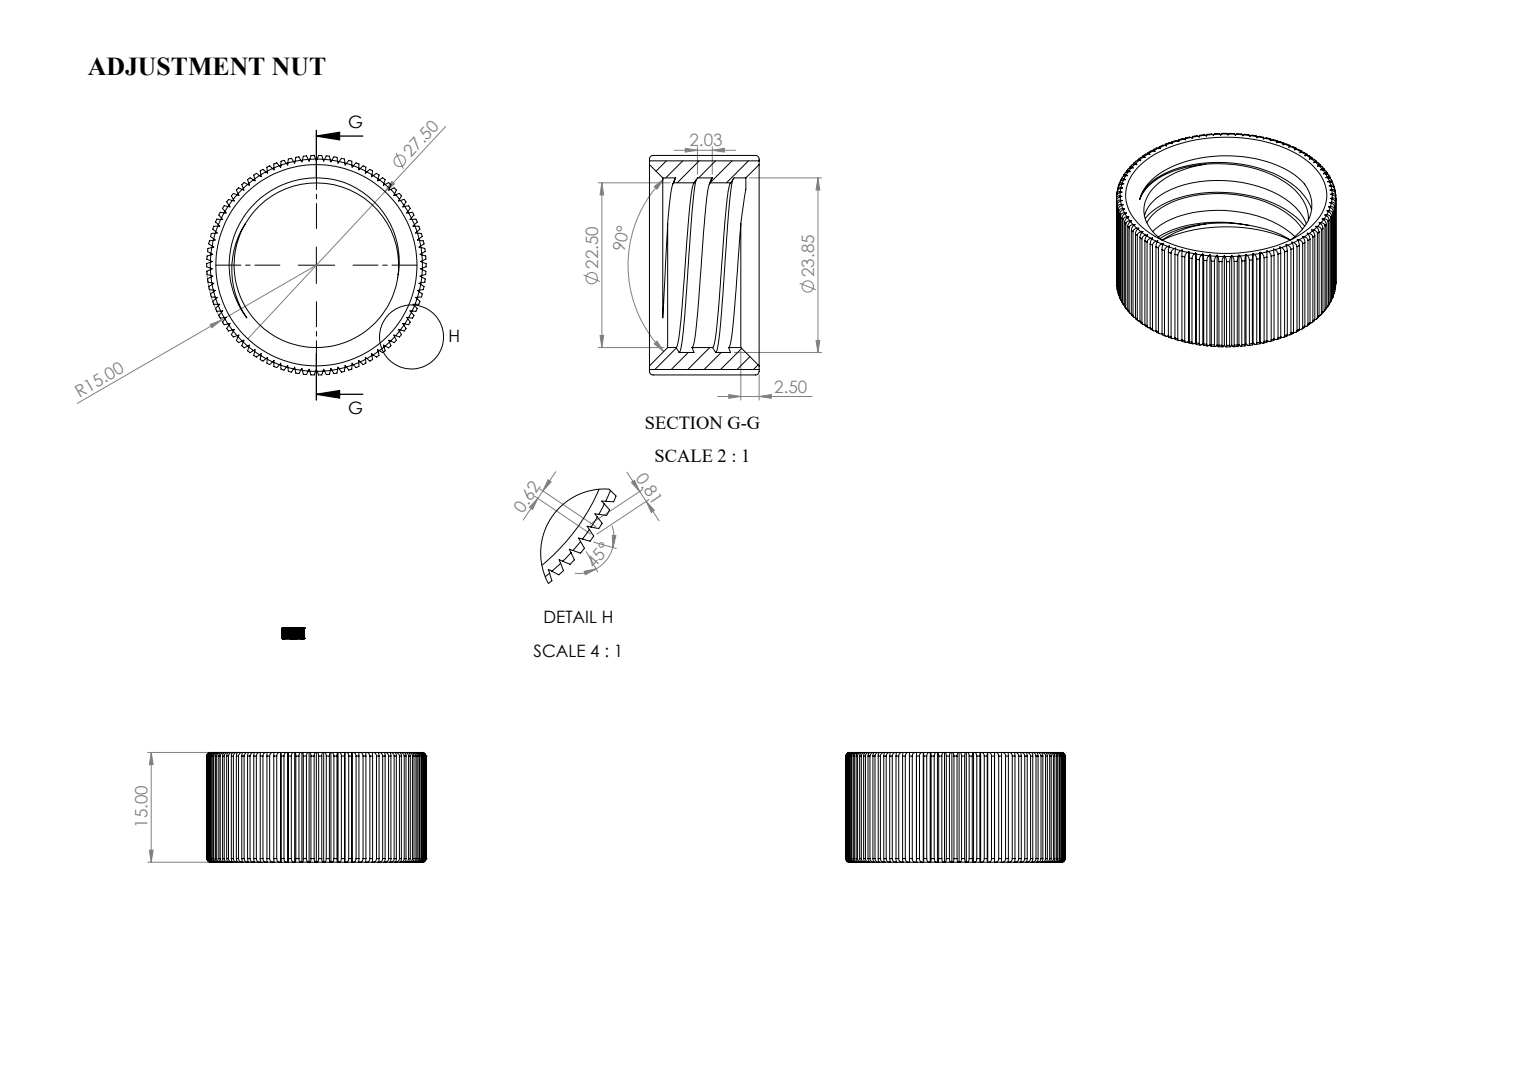
ISO-10303-21;
HEADER;
FILE_DESCRIPTION (('STEP AP214'),
    '1' );
FILE_NAME ('1.3 Adjustment Nut.step',
    '2026-10-07T05:30:18',
    ( '' ),
    ( '' ),
    'SwSTEP 2.0',
    'SolidWorks 2021',
    '' );
FILE_SCHEMA (( 'AUTOMOTIVE_DESIGN' ));
ENDSEC;

DATA;
#2=CARTESIAN_POINT ( 'NONE',  ( 14.03351048042397231, -0.03417435944610275333, -2.474486531753715024 ) ) ;
#4=CARTESIAN_POINT ( 'NONE',  ( 14.71525861348289865, 0.5000000000000004441, -2.908807992686582633 ) ) ;
#7=B_SPLINE_CURVE_WITH_KNOTS ( 'NONE', 3,
 ( #85792, #56757, #94261, #25787, #71286, #3780 ),
 .UNSPECIFIED., .F., .F.,
 ( 4, 2, 4 ),
 ( 0.0002800003243993068715, 0.0006862055569927260918, 0.001092410789586145421 ),
 .UNSPECIFIED. ) ;
#8=CARTESIAN_POINT ( 'NONE',  ( 7.082119434687054849, -1.529584498419354954, 12.26659068614894288 ) ) ;
#12=ORIENTED_EDGE ( 'NONE', *, *, #89075, .F. ) ;
#15=CARTESIAN_POINT ( 'NONE',  ( 1.915564264621432589, 3.914659629196372862E-16, -14.37291249357990530 ) ) ;
#20=DIRECTION ( 'NONE',  ( -0.000000000000000000, 1.000000000000000000, -0.000000000000000000 ) ) ;
#24=CARTESIAN_POINT ( 'NONE',  ( -10.88017736071110342, 33.06368534415485527, 3.903127820947815962E-15 ) ) ;
#31=ORIENTED_EDGE ( 'NONE', *, *, #54443, .T. ) ;
#32=EDGE_CURVE ( 'NONE', #89546, #61124, #1756, .T. ) ;
#33=VECTOR ( 'NONE', #15415, 1000.000000000000114 ) ;
#36=CARTESIAN_POINT ( 'NONE',  ( 0.000000000000000000, 0.000000000000000000, 0.000000000000000000 ) ) ;
#44=ORIENTED_EDGE ( 'NONE', *, *, #85385, .F. ) ;
#55=CARTESIAN_POINT ( 'NONE',  ( 5.361923921558577000, 0.000000000000000000, -0.9937738586171993571 ) ) ;
#57=CARTESIAN_POINT ( 'NONE',  ( -14.09394518620607606, 3.895088541583166744E-16, -3.407449058785548157 ) ) ;
#59=CARTESIAN_POINT ( 'NONE',  ( -14.35840480524194440, 15.00000000000000000, -4.340070442839038201 ) ) ;
#67=LINE ( 'NONE', #92990, #97116 ) ;
#68=FACE_OUTER_BOUND ( 'NONE', #36092, .T. ) ;
#73=ADVANCED_FACE ( 'NONE', ( #77721, #92241 ), #62222, .F. ) ;
#77=CARTESIAN_POINT ( 'NONE',  ( 8.527530157486175710, 13.92559781766745886, -4.923371831947298993 ) ) ;
#79=CARTESIAN_POINT ( 'NONE',  ( -6.715867195167276371, 15.00000000000000000, -12.85095824508335838 ) ) ;
#80=ORIENTED_EDGE ( 'NONE', *, *, #34109, .F. ) ;
#93=ORIENTED_EDGE ( 'NONE', *, *, #11884, .T. ) ;
#101=CIRCLE ( 'NONE', #95854, 15.00000000000000000 ) ;
#112=DIRECTION ( 'NONE',  ( 0.000000000000000000, 1.000000000000000000, 0.000000000000000000 ) ) ;
#117=CARTESIAN_POINT ( 'NONE',  ( -10.32896413005679648, 5.104976035794177136, 5.963430220938290560 ) ) ;
#127=ORIENTED_EDGE ( 'NONE', *, *, #93931, .T. ) ;
#135=DIRECTION ( 'NONE',  ( 0.000000000000000000, 0.000000000000000000, -1.000000000000000000 ) ) ;
#139=CARTESIAN_POINT ( 'NONE',  ( -10.88017736071110342, -6.936314655845155386, 3.903127820947815962E-15 ) ) ;
#141=CARTESIAN_POINT ( 'NONE',  ( 13.59972906620400401, 0.04962881387626714991, -5.718800721548577215 ) ) ;
#143=CARTESIAN_POINT ( 'NONE',  ( 11.29222593019770393, 14.76930270348882068, 9.783848334571327854 ) ) ;
#145=CARTESIAN_POINT ( 'NONE',  ( 1.460619146402132233E-15, 35.00000000000000000, 11.92686044187656513 ) ) ;
#154=AXIS2_PLACEMENT_3D ( 'NONE', #61355, #15392, #78324 ) ;
#166=DIRECTION ( 'NONE',  ( 0.000000000000000000, 1.000000000000000000, 0.000000000000000000 ) ) ;
#169=ORIENTED_EDGE ( 'NONE', *, *, #60294, .T. ) ;
#172=ADVANCED_FACE ( 'NONE', ( #58883 ), #90560, .T. ) ;
#181=LINE ( 'NONE', #61621, #10834 ) ;
#184=CARTESIAN_POINT ( 'NONE',  ( -8.527530157486182816, -29.40773551566588040, -4.923371831947288335 ) ) ;
#186=CARTESIAN_POINT ( 'NONE',  ( 0.2074183518478781019, 14.95123636042159454, -14.75075219811622773 ) ) ;
#187=CARTESIAN_POINT ( 'NONE',  ( 0.7375392941517235901, 0.5000000000000004441, 14.98185688723471110 ) ) ;
#189=VERTEX_POINT ( 'NONE', #73386 ) ;
#190=CARTESIAN_POINT ( 'NONE',  ( -0.8653096853335169314, -2.832054659144752395E-15, 14.59999144042650521 ) ) ;
#198=CARTESIAN_POINT ( 'NONE',  ( 12.81628187352647608, 21.41530133659708923, 3.434112377981052511 ) ) ;
#203=ORIENTED_EDGE ( 'NONE', *, *, #30154, .T. ) ;
#205=EDGE_CURVE ( 'NONE', #59600, #64703, #44234, .T. ) ;
#213=EDGE_CURVE ( 'NONE', #70990, #82368, #80902, .T. ) ;
#217=CARTESIAN_POINT ( 'NONE',  ( 0.7375392941518293943, 15.00000000000000000, -14.98185688723470932 ) ) ;
#219=CARTESIAN_POINT ( 'NONE',  ( -9.010802615327746068, 0.2301505768537817076, -11.91753657575794811 ) ) ;
#220=ORIENTED_EDGE ( 'NONE', *, *, #48530, .T. ) ;
#226=CARTESIAN_POINT ( 'NONE',  ( 0.000000000000000000, 15.00000000000000000, 0.000000000000000000 ) ) ;
#227=CARTESIAN_POINT ( 'NONE',  ( -14.15281240980449873, -3.182726299308032341E-15, 3.688687068602606089 ) ) ;
#230=DIRECTION ( 'NONE',  ( 0.000000000000000000, 1.000000000000000000, 0.000000000000000000 ) ) ;
#234=LINE ( 'NONE', #46200, #73516 ) ;
#241=DIRECTION ( 'NONE',  ( -0.2164396139381037087, 0.000000000000000000, 0.9762960071199331402 ) ) ;
#243=VERTEX_POINT ( 'NONE', #19901 ) ;
#248=LINE ( 'NONE', #13741, #50377 ) ;
#255=CARTESIAN_POINT ( 'NONE',  ( 14.16423886937410437, 14.09541550158063750, 3.795296366450304770 ) ) ;
#259=CARTESIAN_POINT ( 'NONE',  ( -10.17177286909477552, 0.2301502795151870728, 10.94336654633674399 ) ) ;
#260=AXIS2_PLACEMENT_3D ( 'NONE', #53452, #62422, #47430 ) ;
#264=B_SPLINE_CURVE_WITH_KNOTS ( 'NONE', 3,
 ( #34760, #66749, #89251, #97273, #64755, #95267 ),
 .UNSPECIFIED., .F., .F.,
 ( 4, 2, 4 ),
 ( 3.409110551496085967E-05, 0.0004400426677367861379, 0.0008459942299586114840 ),
 .UNSPECIFIED. ) ;
#269=ORIENTED_EDGE ( 'NONE', *, *, #30362, .T. ) ;
#275=CARTESIAN_POINT ( 'NONE',  ( -11.49658347684029813, 0.04962891477616592634, 9.245857368719700986 ) ) ;
#279=EDGE_LOOP ( 'NONE', ( #9235, #51853, #64977, #5678 ) ) ;
#282=CARTESIAN_POINT ( 'NONE',  ( 5.795997163830076460, -0.03417435944610275333, 13.01802277140709663 ) ) ;
#285=DIRECTION ( 'NONE',  ( -0.9999619230641714207, 0.000000000000000000, 0.008726535498367550894 ) ) ;
#290=CARTESIAN_POINT ( 'NONE',  ( 5.817157072110707539, 0.3640475087720986824, 13.82608706751091532 ) ) ;
#294=AXIS2_PLACEMENT_3D ( 'NONE', #67632, #98653, #53107 ) ;
#296=ORIENTED_EDGE ( 'NONE', *, *, #42464, .F. ) ;
#297=CARTESIAN_POINT ( 'NONE',  ( -14.73551000134586353, 0.04962893459885742153, 0.7225335126796733620 ) ) ;
#311=EDGE_CURVE ( 'NONE', #38139, #1776, #53773, .T. ) ;
#315=AXIS2_PLACEMENT_3D ( 'NONE', #61065, #112, #24072 ) ;
#316=ORIENTED_EDGE ( 'NONE', *, *, #50365, .T. ) ;
#318=ORIENTED_EDGE ( 'NONE', *, *, #77420, .F. ) ;
#323=ORIENTED_EDGE ( 'NONE', *, *, #6440, .F. ) ;
#325=VERTEX_POINT ( 'NONE', #97886 ) ;
#334=DIRECTION ( 'NONE',  ( -0.000000000000000000, -1.000000000000000000, -0.000000000000000000 ) ) ;
#339=VERTEX_POINT ( 'NONE', #7364 ) ;
#344=CARTESIAN_POINT ( 'NONE',  ( 7.684764310694891520, 14.49999999999999112, -12.88194075009941564 ) ) ;
#357=CARTESIAN_POINT ( 'NONE',  ( 12.21130863673200473, -3.098870037529856607E-15, 8.049375889233058246 ) ) ;
#364=CARTESIAN_POINT ( 'NONE',  ( -0.7575892234029697470, 0.2306972965111908358, -14.92193396517714099 ) ) ;
#368=EDGE_CURVE ( 'NONE', #36285, #1044, #68358, .T. ) ;
#370=B_SPLINE_CURVE_WITH_KNOTS ( 'NONE', 3,
 ( #59553, #52060, #6070, #61027, #30031, #36570 ),
 .UNSPECIFIED., .F., .F.,
 ( 4, 2, 4 ),
 ( 0.0002800267093156125989, 0.0006862322000234134670, 0.001092437690731214335 ),
 .UNSPECIFIED. ) ;
#373=CIRCLE ( 'NONE', #80196, 14.49999999999999822 ) ;
#380=PLANE ( 'NONE',  #76873 ) ;
#382=DIRECTION ( 'NONE',  ( 0.000000000000000000, 0.000000000000000000, 1.000000000000000000 ) ) ;
#389=EDGE_CURVE ( 'NONE', #33071, #18961, #10309, .T. ) ;
#392=DIRECTION ( 'NONE',  ( -0.9170600743851266001, 0.000000000000000000, 0.3987490689252404796 ) ) ;
#399=DIRECTION ( 'NONE',  ( 0.8870108331782213806, 0.000000000000000000, -0.4617486132350345773 ) ) ;
#405=LINE ( 'NONE', #8848, #3141 ) ;
#411=DIRECTION ( 'NONE',  ( 0.9537169507482300412, 0.000000000000000000, -0.3007057995042635157 ) ) ;
#414=AXIS2_PLACEMENT_3D ( 'NONE', #78877, #40404, #49357 ) ;
#436=ORIENTED_EDGE ( 'NONE', *, *, #19518, .T. ) ;
#438=CARTESIAN_POINT ( 'NONE',  ( 4.096035146093440993, 4.852245006323173772E-16, 13.90943910019262120 ) ) ;
#441=DIRECTION ( 'NONE',  ( -0.2503800040544453820, 0.000000000000000000, 0.9681476403781066331 ) ) ;
#443=CARTESIAN_POINT ( 'NONE',  ( 0.000000000000000000, 0.000000000000000000, 0.000000000000000000 ) ) ;
#446=AXIS2_PLACEMENT_3D ( 'NONE', #98952, #30408, #60911 ) ;
#460=EDGE_LOOP ( 'NONE', ( #79001, #10921, #93802, #41323 ) ) ;
#471=DIRECTION ( 'NONE',  ( 0.9537169507482238240, 0.000000000000000000, 0.3007057995042832221 ) ) ;
#483=CARTESIAN_POINT ( 'NONE',  ( -10.96178847474192075, 12.64502661508361214, -3.125209426587095329 ) ) ;
#489=CARTESIAN_POINT ( 'NONE',  ( -9.705452947461466806, 12.49999999999999289, -5.689172442861226031 ) ) ;
#492=EDGE_CURVE ( 'NONE', #47923, #47609, #86304, .T. ) ;
#501=CARTESIAN_POINT ( 'NONE',  ( 7.082119434687054849, -6.529584498419358951, 12.26659068614894288 ) ) ;
#502=VECTOR ( 'NONE', #65777, 1000.000000000000114 ) ;
#505=EDGE_CURVE ( 'NONE', #98966, #86629, #49108, .T. ) ;
#509=VECTOR ( 'NONE', #13114, 1000.000000000000000 ) ;
#512=CARTESIAN_POINT ( 'NONE',  ( 1.881645754503864953, -2.851112900457974152E-15, -14.50406564081096406 ) ) ;
#518=CARTESIAN_POINT ( 'NONE',  ( -6.728956594450633766, -2.083701050245576615E-16, -12.98689685418151640 ) ) ;
#527=CARTESIAN_POINT ( 'NONE',  ( 0.000000000000000000, 0.000000000000000000, 0.000000000000000000 ) ) ;
#536=CARTESIAN_POINT ( 'NONE',  ( 13.30119215211282047, 0.2301510699511992164, -6.804450086557198851 ) ) ;
#543=EDGE_CURVE ( 'NONE', #1556, #53389, #1840, .T. ) ;
#544=AXIS2_PLACEMENT_3D ( 'NONE', #93741, #61758, #9760 ) ;
#553=EDGE_CURVE ( 'NONE', #69641, #95502, #9313, .T. ) ;
#563=DIRECTION ( 'NONE',  ( -8.881784197001252323E-16, 0.000000000000000000, 1.000000000000000000 ) ) ;
#568=LINE ( 'NONE', #15061, #79560 ) ;
#571=CARTESIAN_POINT ( 'NONE',  ( -3.434112377981067610, -41.91803199673623936, -12.81628187352647252 ) ) ;
#572=ORIENTED_EDGE ( 'NONE', *, *, #57066, .F. ) ;
#574=ORIENTED_EDGE ( 'NONE', *, *, #38436, .F. ) ;
#584=AXIS2_PLACEMENT_3D ( 'NONE', #70041, #3034, #55528 ) ;
#587=VERTEX_POINT ( 'NONE', #25325 ) ;
#590=ORIENTED_EDGE ( 'NONE', *, *, #95067, .T. ) ;
#594=ADVANCED_FACE ( 'NONE', ( #47799 ), #2628, .T. ) ;
#602=ORIENTED_EDGE ( 'NONE', *, *, #96478, .F. ) ;
#604=ORIENTED_EDGE ( 'NONE', *, *, #21453, .F. ) ;
#605=ORIENTED_EDGE ( 'NONE', *, *, #79248, .F. ) ;
#606=CARTESIAN_POINT ( 'NONE',  ( -2.261421327065782805, 0.000000000000000000, 4.962236210031227834 ) ) ;
#607=CARTESIAN_POINT ( 'NONE',  ( 15.99538290524656503, 15.00000000000000000, 0.1584996864329874799 ) ) ;
#618=PLANE ( 'NONE',  #88836 ) ;
#623=ORIENTED_EDGE ( 'NONE', *, *, #11453, .T. ) ;
#630=DIRECTION ( 'NONE',  ( 0.000000000000000000, 1.000000000000000000, 0.000000000000000000 ) ) ;
#632=CARTESIAN_POINT ( 'NONE',  ( 7.313705784284644906, 14.49999999999999112, -13.09617149020747817 ) ) ;
#636=CARTESIAN_POINT ( 'NONE',  ( 5.440088680355549045, -8.602981322511817908, -9.422509992056141925 ) ) ;
#639=DIRECTION ( 'NONE',  ( 0.000000000000000000, 0.000000000000000000, 1.000000000000000000 ) ) ;
#640=CARTESIAN_POINT ( 'NONE',  ( -14.62617646268086524, 0.3639308321805994062, -3.327906561567071986 ) ) ;
#649=DIRECTION ( 'NONE',  ( 0.000000000000000000, 1.000000000000000000, 0.000000000000000000 ) ) ;
#675=CARTESIAN_POINT ( 'NONE',  ( -8.606322355891443010, 15.00000000000000000, 11.66967075398801335 ) ) ;
#678=CARTESIAN_POINT ( 'NONE',  ( -4.923371831947292776, -8.157735515665876846, 8.527530157486181039 ) ) ;
#691=CARTESIAN_POINT ( 'NONE',  ( 12.81628187352647608, 26.62363466993042493, -2.602085213965210642E-15 ) ) ;
#696=EDGE_LOOP ( 'NONE', ( #40227, #25908, #8282, #49239, #90855, #86389 ) ) ;
#704=EDGE_CURVE ( 'NONE', #20604, #37674, #29970, .T. ) ;
#705=CARTESIAN_POINT ( 'NONE',  ( 0.000000000000000000, 14.49999999999999822, 0.000000000000000000 ) ) ;
#706=CARTESIAN_POINT ( 'NONE',  ( -14.35840480524201190, 14.49999999999999112, -4.340070442839034648 ) ) ;
#712=CARTESIAN_POINT ( 'NONE',  ( -15.94536257719939698, 15.00000000000000000, -1.273895096820171657 ) ) ;
#714=AXIS2_PLACEMENT_3D ( 'NONE', #93061, #56067, #79045 ) ;
#719=CARTESIAN_POINT ( 'NONE',  ( -11.59580422753514384, 14.76984949557107640, -9.421229451860563486 ) ) ;
#723=FACE_OUTER_BOUND ( 'NONE', #60066, .T. ) ;
#735=CARTESIAN_POINT ( 'NONE',  ( 14.82269085861167390, 14.49999999999999822, 2.299529454047062327 ) ) ;
#741=CARTESIAN_POINT ( 'NONE',  ( 3.195792623639593266, 4.120456701841152203, 11.92686044187653494 ) ) ;
#746=CARTESIAN_POINT ( 'NONE',  ( 14.16423886937410082, 19.51208216824730712, -3.795296366450314096 ) ) ;
#749=CARTESIAN_POINT ( 'NONE',  ( 3.270351084886796933, 14.95037111082768000, -14.38617789677962655 ) ) ;
#755=DIRECTION ( 'NONE',  ( -0.000000000000000000, -1.000000000000000000, -0.000000000000000000 ) ) ;
#756=ORIENTED_EDGE ( 'NONE', *, *, #56154, .F. ) ;
#765=VERTEX_POINT ( 'NONE', #66241 ) ;
#781=CARTESIAN_POINT ( 'NONE',  ( 14.03351048042397231, 0.000000000000000000, -2.474486531753715024 ) ) ;
#787=LINE ( 'NONE', #31240, #15154 ) ;
#792=AXIS2_PLACEMENT_3D ( 'NONE', #36008, #73504, #34024 ) ;
#797=LINE ( 'NONE', #31249, #42721 ) ;
#798=ORIENTED_EDGE ( 'NONE', *, *, #95058, .F. ) ;
#804=CARTESIAN_POINT ( 'NONE',  ( -5.803070148808146200, 15.00000000000000000, -13.28812917035395813 ) ) ;
#807=CARTESIAN_POINT ( 'NONE',  ( 2.602060718268849104, 0.000000000000000000, -4.792399674598859072 ) ) ;
#808=VECTOR ( 'NONE', #6367, 1000.000000000000000 ) ;
#811=FACE_OUTER_BOUND ( 'NONE', #83164, .T. ) ;
#819=B_SPLINE_CURVE_WITH_KNOTS ( 'NONE', 3,
 ( #42826, #41374, #64319, #73311, #4834, #33813 ),
 .UNSPECIFIED., .F., .F.,
 ( 4, 2, 4 ),
 ( 0.0002800005319459006065, 0.0006862057665691816740, 0.001092411001192462741 ),
 .UNSPECIFIED. ) ;
#850=DIRECTION ( 'NONE',  ( 0.5664062369248313855, 0.000000000000000000, -0.8241261886220165866 ) ) ;
#853=CARTESIAN_POINT ( 'NONE',  ( 14.29730467489532408, 4.491438197698105257E-16, 2.416004766803315995 ) ) ;
#857=DIRECTION ( 'NONE',  ( 0.000000000000000000, 0.000000000000000000, 1.000000000000000000 ) ) ;
#858=CARTESIAN_POINT ( 'NONE',  ( 6.742022620658236320, 0.04962897188439623769, -13.12259272460504533 ) ) ;
#864=DIRECTION ( 'NONE',  ( 0.000000000000000000, 1.000000000000000000, -0.000000000000000000 ) ) ;
#865=STYLED_ITEM ( 'NONE', ( #71034 ), #8224 ) ;
#877=CARTESIAN_POINT ( 'NONE',  ( -14.93875075227008509, 0.2301502577613187550, -0.2365588874161651534 ) ) ;
#882=CARTESIAN_POINT ( 'NONE',  ( 9.519554572442958218, 15.00000000000000178, -11.10344954678180329 ) ) ;
#887=DIRECTION ( 'NONE',  ( 0.1650476058606741014, 0.000000000000000000, 0.9862856015372319929 ) ) ;
#907=ORIENTED_EDGE ( 'NONE', *, *, #41162, .F. ) ;
#921=ORIENTED_EDGE ( 'NONE', *, *, #98148, .F. ) ;
#930=EDGE_CURVE ( 'NONE', #78202, #91469, #93678, .T. ) ;
#931=AXIS2_PLACEMENT_3D ( 'NONE', #97642, #90596, #92936 ) ;
#933=CARTESIAN_POINT ( 'NONE',  ( -9.876730923139145801, 0.5000000000000004441, -11.28938378619076843 ) ) ;
#934=EDGE_CURVE ( 'NONE', #70902, #7776, #71189, .T. ) ;
#935=VERTEX_POINT ( 'NONE', #12147 ) ;
#949=CARTESIAN_POINT ( 'NONE',  ( 12.25993886608599759, 0.3640475087720986269, 8.642563219313707634 ) ) ;
#952=VERTEX_POINT ( 'NONE', #4168 ) ;
#953=CARTESIAN_POINT ( 'NONE',  ( 2.863771337576527021, 0.04962896698837649528, -14.47259902956229283 ) ) ;
#960=ADVANCED_FACE ( 'NONE', ( #34637 ), #97527, .T. ) ;
#966=CARTESIAN_POINT ( 'NONE',  ( -8.235571585149862983, 10.74303362898264602, 8.235571585149875418 ) ) ;
#975=CARTESIAN_POINT ( 'NONE',  ( 14.16423886937410082, -5.487917831752695541, -3.795296366450314096 ) ) ;
#984=CARTESIAN_POINT ( 'NONE',  ( 0.000000000000000000, 15.00000000000000000, -11.25000000000000178 ) ) ;
#986=CARTESIAN_POINT ( 'NONE',  ( 7.154372922009559765, -0.03417435944610275333, -14.30707323420376831 ) ) ;
#1000=DIRECTION ( 'NONE',  ( -0.9426414910921759871, 0.000000000000000000, -0.3338068592337775642 ) ) ;
#1010=CARTESIAN_POINT ( 'NONE',  ( 13.16767742306216604, 0.04962884061926501472, -6.653539137814636462 ) ) ;
#1011=CARTESIAN_POINT ( 'NONE',  ( 0.000000000000000000, 0.000000000000000000, 0.000000000000000000 ) ) ;
#1013=ORIENTED_EDGE ( 'NONE', *, *, #57799, .T. ) ;
#1021=DIRECTION ( 'NONE',  ( -0.02617694830787627158, 0.000000000000000000, 0.9996573249755572599 ) ) ;
#1023=VERTEX_POINT ( 'NONE', #50645 ) ;
#1024=CIRCLE ( 'NONE', #98383, 15.00000000000000000 ) ;
#1027=LINE ( 'NONE', #92490, #16884 ) ;
#1042=CARTESIAN_POINT ( 'NONE',  ( -4.923371831947302546, 30.17559781766745886, -8.527530157486173934 ) ) ;
#1043=EDGE_LOOP ( 'NONE', ( #66084, #36581, #93814, #49851, #67190, #80121 ) ) ;
#1044=VERTEX_POINT ( 'NONE', #73627 ) ;
#1052=ORIENTED_EDGE ( 'NONE', *, *, #1534, .F. ) ;
#1057=EDGE_LOOP ( 'NONE', ( #46401, #67806, #92729, #95178, #5184, #32431 ) ) ;
#1062=B_SPLINE_CURVE_WITH_KNOTS ( 'NONE', 3,
 ( #33138, #63633, #11628, #71651, #19621, #50115 ),
 .UNSPECIFIED., .F., .F.,
 ( 4, 2, 4 ),
 ( 0.0002800452451301727584, 0.0006862509172429725589, 0.001092456589355772414 ),
 .UNSPECIFIED. ) ;
#1073=ORIENTED_EDGE ( 'NONE', *, *, #35562, .F. ) ;
#1074=AXIS2_PLACEMENT_3D ( 'NONE', #31900, #47402, #86886 ) ;
#1077=EDGE_LOOP ( 'NONE', ( #4944, #29200, #60589, #70264, #59437, #51331 ) ) ;
#1082=EDGE_CURVE ( 'NONE', #46208, #94458, #57424, .T. ) ;
#1085=DIRECTION ( 'NONE',  ( 0.000000000000000000, 0.000000000000000000, 1.000000000000000000 ) ) ;
#1089=ORIENTED_EDGE ( 'NONE', *, *, #45048, .F. ) ;
#1094=CARTESIAN_POINT ( 'NONE',  ( 7.618485323809272458, 15.00000000000000888, -12.48587314215760458 ) ) ;
#1099=EDGE_LOOP ( 'NONE', ( #77070, #42549, #66446, #65909, #31655, #89303 ) ) ;
#1111=CARTESIAN_POINT ( 'NONE',  ( 9.422509992056141925, 0.1470186774881754310, 5.440088680355547268 ) ) ;
#1114=CARTESIAN_POINT ( 'NONE',  ( 4.862001128006775197, 15.00000000000000000, -13.66056166602457367 ) ) ;
#1116=DIRECTION ( 'NONE',  ( 0.000000000000000000, 1.000000000000000000, 0.000000000000000000 ) ) ;
#1122=CARTESIAN_POINT ( 'NONE',  ( 8.209432707284918251, 14.49999999999999112, -12.55409154915490255 ) ) ;
#1132=CARTESIAN_POINT ( 'NONE',  ( -12.58781651029209492, -3.178914651045387989E-15, 7.446837378630629445 ) ) ;
#1138=CARTESIAN_POINT ( 'NONE',  ( 0.000000000000000000, 0.000000000000000000, 0.000000000000000000 ) ) ;
#1140=VECTOR ( 'NONE', #36904, 1000.000000000000000 ) ;
#1141=EDGE_CURVE ( 'NONE', #84500, #74647, #63450, .T. ) ;
#1143=CARTESIAN_POINT ( 'NONE',  ( 5.806616290881413178, -3.171291354520099286E-15, -13.42355087257362278 ) ) ;
#1145=AXIS2_PLACEMENT_3D ( 'NONE', #11568, #56586, #78594 ) ;
#1146=VERTEX_POINT ( 'NONE', #6136 ) ;
#1159=DIRECTION ( 'NONE',  ( -0.7604059656000340395, 0.000000000000000000, 0.6494480483301799945 ) ) ;
#1161=CARTESIAN_POINT ( 'NONE',  ( 3.469446951953614189E-15, -12.74106884899921255, 9.846743663894594434 ) ) ;
#1162=VERTEX_POINT ( 'NONE', #38126 ) ;
#1163=FACE_OUTER_BOUND ( 'NONE', #27124, .T. ) ;
#1164=EDGE_LOOP ( 'NONE', ( #40551, #53847, #17244, #68763 ) ) ;
#1165=AXIS2_PLACEMENT_3D ( 'NONE', #34895, #57889, #50892 ) ;
#1166=FACE_OUTER_BOUND ( 'NONE', #61543, .T. ) ;
#1167=EDGE_CURVE ( 'NONE', #65699, #33104, #6078, .T. ) ;
#1178=ADVANCED_FACE ( 'NONE', ( #20644 ), #36125, .F. ) ;
#1179=VERTEX_POINT ( 'NONE', #14643 ) ;
#1182=EDGE_LOOP ( 'NONE', ( #21964, #53207, #68054, #84302 ) ) ;
#1192=FACE_OUTER_BOUND ( 'NONE', #20968, .T. ) ;
#1195=CARTESIAN_POINT ( 'NONE',  ( 9.065164099344512394, 14.49999999999999112, 11.95084933600776722 ) ) ;
#1197=FACE_OUTER_BOUND ( 'NONE', #80893, .T. ) ;
#1198=ORIENTED_EDGE ( 'NONE', *, *, #54099, .T. ) ;
#1199=EDGE_CURVE ( 'NONE', #67320, #77856, #28630, .T. ) ;
#1205=EDGE_CURVE ( 'NONE', #2423, #23291, #59166, .T. ) ;
#1206=CARTESIAN_POINT ( 'NONE',  ( -14.24131928502211863, 15.00000000000000000, 0.4973178280104966764 ) ) ;
#1207=VECTOR ( 'NONE', #86265, 1000.000000000000000 ) ;
#1208=VERTEX_POINT ( 'NONE', #30098 ) ;
#1210=FACE_OUTER_BOUND ( 'NONE', #79066, .T. ) ;
#1219=VECTOR ( 'NONE', #42137, 1000.000000000000114 ) ;
#1224=ORIENTED_EDGE ( 'NONE', *, *, #61317, .F. ) ;
#1225=CARTESIAN_POINT ( 'NONE',  ( -8.375939845167600595, -0.03417435944610275333, -11.52849216984310310 ) ) ;
#1229=DIRECTION ( 'NONE',  ( 1.776356839400250780E-14, 0.000000000000000000, 1.000000000000000000 ) ) ;
#1230=CARTESIAN_POINT ( 'NONE',  ( -7.684764310694971456, 0.5000000000000004441, 12.88194075009929840 ) ) ;
#1231=CARTESIAN_POINT ( 'NONE',  ( 3.195792623639528873, 6.203790035174478135, -11.92686044187656513 ) ) ;
#1236=CARTESIAN_POINT ( 'NONE',  ( -10.36894250292378317, 32.42874883491396076, 10.36894250292379560 ) ) ;
#1245=ORIENTED_EDGE ( 'NONE', *, *, #9371, .T. ) ;
#1250=DIRECTION ( 'NONE',  ( 0.000000000000000000, 0.000000000000000000, 1.000000000000000000 ) ) ;
#1251=CARTESIAN_POINT ( 'NONE',  ( 0.000000000000000000, 15.00000000000000000, 0.000000000000000000 ) ) ;
#1262=AXIS2_PLACEMENT_3D ( 'NONE', #21741, #97750, #29215 ) ;
#1274=ORIENTED_EDGE ( 'NONE', *, *, #47851, .F. ) ;
#1275=ORIENTED_EDGE ( 'NONE', *, *, #42360, .T. ) ;
#1276=DIRECTION ( 'NONE',  ( 0.000000000000000000, 1.000000000000000000, 0.000000000000000000 ) ) ;
#1293=CARTESIAN_POINT ( 'NONE',  ( -14.47650479471830387, 14.49999999999999112, 3.928206833721953561 ) ) ;
#1294=ORIENTED_EDGE ( 'NONE', *, *, #27831, .T. ) ;
#1297=ORIENTED_EDGE ( 'NONE', *, *, #81961, .T. ) ;
#1302=VERTEX_POINT ( 'NONE', #29114 ) ;
#1305=EDGE_CURVE ( 'NONE', #76195, #10376, #22926, .T. ) ;
#1307=EDGE_CURVE ( 'NONE', #94129, #86936, #40796, .T. ) ;
#1310=ORIENTED_EDGE ( 'NONE', *, *, #27596, .T. ) ;
#1314=CARTESIAN_POINT ( 'NONE',  ( 14.16722289976681814, 0.5000000000000004441, 4.928467845925615265 ) ) ;
#1318=ORIENTED_EDGE ( 'NONE', *, *, #78245, .F. ) ;
#1322=CARTESIAN_POINT ( 'NONE',  ( -1.354709868695727959, 0.3640475087720941305, 14.93870011653151231 ) ) ;
#1324=CARTESIAN_POINT ( 'NONE',  ( 11.75249112336553381, 0.04962895880866900755, 8.918310463590511716 ) ) ;
#1330=PLANE ( 'NONE',  #13321 ) ;
#1334=DIRECTION ( 'NONE',  ( 0.1822355254921578516, 0.000000000000000000, -0.9832549075639526182 ) ) ;
#1346=CARTESIAN_POINT ( 'NONE',  ( 0.000000000000000000, 0.5000000000000004441, 0.000000000000000000 ) ) ;
#1355=CIRCLE ( 'NONE', #90757, 15.00000000000000000 ) ;
#1356=CARTESIAN_POINT ( 'NONE',  ( -5.795997163829992083, -0.03417435944610275333, -13.01802277140713926 ) ) ;
#1357=VECTOR ( 'NONE', #75041, 1000.000000000000114 ) ;
#1362=ORIENTED_EDGE ( 'NONE', *, *, #16997, .T. ) ;
#1366=CARTESIAN_POINT ( 'NONE',  ( 4.431036607602471200, 14.63595249122791131, 14.33059365769914173 ) ) ;
#1372=VERTEX_POINT ( 'NONE', #7635 ) ;
#1373=CARTESIAN_POINT ( 'NONE',  ( 0.7166339456633684657, 15.00000000000000000, -15.98010739087745868 ) ) ;
#1387=EDGE_CURVE ( 'NONE', #78530, #49977, #45607, .T. ) ;
#1391=LINE ( 'NONE', #31846, #2543 ) ;
#1400=ORIENTED_EDGE ( 'NONE', *, *, #12642, .F. ) ;
#1407=EDGE_LOOP ( 'NONE', ( #82520, #59091, #75364, #18143 ) ) ;
#1410=EDGE_CURVE ( 'NONE', #51188, #59403, #75116, .T. ) ;
#1425=DIRECTION ( 'NONE',  ( -0.000000000000000000, -1.000000000000000000, -0.000000000000000000 ) ) ;
#1431=CARTESIAN_POINT ( 'NONE',  ( -9.641450013144313047, 0.04962892333243928977, -11.16690429682362407 ) ) ;
#1436=VERTEX_POINT ( 'NONE', #60103 ) ;
#1437=EDGE_CURVE ( 'NONE', #63858, #63123, #76557, .T. ) ;
#1441=CARTESIAN_POINT ( 'NONE',  ( 10.64017930668209466, 14.63606904708525747, -10.57291749337217368 ) ) ;
#1444=FACE_OUTER_BOUND ( 'NONE', #61728, .T. ) ;
#1446=VECTOR ( 'NONE', #14096, 1000.000000000000114 ) ;
#1450=VERTEX_POINT ( 'NONE', #71076 ) ;
#1456=CARTESIAN_POINT ( 'NONE',  ( -14.11874224319634763, 0.2301510088455466507, 4.887061453529934596 ) ) ;
#1471=CARTESIAN_POINT ( 'NONE',  ( 3.795296366450306547, -4.654584498419360727, -14.16423886937410259 ) ) ;
#1475=VERTEX_POINT ( 'NONE', #31088 ) ;
#1477=CARTESIAN_POINT ( 'NONE',  ( -4.792102989642738287, -0.03417435944610275333, -15.26149223938179134 ) ) ;
#1478=LINE ( 'NONE', #16961, #22770 ) ;
#1497=CIRCLE ( 'NONE', #4696, 14.49999999999999822 ) ;
#1503=B_SPLINE_CURVE_WITH_KNOTS ( 'NONE', 3,
 ( #37866, #6860, #858, #15368, #76338, #23356 ),
 .UNSPECIFIED., .F., .F.,
 ( 4, 2, 4 ),
 ( 0.0002800011564896236595, 0.0006862063972211524237, 0.001092411637952681296 ),
 .UNSPECIFIED. ) ;
#1507=B_SPLINE_CURVE_WITH_KNOTS ( 'NONE', 3,
 ( #54219, #55204, #84735, #8248, #69247, #85718 ),
 .UNSPECIFIED., .F., .F.,
 ( 4, 2, 4 ),
 ( 0.0002800026249563192867, 0.0006862078800502534673, 0.001092413135144187485 ),
 .UNSPECIFIED. ) ;
#1515=EDGE_LOOP ( 'NONE', ( #41990, #18383, #25113, #84572 ) ) ;
#1516=CARTESIAN_POINT ( 'NONE',  ( 3.866399090317181653, 0.04922511925147171619, 14.23717170745775107 ) ) ;
#1523=DIRECTION ( 'NONE',  ( 0.1822355254921448342, -0.000000000000000000, 0.9832549075639550606 ) ) ;
#1525=ORIENTED_EDGE ( 'NONE', *, *, #93455, .T. ) ;
#1526=CARTESIAN_POINT ( 'NONE',  ( 0.000000000000000000, 15.00000000000000000, 0.000000000000000000 ) ) ;
#1534=EDGE_CURVE ( 'NONE', #10597, #8161, #55979, .T. ) ;
#1545=CARTESIAN_POINT ( 'NONE',  ( -3.469446951953614189E-15, 29.75893115100078390, -9.846743663894594434 ) ) ;
#1554=TOROIDAL_SURFACE ( 'NONE', #49394, 14.49999999999999822, 0.5000000000000000000 ) ;
#1556=VERTEX_POINT ( 'NONE', #77571 ) ;
#1561=VERTEX_POINT ( 'NONE', #39601 ) ;
#1566=CARTESIAN_POINT ( 'NONE',  ( -10.19513985507818177, 0.3640475087720994041, -11.00268709613231977 ) ) ;
#1567=EDGE_CURVE ( 'NONE', #22543, #76539, #36838, .T. ) ;
#1570=ORIENTED_EDGE ( 'NONE', *, *, #53671, .F. ) ;
#1579=LINE ( 'NONE', #33027, #36213 ) ;
#1580=LINE ( 'NONE', #93040, #88114 ) ;
#1584=ORIENTED_EDGE ( 'NONE', *, *, #76121, .F. ) ;
#1587=VECTOR ( 'NONE', #22324, 1000.000000000000000 ) ;
#1590=CARTESIAN_POINT ( 'NONE',  ( 7.640917710489005366, 14.95077488074853456, -12.61992379908754458 ) ) ;
#1592=CARTESIAN_POINT ( 'NONE',  ( -6.189644032515865035, 0.04922511925147087658, 13.39157970158793276 ) ) ;
#1594=ORIENTED_EDGE ( 'NONE', *, *, #90193, .F. ) ;
#1605=DIRECTION ( 'NONE',  ( -0.000000000000000000, -1.000000000000000000, -0.000000000000000000 ) ) ;
#1606=CIRCLE ( 'NONE', #6355, 14.49999999999999822 ) ;
#1609=CARTESIAN_POINT ( 'NONE',  ( -9.422509992056136596, -1.519647989178487979, 5.440088680355559703 ) ) ;
#1619=DIRECTION ( 'NONE',  ( -0.000000000000000000, -1.000000000000000000, -0.000000000000000000 ) ) ;
#1620=CARTESIAN_POINT ( 'NONE',  ( 11.92686044187655980, 12.39664270246084676, -3.195792623639533314 ) ) ;
#1622=EDGE_CURVE ( 'NONE', #36305, #50106, #94278, .T. ) ;
#1626=CARTESIAN_POINT ( 'NONE',  ( 9.383624259804085099, 0.2301501999354983174, -11.62625599701879509 ) ) ;
#1628=ORIENTED_EDGE ( 'NONE', *, *, #70114, .F. ) ;
#1631=CARTESIAN_POINT ( 'NONE',  ( -12.83294900548071205, 0.3639312116172442879, 7.766300266068302705 ) ) ;
#1650=B_SPLINE_CURVE_WITH_KNOTS ( 'NONE', 3,
 ( #92412, #93890, #85907, #25418, #40902, #2919 ),
 .UNSPECIFIED., .F., .F.,
 ( 4, 2, 4 ),
 ( 0.0002800075630785962052, 0.0006862128664728917634, 0.001092418169867187322 ),
 .UNSPECIFIED. ) ;
#1653=FACE_OUTER_BOUND ( 'NONE', #20086, .T. ) ;
#1656=CARTESIAN_POINT ( 'NONE',  ( 4.923371831947301658, -12.32440218233254292, 8.527530157486175710 ) ) ;
#1657=ORIENTED_EDGE ( 'NONE', *, *, #930, .T. ) ;
#1658=CYLINDRICAL_SURFACE ( 'NONE', #12376, 15.00000000000000000 ) ;
#1659=ORIENTED_EDGE ( 'NONE', *, *, #52501, .T. ) ;
#1660=FACE_OUTER_BOUND ( 'NONE', #3950, .T. ) ;
#1661=VECTOR ( 'NONE', #96367, 1000.000000000000000 ) ;
#1662=ORIENTED_EDGE ( 'NONE', *, *, #74034, .F. ) ;
#1672=ORIENTED_EDGE ( 'NONE', *, *, #41805, .F. ) ;
#1676=AXIS2_PLACEMENT_3D ( 'NONE', #76704, #7236, #53220 ) ;
#1680=CARTESIAN_POINT ( 'NONE',  ( 10.39655283154076848, 14.95077488074853456, 10.46698568711271093 ) ) ;
#1683=B_SPLINE_CURVE_WITH_KNOTS ( 'NONE', 3,
 ( #94947, #20440, #87450, #88930, #57928, #73423 ),
 .UNSPECIFIED., .F., .F.,
 ( 4, 2, 4 ),
 ( 3.409110551495869127E-05, 0.0004400426677367973052, 0.0008459942299586359869 ),
 .UNSPECIFIED. ) ;
#1687=ORIENTED_EDGE ( 'NONE', *, *, #24059, .T. ) ;
#1692=CARTESIAN_POINT ( 'NONE',  ( 14.47650479471822216, 0.5000000000000004441, -3.928206833722012625 ) ) ;
#1705=VERTEX_POINT ( 'NONE', #76594 ) ;
#1707=DIRECTION ( 'NONE',  ( -0.9914448613738113814, 0.000000000000000000, 0.1305261922200445512 ) ) ;
#1714=CARTESIAN_POINT ( 'NONE',  ( -9.159723438033276821, 0.000000000000000000, 10.91613331444536250 ) ) ;
#1715=VECTOR ( 'NONE', #13530, 1000.000000000000000 ) ;
#1720=CARTESIAN_POINT ( 'NONE',  ( 2.915334737309928315, -35.47798132251182324, 10.88017736071109987 ) ) ;
#1733=ORIENTED_EDGE ( 'NONE', *, *, #95525, .T. ) ;
#1740=EDGE_CURVE ( 'NONE', #77207, #79612, #51888, .T. ) ;
#1744=ORIENTED_EDGE ( 'NONE', *, *, #48499, .F. ) ;
#1745=CARTESIAN_POINT ( 'NONE',  ( 12.83294900548063744, 0.5000000000000004441, -7.766300266068363101 ) ) ;
#1746=CARTESIAN_POINT ( 'NONE',  ( 0.000000000000000000, 0.000000000000000000, 0.000000000000000000 ) ) ;
#1756=LINE ( 'NONE', #53749, #85727 ) ;
#1757=VERTEX_POINT ( 'NONE', #35887 ) ;
#1759=AXIS2_PLACEMENT_3D ( 'NONE', #38100, #97133, #68094 ) ;
#1761=DIRECTION ( 'NONE',  ( -0.5224985647159612334, -0.000000000000000000, 0.8526401643540847397 ) ) ;
#1767=CARTESIAN_POINT ( 'NONE',  ( 0.000000000000000000, 0.5000000000000004441, 0.000000000000000000 ) ) ;
#1770=DIRECTION ( 'NONE',  ( 0.000000000000000000, 0.000000000000000000, 1.000000000000000000 ) ) ;
#1776=VERTEX_POINT ( 'NONE', #64034 ) ;
#1780=VERTEX_POINT ( 'NONE', #21394 ) ;
#1788=CARTESIAN_POINT ( 'NONE',  ( 14.75001642003105395, 0.04962894700187066993, 0.3071237627330382636 ) ) ;
#1789=CARTESIAN_POINT ( 'NONE',  ( -6.408140936763246032, -6.709698663402908991, -11.09922568453594316 ) ) ;
#1790=ORIENTED_EDGE ( 'NONE', *, *, #67877, .F. ) ;
#1792=VECTOR ( 'NONE', #20290, 1000.000000000000000 ) ;
#1802=ORIENTED_EDGE ( 'NONE', *, *, #84904, .T. ) ;
#1810=EDGE_CURVE ( 'NONE', #65059, #16083, #5417, .T. ) ;
#1822=EDGE_CURVE ( 'NONE', #51220, #2779, #49053, .T. ) ;
#1840=LINE ( 'NONE', #10798, #58539 ) ;
#1847=ADVANCED_FACE ( 'NONE', ( #82370 ), #1554, .T. ) ;
#1848=CARTESIAN_POINT ( 'NONE',  ( -15.41943733314634635, -0.03417435944610275333, 4.256565371896233962 ) ) ;
#1851=DIRECTION ( 'NONE',  ( -0.4771587602596096822, 0.000000000000000000, 0.8788171126619647167 ) ) ;
#1854=CARTESIAN_POINT ( 'NONE',  ( -8.564643372776448160, 0.5000000000000004441, -12.31449893000752205 ) ) ;
#1861=ORIENTED_EDGE ( 'NONE', *, *, #32, .T. ) ;
#1863=CARTESIAN_POINT ( 'NONE',  ( 0.000000000000000000, 0.5000000000000004441, 0.000000000000000000 ) ) ;
#1868=CARTESIAN_POINT ( 'NONE',  ( -0.9082943533635161604, 4.683954948888111413E-16, -14.47152380945586359 ) ) ;
#1869=CARTESIAN_POINT ( 'NONE',  ( -1.983216688681034068, 15.00000000000000000, 14.11131997956736406 ) ) ;
#1873=CARTESIAN_POINT ( 'NONE',  ( 5.419894505350487002, 0.5000000000000004441, 13.98659156302462314 ) ) ;
#1874=AXIS2_PLACEMENT_3D ( 'NONE', #4581, #86104, #3112 ) ;
#1884=CARTESIAN_POINT ( 'NONE',  ( 0.000000000000000000, 15.00000000000000000, 0.000000000000000000 ) ) ;
#1897=AXIS2_PLACEMENT_3D ( 'NONE', #81738, #73253, #28746 ) ;
#1901=VERTEX_POINT ( 'NONE', #73886 ) ;
#1924=ORIENTED_EDGE ( 'NONE', *, *, #27259, .T. ) ;
#1935=CARTESIAN_POINT ( 'NONE',  ( -13.95692576442123034, 0.2301500530278518253, -5.331646315825927296 ) ) ;
#1940=DIRECTION ( 'NONE',  ( 0.000000000000000000, 1.000000000000000000, 0.000000000000000000 ) ) ;
#1943=DIRECTION ( 'NONE',  ( -0.9588197348681947174, 0.000000000000000000, 0.2840153447039170387 ) ) ;
#1948=DIRECTION ( 'NONE',  ( 0.000000000000000000, 1.000000000000000000, 0.000000000000000000 ) ) ;
#1955=CARTESIAN_POINT ( 'NONE',  ( 13.61912076658542325, 15.00000000000000888, 5.334594295380997053 ) ) ;
#1962=CARTESIAN_POINT ( 'NONE',  ( -7.082119434687044190, -2.362917831752693765, 12.26659068614894998 ) ) ;
#1964=PLANE ( 'NONE',  #68910 ) ;
#1965=AXIS2_PLACEMENT_3D ( 'NONE', #90045, #52540, #82549 ) ;
#1969=DIRECTION ( 'NONE',  ( 0.04361938736534638067, 0.000000000000000000, -0.9990482215818573541 ) ) ;
#1970=CARTESIAN_POINT ( 'NONE',  ( 1.780824192092501423, 0.5000000000000004441, -14.89391369643513485 ) ) ;
#1971=CARTESIAN_POINT ( 'NONE',  ( -5.991992585808429972, 15.00000000000000000, -13.20401548210301357 ) ) ;
#1974=EDGE_CURVE ( 'NONE', #13755, #54264, #90903, .T. ) ;
#1998=AXIS2_PLACEMENT_3D ( 'NONE', #63257, #93765, #25292 ) ;
#2003=ORIENTED_EDGE ( 'NONE', *, *, #2547, .F. ) ;
#2015=CARTESIAN_POINT ( 'NONE',  ( 12.00809552683958614, 0.5000000000000004441, -8.989195838243546177 ) ) ;
#2016=EDGE_CURVE ( 'NONE', #38851, #45156, #79036, .T. ) ;
#2019=VECTOR ( 'NONE', #11768, 999.9999999999998863 ) ;
#2020=ORIENTED_EDGE ( 'NONE', *, *, #74478, .T. ) ;
#2027=CARTESIAN_POINT ( 'NONE',  ( -9.402796353260987061, 14.49999999999999112, -11.68706210897776465 ) ) ;
#2034=AXIS2_PLACEMENT_3D ( 'NONE', #76436, #7952, #38447 ) ;
#2036=CARTESIAN_POINT ( 'NONE',  ( -4.923371831947302546, 25.17559781766745530, -8.527530157486173934 ) ) ;
#2037=EDGE_LOOP ( 'NONE', ( #97126, #36813, #40941, #13080 ) ) ;
#2046=CIRCLE ( 'NONE', #96235, 14.49999999999999822 ) ;
#2048=ORIENTED_EDGE ( 'NONE', *, *, #64961, .T. ) ;
#2058=EDGE_CURVE ( 'NONE', #58154, #8981, #69489, .T. ) ;
#2063=VECTOR ( 'NONE', #88908, 1000.000000000000000 ) ;
#2065=LINE ( 'NONE', #63025, #37451 ) ;
#2068=ORIENTED_EDGE ( 'NONE', *, *, #24511, .F. ) ;
#2077=CARTESIAN_POINT ( 'NONE',  ( 13.82671409943293739, -0.03417435944610275333, 3.447387012295318076 ) ) ;
#2089=EDGE_CURVE ( 'NONE', #62241, #76019, #83370, .T. ) ;
#2090=EDGE_LOOP ( 'NONE', ( #32914, #87501, #15357, #45766, #28426, #93141 ) ) ;
#2091=ORIENTED_EDGE ( 'NONE', *, *, #77384, .F. ) ;
#2104=CARTESIAN_POINT ( 'NONE',  ( 10.88017736071110164, 0.3553520108215071915, 2.915334737309921209 ) ) ;
#2110=DIRECTION ( 'NONE',  ( 3.375077994860475883E-14, 0.000000000000000000, 1.000000000000000000 ) ) ;
#2114=CARTESIAN_POINT ( 'NONE',  ( -11.62719953690074881, 14.49999999999999112, 9.476720473301769587 ) ) ;
#2115=CARTESIAN_POINT ( 'NONE',  ( 5.963430220938279902, 13.02164270246083966, -10.32896413005680181 ) ) ;
#2122=VERTEX_POINT ( 'NONE', #45871 ) ;
#2134=EDGE_CURVE ( 'NONE', #92052, #81238, #82877, .T. ) ;
#2135=CARTESIAN_POINT ( 'NONE',  ( 5.803070148808322948, 4.011383936018713867E-16, -13.28812917035388175 ) ) ;
#2136=DIRECTION ( 'NONE',  ( 0.000000000000000000, 1.000000000000000000, 0.000000000000000000 ) ) ;
#2138=ORIENTED_EDGE ( 'NONE', *, *, #4766, .T. ) ;
#2149=CARTESIAN_POINT ( 'NONE',  ( 0.000000000000000000, 15.00000000000000000, 0.000000000000000000 ) ) ;
#2153=CARTESIAN_POINT ( 'NONE',  ( -2.638427012816824124, -7.949402182332544697, 9.846743663894596210 ) ) ;
#2155=ORIENTED_EDGE ( 'NONE', *, *, #40456, .T. ) ;
#2158=EDGE_LOOP ( 'NONE', ( #70563, #51808, #69008, #45306, #49863, #97582 ) ) ;
#2159=DIRECTION ( 'NONE',  ( 0.000000000000000000, 0.000000000000000000, 1.000000000000000000 ) ) ;
#2160=ORIENTED_EDGE ( 'NONE', *, *, #16954, .T. ) ;
#2165=DIRECTION ( 'NONE',  ( -0.09584575252021386438, 0.000000000000000000, -0.9953961983671798519 ) ) ;
#2166=CARTESIAN_POINT ( 'NONE',  ( 8.439016546559898302, 4.734672723634894724E-16, -11.79122553964973541 ) ) ;
#2168=ORIENTED_EDGE ( 'NONE', *, *, #97101, .T. ) ;
#2170=ORIENTED_EDGE ( 'NONE', *, *, #68560, .F. ) ;
#2180=AXIS2_PLACEMENT_3D ( 'NONE', #30426, #471, #30918 ) ;
#2188=DIRECTION ( 'NONE',  ( -0.2503800040544453820, 0.000000000000000000, 0.9681476403781066331 ) ) ;
#2201=CARTESIAN_POINT ( 'NONE',  ( 12.83294900548060724, 14.63606878838274206, 7.766300266068485669 ) ) ;
#2209=TOROIDAL_SURFACE ( 'NONE', #46864, 14.49999999999999822, 0.5000000000000000000 ) ;
#2211=DIRECTION ( 'NONE',  ( 0.000000000000000000, 1.000000000000000000, 0.000000000000000000 ) ) ;
#2212=DIRECTION ( 'NONE',  ( 0.000000000000000000, 1.000000000000000000, 0.000000000000000000 ) ) ;
#2215=CARTESIAN_POINT ( 'NONE',  ( -3.795296366450300773, 27.84541550158064283, 14.16423886937410437 ) ) ;
#2217=B_SPLINE_CURVE_WITH_KNOTS ( 'NONE', 3,
 ( #34173, #49193, #72665, #64663, #64178, #4199 ),
 .UNSPECIFIED., .F., .F.,
 ( 4, 2, 4 ),
 ( 3.409110551496104941E-05, 0.0004400426677367861921, 0.0008459942299586112671 ),
 .UNSPECIFIED. ) ;
#2232=CARTESIAN_POINT ( 'NONE',  ( 0.000000000000000000, 0.5000000000000004441, 0.000000000000000000 ) ) ;
#2238=DIRECTION ( 'NONE',  ( 0.9238795325112876267, 0.000000000000000000, -0.3826834323650877279 ) ) ;
#2248=EDGE_CURVE ( 'NONE', #61223, #42327, #18320, .T. ) ;
#2255=DIRECTION ( 'NONE',  ( 0.000000000000000000, 0.000000000000000000, 1.000000000000000000 ) ) ;
#2271=ORIENTED_EDGE ( 'NONE', *, *, #89095, .F. ) ;
#2275=ORIENTED_EDGE ( 'NONE', *, *, #34522, .F. ) ;
#2279=CARTESIAN_POINT ( 'NONE',  ( -2.849309504156504413, 0.000000000000000000, 4.649650521509808954 ) ) ;
#2280=ORIENTED_EDGE ( 'NONE', *, *, #80937, .F. ) ;
#2282=CARTESIAN_POINT ( 'NONE',  ( 12.54397927573563365, 14.76930270348881180, 8.117058495689102315 ) ) ;
#2283=VECTOR ( 'NONE', #25246, 1000.000000000000000 ) ;
#2284=CARTESIAN_POINT ( 'NONE',  ( 6.408140936763243367, -4.209698663402907215, 11.09922568453594494 ) ) ;
#2285=ORIENTED_EDGE ( 'NONE', *, *, #5834, .T. ) ;
#2288=VERTEX_POINT ( 'NONE', #63306 ) ;
#2296=ADVANCED_FACE ( 'NONE', ( #40339 ), #95730, .T. ) ;
#2298=CARTESIAN_POINT ( 'NONE',  ( 1.326515405096126976, 0.2306972965111660223, -14.88215077106012529 ) ) ;
#2304=EDGE_CURVE ( 'NONE', #91405, #41669, #8746, .T. ) ;
#2317=EDGE_CURVE ( 'NONE', #39241, #14667, #25347, .T. ) ;
#2337=CARTESIAN_POINT ( 'NONE',  ( -0.1558200433086290304, 15.00000000000000178, -14.62618286184525829 ) ) ;
#2355=DIRECTION ( 'NONE',  ( 0.000000000000000000, 1.000000000000000000, 0.000000000000000000 ) ) ;
#2361=DIRECTION ( 'NONE',  ( -0.000000000000000000, -1.000000000000000000, -0.000000000000000000 ) ) ;
#2371=VECTOR ( 'NONE', #55317, 1000.000000000000000 ) ;
#2376=DIRECTION ( 'NONE',  ( -0.3007057995042766718, 0.000000000000000000, 0.9537169507482258224 ) ) ;
#2386=EDGE_CURVE ( 'NONE', #63123, #89545, #48801, .T. ) ;
#2392=EDGE_CURVE ( 'NONE', #70551, #70990, #85834, .T. ) ;
#2398=FACE_OUTER_BOUND ( 'NONE', #84995, .T. ) ;
#2401=VERTEX_POINT ( 'NONE', #47818 ) ;
#2411=CARTESIAN_POINT ( 'NONE',  ( 0.000000000000000000, 15.00000000000000000, 0.000000000000000000 ) ) ;
#2419=VECTOR ( 'NONE', #1334, 1000.000000000000114 ) ;
#2423=VERTEX_POINT ( 'NONE', #39357 ) ;
#2424=ORIENTED_EDGE ( 'NONE', *, *, #97101, .F. ) ;
#2429=DIRECTION ( 'NONE',  ( -0.000000000000000000, -1.000000000000000000, -0.000000000000000000 ) ) ;
#2430=DIRECTION ( 'NONE',  ( -0.000000000000000000, -1.000000000000000000, -0.000000000000000000 ) ) ;
#2432=DIRECTION ( 'NONE',  ( 0.000000000000000000, 1.000000000000000000, 0.000000000000000000 ) ) ;
#2436=DIRECTION ( 'NONE',  ( 0.000000000000000000, 1.000000000000000000, 0.000000000000000000 ) ) ;
#2439=CARTESIAN_POINT ( 'NONE',  ( -14.47650479471817242, 0.5000000000000004441, -3.928206833722204028 ) ) ;
#2443=CARTESIAN_POINT ( 'NONE',  ( -7.860426697680325425, 15.00000000000000000, -13.93165778241942832 ) ) ;
#2461=CARTESIAN_POINT ( 'NONE',  ( -14.49440716394873085, 4.311470567659570904E-16, -0.4026921475168178111 ) ) ;
#2464=CARTESIAN_POINT ( 'NONE',  ( 10.36894250292379027, 8.678748834913974974, 10.36894250292378672 ) ) ;
#2468=AXIS2_PLACEMENT_3D ( 'NONE', #2232, #32691, #26186 ) ;
#2470=CARTESIAN_POINT ( 'NONE',  ( -6.090257717040430840, -2.687212025164267037E-15, -13.29726560978576799 ) ) ;
#2472=CARTESIAN_POINT ( 'NONE',  ( -6.336512077239706109, 14.76930270348881180, -13.53095227201393413 ) ) ;
#2480=AXIS2_PLACEMENT_3D ( 'NONE', #27488, #19503, #42990 ) ;
#2484=AXIS2_PLACEMENT_3D ( 'NONE', #92075, #85069, #39580 ) ;
#2489=VERTEX_POINT ( 'NONE', #92832 ) ;
#2495=TOROIDAL_SURFACE ( 'NONE', #71133, 14.49999999999999822, 0.5000000000000000000 ) ;
#2499=CARTESIAN_POINT ( 'NONE',  ( -4.862001128006866679, 15.00000000000000000, 13.66056166602454347 ) ) ;
#2500=CARTESIAN_POINT ( 'NONE',  ( 10.76493118081685019, 1.524659305057740610E-16, 9.902252441915806003 ) ) ;
#2512=ORIENTED_EDGE ( 'NONE', *, *, #65266, .T. ) ;
#2514=EDGE_CURVE ( 'NONE', #98693, #52439, #24845, .T. ) ;
#2516=DIRECTION ( 'NONE',  ( 0.000000000000000000, 0.000000000000000000, 1.000000000000000000 ) ) ;
#2522=DIRECTION ( 'NONE',  ( 0.000000000000000000, 0.000000000000000000, -1.000000000000000000 ) ) ;
#2528=B_SPLINE_CURVE_WITH_KNOTS ( 'NONE', 3,
 ( #81225, #81706, #5246, #96244, #97245, #59701 ),
 .UNSPECIFIED., .F., .F.,
 ( 4, 2, 4 ),
 ( 3.409110551496071059E-05, 0.0004400426677367861921, 0.0008459942299586115924 ),
 .UNSPECIFIED. ) ;
#2532=CARTESIAN_POINT ( 'NONE',  ( 9.846743663894590881, 28.71726448433412671, -2.638427012816833894 ) ) ;
#2541=AXIS2_PLACEMENT_3D ( 'NONE', #67737, #14747, #67235 ) ;
#2543=VECTOR ( 'NONE', #8861, 1000.000000000000227 ) ;
#2547=EDGE_CURVE ( 'NONE', #23291, #42121, #26615, .T. ) ;
#2555=CARTESIAN_POINT ( 'NONE',  ( -5.376821459229932820, 0.2301511342434834628, -13.93958558162645112 ) ) ;
#2560=CIRCLE ( 'NONE', #58395, 15.00000000000000000 ) ;
#2564=ORIENTED_EDGE ( 'NONE', *, *, #16836, .T. ) ;
#2573=DIRECTION ( 'NONE',  ( -0.4461978131098131573, 0.000000000000000000, 0.8949343616020228875 ) ) ;
#2592=LINE ( 'NONE', #10555, #38498 ) ;
#2598=CARTESIAN_POINT ( 'NONE',  ( -2.915334737309934532, -2.977981322511826789, -10.88017736071109987 ) ) ;
#2605=PLANE ( 'NONE',  #62401 ) ;
#2620=CARTESIAN_POINT ( 'NONE',  ( 14.94699059465108171, 14.49999999999999112, -1.259949270174796965 ) ) ;
#2628=TOROIDAL_SURFACE ( 'NONE', #18587, 14.49999999999999822, 0.5000000000000000000 ) ;
#2629=EDGE_CURVE ( 'NONE', #59148, #50110, #58257, .T. ) ;
#2632=VECTOR ( 'NONE', #83832, 1000.000000000000000 ) ;
#2634=ORIENTED_EDGE ( 'NONE', *, *, #82984, .T. ) ;
#2645=CARTESIAN_POINT ( 'NONE',  ( 9.997910040112605756, 4.102332422533249404E-16, -10.50199004140717562 ) ) ;
#2647=CARTESIAN_POINT ( 'NONE',  ( 9.846743663894590881, -6.699402182332541145, 2.638427012816828565 ) ) ;
#2648=ORIENTED_EDGE ( 'NONE', *, *, #71276, .F. ) ;
#2650=ORIENTED_EDGE ( 'NONE', *, *, #57319, .T. ) ;
#2667=ORIENTED_EDGE ( 'NONE', *, *, #23207, .T. ) ;
#2675=VECTOR ( 'NONE', #43581, 1000.000000000000000 ) ;
#2677=LINE ( 'NONE', #80977, #85163 ) ;
#2683=DIRECTION ( 'NONE',  ( 0.000000000000000000, 0.000000000000000000, -1.000000000000000000 ) ) ;
#2684=CARTESIAN_POINT ( 'NONE',  ( -8.209432707285007069, 14.49999999999999112, 12.55409154915484393 ) ) ;
#2689=CARTESIAN_POINT ( 'NONE',  ( 14.04391541078763161, 15.00000000000000000, 3.608107528142933340 ) ) ;
#2694=EDGE_CURVE ( 'NONE', #7312, #11472, #19363, .T. ) ;
#2697=DIRECTION ( 'NONE',  ( -1.154631945610162802E-14, 0.000000000000000000, 1.000000000000000000 ) ) ;
#2702=CARTESIAN_POINT ( 'NONE',  ( -14.03351048042393856, 0.000000000000000000, -2.474486531753901541 ) ) ;
#2706=CARTESIAN_POINT ( 'NONE',  ( 10.91036564011041676, 0.2301503799940547990, -10.20716212663437261 ) ) ;
#2711=CARTESIAN_POINT ( 'NONE',  ( 3.469446951953614189E-15, 33.05374883491396787, 14.16423886937410259 ) ) ;
#2719=TOROIDAL_SURFACE ( 'NONE', #58571, 14.49999999999999822, 0.5000000000000000000 ) ;
#2722=VERTEX_POINT ( 'NONE', #4306 ) ;
#2728=DIRECTION ( 'NONE',  ( 0.000000000000000000, 1.000000000000000000, 0.000000000000000000 ) ) ;
#2739=DIRECTION ( 'NONE',  ( -0.000000000000000000, -1.000000000000000000, -0.000000000000000000 ) ) ;
#2740=DIRECTION ( 'NONE',  ( 0.000000000000000000, 1.000000000000000000, 0.000000000000000000 ) ) ;
#2741=ADVANCED_FACE ( 'NONE', ( #5781 ), #20283, .F. ) ;
#2742=CARTESIAN_POINT ( 'NONE',  ( 0.000000000000000000, 0.000000000000000000, 0.000000000000000000 ) ) ;
#2747=DIRECTION ( 'NONE',  ( 0.000000000000000000, 1.000000000000000000, 0.000000000000000000 ) ) ;
#2755=FACE_OUTER_BOUND ( 'NONE', #4071, .T. ) ;
#2760=CARTESIAN_POINT ( 'NONE',  ( 11.39601241150452182, -0.03417435944610275333, 11.22534175661874301 ) ) ;
#2767=ORIENTED_EDGE ( 'NONE', *, *, #73708, .F. ) ;
#2778=CARTESIAN_POINT ( 'NONE',  ( -12.81628187352647252, -5.668031996736239364, 3.434112377981066722 ) ) ;
#2779=VERTEX_POINT ( 'NONE', #1745 ) ;
#2782=EDGE_CURVE ( 'NONE', #60677, #50878, #54707, .T. ) ;
#2796=CARTESIAN_POINT ( 'NONE',  ( 9.402796353261049234, 0.3640475087720986824, 11.68706210897764031 ) ) ;
#2810=CARTESIAN_POINT ( 'NONE',  ( 13.75543905097946151, 14.95037102630295500, -5.333404663735534790 ) ) ;
#2815=PRESENTATION_STYLE_ASSIGNMENT (( #41300 ) ) ;
#2817=AXIS2_PLACEMENT_3D ( 'NONE', #13902, #44387, #20418 ) ;
#2818=ORIENTED_EDGE ( 'NONE', *, *, #9036, .F. ) ;
#2829=CARTESIAN_POINT ( 'NONE',  ( 0.000000000000000000, 14.49999999999999822, 0.000000000000000000 ) ) ;
#2839=ORIENTED_EDGE ( 'NONE', *, *, #66128, .F. ) ;
#2841=DIRECTION ( 'NONE',  ( 0.2672383760782636175, 0.000000000000000000, -0.9636304532086211738 ) ) ;
#2843=B_SPLINE_CURVE_WITH_KNOTS ( 'NONE', 3,
 ( #83444, #37960, #46425, #98476, #61908, #46907 ),
 .UNSPECIFIED., .F., .F.,
 ( 4, 2, 4 ),
 ( 0.0002800098399050243367, 0.0006862151655664761127, 0.001092420491227927889 ),
 .UNSPECIFIED. ) ;
#2852=CARTESIAN_POINT ( 'NONE',  ( -12.74414838903283531, 7.504711912673099032E-16, 7.178093659841884744 ) ) ;
#2861=CIRCLE ( 'NONE', #97072, 15.00000000000000000 ) ;
#2868=LINE ( 'NONE', #39860, #28051 ) ;
#2869=EDGE_CURVE ( 'NONE', #16281, #17551, #93201, .T. ) ;
#2870=ADVANCED_FACE ( 'NONE', ( #78203 ), #33188, .F. ) ;
#2887=CARTESIAN_POINT ( 'NONE',  ( 13.07751017357379730, 4.171195230237741069E-16, 6.263284095430596388 ) ) ;
#2888=DIRECTION ( 'NONE',  ( -5.151434834260726979E-14, 0.000000000000000000, 1.000000000000000000 ) ) ;
#2902=DIRECTION ( 'NONE',  ( 0.000000000000000000, 0.000000000000000000, 1.000000000000000000 ) ) ;
#2907=CARTESIAN_POINT ( 'NONE',  ( 0.000000000000000000, 14.49999999999999822, 0.000000000000000000 ) ) ;
#2911=ORIENTED_EDGE ( 'NONE', *, *, #30927, .T. ) ;
#2919=CARTESIAN_POINT ( 'NONE',  ( -1.780824192092605562, 0.5000000000000004441, 14.89391369643512064 ) ) ;
#2922=LINE ( 'NONE', #56872, #56403 ) ;
#2924=TOROIDAL_SURFACE ( 'NONE', #6113, 14.49999999999999822, 0.5000000000000000000 ) ;
#2925=CARTESIAN_POINT ( 'NONE',  ( 0.7575892234030736638, 0.2306972965111896423, 14.92193396517714454 ) ) ;
#2926=FACE_OUTER_BOUND ( 'NONE', #51310, .T. ) ;
#2929=CIRCLE ( 'NONE', #60423, 14.49999999999999822 ) ;
#2946=CARTESIAN_POINT ( 'NONE',  ( 3.881909499400429286, -2.725328507790710552E-15, -14.10103859407594840 ) ) ;
#2947=ADVANCED_FACE ( 'NONE', ( #70724 ), #63680, .F. ) ;
#2950=CARTESIAN_POINT ( 'NONE',  ( -3.795296366450322534, 5.762082168247310676, -14.16423886937409904 ) ) ;
#2957=CARTESIAN_POINT ( 'NONE',  ( 0.000000000000000000, 0.000000000000000000, 0.000000000000000000 ) ) ;
#2966=CARTESIAN_POINT ( 'NONE',  ( 12.83294900548063744, 0.5000000000000004441, -7.766300266068363101 ) ) ;
#2974=ORIENTED_EDGE ( 'NONE', *, *, #76441, .T. ) ;
#2981=EDGE_CURVE ( 'NONE', #27481, #37579, #94009, .T. ) ;
#2985=CARTESIAN_POINT ( 'NONE',  ( -4.838527690343711996, 14.63595249122789177, 14.19819177887725026 ) ) ;
#2987=DIRECTION ( 'NONE',  ( 0.000000000000000000, 0.000000000000000000, 1.000000000000000000 ) ) ;
#2989=B_SPLINE_CURVE_WITH_KNOTS ( 'NONE', 3,
 ( #57896, #80423, #41458, #26417, #48924, #2966 ),
 .UNSPECIFIED., .F., .F.,
 ( 4, 2, 4 ),
 ( 0.0002800591277523076304, 0.0006862649357714271578, 0.001092470743790546848 ),
 .UNSPECIFIED. ) ;
#2992=VECTOR ( 'NONE', #61922, 1000.000000000000000 ) ;
#3001=AXIS2_PLACEMENT_3D ( 'NONE', #73934, #5463, #59417 ) ;
#3002=ORIENTED_EDGE ( 'NONE', *, *, #70897, .T. ) ;
#3007=CARTESIAN_POINT ( 'NONE',  ( 0.000000000000000000, 15.00000000000000000, 0.000000000000000000 ) ) ;
#3012=CARTESIAN_POINT ( 'NONE',  ( 7.684764310694791156, 15.00000000000000000, 12.88194075009940498 ) ) ;
#3016=CARTESIAN_POINT ( 'NONE',  ( -12.81628187352647963, -31.08469866340290721, -3.434112377981046293 ) ) ;
#3034=DIRECTION ( 'NONE',  ( 0.000000000000000000, 1.000000000000000000, 0.000000000000000000 ) ) ;
#3042=DIRECTION ( 'NONE',  ( 0.000000000000000000, 1.000000000000000000, 0.000000000000000000 ) ) ;
#3045=CARTESIAN_POINT ( 'NONE',  ( -12.25993886608615568, 14.49999999999999112, 8.642563219313586842 ) ) ;
#3067=CARTESIAN_POINT ( 'NONE',  ( 12.26659068614894821, -36.11291783175269643, 7.082119434687044190 ) ) ;
#3075=DIRECTION ( 'NONE',  ( 0.000000000000000000, 0.000000000000000000, 1.000000000000000000 ) ) ;
#3079=CARTESIAN_POINT ( 'NONE',  ( 10.88017736071109987, 20.77201867748817676, -2.915334737309928315 ) ) ;
#3085=DIRECTION ( 'NONE',  ( 0.7933533402912281707, 0.000000000000000000, 0.6087614290087297597 ) ) ;
#3089=EDGE_CURVE ( 'NONE', #70273, #56575, #35655, .T. ) ;
#3099=ORIENTED_EDGE ( 'NONE', *, *, #32567, .T. ) ;
#3107=VECTOR ( 'NONE', #88381, 1000.000000000000114 ) ;
#3110=DIRECTION ( 'NONE',  ( -0.1132032137678971873, 0.000000000000000000, -0.9935718556765885667 ) ) ;
#3112=DIRECTION ( 'NONE',  ( 0.000000000000000000, 0.000000000000000000, 1.000000000000000000 ) ) ;
#3114=EDGE_LOOP ( 'NONE', ( #52086, #27172, #32033, #12314 ) ) ;
#3124=CARTESIAN_POINT ( 'NONE',  ( 3.469446951953614189E-15, -2.741068848999210328, 9.846743663894594434 ) ) ;
#3125=ORIENTED_EDGE ( 'NONE', *, *, #49226, .F. ) ;
#3133=CARTESIAN_POINT ( 'NONE',  ( -14.11874224319625348, 14.76984899115443994, -4.887061453530224142 ) ) ;
#3141=VECTOR ( 'NONE', #37398, 1000.000000000000114 ) ;
#3151=DIRECTION ( 'NONE',  ( 0.000000000000000000, 0.000000000000000000, 1.000000000000000000 ) ) ;
#3157=DIRECTION ( 'NONE',  ( 0.000000000000000000, 0.000000000000000000, 1.000000000000000000 ) ) ;
#3160=ORIENTED_EDGE ( 'NONE', *, *, #47359, .F. ) ;
#3170=ORIENTED_EDGE ( 'NONE', *, *, #59868, .F. ) ;
#3172=CARTESIAN_POINT ( 'NONE',  ( -0.7375392941515958034, 14.49999999999999112, -14.98185688723478215 ) ) ;
#3175=CARTESIAN_POINT ( 'NONE',  ( 6.236392532960747914, 13.06690530480599577, -10.05961789237413129 ) ) ;
#3177=DIRECTION ( 'NONE',  ( 0.000000000000000000, 1.000000000000000000, 0.000000000000000000 ) ) ;
#3181=CARTESIAN_POINT ( 'NONE',  ( -10.88017736071110342, -31.93631465584515539, 3.903127820947815962E-15 ) ) ;
#3193=ORIENTED_EDGE ( 'NONE', *, *, #78604, .T. ) ;
#3195=EDGE_CURVE ( 'NONE', #95706, #77766, #60460, .T. ) ;
#3200=CARTESIAN_POINT ( 'NONE',  ( -2.361410439757122059, 14.76930270348881180, -14.75336556272939781 ) ) ;
#3208=AXIS2_PLACEMENT_3D ( 'NONE', #58771, #7135, #42302 ) ;
#3216=VERTEX_POINT ( 'NONE', #4685 ) ;
#3218=ORIENTED_EDGE ( 'NONE', *, *, #60294, .F. ) ;
#3220=CARTESIAN_POINT ( 'NONE',  ( -4.698669664746495833, 0.000000000000000000, 2.767727949825290690 ) ) ;
#3225=DIRECTION ( 'NONE',  ( -0.000000000000000000, -1.000000000000000000, -0.000000000000000000 ) ) ;
#3236=DIRECTION ( 'NONE',  ( -0.4461978131098006117, 0.000000000000000000, -0.8949343616020291048 ) ) ;
#3246=CARTESIAN_POINT ( 'NONE',  ( -12.81628187352647963, -6.084698663402908991, -3.434112377981046293 ) ) ;
#3247=ORIENTED_EDGE ( 'NONE', *, *, #16788, .T. ) ;
#3253=CARTESIAN_POINT ( 'NONE',  ( 14.52844422123121682, -3.613442552986844458E-15, -1.683098224408302368 ) ) ;
#3255=LINE ( 'NONE', #66703, #12827 ) ;
#3262=CARTESIAN_POINT ( 'NONE',  ( 13.95692576442126942, 0.2301500530278525469, 5.331646315825828708 ) ) ;
#3265=VECTOR ( 'NONE', #52377, 1000.000000000000000 ) ;
#3273=CARTESIAN_POINT ( 'NONE',  ( 9.075906804202286793, -0.03417435944610275333, -13.17214151599837990 ) ) ;
#3274=DIRECTION ( 'NONE',  ( 0.000000000000000000, 0.000000000000000000, 1.000000000000000000 ) ) ;
#3277=CARTESIAN_POINT ( 'NONE',  ( 9.820682251645170169, 0.2306972965111888652, -11.26020669458359436 ) ) ;
#3280=EDGE_CURVE ( 'NONE', #54272, #19669, #65298, .T. ) ;
#3283=( NAMED_UNIT ( * ) SI_UNIT ( $, .STERADIAN. ) SOLID_ANGLE_UNIT ( ) );
#3284=CARTESIAN_POINT ( 'NONE',  ( -0.8649609010931206265, -2.456395547037469011E-16, -14.60103384664012971 ) ) ;
#3299=CIRCLE ( 'NONE', #38429, 14.49999999999999822 ) ;
#3302=EDGE_CURVE ( 'NONE', #86850, #53420, #50661, .T. ) ;
#3305=DIRECTION ( 'NONE',  ( -0.000000000000000000, -1.000000000000000000, -0.000000000000000000 ) ) ;
#3312=EDGE_CURVE ( 'NONE', #2779, #94935, #84456, .T. ) ;
#3314=DIRECTION ( 'NONE',  ( 0.000000000000000000, 0.000000000000000000, 1.000000000000000000 ) ) ;
#3319=CARTESIAN_POINT ( 'NONE',  ( 0.1034006766821536916, 0.000000000000000000, -14.49963131600461352 ) ) ;
#3324=CARTESIAN_POINT ( 'NONE',  ( -14.82679024690672875, 14.76930270348881002, 1.845086899513189049 ) ) ;
#3337=CARTESIAN_POINT ( 'NONE',  ( 14.24131928502211331, 15.00000000000000000, 0.4973178280106892446 ) ) ;
#3342=LINE ( 'NONE', #95316, #42729 ) ;
#3346=EDGE_LOOP ( 'NONE', ( #87923, #29571, #54331, #19511, #55798, #63038 ) ) ;
#3350=CARTESIAN_POINT ( 'NONE',  ( 2.518025504887051458, 0.000000000000000000, 4.837081990145644106 ) ) ;
#3357=CARTESIAN_POINT ( 'NONE',  ( 14.82269085861175384, 14.49999999999999112, -2.299529454046946864 ) ) ;
#3366=B_SPLINE_CURVE_WITH_KNOTS ( 'NONE', 3,
 ( #72381, #41919, #47423, #9430, #1955, #39934 ),
 .UNSPECIFIED., .F., .F.,
 ( 4, 2, 4 ),
 ( 3.409110551494645334E-05, 0.0004400426677367947573, 0.0008459942299586430342 ),
 .UNSPECIFIED. ) ;
#3378=DIRECTION ( 'NONE',  ( 0.000000000000000000, 1.000000000000000000, 0.000000000000000000 ) ) ;
#3382=EDGE_LOOP ( 'NONE', ( #10392, #45282, #71683, #68252 ) ) ;
#3389=CIRCLE ( 'NONE', #11373, 14.49999999999999822 ) ;
#3396=EDGE_CURVE ( 'NONE', #83574, #67150, #22221, .T. ) ;
#3399=VECTOR ( 'NONE', #5653, 1000.000000000000114 ) ;
#3404=ADVANCED_FACE ( 'NONE', ( #74637 ), #83632, .F. ) ;
#3405=CARTESIAN_POINT ( 'NONE',  ( -1.915564264621232748, 15.00000000000000000, -14.37291249357993372 ) ) ;
#3407=ADVANCED_FACE ( 'NONE', ( #61113 ), #83128, .F. ) ;
#3418=VECTOR ( 'NONE', #96069, 1000.000000000000114 ) ;
#3422=VERTEX_POINT ( 'NONE', #30113 ) ;
#3426=DIRECTION ( 'NONE',  ( -0.000000000000000000, -1.000000000000000000, -0.000000000000000000 ) ) ;
#3427=CARTESIAN_POINT ( 'NONE',  ( -7.082119434687058401, 0.9704155015806334994, -12.26659068614894110 ) ) ;
#3430=ORIENTED_EDGE ( 'NONE', *, *, #28357, .T. ) ;
#3454=VERTEX_POINT ( 'NONE', #45119 ) ;
#3476=EDGE_CURVE ( 'NONE', #587, #18033, #97663, .T. ) ;
#3485=CARTESIAN_POINT ( 'NONE',  ( -8.564643372776705732, 14.63595249122789177, 12.31449893000736040 ) ) ;
#3493=CIRCLE ( 'NONE', #6686, 14.49999999999999822 ) ;
#3495=CARTESIAN_POINT ( 'NONE',  ( -11.09922568453594316, -35.45969866340291077, 6.408140936763246920 ) ) ;
#3505=CARTESIAN_POINT ( 'NONE',  ( -14.97687855664607248, 0.5000000000000004441, -0.8325315005902533816 ) ) ;
#3509=CARTESIAN_POINT ( 'NONE',  ( -14.82269085861165792, 0.5000000000000004441, -2.299529454047158250 ) ) ;
#3511=ORIENTED_EDGE ( 'NONE', *, *, #78014, .T. ) ;
#3513=CARTESIAN_POINT ( 'NONE',  ( 8.731067818237031375, 7.813309369127511061, -8.731067818237036704 ) ) ;
#3516=ADVANCED_FACE ( 'NONE', ( #98158 ), #51654, .T. ) ;
#3520=FILL_AREA_STYLE_COLOUR ( '', #12041 ) ;
#3525=AXIS2_PLACEMENT_3D ( 'NONE', #97580, #29041, #59549 ) ;
#3529=FACE_OUTER_BOUND ( 'NONE', #93113, .T. ) ;
#3534=FACE_OUTER_BOUND ( 'NONE', #20812, .T. ) ;
#3540=CARTESIAN_POINT ( 'NONE',  ( -1.829604203029787435, 15.00000000000000000, 15.89119079541584334 ) ) ;
#3541=VERTEX_POINT ( 'NONE', #60619 ) ;
#3549=DIRECTION ( 'NONE',  ( 0.000000000000000000, 1.000000000000000000, 0.000000000000000000 ) ) ;
#3551=CARTESIAN_POINT ( 'NONE',  ( 3.795296366450306547, -34.65458449841935362, -14.16423886937410259 ) ) ;
#3555=EDGE_LOOP ( 'NONE', ( #49020, #19116, #92730, #26142 ) ) ;
#3561=CIRCLE ( 'NONE', #80194, 14.49999999999999822 ) ;
#3562=CARTESIAN_POINT ( 'NONE',  ( 1.114591949024916984, 15.00000000000000000, 14.45709807627962817 ) ) ;
#3563=CARTESIAN_POINT ( 'NONE',  ( 0.000000000000000000, 15.00000000000000000, 0.000000000000000000 ) ) ;
#3566=VECTOR ( 'NONE', #79091, 1000.000000000000000 ) ;
#3570=CARTESIAN_POINT ( 'NONE',  ( 10.88017736071110519, 15.56368534415484461, -2.602085213965210642E-15 ) ) ;
#3572=VECTOR ( 'NONE', #46827, 1000.000000000000114 ) ;
#3575=DIRECTION ( 'NONE',  ( -0.8703556959398977000, 0.000000000000000000, -0.4924235601034707699 ) ) ;
#3579=DIRECTION ( 'NONE',  ( 0.000000000000000000, 0.000000000000000000, 1.000000000000000000 ) ) ;
#3597=CARTESIAN_POINT ( 'NONE',  ( 9.065164099344587001, 14.49999999999999112, -11.95084933600771038 ) ) ;
#3604=CARTESIAN_POINT ( 'NONE',  ( 11.36220558718857099, 4.586546245355948473E-16, 9.008345252845320061 ) ) ;
#3609=CARTESIAN_POINT ( 'NONE',  ( 9.846743663894590881, -1.699402182332547362, 2.638427012816828565 ) ) ;
#3623=ORIENTED_EDGE ( 'NONE', *, *, #17437, .T. ) ;
#3629=ORIENTED_EDGE ( 'NONE', *, *, #87817, .F. ) ;
#3639=ORIENTED_EDGE ( 'NONE', *, *, #10567, .T. ) ;
#3645=VECTOR ( 'NONE', #52937, 1000.000000000000000 ) ;
#3649=CARTESIAN_POINT ( 'NONE',  ( 0.000000000000000000, 14.49999999999999822, 0.000000000000000000 ) ) ;
#3663=EDGE_CURVE ( 'NONE', #95321, #60992, #18094, .T. ) ;
#3666=FACE_OUTER_BOUND ( 'NONE', #86022, .T. ) ;
#3669=CARTESIAN_POINT ( 'NONE',  ( 11.23445519025490036, 12.65797429472845792, -2.010653977028116213 ) ) ;
#3671=EDGE_CURVE ( 'NONE', #42104, #71871, #71908, .T. ) ;
#3676=CARTESIAN_POINT ( 'NONE',  ( 7.964842623401177768, -18.81131465584515894, -7.964842623401181321 ) ) ;
#3680=CARTESIAN_POINT ( 'NONE',  ( 8.470897558477529898, 2.354751593366954943E-16, 11.92401951126086779 ) ) ;
#3681=DIRECTION ( 'NONE',  ( 0.000000000000000000, 1.000000000000000000, 0.000000000000000000 ) ) ;
#3698=ORIENTED_EDGE ( 'NONE', *, *, #74061, .F. ) ;
#3708=CIRCLE ( 'NONE', #14922, 15.00000000000000000 ) ;
#3709=CARTESIAN_POINT ( 'NONE',  ( 0.000000000000000000, 15.00000000000000000, 0.000000000000000000 ) ) ;
#3711=ORIENTED_EDGE ( 'NONE', *, *, #553, .F. ) ;
#3714=ORIENTED_EDGE ( 'NONE', *, *, #98402, .F. ) ;
#3715=CARTESIAN_POINT ( 'NONE',  ( -5.302565485995475392, 0.000000000000000000, -1.273033341818904818 ) ) ;
#3727=FACE_OUTER_BOUND ( 'NONE', #57692, .T. ) ;
#3731=CARTESIAN_POINT ( 'NONE',  ( -3.469446951953614189E-15, -40.24106884899921255, -9.846743663894594434 ) ) ;
#3732=VERTEX_POINT ( 'NONE', #2620 ) ;
#3737=ORIENTED_EDGE ( 'NONE', *, *, #98702, .T. ) ;
#3747=CARTESIAN_POINT ( 'NONE',  ( -11.09922568453594316, 14.54030133659709634, 6.408140936763246920 ) ) ;
#3748=ORIENTED_EDGE ( 'NONE', *, *, #55444, .F. ) ;
#3750=EDGE_LOOP ( 'NONE', ( #53698, #7579, #8790, #57197, #21652, #23651 ) ) ;
#3751=EDGE_LOOP ( 'NONE', ( #70168, #28982, #43924, #31444, #82295, #45389 ) ) ;
#3758=CARTESIAN_POINT ( 'NONE',  ( 10.09777502097877289, 0.04922511925147150802, 10.75551206493387824 ) ) ;
#3760=TOROIDAL_SURFACE ( 'NONE', #30867, 14.49999999999999822, 0.5000000000000000000 ) ;
#3763=CARTESIAN_POINT ( 'NONE',  ( 1.915564264621439472, 15.00000000000000000, -14.37291249357988043 ) ) ;
#3765=AXIS2_PLACEMENT_3D ( 'NONE', #39904, #85900, #55400 ) ;
#3771=LINE ( 'NONE', #25294, #10607 ) ;
#3774=AXIS2_PLACEMENT_3D ( 'NONE', #88231, #42743, #4260 ) ;
#3780=CARTESIAN_POINT ( 'NONE',  ( 4.838527690343520149, 14.49999999999999112, 14.19819177887736927 ) ) ;
#3798=FACE_OUTER_BOUND ( 'NONE', #59290, .T. ) ;
#3799=ADVANCED_FACE ( 'NONE', ( #72541 ), #9510, .T. ) ;
#3800=CARTESIAN_POINT ( 'NONE',  ( -12.60589901313216998, 14.49999999999999112, -8.129656208642240145 ) ) ;
#3803=VERTEX_POINT ( 'NONE', #41595 ) ;
#3814=ORIENTED_EDGE ( 'NONE', *, *, #25409, .F. ) ;
#3821=CARTESIAN_POINT ( 'NONE',  ( -2.815433093576927170, 0.5000000000000004441, -14.73340885523753663 ) ) ;
#3822=CARTESIAN_POINT ( 'NONE',  ( -7.595945211628163385, 4.385640548506873962E-16, -12.35117874301652030 ) ) ;
#3841=PLANE ( 'NONE',  #95399 ) ;
#3843=CIRCLE ( 'NONE', #67712, 11.92686044187656513 ) ;
#3845=CARTESIAN_POINT ( 'NONE',  ( 13.75801628063879711, 15.00000000000000000, -4.578972376164444746 ) ) ;
#3849=VERTEX_POINT ( 'NONE', #58034 ) ;
#3851=EDGE_CURVE ( 'NONE', #88606, #59795, #66031, .T. ) ;
#3853=ORIENTED_EDGE ( 'NONE', *, *, #76791, .T. ) ;
#3855=DIRECTION ( 'NONE',  ( -0.8338858220671658827, 0.000000000000000000, -0.5519369853120617009 ) ) ;
#3856=CARTESIAN_POINT ( 'NONE',  ( 0.000000000000000000, 0.5000000000000004441, 0.000000000000000000 ) ) ;
#3873=VERTEX_POINT ( 'NONE', #12051 ) ;
#3877=DIRECTION ( 'NONE',  ( 0.000000000000000000, 1.000000000000000000, 0.000000000000000000 ) ) ;
#3890=CARTESIAN_POINT ( 'NONE',  ( 14.94699059465101776, 0.5000000000000004441, -1.259949270174818059 ) ) ;
#3893=LINE ( 'NONE', #34361, #45735 ) ;
#3895=ORIENTED_EDGE ( 'NONE', *, *, #37450, .T. ) ;
#3911=CARTESIAN_POINT ( 'NONE',  ( -8.209432707284724628, 0.3639311627136666005, -12.55409154915499492 ) ) ;
#3915=EDGE_CURVE ( 'NONE', #62655, #12737, #90924, .T. ) ;
#3919=VERTEX_POINT ( 'NONE', #42552 ) ;
#3923=CARTESIAN_POINT ( 'NONE',  ( -12.25993886608593364, 0.5000000000000004441, -8.642563219313787570 ) ) ;
#3926=CARTESIAN_POINT ( 'NONE',  ( -14.35840480524201190, 14.49999999999999112, -4.340070442839034648 ) ) ;
#3928=VERTEX_POINT ( 'NONE', #58529 ) ;
#3930=ADVANCED_FACE ( 'NONE', ( #57545 ), #81039, .F. ) ;
#3934=CARTESIAN_POINT ( 'NONE',  ( 4.181050312905074229, 2.541098841762901017E-16, -14.01631781289604106 ) ) ;
#3942=TOROIDAL_SURFACE ( 'NONE', #74139, 14.49999999999999822, 0.5000000000000000000 ) ;
#3950=EDGE_LOOP ( 'NONE', ( #20486, #28079, #72349, #18746 ) ) ;
#3951=CARTESIAN_POINT ( 'NONE',  ( 4.873787042390789637, 15.00000000000000000, -13.39061984619918988 ) ) ;
#3959=VERTEX_POINT ( 'NONE', #80056 ) ;
#3960=VECTOR ( 'NONE', #4331, 1000.000000000000000 ) ;
#3964=DIRECTION ( 'NONE',  ( -0.2164396139380971307, 0.000000000000000000, -0.9762960071199346945 ) ) ;
#3979=AXIS2_PLACEMENT_3D ( 'NONE', #75483, #92447, #10437 ) ;
#3981=VECTOR ( 'NONE', #89387, 1000.000000000000000 ) ;
#3984=CARTESIAN_POINT ( 'NONE',  ( -6.408140936763246032, -36.70969866340291077, -11.09922568453594316 ) ) ;
#3986=AXIS2_PLACEMENT_3D ( 'NONE', #30316, #15352, #45838 ) ;
#3997=AXIS2_PLACEMENT_3D ( 'NONE', #60355, #44853, #91851 ) ;
#4000=EDGE_LOOP ( 'NONE', ( #88897, #61277, #8691, #69244, #4087, #19191 ) ) ;
#4004=LINE ( 'NONE', #4497, #95246 ) ;
#4015=CARTESIAN_POINT ( 'NONE',  ( -14.47650479471830387, 14.49999999999999112, 3.928206833721953561 ) ) ;
#4018=ORIENTED_EDGE ( 'NONE', *, *, #69832, .T. ) ;
#4019=CARTESIAN_POINT ( 'NONE',  ( -9.065164099344617199, 0.3640475087720972946, 11.95084933600761623 ) ) ;
#4024=B_SPLINE_CURVE_WITH_KNOTS ( 'NONE', 3,
 ( #18326, #33307, #48807, #79315, #41343, #3822 ),
 .UNSPECIFIED., .F., .F.,
 ( 4, 2, 4 ),
 ( 3.409110551496115105E-05, 0.0004400426677367866800, 0.0008459942299586121345 ),
 .UNSPECIFIED. ) ;
#4025=CARTESIAN_POINT ( 'NONE',  ( 0.000000000000000000, 0.5000000000000004441, 0.000000000000000000 ) ) ;
#4028=LINE ( 'NONE', #73476, #50263 ) ;
#4031=CARTESIAN_POINT ( 'NONE',  ( -6.689969769698787871, 0.000000000000000000, -12.58200319823979285 ) ) ;
#4039=EDGE_CURVE ( 'NONE', #7321, #79142, #30291, .T. ) ;
#4041=CARTESIAN_POINT ( 'NONE',  ( 12.26659068614894466, -30.27958449841936428, -7.082119434687053960 ) ) ;
#4044=ORIENTED_EDGE ( 'NONE', *, *, #36141, .F. ) ;
#4045=DIRECTION ( 'NONE',  ( -0.000000000000000000, 1.000000000000000000, -0.000000000000000000 ) ) ;
#4046=AXIS2_PLACEMENT_3D ( 'NONE', #90205, #20241, #50744 ) ;
#4052=CARTESIAN_POINT ( 'NONE',  ( -14.88232117145532030, 14.63606897487788849, -1.875237731503358152 ) ) ;
#4057=CARTESIAN_POINT ( 'NONE',  ( 2.915334737309921209, 16.60535201082150891, -10.88017736071110164 ) ) ;
#4071=EDGE_LOOP ( 'NONE', ( #17052, #49010, #96186, #82986, #22920, #1584 ) ) ;
#4081=CARTESIAN_POINT ( 'NONE',  ( -8.549759589250404801, 14.76984986100782393, -12.25250350990841319 ) ) ;
#4083=CARTESIAN_POINT ( 'NONE',  ( 6.689969769698956625, 0.000000000000000000, -12.58200319823970226 ) ) ;
#4086=VERTEX_POINT ( 'NONE', #61437 ) ;
#4087=ORIENTED_EDGE ( 'NONE', *, *, #95830, .F. ) ;
#4093=CARTESIAN_POINT ( 'NONE',  ( -1.354709868695410657, 14.49999999999999822, -14.93870011653153718 ) ) ;
#4094=DIRECTION ( 'NONE',  ( 0.7132504491541801217, -0.000000000000000000, 0.7009092642998523415 ) ) ;
#4099=EDGE_CURVE ( 'NONE', #40524, #88245, #31425, .T. ) ;
#4100=DIRECTION ( 'NONE',  ( 2.220446049250313396E-14, 0.000000000000000000, 1.000000000000000000 ) ) ;
#4102=CARTESIAN_POINT ( 'NONE',  ( 3.469446951953614189E-15, 2.258931151000794113, 9.846743663894594434 ) ) ;
#4103=ORIENTED_EDGE ( 'NONE', *, *, #18120, .T. ) ;
#4118=ORIENTED_EDGE ( 'NONE', *, *, #43513, .T. ) ;
#4127=CARTESIAN_POINT ( 'NONE',  ( 1.236172813752370869, 0.04922511925149002099, -14.70095156538450176 ) ) ;
#4129=CARTESIAN_POINT ( 'NONE',  ( 9.997910040112534702, 15.00000000000000000, 10.50199004140724490 ) ) ;
#4136=DIRECTION ( 'NONE',  ( 0.000000000000000000, 0.000000000000000000, 1.000000000000000000 ) ) ;
#4138=DIRECTION ( 'NONE',  ( 0.000000000000000000, 0.000000000000000000, 1.000000000000000000 ) ) ;
#4141=CARTESIAN_POINT ( 'NONE',  ( -3.420591144908373682, 0.3639311400139669250, -14.60477854057963931 ) ) ;
#4144=VERTEX_POINT ( 'NONE', #489 ) ;
#4153=FACE_OUTER_BOUND ( 'NONE', #9824, .T. ) ;
#4154=ORIENTED_EDGE ( 'NONE', *, *, #35093, .F. ) ;
#4159=CARTESIAN_POINT ( 'NONE',  ( 10.90209973789213116, 12.73026364691592072, -3.659052390917571174 ) ) ;
#4164=CARTESIAN_POINT ( 'NONE',  ( 2.915334737309928315, -20.47798132251182679, 10.88017736071109987 ) ) ;
#4168=CARTESIAN_POINT ( 'NONE',  ( -6.767445849361341637, 14.49999999999999112, 13.38662304974498873 ) ) ;
#4169=CARTESIAN_POINT ( 'NONE',  ( 7.684764310694791156, 0.5000000000000004441, 12.88194075009940498 ) ) ;
#4172=DIRECTION ( 'NONE',  ( 0.000000000000000000, 1.000000000000000000, 0.000000000000000000 ) ) ;
#4180=CARTESIAN_POINT ( 'NONE',  ( 0.000000000000000000, 14.49999999999999822, 0.000000000000000000 ) ) ;
#4195=LINE ( 'NONE', #20166, #16040 ) ;
#4197=EDGE_CURVE ( 'NONE', #61531, #89575, #68957, .T. ) ;
#4198=EDGE_LOOP ( 'NONE', ( #31507, #60425, #30575, #60085, #77162, #13104 ) ) ;
#4199=CARTESIAN_POINT ( 'NONE',  ( -4.862001128006591344, 4.779775600002961917E-16, -13.66056166602466604 ) ) ;
#4201=ORIENTED_EDGE ( 'NONE', *, *, #92578, .T. ) ;
#4203=CARTESIAN_POINT ( 'NONE',  ( 0.000000000000000000, 0.5000000000000004441, 0.000000000000000000 ) ) ;
#4218=DIRECTION ( 'NONE',  ( 0.000000000000000000, 1.000000000000000000, 0.000000000000000000 ) ) ;
#4219=CARTESIAN_POINT ( 'NONE',  ( -2.638427012816840111, -40.03273551566587685, -9.846743663894590881 ) ) ;
#4221=CARTESIAN_POINT ( 'NONE',  ( -7.551349515323020789, -0.03417435944610275333, -12.08468537022916323 ) ) ;
#4222=ORIENTED_EDGE ( 'NONE', *, *, #59994, .F. ) ;
#4225=VECTOR ( 'NONE', #90119, 1000.000000000000000 ) ;
#4232=CARTESIAN_POINT ( 'NONE',  ( 6.408140936763243367, 10.79030133659709279, 11.09922568453594494 ) ) ;
#4246=FACE_OUTER_BOUND ( 'NONE', #85101, .T. ) ;
#4256=LINE ( 'NONE', #82208, #74544 ) ;
#4260=DIRECTION ( 'NONE',  ( 0.000000000000000000, 0.000000000000000000, 1.000000000000000000 ) ) ;
#4267=VECTOR ( 'NONE', #45715, 1000.000000000000114 ) ;
#4273=CARTESIAN_POINT ( 'NONE',  ( -11.25000000000000178, 2.921802177851545945, 3.951965214266261022E-15 ) ) ;
#4277=DIRECTION ( 'NONE',  ( 0.000000000000000000, 1.000000000000000000, 0.000000000000000000 ) ) ;
#4280=DIRECTION ( 'NONE',  ( 0.000000000000000000, 1.000000000000000000, 0.000000000000000000 ) ) ;
#4290=VECTOR ( 'NONE', #80103, 1000.000000000000227 ) ;
#4293=ORIENTED_EDGE ( 'NONE', *, *, #65811, .F. ) ;
#4297=CARTESIAN_POINT ( 'NONE',  ( -12.80781515976318907, 0.000000000000000000, 6.246788841744232990 ) ) ;
#4304=ORIENTED_EDGE ( 'NONE', *, *, #93124, .F. ) ;
#4306=CARTESIAN_POINT ( 'NONE',  ( 0.000000000000000000, 0.000000000000000000, -14.25000000000000000 ) ) ;
#4311=CARTESIAN_POINT ( 'NONE',  ( -11.62719953690051788, 15.00000000000000000, -9.476720473301954328 ) ) ;
#4324=DIRECTION ( 'NONE',  ( 0.000000000000000000, 0.000000000000000000, 1.000000000000000000 ) ) ;
#4331=DIRECTION ( 'NONE',  ( 0.000000000000000000, 1.000000000000000000, 0.000000000000000000 ) ) ;
#4333=EDGE_CURVE ( 'NONE', #7776, #62748, #65865, .T. ) ;
#4336=DIRECTION ( 'NONE',  ( 0.000000000000000000, 0.000000000000000000, 1.000000000000000000 ) ) ;
#4339=CARTESIAN_POINT ( 'NONE',  ( 14.17193700899789022, 15.00000000000000000, 1.489530601564113654 ) ) ;
#4340=ORIENTED_EDGE ( 'NONE', *, *, #58179, .T. ) ;
#4342=PRODUCT_DEFINITION ( 'UNKNOWN', '', #18381, #74461 ) ;
#4343=ORIENTED_EDGE ( 'NONE', *, *, #22957, .T. ) ;
#4346=EDGE_LOOP ( 'NONE', ( #80800, #84672, #36624, #58557 ) ) ;
#4347=CARTESIAN_POINT ( 'NONE',  ( -9.383624259803923451, 14.76984980006450066, -11.62625599701892298 ) ) ;
#4348=TOROIDAL_SURFACE ( 'NONE', #42655, 14.49999999999999822, 0.5000000000000000000 ) ;
#4350=VERTEX_POINT ( 'NONE', #89851 ) ;
#4351=VECTOR ( 'NONE', #72548, 1000.000000000000000 ) ;
#4354=CARTESIAN_POINT ( 'NONE',  ( -10.64017930668212664, 15.00000000000000000, 10.57291749337208309 ) ) ;
#4355=DIRECTION ( 'NONE',  ( 0.000000000000000000, 1.000000000000000000, 0.000000000000000000 ) ) ;
#4363=VERTEX_POINT ( 'NONE', #58352 ) ;
#4364=DIRECTION ( 'NONE',  ( 0.000000000000000000, 0.000000000000000000, -1.000000000000000000 ) ) ;
#4369=CARTESIAN_POINT ( 'NONE',  ( -7.793944756043282851, 2.100340034815855628, -8.673230486701367425 ) ) ;
#4375=EDGE_LOOP ( 'NONE', ( #49231, #70006, #82050, #1924, #46258, #57177 ) ) ;
#4381=CARTESIAN_POINT ( 'NONE',  ( 11.96291822454875842, 4.834832779786913688E-16, 8.193813980849165901 ) ) ;
#4407=CARTESIAN_POINT ( 'NONE',  ( 7.313705784284644906, 14.49999999999999112, -13.09617149020747817 ) ) ;
#4415=EDGE_CURVE ( 'NONE', #45767, #94563, #26889, .T. ) ;
#4417=VECTOR ( 'NONE', #17180, 1000.000000000000227 ) ;
#4418=TOROIDAL_SURFACE ( 'NONE', #53878, 14.49999999999999822, 0.5000000000000000000 ) ;
#4427=CARTESIAN_POINT ( 'NONE',  ( 11.35178980618980304, 14.49999999999999112, -9.804941009311946232 ) ) ;
#4436=CARTESIAN_POINT ( 'NONE',  ( -13.21236992757665973, -0.03417435944610275333, -5.338143956176898186 ) ) ;
#4452=ORIENTED_EDGE ( 'NONE', *, *, #61724, .F. ) ;
#4453=LINE ( 'NONE', #3951, #67648 ) ;
#4454=CARTESIAN_POINT ( 'NONE',  ( 0.7117905103454439386, 0.000000000000000000, 5.406585696355436177 ) ) ;
#4456=DIRECTION ( 'NONE',  ( -0.7604059656000257128, 0.000000000000000000, -0.6494480483301898754 ) ) ;
#4460=ORIENTED_EDGE ( 'NONE', *, *, #38762, .F. ) ;
#4463=CARTESIAN_POINT ( 'NONE',  ( 6.336512077239887297, 0.2306972965111900864, -13.53095227201384354 ) ) ;
#4469=DIRECTION ( 'NONE',  ( -0.9025852843498589628, 0.000000000000000000, -0.4305110968082987433 ) ) ;
#4479=CARTESIAN_POINT ( 'NONE',  ( 3.434112377981054287, -32.33469866340291077, -12.81628187352647608 ) ) ;
#4488=EDGE_CURVE ( 'NONE', #96588, #16656, #12865, .T. ) ;
#4495=DIRECTION ( 'NONE',  ( 0.000000000000000000, 0.000000000000000000, 1.000000000000000000 ) ) ;
#4497=CARTESIAN_POINT ( 'NONE',  ( -9.075906804202377387, 15.00000000000000000, 13.17214151599831595 ) ) ;
#4498=VERTEX_POINT ( 'NONE', #4407 ) ;
#4500=CARTESIAN_POINT ( 'NONE',  ( 11.92686044187655980, 7.396642702460839658, -3.195792623639533314 ) ) ;
#4517=FACE_OUTER_BOUND ( 'NONE', #44073, .T. ) ;
#4530=CARTESIAN_POINT ( 'NONE',  ( 12.00809552683958614, 0.5000000000000004441, -8.989195838243546177 ) ) ;
#4531=EDGE_CURVE ( 'NONE', #22303, #88333, #57870, .T. ) ;
#4533=CARTESIAN_POINT ( 'NONE',  ( -14.16423886937410437, -28.40458449841936428, -3.795296366450299885 ) ) ;
#4538=CARTESIAN_POINT ( 'NONE',  ( -11.35178980618960409, 15.00000000000000000, -9.804941009312079458 ) ) ;
#4544=CARTESIAN_POINT ( 'NONE',  ( -4.873787042390880231, 15.00000000000000000, 13.39061984619915791 ) ) ;
#4546=CARTESIAN_POINT ( 'NONE',  ( -6.728851239469183732, -2.645283894275179170E-15, 12.98580270086196542 ) ) ;
#4547=AXIS2_PLACEMENT_3D ( 'NONE', #15217, #54657, #91691 ) ;
#4549=CARTESIAN_POINT ( 'NONE',  ( 9.422509992056141925, 15.14701867748818209, 5.440088680355547268 ) ) ;
#4553=CARTESIAN_POINT ( 'NONE',  ( 0.000000000000000000, 0.000000000000000000, 0.000000000000000000 ) ) ;
#4559=EDGE_CURVE ( 'NONE', #97832, #31539, #1606, .T. ) ;
#4567=EDGE_LOOP ( 'NONE', ( #94794, #37321, #67176, #9373 ) ) ;
#4569=EDGE_CURVE ( 'NONE', #84772, #86520, #32600, .T. ) ;
#4581=CARTESIAN_POINT ( 'NONE',  ( 0.000000000000000000, 14.49999999999999822, 0.000000000000000000 ) ) ;
#4583=ORIENTED_EDGE ( 'NONE', *, *, #90769, .T. ) ;
#4584=ORIENTED_EDGE ( 'NONE', *, *, #9279, .T. ) ;
#4590=CARTESIAN_POINT ( 'NONE',  ( 8.606322355891363074, 4.859979058039186735E-16, -11.66967075398807374 ) ) ;
#4593=DIRECTION ( 'NONE',  ( -0.000000000000000000, -1.000000000000000000, -0.000000000000000000 ) ) ;
#4595=CARTESIAN_POINT ( 'NONE',  ( -4.922013193295410538, 0.000000000000000000, -2.347679864819515405 ) ) ;
#4596=CARTESIAN_POINT ( 'NONE',  ( -7.208316651077756099, -3.366068848999213881, 7.208316651077766757 ) ) ;
#4600=EDGE_LOOP ( 'NONE', ( #55398, #23260, #22155, #55093, #53646, #56206 ) ) ;
#4609=EDGE_CURVE ( 'NONE', #15452, #82266, #97377, .T. ) ;
#4614=ORIENTED_EDGE ( 'NONE', *, *, #90296, .T. ) ;
#4616=ORIENTED_EDGE ( 'NONE', *, *, #36367, .F. ) ;
#4622=CARTESIAN_POINT ( 'NONE',  ( 5.991992585808628036, 15.00000000000000000, -13.20401548210295140 ) ) ;
#4625=CARTESIAN_POINT ( 'NONE',  ( -10.64017930668191170, 15.00000000000000000, -10.57291749337230158 ) ) ;
#4626=ORIENTED_EDGE ( 'NONE', *, *, #54069, .T. ) ;
#4630=DIRECTION ( 'NONE',  ( 0.000000000000000000, 1.000000000000000000, 0.000000000000000000 ) ) ;
#4633=LINE ( 'NONE', #5616, #50786 ) ;
#4638=CARTESIAN_POINT ( 'NONE',  ( -14.02068044289382875, 15.00000000000000000, 5.331089937175565119 ) ) ;
#4640=CARTESIAN_POINT ( 'NONE',  ( -5.204170427930421283E-15, 3.438309369127513726, -11.92686044187656513 ) ) ;
#4646=CARTESIAN_POINT ( 'NONE',  ( -4.096035146093346846, 4.802464241948007172E-16, -13.90943910019264429 ) ) ;
#4660=DIRECTION ( 'NONE',  ( 0.000000000000000000, 1.000000000000000000, 0.000000000000000000 ) ) ;
#4666=CARTESIAN_POINT ( 'NONE',  ( 10.88017736071109987, -19.22798132251182324, -2.915334737309928315 ) ) ;
#4671=DIRECTION ( 'NONE',  ( 0.9099612708765425495, -0.000000000000000000, 0.4146932426562403018 ) ) ;
#4679=DIRECTION ( 'NONE',  ( 0.7372773368101250835, 0.000000000000000000, 0.6755902076156591329 ) ) ;
#4683=VERTEX_POINT ( 'NONE', #853 ) ;
#4685=CARTESIAN_POINT ( 'NONE',  ( 8.375939845167756914, 15.00000000000000000, -11.52849216984298941 ) ) ;
#4694=FACE_OUTER_BOUND ( 'NONE', #6859, .T. ) ;
#4695=CARTESIAN_POINT ( 'NONE',  ( -4.494156999534613561, 0.000000000000000000, 3.088748530746243670 ) ) ;
#4696=AXIS2_PLACEMENT_3D ( 'NONE', #8045, #84038, #91032 ) ;
#4697=VERTEX_POINT ( 'NONE', #75340 ) ;
#4700=VERTEX_POINT ( 'NONE', #15362 ) ;
#4719=ORIENTED_EDGE ( 'NONE', *, *, #18023, .F. ) ;
#4725=DIRECTION ( 'NONE',  ( -0.000000000000000000, -1.000000000000000000, -0.000000000000000000 ) ) ;
#4727=CARTESIAN_POINT ( 'NONE',  ( 9.382169495545419124, 5.998634669930423158, 9.382169495545417348 ) ) ;
#4731=ORIENTED_EDGE ( 'NONE', *, *, #94472, .F. ) ;
#4738=CARTESIAN_POINT ( 'NONE',  ( 12.60874940350947959, 4.146618495107105809E-16, -7.160268045227032196 ) ) ;
#4739=ORIENTED_EDGE ( 'NONE', *, *, #87973, .F. ) ;
#4740=CARTESIAN_POINT ( 'NONE',  ( 0.000000000000000000, 14.49999999999999822, 0.000000000000000000 ) ) ;
#4748=CARTESIAN_POINT ( 'NONE',  ( 13.48255862862752430, 15.00000000000000000, -5.335786055104087211 ) ) ;
#4755=EDGE_CURVE ( 'NONE', #29308, #48625, #45847, .T. ) ;
#4766=EDGE_CURVE ( 'NONE', #75327, #39241, #33467, .T. ) ;
#4771=AXIS2_PLACEMENT_3D ( 'NONE', #57895, #5901, #5422 ) ;
#4779=LINE ( 'NONE', #12262, #6644 ) ;
#4780=VECTOR ( 'NONE', #71970, 1000.000000000000114 ) ;
#4793=ORIENTED_EDGE ( 'NONE', *, *, #98702, .F. ) ;
#4802=PLANE ( 'NONE',  #6401 ) ;
#4803=VECTOR ( 'NONE', #82347, 1000.000000000000000 ) ;
#4804=LINE ( 'NONE', #27779, #1792 ) ;
#4813=ORIENTED_EDGE ( 'NONE', *, *, #70131, .F. ) ;
#4820=DIRECTION ( 'NONE',  ( 0.6626200482157357241, -0.000000000000000000, 0.7489557207890036317 ) ) ;
#4832=ORIENTED_EDGE ( 'NONE', *, *, #8372, .T. ) ;
#4833=LINE ( 'NONE', #24027, #89754 ) ;
#4834=CARTESIAN_POINT ( 'NONE',  ( 13.61464873478171178, 14.63606918187825201, -6.296136897217842865 ) ) ;
#4837=AXIS2_PLACEMENT_3D ( 'NONE', #3709, #88659, #96178 ) ;
#4840=CARTESIAN_POINT ( 'NONE',  ( -10.32896413005679470, 13.07879003517447458, 5.963430220938290560 ) ) ;
#4847=VERTEX_POINT ( 'NONE', #61812 ) ;
#4848=EDGE_CURVE ( 'NONE', #14809, #75433, #98872, .T. ) ;
#4858=EDGE_LOOP ( 'NONE', ( #269, #32627, #83795, #19104 ) ) ;
#4865=VERTEX_POINT ( 'NONE', #29834 ) ;
#4878=EDGE_LOOP ( 'NONE', ( #22808, #90174, #23553, #77987 ) ) ;
#4879=CYLINDRICAL_SURFACE ( 'NONE', #7182, 15.00000000000000000 ) ;
#4880=EDGE_CURVE ( 'NONE', #84834, #53609, #31354, .T. ) ;
#4884=CYLINDRICAL_SURFACE ( 'NONE', #21739, 11.25000000000000178 ) ;
#4903=EDGE_LOOP ( 'NONE', ( #95175, #80610, #75450, #11905, #78013 ) ) ;
#4910=CARTESIAN_POINT ( 'NONE',  ( -7.264948169187289473, 14.76930270348881002, -13.05597881399728699 ) ) ;
#4913=ORIENTED_EDGE ( 'NONE', *, *, #67842, .F. ) ;
#4921=DIRECTION ( 'NONE',  ( 0.008726535498360278933, 0.000000000000000000, 0.9999619230641714207 ) ) ;
#4944=ORIENTED_EDGE ( 'NONE', *, *, #42116, .T. ) ;
#4947=CARTESIAN_POINT ( 'NONE',  ( -12.54342190210052621, 14.76984988503095764, 8.116945096741206456 ) ) ;
#4952=DIRECTION ( 'NONE',  ( -0.4305110968082986878, 0.000000000000000000, 0.9025852843498588518 ) ) ;
#4960=CARTESIAN_POINT ( 'NONE',  ( 3.715841784917714108, -0.03417435944610275333, 15.55859621770270529 ) ) ;
#4961=CARTESIAN_POINT ( 'NONE',  ( -4.838527690343430443, 0.5000000000000004441, -14.19819177887733375 ) ) ;
#4966=CARTESIAN_POINT ( 'NONE',  ( 12.81628187352647252, -28.16803199673624292, -3.434112377981059172 ) ) ;
#4976=CIRCLE ( 'NONE', #8186, 14.49999999999999822 ) ;
#4991=CARTESIAN_POINT ( 'NONE',  ( -14.17193700899788134, 15.00000000000000000, -1.489530601564206247 ) ) ;
#4994=VERTEX_POINT ( 'NONE', #11273 ) ;
#4995=LINE ( 'NONE', #52455, #67780 ) ;
#5001=EDGE_CURVE ( 'NONE', #41516, #16129, #40805, .T. ) ;
#5002=FACE_OUTER_BOUND ( 'NONE', #78804, .T. ) ;
#5016=DIRECTION ( 'NONE',  ( 0.000000000000000000, 1.000000000000000000, 0.000000000000000000 ) ) ;
#5018=CARTESIAN_POINT ( 'NONE',  ( -3.795296366450322534, -34.23791783175269643, -14.16423886937409904 ) ) ;
#5032=CARTESIAN_POINT ( 'NONE',  ( 5.440088680355556150, 14.73035201082151247, 9.422509992056138373 ) ) ;
#5033=DIRECTION ( 'NONE',  ( -0.7132504491541751257, 0.000000000000000000, -0.7009092642998574485 ) ) ;
#5037=ORIENTED_EDGE ( 'NONE', *, *, #82084, .F. ) ;
#5042=VECTOR ( 'NONE', #62567, 1000.000000000000000 ) ;
#5044=FACE_OUTER_BOUND ( 'NONE', #18124, .T. ) ;
#5049=CARTESIAN_POINT ( 'NONE',  ( 13.75801628063878645, 15.00000000000000000, 4.578972376164554881 ) ) ;
#5050=CARTESIAN_POINT ( 'NONE',  ( 9.159723438033129383, -0.03417435944610275333, 10.91613331444548507 ) ) ;
#5052=ORIENTED_EDGE ( 'NONE', *, *, #47299, .T. ) ;
#5065=CARTESIAN_POINT ( 'NONE',  ( 13.95749458852080949, 0.2306972965111896423, -5.331641351773021675 ) ) ;
#5066=ORIENTED_EDGE ( 'NONE', *, *, #32622, .F. ) ;
#5079=CARTESIAN_POINT ( 'NONE',  ( 9.846743663894590881, 8.300597817667446421, 2.638427012816828565 ) ) ;
#5083=VERTEX_POINT ( 'NONE', #55299 ) ;
#5089=ADVANCED_FACE ( 'NONE', ( #66742 ), #24009, .T. ) ;
#5092=ORIENTED_EDGE ( 'NONE', *, *, #42012, .F. ) ;
#5095=VERTEX_POINT ( 'NONE', #43737 ) ;
#5114=AXIS2_PLACEMENT_3D ( 'NONE', #27559, #73547, #21060 ) ;
#5115=B_SPLINE_CURVE_WITH_KNOTS ( 'NONE', 3,
 ( #76016, #68032, #59037, #60019, #75520, #30010 ),
 .UNSPECIFIED., .F., .F.,
 ( 4, 2, 4 ),
 ( 0.0002800452451363350925, 0.0006862509172491815680, 0.001092456589362028043 ),
 .UNSPECIFIED. ) ;
#5117=VERTEX_POINT ( 'NONE', #41793 ) ;
#5123=ORIENTED_EDGE ( 'NONE', *, *, #30312, .T. ) ;
#5141=DIRECTION ( 'NONE',  ( 0.000000000000000000, 1.000000000000000000, 0.000000000000000000 ) ) ;
#5142=CARTESIAN_POINT ( 'NONE',  ( 8.606322355891363074, 4.859979058039186735E-16, -11.66967075398807374 ) ) ;
#5146=CARTESIAN_POINT ( 'NONE',  ( -5.440088680355547268, -26.10298132251182324, 9.422509992056143702 ) ) ;
#5150=CARTESIAN_POINT ( 'NONE',  ( 0.000000000000000000, 14.49999999999999822, 0.000000000000000000 ) ) ;
#5151=LINE ( 'NONE', #57151, #10080 ) ;
#5152=B_SPLINE_CURVE_WITH_KNOTS ( 'NONE', 3,
 ( #3505, #64467, #41998, #94001, #95978, #10993 ),
 .UNSPECIFIED., .F., .F.,
 ( 4, 2, 4 ),
 ( 3.409110551496115783E-05, 0.0004400426677367864632, 0.0008459942299586117008 ),
 .UNSPECIFIED. ) ;
#5154=ADVANCED_FACE ( 'NONE', ( #89245 ), #73246, .F. ) ;
#5178=CARTESIAN_POINT ( 'NONE',  ( 0.000000000000000000, 15.00000000000000000, 0.000000000000000000 ) ) ;
#5180=AXIS2_PLACEMENT_3D ( 'NONE', #6702, #73703, #5237 ) ;
#5181=CARTESIAN_POINT ( 'NONE',  ( 14.88232117145531141, 0.5000000000000004441, -1.875237731503139438 ) ) ;
#5184=ORIENTED_EDGE ( 'NONE', *, *, #64565, .F. ) ;
#5185=LINE ( 'NONE', #51169, #75688 ) ;
#5191=DIRECTION ( 'NONE',  ( -0.7132504491541751257, 0.000000000000000000, -0.7009092642998575595 ) ) ;
#5196=AXIS2_PLACEMENT_3D ( 'NONE', #85784, #86766, #47272 ) ;
#5199=AXIS2_PLACEMENT_3D ( 'NONE', #49610, #49136, #12119 ) ;
#5200=DIRECTION ( 'NONE',  ( 0.000000000000000000, 1.000000000000000000, 0.000000000000000000 ) ) ;
#5203=CARTESIAN_POINT ( 'NONE',  ( 0.000000000000000000, 15.00000000000000000, 0.000000000000000000 ) ) ;
#5212=CARTESIAN_POINT ( 'NONE',  ( 0.000000000000000000, 14.49999999999999822, 0.000000000000000000 ) ) ;
#5216=EDGE_CURVE ( 'NONE', #42731, #37334, #43103, .T. ) ;
#5219=CARTESIAN_POINT ( 'NONE',  ( -6.408140936763232709, 9.956968003263760636, 11.09922568453595026 ) ) ;
#5224=ORIENTED_EDGE ( 'NONE', *, *, #23694, .T. ) ;
#5225=TOROIDAL_SURFACE ( 'NONE', #37128, 14.49999999999999822, 0.5000000000000000000 ) ;
#5230=EDGE_CURVE ( 'NONE', #73066, #9875, #69217, .T. ) ;
#5237=DIRECTION ( 'NONE',  ( 4.263256414560601115E-14, 0.000000000000000000, 1.000000000000000000 ) ) ;
#5242=ADVANCED_FACE ( 'NONE', ( #13745 ), #52235, .F. ) ;
#5244=VERTEX_POINT ( 'NONE', #61211 ) ;
#5246=CARTESIAN_POINT ( 'NONE',  ( -13.30156849913876904, 0.2306972965111889762, -6.804875469488247397 ) ) ;
#5250=CARTESIAN_POINT ( 'NONE',  ( -14.47650479471817242, 0.5000000000000004441, -3.928206833722204028 ) ) ;
#5253=DIRECTION ( 'NONE',  ( 0.000000000000000000, 1.000000000000000000, 0.000000000000000000 ) ) ;
#5260=ORIENTED_EDGE ( 'NONE', *, *, #66249, .T. ) ;
#5261=CIRCLE ( 'NONE', #77052, 15.00000000000000000 ) ;
#5274=CARTESIAN_POINT ( 'NONE',  ( 3.795296366450314540, 3.262082168247304015, 14.16423886937410082 ) ) ;
#5286=DIRECTION ( 'NONE',  ( -0.9799247046208311440, 0.000000000000000000, 0.1993679344171901957 ) ) ;
#5287=CARTESIAN_POINT ( 'NONE',  ( 0.000000000000000000, 14.49999999999999822, 0.000000000000000000 ) ) ;
#5292=VERTEX_POINT ( 'NONE', #90719 ) ;
#5311=DIRECTION ( 'NONE',  ( -0.5075383629606967650, 0.000000000000000000, -0.8616291604415300398 ) ) ;
#5316=CARTESIAN_POINT ( 'NONE',  ( 0.000000000000000000, 15.00000000000000000, 0.000000000000000000 ) ) ;
#5328=ORIENTED_EDGE ( 'NONE', *, *, #4766, .F. ) ;
#5336=DIRECTION ( 'NONE',  ( -0.5519369853120617009, 0.000000000000000000, 0.8338858220671658827 ) ) ;
#5340=VECTOR ( 'NONE', #53191, 1000.000000000000227 ) ;
#5365=CARTESIAN_POINT ( 'NONE',  ( 10.64017930668202183, 0.3639309529147286004, 10.57291749337224296 ) ) ;
#5375=ORIENTED_EDGE ( 'NONE', *, *, #66083, .F. ) ;
#5378=CARTESIAN_POINT ( 'NONE',  ( 6.898461952320324109, 15.00000000000000000, 12.75387089053312373 ) ) ;
#5384=ORIENTED_EDGE ( 'NONE', *, *, #66318, .F. ) ;
#5385=CARTESIAN_POINT ( 'NONE',  ( -9.399392868737665552, 3.795627280083113010E-16, -11.04089732309487104 ) ) ;
#5392=LINE ( 'NONE', #81367, #64332 ) ;
#5399=CARTESIAN_POINT ( 'NONE',  ( 4.267749253172036461, 0.000000000000000000, 3.394721039305376387 ) ) ;
#5402=ORIENTED_EDGE ( 'NONE', *, *, #67548, .T. ) ;
#5403=CIRCLE ( 'NONE', #61273, 15.00000000000000000 ) ;
#5408=CARTESIAN_POINT ( 'NONE',  ( -3.014428414850141458, 6.880135511184874986, -11.24999999999999822 ) ) ;
#5414=ORIENTED_EDGE ( 'NONE', *, *, #90421, .T. ) ;
#5416=CARTESIAN_POINT ( 'NONE',  ( -10.82078848414227146, 15.00000000000000000, 11.78082904627290795 ) ) ;
#5417=LINE ( 'NONE', #35395, #87722 ) ;
#5420=CARTESIAN_POINT ( 'NONE',  ( 14.43100913236846772, 15.00000000000000000, 1.412789942453269054 ) ) ;
#5422=DIRECTION ( 'NONE',  ( 0.000000000000000000, 0.000000000000000000, 1.000000000000000000 ) ) ;
#5428=DIRECTION ( 'NONE',  ( -0.000000000000000000, -1.000000000000000000, -0.000000000000000000 ) ) ;
#5447=ORIENTED_EDGE ( 'NONE', *, *, #15921, .F. ) ;
#5450=CARTESIAN_POINT ( 'NONE',  ( 5.991992585808628036, 4.207234274712436881E-16, -13.20401548210295140 ) ) ;
#5454=ADVANCED_FACE ( 'NONE', ( #61689 ), #60712, .T. ) ;
#5456=CARTESIAN_POINT ( 'NONE',  ( 14.82269085861167035, 0.5000000000000004441, 2.299529454047060550 ) ) ;
#5461=FACE_OUTER_BOUND ( 'NONE', #89791, .T. ) ;
#5463=DIRECTION ( 'NONE',  ( 0.000000000000000000, 1.000000000000000000, 0.000000000000000000 ) ) ;
#5466=DIRECTION ( 'NONE',  ( -0.1650476058606810681, 0.000000000000000000, 0.9862856015372308827 ) ) ;
#5468=CARTESIAN_POINT ( 'NONE',  ( -3.434112377981067610, -11.91803199673624292, -12.81628187352647252 ) ) ;
#5484=ORIENTED_EDGE ( 'NONE', *, *, #27324, .F. ) ;
#5501=DIRECTION ( 'NONE',  ( 0.000000000000000000, 1.000000000000000000, 0.000000000000000000 ) ) ;
#5507=ORIENTED_EDGE ( 'NONE', *, *, #65382, .T. ) ;
#5514=AXIS2_PLACEMENT_3D ( 'NONE', #1767, #78227, #10237 ) ;
#5515=DIRECTION ( 'NONE',  ( 0.000000000000000000, 1.000000000000000000, 0.000000000000000000 ) ) ;
#5517=CARTESIAN_POINT ( 'NONE',  ( -14.16423886937410437, -23.40458449841936428, -3.795296366450299885 ) ) ;
#5531=CARTESIAN_POINT ( 'NONE',  ( -5.440088680355547268, 33.89701867748817676, 9.422509992056143702 ) ) ;
#5535=ORIENTED_EDGE ( 'NONE', *, *, #71276, .T. ) ;
#5548=CARTESIAN_POINT ( 'NONE',  ( 13.96552416078064063, 14.95037115134969241, 4.756200848675177006 ) ) ;
#5557=CARTESIAN_POINT ( 'NONE',  ( 0.000000000000000000, 0.5000000000000004441, 0.000000000000000000 ) ) ;
#5562=CARTESIAN_POINT ( 'NONE',  ( 5.795997163830165277, -0.03417435944610275333, -13.01802277140705932 ) ) ;
#5564=LINE ( 'NONE', #36040, #53827 ) ;
#5571=EDGE_CURVE ( 'NONE', #83513, #20604, #50436, .T. ) ;
#5573=AXIS2_PLACEMENT_3D ( 'NONE', #5287, #6262, #36765 ) ;
#5575=DIRECTION ( 'NONE',  ( 0.000000000000000000, 1.000000000000000000, 0.000000000000000000 ) ) ;
#5581=CARTESIAN_POINT ( 'NONE',  ( -14.26139399674459263, 4.837279266207889341E-16, 2.619664342929711509 ) ) ;
#5584=CARTESIAN_POINT ( 'NONE',  ( 9.846743663894590881, 18.30059781766744820, 2.638427012816828565 ) ) ;
#5585=ORIENTED_EDGE ( 'NONE', *, *, #97321, .F. ) ;
#5586=VERTEX_POINT ( 'NONE', #77194 ) ;
#5605=DIRECTION ( 'NONE',  ( -0.000000000000000000, -1.000000000000000000, -0.000000000000000000 ) ) ;
#5608=ORIENTED_EDGE ( 'NONE', *, *, #17531, .T. ) ;
#5616=CARTESIAN_POINT ( 'NONE',  ( 12.80781515976314822, 15.00000000000000000, -6.246788841744324472 ) ) ;
#5620=CARTESIAN_POINT ( 'NONE',  ( -9.065164099344370285, 0.5000000000000004441, -11.95084933600779564 ) ) ;
#5622=DIRECTION ( 'NONE',  ( 0.000000000000000000, 1.000000000000000000, 0.000000000000000000 ) ) ;
#5627=DIRECTION ( 'NONE',  ( 0.000000000000000000, 1.000000000000000000, 0.000000000000000000 ) ) ;
#5630=CARTESIAN_POINT ( 'NONE',  ( 0.000000000000000000, 0.5000000000000004441, 0.000000000000000000 ) ) ;
#5631=CIRCLE ( 'NONE', #50358, 14.49999999999999822 ) ;
#5638=CARTESIAN_POINT ( 'NONE',  ( -4.084234479374258875, 0.000000000000000000, -3.613425430272983352 ) ) ;
#5645=CARTESIAN_POINT ( 'NONE',  ( -7.964842623401179544, -22.56131465584515894, -7.964842623401174215 ) ) ;
#5650=CARTESIAN_POINT ( 'NONE',  ( 0.000000000000000000, 0.5000000000000004441, 0.000000000000000000 ) ) ;
#5651=VECTOR ( 'NONE', #850, 1000.000000000000000 ) ;
#5653=DIRECTION ( 'NONE',  ( -0.9890158633619177131, 0.000000000000000000, 0.1478094111296046342 ) ) ;
#5658=VECTOR ( 'NONE', #2728, 1000.000000000000000 ) ;
#5672=CARTESIAN_POINT ( 'NONE',  ( -7.551349515323269479, 15.00000000000000000, 12.08468537022900868 ) ) ;
#5678=ORIENTED_EDGE ( 'NONE', *, *, #87817, .T. ) ;
#5679=CARTESIAN_POINT ( 'NONE',  ( -14.88232117145529365, 0.3640475087720984049, -1.875237731503342609 ) ) ;
#5695=CARTESIAN_POINT ( 'NONE',  ( 7.208316651077762316, -35.86606884899921255, -7.208316651077764980 ) ) ;
#5698=ORIENTED_EDGE ( 'NONE', *, *, #88507, .F. ) ;
#5703=CARTESIAN_POINT ( 'NONE',  ( 10.64017930668205736, 15.00000000000000000, -10.57291749337215592 ) ) ;
#5707=CARTESIAN_POINT ( 'NONE',  ( 3.434112377981054287, 12.66530133659709101, -12.81628187352647608 ) ) ;
#5708=ORIENTED_EDGE ( 'NONE', *, *, #7546, .T. ) ;
#5711=VERTEX_POINT ( 'NONE', #40186 ) ;
#5713=ADVANCED_FACE ( 'NONE', ( #24702 ), #9690, .F. ) ;
#5717=DIRECTION ( 'NONE',  ( -0.3826834323650877279, 0.000000000000000000, -0.9238795325112876267 ) ) ;
#5724=FACE_OUTER_BOUND ( 'NONE', #13078, .T. ) ;
#5731=ADVANCED_FACE ( 'NONE', ( #84709 ), #70693, .T. ) ;
#5738=CARTESIAN_POINT ( 'NONE',  ( -14.42571047809455642, 0.2306972965111904750, -3.890621016588054815 ) ) ;
#5742=TOROIDAL_SURFACE ( 'NONE', #87158, 14.49999999999999822, 0.5000000000000000000 ) ;
#5745=FACE_OUTER_BOUND ( 'NONE', #26438, .T. ) ;
#5746=AXIS2_PLACEMENT_3D ( 'NONE', #95832, #27314, #58297 ) ;
#5749=ORIENTED_EDGE ( 'NONE', *, *, #4333, .F. ) ;
#5750=CARTESIAN_POINT ( 'NONE',  ( 3.897244926436219892, 4.401207273199346175E-16, -13.96644127841330807 ) ) ;
#5757=CARTESIAN_POINT ( 'NONE',  ( 0.000000000000000000, 0.5000000000000004441, 0.000000000000000000 ) ) ;
#5761=CARTESIAN_POINT ( 'NONE',  ( -12.26659068614895354, 11.38708216824730535, -7.082119434687038861 ) ) ;
#5769=EDGE_LOOP ( 'NONE', ( #94368, #14118, #42047, #79944 ) ) ;
#5773=FACE_OUTER_BOUND ( 'NONE', #62963, .T. ) ;
#5781=FACE_OUTER_BOUND ( 'NONE', #20887, .T. ) ;
#5797=ADVANCED_FACE ( 'NONE', ( #63165 ), #53575, .T. ) ;
#5809=ORIENTED_EDGE ( 'NONE', *, *, #98463, .T. ) ;
#5811=EDGE_LOOP ( 'NONE', ( #23535, #58184, #19969, #31551 ) ) ;
#5813=VERTEX_POINT ( 'NONE', #17208 ) ;
#5820=PLANE ( 'NONE',  #35601 ) ;
#5824=ORIENTED_EDGE ( 'NONE', *, *, #68460, .T. ) ;
#5826=ORIENTED_EDGE ( 'NONE', *, *, #43014, .T. ) ;
#5831=CARTESIAN_POINT ( 'NONE',  ( 14.24131928502211686, -0.03417435944610275333, -0.4973178280105898241 ) ) ;
#5834=EDGE_CURVE ( 'NONE', #92561, #38139, #98147, .T. ) ;
#5835=AXIS2_PLACEMENT_3D ( 'NONE', #47170, #64133, #94155 ) ;
#5853=FACE_OUTER_BOUND ( 'NONE', #69431, .T. ) ;
#5856=CARTESIAN_POINT ( 'NONE',  ( -10.70613742633263321, 15.00000000000000000, 9.778988772285140740 ) ) ;
#5857=DIRECTION ( 'NONE',  ( 0.000000000000000000, 0.000000000000000000, -1.000000000000000000 ) ) ;
#5860=CARTESIAN_POINT ( 'NONE',  ( 5.624999999999999112, 8.451366962315987053, -9.742785792574936821 ) ) ;
#5864=ORIENTED_EDGE ( 'NONE', *, *, #69035, .F. ) ;
#5865=EDGE_CURVE ( 'NONE', #34058, #91342, #57562, .T. ) ;
#5866=LINE ( 'NONE', #22849, #40869 ) ;
#5872=CARTESIAN_POINT ( 'NONE',  ( -10.93781366033354097, 0.5000000000000004441, 10.26470809774057713 ) ) ;
#5876=LINE ( 'NONE', #60835, #64089 ) ;
#5896=ORIENTED_EDGE ( 'NONE', *, *, #74548, .T. ) ;
#5901=DIRECTION ( 'NONE',  ( 0.000000000000000000, 1.000000000000000000, 0.000000000000000000 ) ) ;
#5912=AXIS2_PLACEMENT_3D ( 'NONE', #17568, #11518, #18051 ) ;
#5923=EDGE_CURVE ( 'NONE', #19871, #84722, #88762, .T. ) ;
#5926=PRODUCT ( '1.3 Adjustment Nut', '1.3 Adjustment Nut', '', ( #13731 ) ) ;
#5928=VERTEX_POINT ( 'NONE', #88132 ) ;
#5935=ORIENTED_EDGE ( 'NONE', *, *, #46190, .T. ) ;
#5942=CARTESIAN_POINT ( 'NONE',  ( 1.377727649040772586E-15, 2.500000000000005773, 11.25000000000000178 ) ) ;
#5946=AXIS2_PLACEMENT_3D ( 'NONE', #16920, #55902, #47396 ) ;
#5950=ORIENTED_EDGE ( 'NONE', *, *, #29158, .T. ) ;
#5952=CARTESIAN_POINT ( 'NONE',  ( 3.469446951953614189E-15, -24.62636533006957507, 12.81628187352647608 ) ) ;
#5960=CARTESIAN_POINT ( 'NONE',  ( -13.34343830728408697, 0.5000000000000004441, 6.852200678592504701 ) ) ;
#5961=ORIENTED_EDGE ( 'NONE', *, *, #60392, .T. ) ;
#5968=TOROIDAL_SURFACE ( 'NONE', #18749, 14.49999999999999822, 0.5000000000000000000 ) ;
#5973=EDGE_CURVE ( 'NONE', #14667, #61835, #64761, .T. ) ;
#5978=CARTESIAN_POINT ( 'NONE',  ( 12.15129255554608534, 15.00000000000000000, 10.40305174771247998 ) ) ;
#6005=CARTESIAN_POINT ( 'NONE',  ( 12.26659068614894466, -20.27958449841936073, -7.082119434687053960 ) ) ;
#6021=CARTESIAN_POINT ( 'NONE',  ( -7.964842623401179544, 27.43868534415484461, -7.964842623401174215 ) ) ;
#6026=ORIENTED_EDGE ( 'NONE', *, *, #28276, .F. ) ;
#6049=CARTESIAN_POINT ( 'NONE',  ( 13.07751017357383994, 4.340377266345630487E-16, -6.263284095430506682 ) ) ;
#6051=CARTESIAN_POINT ( 'NONE',  ( -14.29730467490344736, 15.00000000000000000, 2.416004766801328696 ) ) ;
#6053=AXIS2_PLACEMENT_3D ( 'NONE', #16267, #78731, #15780 ) ;
#6064=PLANE ( 'NONE',  #71575 ) ;
#6067=CARTESIAN_POINT ( 'NONE',  ( -2.638427012816824124, 17.05059781766745530, 9.846743663894596210 ) ) ;
#6070=CARTESIAN_POINT ( 'NONE',  ( 1.236355250167371800, 14.95037107271117982, -14.70131747622448515 ) ) ;
#6078=B_SPLINE_CURVE_WITH_KNOTS ( 'NONE', 3,
 ( #59617, #98649, #36641, #67124, #51639, #15131 ),
 .UNSPECIFIED., .F., .F.,
 ( 4, 2, 4 ),
 ( 3.409110551496073092E-05, 0.0004400426677367845658, 0.0008459942299586083398 ),
 .UNSPECIFIED. ) ;
#6089=EDGE_CURVE ( 'NONE', #72594, #61531, #72629, .T. ) ;
#6090=FACE_OUTER_BOUND ( 'NONE', #59272, .T. ) ;
#6093=EDGE_CURVE ( 'NONE', #37275, #74987, #90320, .T. ) ;
#6094=AXIS2_PLACEMENT_3D ( 'NONE', #88938, #89430, #29899 ) ;
#6096=ORIENTED_EDGE ( 'NONE', *, *, #42064, .T. ) ;
#6104=CARTESIAN_POINT ( 'NONE',  ( -7.595945211628411187, 15.00000000000000000, 12.35117874301633734 ) ) ;
#6106=LINE ( 'NONE', #21611, #17970 ) ;
#6110=DIRECTION ( 'NONE',  ( 0.8870108331782213806, 0.000000000000000000, -0.4617486132350345773 ) ) ;
#6113=AXIS2_PLACEMENT_3D ( 'NONE', #45266, #91755, #10715 ) ;
#6116=EDGE_CURVE ( 'NONE', #84655, #12575, #23277, .T. ) ;
#6118=EDGE_CURVE ( 'NONE', #66530, #50127, #36633, .T. ) ;
#6127=DIRECTION ( 'NONE',  ( 0.9723699203976789995, 0.000000000000000000, -0.2334453638558957045 ) ) ;
#6132=CARTESIAN_POINT ( 'NONE',  ( 5.440088680355556150, -5.269647989178491088, 9.422509992056138373 ) ) ;
#6136=CARTESIAN_POINT ( 'NONE',  ( 4.862001128006773421, 4.807100664002271835E-16, -13.66056166602460031 ) ) ;
#6143=EDGE_CURVE ( 'NONE', #10324, #49672, #16466, .T. ) ;
#6147=ORIENTED_EDGE ( 'NONE', *, *, #58991, .T. ) ;
#6155=LINE ( 'NONE', #21160, #74563 ) ;
#6162=ORIENTED_EDGE ( 'NONE', *, *, #19398, .F. ) ;
#6180=CARTESIAN_POINT ( 'NONE',  ( 7.208316651077764980, -22.11606884899921610, 7.208316651077762316 ) ) ;
#6191=LINE ( 'NONE', #82675, #29461 ) ;
#6192=TOROIDAL_SURFACE ( 'NONE', #62051, 14.49999999999999822, 0.5000000000000000000 ) ;
#6196=CARTESIAN_POINT ( 'NONE',  ( 3.434112377981054287, 27.66530133659709279, -12.81628187352647608 ) ) ;
#6197=ORIENTED_EDGE ( 'NONE', *, *, #11929, .F. ) ;
#6200=ORIENTED_EDGE ( 'NONE', *, *, #28772, .T. ) ;
#6206=PLANE ( 'NONE',  #46385 ) ;
#6209=ADVANCED_FACE ( 'NONE', ( #67117 ), #90107, .F. ) ;
#6210=CARTESIAN_POINT ( 'NONE',  ( -1.087200977609927843, 0.000000000000000000, -5.343763529286924552 ) ) ;
#6211=ORIENTED_EDGE ( 'NONE', *, *, #22377, .F. ) ;
#6212=CARTESIAN_POINT ( 'NONE',  ( -13.55255535720589322, 0.000000000000000000, -4.403492169843143067 ) ) ;
#6213=DIRECTION ( 'NONE',  ( -0.9238795325112876267, 0.000000000000000000, -0.3826834323650877279 ) ) ;
#6218=CARTESIAN_POINT ( 'NONE',  ( 3.897244926435189161, 15.00000000000000000, 13.96644127842154148 ) ) ;
#6219=ORIENTED_EDGE ( 'NONE', *, *, #72351, .T. ) ;
#6226=B_SPLINE_CURVE_WITH_KNOTS ( 'NONE', 3,
 ( #38452, #38943, #7956, #31414, #83943, #23946 ),
 .UNSPECIFIED., .F., .F.,
 ( 4, 2, 4 ),
 ( 3.409110551495695654E-05, 0.0004400426677367964921, 0.0008459942299586360953 ),
 .UNSPECIFIED. ) ;
#6227=PLANE ( 'NONE',  #43194 ) ;
#6228=CARTESIAN_POINT ( 'NONE',  ( 8.721827932831768493, -3.224654430197120208E-15, 11.74045266257181375 ) ) ;
#6230=CARTESIAN_POINT ( 'NONE',  ( -10.93781366033333136, 0.5000000000000004441, -10.26470809774080628 ) ) ;
#6234=EDGE_CURVE ( 'NONE', #86532, #77069, #8953, .T. ) ;
#6237=EDGE_CURVE ( 'NONE', #43424, #85655, #91911, .T. ) ;
#6248=CARTESIAN_POINT ( 'NONE',  ( 1.796645268984623511, 0.2306972965111892537, 14.83273813124059615 ) ) ;
#6249=CARTESIAN_POINT ( 'NONE',  ( -5.204170427930421283E-15, 15.55374883491396965, -14.16423886937410082 ) ) ;
#6262=DIRECTION ( 'NONE',  ( 0.000000000000000000, 1.000000000000000000, 0.000000000000000000 ) ) ;
#6279=EDGE_CURVE ( 'NONE', #21503, #3919, #24908, .T. ) ;
#6285=DIRECTION ( 'NONE',  ( -0.9238795325112876267, 0.000000000000000000, 0.3826834323650877279 ) ) ;
#6298=VECTOR ( 'NONE', #51862, 1000.000000000000227 ) ;
#6302=ORIENTED_EDGE ( 'NONE', *, *, #34725, .T. ) ;
#6305=DIRECTION ( 'NONE',  ( 0.7372773368101297464, 0.000000000000000000, -0.6755902076156540259 ) ) ;
#6306=VERTEX_POINT ( 'NONE', #52118 ) ;
#6316=DIRECTION ( 'NONE',  ( -0.4146932426562339180, 0.000000000000000000, -0.9099612708765455471 ) ) ;
#6319=EDGE_CURVE ( 'NONE', #45246, #51268, #6614, .T. ) ;
#6325=DIRECTION ( 'NONE',  ( -0.7132504491541751257, 0.000000000000000000, -0.7009092642998574485 ) ) ;
#6332=AXIS2_PLACEMENT_3D ( 'NONE', #5831, #6316, #36823 ) ;
#6334=LINE ( 'NONE', #19856, #69491 ) ;
#6338=EDGE_LOOP ( 'NONE', ( #83126, #95982, #84054, #41437 ) ) ;
#6348=EDGE_CURVE ( 'NONE', #29544, #97832, #39949, .T. ) ;
#6355=AXIS2_PLACEMENT_3D ( 'NONE', #21367, #27867, #43363 ) ;
#6367=DIRECTION ( 'NONE',  ( -0.5664062369248259454, 0.000000000000000000, -0.8241261886220204724 ) ) ;
#6387=ADVANCED_FACE ( 'NONE', ( #98132 ), #54933, .F. ) ;
#6401=AXIS2_PLACEMENT_3D ( 'NONE', #35278, #28275, #49788 ) ;
#6405=ORIENTED_EDGE ( 'NONE', *, *, #65569, .F. ) ;
#6417=DIRECTION ( 'NONE',  ( -0.000000000000000000, -1.000000000000000000, -0.000000000000000000 ) ) ;
#6421=CARTESIAN_POINT ( 'NONE',  ( 8.470640952597488393, 15.00000000000000711, 11.92295067084773130 ) ) ;
#6428=CARTESIAN_POINT ( 'NONE',  ( 9.382169495545419124, -24.00136533006957507, 9.382169495545417348 ) ) ;
#6431=CARTESIAN_POINT ( 'NONE',  ( -4.838527690343710219, 14.49999999999999112, 14.19819177887730355 ) ) ;
#6438=EDGE_CURVE ( 'NONE', #87330, #86977, #58613, .T. ) ;
#6440=EDGE_CURVE ( 'NONE', #43121, #57214, #76516, .T. ) ;
#6450=EDGE_CURVE ( 'NONE', #70139, #94698, #18080, .T. ) ;
#6460=AXIS2_PLACEMENT_3D ( 'NONE', #14285, #44758, #22771 ) ;
#6462=LINE ( 'NONE', #21474, #34205 ) ;
#6466=VECTOR ( 'NONE', #21900, 1000.000000000000000 ) ;
#6468=CARTESIAN_POINT ( 'NONE',  ( -14.82629065241270716, 0.2301504708693010715, 1.844815641835153563 ) ) ;
#6476=CARTESIAN_POINT ( 'NONE',  ( -11.36220558718868290, 15.00000000000000000, 9.008345252845137097 ) ) ;
#6480=AXIS2_PLACEMENT_3D ( 'NONE', #53177, #45680, #76178 ) ;
#6486=CARTESIAN_POINT ( 'NONE',  ( 7.082119434687054849, -21.52958449841935717, 12.26659068614894288 ) ) ;
#6498=CARTESIAN_POINT ( 'NONE',  ( -6.761389522993706436, 0.2306972965111901419, -13.32372569557309028 ) ) ;
#6499=VECTOR ( 'NONE', #7123, 1000.000000000000000 ) ;
#6500=CARTESIAN_POINT ( 'NONE',  ( -9.422509992056145478, 22.64701867748818032, -5.440088680355541939 ) ) ;
#6506=VERTEX_POINT ( 'NONE', #3923 ) ;
#6509=EDGE_CURVE ( 'NONE', #74408, #84772, #45669, .T. ) ;
#6520=ORIENTED_EDGE ( 'NONE', *, *, #79035, .T. ) ;
#6530=CARTESIAN_POINT ( 'NONE',  ( 0.000000000000000000, 0.5000000000000004441, 0.000000000000000000 ) ) ;
#6542=CARTESIAN_POINT ( 'NONE',  ( 3.881909499399555319, 14.99999999999807976, 14.10103859408278915 ) ) ;
#6549=AXIS2_PLACEMENT_3D ( 'NONE', #70594, #83753, #18574 ) ;
#6551=CARTESIAN_POINT ( 'NONE',  ( 2.638427012816829897, 9.550597817667449974, -9.846743663894592657 ) ) ;
#6553=ORIENTED_EDGE ( 'NONE', *, *, #6116, .T. ) ;
#6555=ADVANCED_FACE ( 'NONE', ( #78433 ), #80407, .T. ) ;
#6569=ORIENTED_EDGE ( 'NONE', *, *, #88215, .F. ) ;
#6577=EDGE_CURVE ( 'NONE', #43285, #68868, #65601, .T. ) ;
#6578=AXIS2_PLACEMENT_3D ( 'NONE', #11279, #54801, #72270 ) ;
#6579=LINE ( 'NONE', #92529, #65035 ) ;
#6580=ORIENTED_EDGE ( 'NONE', *, *, #85472, .F. ) ;
#6581=AXIS2_PLACEMENT_3D ( 'NONE', #81999, #75488, #29975 ) ;
#6583=ORIENTED_EDGE ( 'NONE', *, *, #75639, .T. ) ;
#6584=DIRECTION ( 'NONE',  ( 0.000000000000000000, 1.000000000000000000, 0.000000000000000000 ) ) ;
#6586=EDGE_CURVE ( 'NONE', #12985, #90692, #50887, .T. ) ;
#6590=DIRECTION ( 'NONE',  ( 0.000000000000000000, 0.000000000000000000, 1.000000000000000000 ) ) ;
#6593=ORIENTED_EDGE ( 'NONE', *, *, #40925, .T. ) ;
#6596=FACE_OUTER_BOUND ( 'NONE', #91739, .T. ) ;
#6611=DIRECTION ( 'NONE',  ( -0.3338068592337842810, -0.000000000000000000, 0.9426414910921737667 ) ) ;
#6613=LINE ( 'NONE', #37620, #91767 ) ;
#6614=LINE ( 'NONE', #89620, #28022 ) ;
#6618=CARTESIAN_POINT ( 'NONE',  ( -9.422509992056145478, -12.35298132251182146, -5.440088680355541939 ) ) ;
#6627=B_SPLINE_CURVE_WITH_KNOTS ( 'NONE', 3,
 ( #82035, #74531, #5065, #57556, #36042, #50064 ),
 .UNSPECIFIED., .F., .F.,
 ( 4, 2, 4 ),
 ( 3.409110551496108329E-05, 0.0004400426677367861921, 0.0008459942299586113755 ),
 .UNSPECIFIED. ) ;
#6642=CARTESIAN_POINT ( 'NONE',  ( 0.000000000000000000, 15.00000000000000000, 0.000000000000000000 ) ) ;
#6644=VECTOR ( 'NONE', #42771, 1000.000000000000000 ) ;
#6646=ORIENTED_EDGE ( 'NONE', *, *, #5230, .F. ) ;
#6652=AXIS2_PLACEMENT_3D ( 'NONE', #63315, #69860, #62832 ) ;
#6653=CARTESIAN_POINT ( 'NONE',  ( -14.40939250469963895, 4.354406223596783273E-16, -1.618458416365949226 ) ) ;
#6669=CARTESIAN_POINT ( 'NONE',  ( -3.469446951953614189E-15, -25.24106884899920900, -9.846743663894594434 ) ) ;
#6673=ORIENTED_EDGE ( 'NONE', *, *, #69829, .F. ) ;
#6683=CARTESIAN_POINT ( 'NONE',  ( 11.09922568453594671, 22.04030133659709634, -6.408140936763241591 ) ) ;
#6684=EDGE_CURVE ( 'NONE', #42806, #68457, #93409, .T. ) ;
#6686=AXIS2_PLACEMENT_3D ( 'NONE', #65324, #88338, #52796 ) ;
#6689=ORIENTED_EDGE ( 'NONE', *, *, #1534, .T. ) ;
#6696=CARTESIAN_POINT ( 'NONE',  ( -3.715841784917612856, -0.03417435944610275333, -15.55859621770273193 ) ) ;
#6700=ORIENTED_EDGE ( 'NONE', *, *, #93124, .T. ) ;
#6702=CARTESIAN_POINT ( 'NONE',  ( 0.000000000000000000, 14.49999999999999822, 0.000000000000000000 ) ) ;
#6704=CARTESIAN_POINT ( 'NONE',  ( -12.50534872682736065, 15.00000000000000000, 7.339363270777414350 ) ) ;
#6711=DIRECTION ( 'NONE',  ( 0.000000000000000000, 0.000000000000000000, 1.000000000000000000 ) ) ;
#6724=FACE_OUTER_BOUND ( 'NONE', #70596, .T. ) ;
#6725=AXIS2_PLACEMENT_3D ( 'NONE', #87202, #18230, #1770 ) ;
#6728=DIRECTION ( 'NONE',  ( 0.000000000000000000, 0.000000000000000000, 1.000000000000000000 ) ) ;
#6732=CARTESIAN_POINT ( 'NONE',  ( -14.62617646268082972, 0.5000000000000004441, -3.327906561567078647 ) ) ;
#6733=DIRECTION ( 'NONE',  ( -0.3007057995042635157, 0.000000000000000000, -0.9537169507482300412 ) ) ;
#6738=PRODUCT_DEFINITION_SHAPE ( 'NONE', 'NONE',  #4342 ) ;
#6741=CARTESIAN_POINT ( 'NONE',  ( 10.36894250292378850, 19.92874883491397497, -10.36894250292379027 ) ) ;
#6754=LINE ( 'NONE', #70713, #24832 ) ;
#6773=AXIS2_PLACEMENT_3D ( 'NONE', #92335, #68370, #8347 ) ;
#6776=EDGE_CURVE ( 'NONE', #4994, #23295, #36530, .T. ) ;
#6794=ORIENTED_EDGE ( 'NONE', *, *, #69233, .F. ) ;
#6801=ORIENTED_EDGE ( 'NONE', *, *, #18314, .F. ) ;
#6803=CIRCLE ( 'NONE', #62663, 14.49999999999999822 ) ;
#6804=EDGE_CURVE ( 'NONE', #97117, #46057, #21886, .T. ) ;
#6805=EDGE_CURVE ( 'NONE', #48230, #25555, #61427, .T. ) ;
#6808=DIRECTION ( 'NONE',  ( 0.000000000000000000, 0.000000000000000000, 1.000000000000000000 ) ) ;
#6812=DIRECTION ( 'NONE',  ( 0.000000000000000000, 1.000000000000000000, 0.000000000000000000 ) ) ;
#6818=ORIENTED_EDGE ( 'NONE', *, *, #66898, .F. ) ;
#6827=CARTESIAN_POINT ( 'NONE',  ( -14.54804176595373555, -0.03417435944610275333, -6.650705016170777917 ) ) ;
#6837=EDGE_CURVE ( 'NONE', #69558, #40424, #80612, .T. ) ;
#6859=EDGE_LOOP ( 'NONE', ( #14580, #4614, #64215, #56215 ) ) ;
#6860=CARTESIAN_POINT ( 'NONE',  ( 6.728851239469101131, -3.114116630580434013E-15, -12.98580270086200628 ) ) ;
#6863=B_SPLINE_CURVE_WITH_KNOTS ( 'NONE', 3,
 ( #88681, #88184, #42214, #26698, #13176, #35685 ),
 .UNSPECIFIED., .F., .F.,
 ( 4, 2, 4 ),
 ( 3.409110551495928758E-05, 0.0004400426677367854332, 0.0008459942299586115924 ),
 .UNSPECIFIED. ) ;
#6869=EDGE_LOOP ( 'NONE', ( #67732, #17552, #6553, #46287 ) ) ;
#6872=FACE_OUTER_BOUND ( 'NONE', #76542, .T. ) ;
#6873=CARTESIAN_POINT ( 'NONE',  ( -12.98685442714190508, 15.00000000000000000, -6.449155920601135072 ) ) ;
#6879=ORIENTED_EDGE ( 'NONE', *, *, #53053, .F. ) ;
#6885=DIRECTION ( 'NONE',  ( -0.000000000000000000, -1.000000000000000000, -0.000000000000000000 ) ) ;
#6886=LINE ( 'NONE', #12897, #3265 ) ;
#6891=CARTESIAN_POINT ( 'NONE',  ( -8.731067818237040257, 2.037123368507817389, -8.731067818237033151 ) ) ;
#6895=AXIS2_PLACEMENT_3D ( 'NONE', #70355, #76855, #8368 ) ;
#6900=CIRCLE ( 'NONE', #49997, 15.00000000000000000 ) ;
#6904=CARTESIAN_POINT ( 'NONE',  ( 5.803070148808322948, 15.00000000000000000, -13.28812917035385510 ) ) ;
#6913=VECTOR ( 'NONE', #30304, 1000.000000000000000 ) ;
#6917=CARTESIAN_POINT ( 'NONE',  ( -12.25993886608597094, 14.49999999999999112, -8.642563219313844414 ) ) ;
#6919=ORIENTED_EDGE ( 'NONE', *, *, #76963, .T. ) ;
#6928=CARTESIAN_POINT ( 'NONE',  ( 8.134956207566084174, -0.03417435944610275333, -13.77315809598639085 ) ) ;
#6933=ORIENTED_EDGE ( 'NONE', *, *, #25432, .F. ) ;
#6935=CARTESIAN_POINT ( 'NONE',  ( -12.81628187352647252, -15.66803199673624114, 3.434112377981066722 ) ) ;
#6945=VECTOR ( 'NONE', #38937, 1000.000000000000000 ) ;
#6958=EDGE_CURVE ( 'NONE', #49583, #50673, #45861, .T. ) ;
#6970=VECTOR ( 'NONE', #74583, 1000.000000000000000 ) ;
#6974=ADVANCED_FACE ( 'NONE', ( #30842 ), #98218, .T. ) ;
#6980=CARTESIAN_POINT ( 'NONE',  ( -3.836325488035984499, 14.63606917487569703, -14.50112432709431864 ) ) ;
#6984=B_SPLINE_CURVE_WITH_KNOTS ( 'NONE', 3,
 ( #45132, #44138, #29139, #30122, #67151, #52150 ),
 .UNSPECIFIED., .F., .F.,
 ( 4, 2, 4 ),
 ( 3.409110551494650755E-05, 0.0004400426677367923721, 0.0008459942299586382638 ),
 .UNSPECIFIED. ) ;
#6988=DIRECTION ( 'NONE',  ( -1.776356839400250780E-14, 0.000000000000000000, 1.000000000000000000 ) ) ;
#6991=CARTESIAN_POINT ( 'NONE',  ( -14.16423886937409726, -22.98791783175269643, 3.795296366450320757 ) ) ;
#7002=CARTESIAN_POINT ( 'NONE',  ( 1.354709868695545216, 14.49999999999999112, 14.93870011653158336 ) ) ;
#7004=CARTESIAN_POINT ( 'NONE',  ( 7.964842623401181321, 24.93868534415484461, 7.964842623401174215 ) ) ;
#7009=DIRECTION ( 'NONE',  ( 0.000000000000000000, 0.000000000000000000, 1.000000000000000000 ) ) ;
#7012=EDGE_CURVE ( 'NONE', #92653, #97221, #25730, .T. ) ;
#7014=PLANE ( 'NONE',  #20966 ) ;
#7022=DIRECTION ( 'NONE',  ( -0.000000000000000000, -1.000000000000000000, -0.000000000000000000 ) ) ;
#7037=FACE_OUTER_BOUND ( 'NONE', #13198, .T. ) ;
#7044=EDGE_CURVE ( 'NONE', #9285, #27759, #54393, .T. ) ;
#7047=AXIS2_PLACEMENT_3D ( 'NONE', #88666, #49196, #19193 ) ;
#7053=CARTESIAN_POINT ( 'NONE',  ( -14.66148682522524993, 0.2301506158824424275, 2.874551585517085783 ) ) ;
#7055=EDGE_CURVE ( 'NONE', #96379, #91469, #53345, .T. ) ;
#7057=CARTESIAN_POINT ( 'NONE',  ( 9.065164099344466209, 14.63595249122789177, 11.95084933600773880 ) ) ;
#7058=CARTESIAN_POINT ( 'NONE',  ( -8.527530157486173934, 11.42559781766745708, 4.923371831947302546 ) ) ;
#7059=EDGE_LOOP ( 'NONE', ( #67714, #6646, #43305, #98960, #52308, #26480 ) ) ;
#7061=DIRECTION ( 'NONE',  ( 0.9999619230641713097, -0.000000000000000000, 0.008726535498374266009 ) ) ;
#7062=ORIENTED_EDGE ( 'NONE', *, *, #18281, .T. ) ;
#7072=ORIENTED_EDGE ( 'NONE', *, *, #21856, .F. ) ;
#7077=ORIENTED_EDGE ( 'NONE', *, *, #6577, .F. ) ;
#7083=ADVANCED_FACE ( 'NONE', ( #29852 ), #45445, .T. ) ;
#7086=EDGE_LOOP ( 'NONE', ( #64096, #44288, #39872, #83251 ) ) ;
#7088=ORIENTED_EDGE ( 'NONE', *, *, #50943, .T. ) ;
#7092=CARTESIAN_POINT ( 'NONE',  ( -1.114591949024815731, 15.00000000000000000, -14.45709807627963350 ) ) ;
#7095=DIRECTION ( 'NONE',  ( 0.000000000000000000, 1.000000000000000000, 0.000000000000000000 ) ) ;
#7097=VERTEX_POINT ( 'NONE', #84360 ) ;
#7098=CARTESIAN_POINT ( 'NONE',  ( -5.963430220938278126, 5.521642702460839658, 10.32896413005680358 ) ) ;
#7100=CARTESIAN_POINT ( 'NONE',  ( -13.30156849913890937, 14.76930270348882068, 6.804875469487965844 ) ) ;
#7108=VECTOR ( 'NONE', #50983, 1000.000000000000000 ) ;
#7119=CARTESIAN_POINT ( 'NONE',  ( -2.915334737309934532, -12.97798132251181968, -10.88017736071109987 ) ) ;
#7123=DIRECTION ( 'NONE',  ( -0.8433914458128813907, 0.000000000000000000, -0.5372996083468306594 ) ) ;
#7131=EDGE_CURVE ( 'NONE', #34423, #47878, #9327, .T. ) ;
#7135=DIRECTION ( 'NONE',  ( 0.1993679344172039347, 0.000000000000000000, -0.9799247046208282574 ) ) ;
#7137=EDGE_LOOP ( 'NONE', ( #50573, #56976, #12048, #88462 ) ) ;
#7139=DIRECTION ( 'NONE',  ( -0.000000000000000000, -1.000000000000000000, -0.000000000000000000 ) ) ;
#7149=CARTESIAN_POINT ( 'NONE',  ( -11.96291822454869802, 4.725512573308054359E-16, -8.193813980849247613 ) ) ;
#7168=CARTESIAN_POINT ( 'NONE',  ( 7.208316651077762316, -25.86606884899920900, -7.208316651077764980 ) ) ;
#7169=VERTEX_POINT ( 'NONE', #10809 ) ;
#7170=CARTESIAN_POINT ( 'NONE',  ( 13.55101055326450599, 0.2301500585724599590, 6.292244619294732999 ) ) ;
#7174=EDGE_LOOP ( 'NONE', ( #45175, #67917, #83781, #48638 ) ) ;
#7182=AXIS2_PLACEMENT_3D ( 'NONE', #66341, #97867, #5857 ) ;
#7183=VECTOR ( 'NONE', #3225, 1000.000000000000000 ) ;
#7184=CARTESIAN_POINT ( 'NONE',  ( 11.09922568453595026, 21.20696800326375708, 6.408140936763232709 ) ) ;
#7189=ORIENTED_EDGE ( 'NONE', *, *, #53785, .T. ) ;
#7195=CARTESIAN_POINT ( 'NONE',  ( -2.393480905992944496, 0.5000000000000004441, -14.80781041047754520 ) ) ;
#7198=CARTESIAN_POINT ( 'NONE',  ( -11.81378540890942119, 15.00000000000000000, 7.968498874458034287 ) ) ;
#7210=ORIENTED_EDGE ( 'NONE', *, *, #29282, .F. ) ;
#7216=FACE_OUTER_BOUND ( 'NONE', #89771, .T. ) ;
#7225=FACE_OUTER_BOUND ( 'NONE', #70406, .T. ) ;
#7228=DIRECTION ( 'NONE',  ( 0.000000000000000000, 1.000000000000000000, 0.000000000000000000 ) ) ;
#7234=CARTESIAN_POINT ( 'NONE',  ( 11.92686044187657224, 4.953790035174480799, 3.195792623639526209 ) ) ;
#7236=DIRECTION ( 'NONE',  ( 0.7826081568524149157, 0.000000000000000000, 0.6225146366376184126 ) ) ;
#7240=DIRECTION ( 'NONE',  ( 0.9935718556765885667, 0.000000000000000000, -0.1132032137678971873 ) ) ;
#7241=CARTESIAN_POINT ( 'NONE',  ( 10.36894250292378850, 24.92874883491397497, -10.36894250292379027 ) ) ;
#7250=EDGE_CURVE ( 'NONE', #5928, #59170, #21264, .T. ) ;
#7251=VERTEX_POINT ( 'NONE', #27268 ) ;
#7258=CARTESIAN_POINT ( 'NONE',  ( -9.402796353261203777, 15.00000000000000000, 11.68706210897750708 ) ) ;
#7262=B_SPLINE_CURVE_WITH_KNOTS ( 'NONE', 3,
 ( #14108, #67102, #98624, #60077, #88605, #52585 ),
 .UNSPECIFIED., .F., .F.,
 ( 4, 2, 4 ),
 ( 3.409110551494646011E-05, 0.0004400426677367926974, 0.0008459942299586389143 ),
 .UNSPECIFIED. ) ;
#7299=ORIENTED_EDGE ( 'NONE', *, *, #86151, .F. ) ;
#7311=ORIENTED_EDGE ( 'NONE', *, *, #27705, .T. ) ;
#7312=VERTEX_POINT ( 'NONE', #88271 ) ;
#7316=DIRECTION ( 'NONE',  ( 0.000000000000000000, 1.000000000000000000, 0.000000000000000000 ) ) ;
#7320=VECTOR ( 'NONE', #52176, 1000.000000000000000 ) ;
#7321=VERTEX_POINT ( 'NONE', #42781 ) ;
#7322=AXIS2_PLACEMENT_3D ( 'NONE', #33384, #95891, #80873 ) ;
#7324=CARTESIAN_POINT ( 'NONE',  ( 0.000000000000000000, 0.5000000000000004441, 0.000000000000000000 ) ) ;
#7327=B_SPLINE_CURVE_WITH_KNOTS ( 'NONE', 3,
 ( #56363, #11340, #42340, #64814, #55869, #3357 ),
 .UNSPECIFIED., .F., .F.,
 ( 4, 2, 4 ),
 ( 0.0002800056097769385239, 0.0006862108940652357231, 0.001092416178353533031 ),
 .UNSPECIFIED. ) ;
#7335=DIRECTION ( 'NONE',  ( 0.000000000000000000, 1.000000000000000000, 0.000000000000000000 ) ) ;
#7343=ADVANCED_FACE ( 'NONE', ( #36262 ), #72619, .T. ) ;
#7347=VERTEX_POINT ( 'NONE', #28261 ) ;
#7356=CARTESIAN_POINT ( 'NONE',  ( -11.81378540890942119, -0.03417435944610275333, 7.968498874458034287 ) ) ;
#7364=CARTESIAN_POINT ( 'NONE',  ( -14.48718990079891888, 4.171500096121077077E-16, -0.6093675230842403590 ) ) ;
#7365=AXIS2_PLACEMENT_3D ( 'NONE', #10225, #2740, #79197 ) ;
#7366=ORIENTED_EDGE ( 'NONE', *, *, #85870, .T. ) ;
#7367=LINE ( 'NONE', #8338, #96015 ) ;
#7369=DIRECTION ( 'NONE',  ( -0.000000000000000000, -1.000000000000000000, -0.000000000000000000 ) ) ;
#7373=EDGE_CURVE ( 'NONE', #8435, #4994, #26315, .T. ) ;
#7375=VERTEX_POINT ( 'NONE', #74241 ) ;
#7379=DIRECTION ( 'NONE',  ( 0.000000000000000000, 1.000000000000000000, 0.000000000000000000 ) ) ;
#7382=EDGE_CURVE ( 'NONE', #52640, #98966, #82197, .T. ) ;
#7385=ORIENTED_EDGE ( 'NONE', *, *, #16385, .F. ) ;
#7393=CARTESIAN_POINT ( 'NONE',  ( -14.74963345907814016, 14.95077488074853456, -0.3072669459662672464 ) ) ;
#7398=CARTESIAN_POINT ( 'NONE',  ( 14.88232117145531319, 14.63595249122790598, -1.875237731503143879 ) ) ;
#7399=CARTESIAN_POINT ( 'NONE',  ( -5.963430220938278126, 3.495456701841148650, 10.32896413005680358 ) ) ;
#7401=VECTOR ( 'NONE', #33935, 1000.000000000000000 ) ;
#7403=TOROIDAL_SURFACE ( 'NONE', #85612, 14.49999999999999822, 0.5000000000000000000 ) ;
#7416=CARTESIAN_POINT ( 'NONE',  ( 11.22915323889580463, 0.000000000000000000, -8.773176023390609757 ) ) ;
#7424=AXIS2_PLACEMENT_3D ( 'NONE', #17687, #34129, #79652 ) ;
#7430=LINE ( 'NONE', #38410, #70046 ) ;
#7436=CARTESIAN_POINT ( 'NONE',  ( -14.99847009497948669, 14.63606908182952715, 0.2142307401079193430 ) ) ;
#7439=CARTESIAN_POINT ( 'NONE',  ( 12.81628187352647608, -23.58469866340291432, 3.434112377981052511 ) ) ;
#7455=VERTEX_POINT ( 'NONE', #4297 ) ;
#7459=AXIS2_PLACEMENT_3D ( 'NONE', #53332, #37864, #37370 ) ;
#7462=FACE_OUTER_BOUND ( 'NONE', #47362, .T. ) ;
#7464=ADVANCED_FACE ( 'NONE', ( #34771 ), #31159, .T. ) ;
#7466=CARTESIAN_POINT ( 'NONE',  ( -5.795997163830251431, -0.03417435944610275333, 13.01802277140702024 ) ) ;
#7468=AXIS2_PLACEMENT_3D ( 'NONE', #71794, #19282, #65254 ) ;
#7471=DIRECTION ( 'NONE',  ( -0.09584575252021386438, 0.000000000000000000, -0.9953961983671798519 ) ) ;
#7493=VECTOR ( 'NONE', #31432, 1000.000000000000000 ) ;
#7495=CARTESIAN_POINT ( 'NONE',  ( -14.16423886937410437, -18.40458449841936073, -3.795296366450299885 ) ) ;
#7508=CYLINDRICAL_SURFACE ( 'NONE', #84814, 15.00000000000000000 ) ;
#7510=CARTESIAN_POINT ( 'NONE',  ( -6.715867195167276371, 4.396228481599465503E-16, -12.85095824508335838 ) ) ;
#7513=CARTESIAN_POINT ( 'NONE',  ( 10.88017736071110519, 30.56368534415485172, -2.602085213965210642E-15 ) ) ;
#7519=ORIENTED_EDGE ( 'NONE', *, *, #30483, .F. ) ;
#7522=DIRECTION ( 'NONE',  ( 0.4146932426562462415, 0.000000000000000000, -0.9099612708765399960 ) ) ;
#7531=EDGE_LOOP ( 'NONE', ( #29161, #50480, #72220, #63227, #60300, #25160 ) ) ;
#7545=DIRECTION ( 'NONE',  ( -0.000000000000000000, -1.000000000000000000, -0.000000000000000000 ) ) ;
#7546=EDGE_CURVE ( 'NONE', #47538, #32615, #74267, .T. ) ;
#7555=CARTESIAN_POINT ( 'NONE',  ( -4.181050312904877941, 15.00000000000000888, -14.01631781289607659 ) ) ;
#7556=CARTESIAN_POINT ( 'NONE',  ( 2.361410439757328117, 0.2306972965111871443, -14.75336556272936228 ) ) ;
#7566=CARTESIAN_POINT ( 'NONE',  ( -3.469446951953614189E-15, 19.75893115100078745, -9.846743663894594434 ) ) ;
#7576=AXIS2_PLACEMENT_3D ( 'NONE', #15215, #81830, #51345 ) ;
#7577=CIRCLE ( 'NONE', #79348, 14.49999999999999822 ) ;
#7579=ORIENTED_EDGE ( 'NONE', *, *, #88779, .F. ) ;
#7584=ORIENTED_EDGE ( 'NONE', *, *, #9982, .T. ) ;
#7596=ORIENTED_EDGE ( 'NONE', *, *, #97466, .T. ) ;
#7598=DIRECTION ( 'NONE',  ( -0.000000000000000000, -1.000000000000000000, -0.000000000000000000 ) ) ;
#7603=ORIENTED_EDGE ( 'NONE', *, *, #44754, .T. ) ;
#7604=DIRECTION ( 'NONE',  ( 0.000000000000000000, 0.000000000000000000, 1.000000000000000000 ) ) ;
#7614=CIRCLE ( 'NONE', #63474, 15.00000000000000000 ) ;
#7618=ORIENTED_EDGE ( 'NONE', *, *, #70921, .F. ) ;
#7626=EDGE_CURVE ( 'NONE', #46052, #62525, #95039, .T. ) ;
#7627=CARTESIAN_POINT ( 'NONE',  ( -14.09397099617986093, 0.04962897248923128779, -4.360881834954357217 ) ) ;
#7631=CARTESIAN_POINT ( 'NONE',  ( -9.422509992056136596, -16.51964798917849109, 5.440088680355559703 ) ) ;
#7635=CARTESIAN_POINT ( 'NONE',  ( -4.096035146093626622, 4.358906096699807873E-16, 13.90943910019256258 ) ) ;
#7646=CARTESIAN_POINT ( 'NONE',  ( -13.34343830728408697, 0.5000000000000004441, 6.852200678592504701 ) ) ;
#7648=VERTEX_POINT ( 'NONE', #30225 ) ;
#7658=EDGE_CURVE ( 'NONE', #22307, #3873, #96637, .T. ) ;
#7661=ORIENTED_EDGE ( 'NONE', *, *, #98035, .F. ) ;
#7662=ORIENTED_EDGE ( 'NONE', *, *, #55770, .T. ) ;
#7675=CARTESIAN_POINT ( 'NONE',  ( -4.923371831947292776, -28.15773551566587685, 8.527530157486181039 ) ) ;
#7677=CARTESIAN_POINT ( 'NONE',  ( 1.514341385896460501, -0.03417435944610275333, 15.92432625271834112 ) ) ;
#7678=ORIENTED_EDGE ( 'NONE', *, *, #13044, .T. ) ;
#7679=VERTEX_POINT ( 'NONE', #84247 ) ;
#7680=DIRECTION ( 'NONE',  ( 0.9636304532086191754, 0.000000000000000000, 0.2672383760782702788 ) ) ;
#7687=CARTESIAN_POINT ( 'NONE',  ( -9.382169495545422677, 18.49863466993041428, -9.382169495545417348 ) ) ;
#7694=CIRCLE ( 'NONE', #63545, 14.49999999999999822 ) ;
#7698=CARTESIAN_POINT ( 'NONE',  ( 12.98685442714194949, 4.417933709739653524E-16, 6.449155920601044478 ) ) ;
#7701=AXIS2_PLACEMENT_3D ( 'NONE', #90716, #52718, #30206 ) ;
#7705=CARTESIAN_POINT ( 'NONE',  ( -14.82269085861169344, 0.3639308522293647763, -2.299529454047150701 ) ) ;
#7711=CARTESIAN_POINT ( 'NONE',  ( 6.715867195167361636, 15.00000000000000000, 12.85095824508331930 ) ) ;
#7714=CARTESIAN_POINT ( 'NONE',  ( 11.10175276307590586, 0.04962894967561130161, 9.716398248524756198 ) ) ;
#7715=ORIENTED_EDGE ( 'NONE', *, *, #83458, .T. ) ;
#7716=CARTESIAN_POINT ( 'NONE',  ( 6.715867195167446901, 15.00000000000000000, -12.85095824508324469 ) ) ;
#7726=PLANE ( 'NONE',  #1262 ) ;
#7727=EDGE_CURVE ( 'NONE', #89266, #28441, #6754, .T. ) ;
#7734=DIRECTION ( 'NONE',  ( 0.000000000000000000, 0.000000000000000000, -1.000000000000000000 ) ) ;
#7743=CARTESIAN_POINT ( 'NONE',  ( 7.082119434687047743, 25.13708216824731068, -12.26659068614894821 ) ) ;
#7746=CARTESIAN_POINT ( 'NONE',  ( 3.420591144908569081, 14.63606885998601825, -14.60477854057959490 ) ) ;
#7752=VERTEX_POINT ( 'NONE', #85711 ) ;
#7758=DIRECTION ( 'NONE',  ( 0.000000000000000000, 0.000000000000000000, -1.000000000000000000 ) ) ;
#7764=DIRECTION ( 'NONE',  ( 0.000000000000000000, 0.000000000000000000, 1.000000000000000000 ) ) ;
#7767=DIRECTION ( 'NONE',  ( -0.000000000000000000, -1.000000000000000000, -0.000000000000000000 ) ) ;
#7776=VERTEX_POINT ( 'NONE', #55194 ) ;
#7784=LINE ( 'NONE', #22293, #83731 ) ;
#7802=ORIENTED_EDGE ( 'NONE', *, *, #67208, .T. ) ;
#7804=CARTESIAN_POINT ( 'NONE',  ( -5.803070148808147088, 3.900978891399319278E-16, -13.28812917035395813 ) ) ;
#7806=ORIENTED_EDGE ( 'NONE', *, *, #30838, .F. ) ;
#7816=ADVANCED_FACE ( 'NONE', ( #71688 ), #92707, .F. ) ;
#7820=DIRECTION ( 'NONE',  ( 0.000000000000000000, 0.000000000000000000, 1.000000000000000000 ) ) ;
#7823=EDGE_CURVE ( 'NONE', #88606, #11086, #5631, .T. ) ;
#7825=DIRECTION ( 'NONE',  ( -0.000000000000000000, -1.000000000000000000, -0.000000000000000000 ) ) ;
#7832=DIRECTION ( 'NONE',  ( 0.000000000000000000, 1.000000000000000000, 0.000000000000000000 ) ) ;
#7835=CARTESIAN_POINT ( 'NONE',  ( 0.000000000000000000, 0.5000000000000004441, 0.000000000000000000 ) ) ;
#7841=CARTESIAN_POINT ( 'NONE',  ( -0.7375392941516176748, 0.5000000000000004441, -14.98185688723471820 ) ) ;
#7845=DIRECTION ( 'NONE',  ( 0.000000000000000000, 0.000000000000000000, 1.000000000000000000 ) ) ;
#7856=CIRCLE ( 'NONE', #25421, 15.00000000000000000 ) ;
#7867=CARTESIAN_POINT ( 'NONE',  ( -13.34343830728398927, 14.49999999999999112, -6.852200678592835104 ) ) ;
#7881=LINE ( 'NONE', #75872, #90972 ) ;
#7883=CARTESIAN_POINT ( 'NONE',  ( 14.73551000134585820, 0.04962893459885754643, -0.7225335126797688412 ) ) ;
#7885=DIRECTION ( 'NONE',  ( 0.2334453638559024768, 0.000000000000000000, 0.9723699203976772232 ) ) ;
#7888=CARTESIAN_POINT ( 'NONE',  ( -3.195792623639463592, 3.703790035174482131, 11.92686044187660421 ) ) ;
#7898=CARTESIAN_POINT ( 'NONE',  ( 5.806645064956531321, 15.00000000000000888, -13.42464971016994113 ) ) ;
#7913=DIRECTION ( 'NONE',  ( -0.9588197348681908316, 0.000000000000000000, -0.2840153447039300283 ) ) ;
#7917=CARTESIAN_POINT ( 'NONE',  ( -13.95697193428315330, 15.00000000000000711, 4.371663894958725649 ) ) ;
#7924=CARTESIAN_POINT ( 'NONE',  ( -12.81628187352647252, -10.66803199673624825, 3.434112377981066722 ) ) ;
#7936=EDGE_LOOP ( 'NONE', ( #14023, #18032, #5066, #7210 ) ) ;
#7939=EDGE_CURVE ( 'NONE', #72059, #69558, #78698, .T. ) ;
#7947=CARTESIAN_POINT ( 'NONE',  ( -12.60589901313210071, 0.5000000000000004441, -8.129656208642224158 ) ) ;
#7948=VECTOR ( 'NONE', #17828, 1000.000000000000114 ) ;
#7952=DIRECTION ( 'NONE',  ( 0.000000000000000000, 1.000000000000000000, 0.000000000000000000 ) ) ;
#7956=CARTESIAN_POINT ( 'NONE',  ( 11.59608414876348448, 14.76930270348882068, -9.421724210956282874 ) ) ;
#7973=LINE ( 'NONE', #84942, #97806 ) ;
#7975=CARTESIAN_POINT ( 'NONE',  ( 12.00809552683965364, 14.49999999999999112, -8.989195838243565717 ) ) ;
#7978=CARTESIAN_POINT ( 'NONE',  ( 14.16423886937410082, -0.4879178317526934872, -3.795296366450314096 ) ) ;
#7985=DIRECTION ( 'NONE',  ( -0.000000000000000000, 1.000000000000000000, -0.000000000000000000 ) ) ;
#7988=DIRECTION ( 'NONE',  ( -0.000000000000000000, 1.000000000000000000, -0.000000000000000000 ) ) ;
#7990=CARTESIAN_POINT ( 'NONE',  ( -6.767445849361066301, 0.3640475087720979608, -13.38662304974506512 ) ) ;
#8001=AXIS2_PLACEMENT_3D ( 'NONE', #60383, #70739, #2255 ) ;
#8004=CARTESIAN_POINT ( 'NONE',  ( 0.1034006766821532752, 4.444999227851523509E-16, 14.49963131600461175 ) ) ;
#8009=DIRECTION ( 'NONE',  ( -0.8433914458128884961, 0.000000000000000000, 0.5372996083468194461 ) ) ;
#8012=ORIENTED_EDGE ( 'NONE', *, *, #56486, .T. ) ;
#8014=CARTESIAN_POINT ( 'NONE',  ( 0.000000000000000000, 15.00000000000000000, 0.000000000000000000 ) ) ;
#8025=EDGE_CURVE ( 'NONE', #73183, #71843, #14594, .T. ) ;
#8027=DIRECTION ( 'NONE',  ( 0.000000000000000000, 1.000000000000000000, 0.000000000000000000 ) ) ;
#8042=CARTESIAN_POINT ( 'NONE',  ( -5.204170427930421283E-15, -42.12636533006957507, -12.81628187352647608 ) ) ;
#8044=B_SPLINE_CURVE_WITH_KNOTS ( 'NONE', 3,
 ( #73704, #43707, #65213, #81217, #65711, #12222 ),
 .UNSPECIFIED., .F., .F.,
 ( 4, 2, 4 ),
 ( 3.409110551417103194E-05, 0.0004400426677359989529, 0.0008459942299578269553 ),
 .UNSPECIFIED. ) ;
#8045=CARTESIAN_POINT ( 'NONE',  ( 0.000000000000000000, 15.00000000000000000, 0.000000000000000000 ) ) ;
#8046=ORIENTED_EDGE ( 'NONE', *, *, #43468, .T. ) ;
#8064=AXIS2_PLACEMENT_3D ( 'NONE', #73280, #91113, #12288 ) ;
#8073=ORIENTED_EDGE ( 'NONE', *, *, #2694, .F. ) ;
#8089=EDGE_CURVE ( 'NONE', #5244, #52640, #47126, .T. ) ;
#8093=AXIS2_PLACEMENT_3D ( 'NONE', #35104, #43601, #58604 ) ;
#8096=ORIENTED_EDGE ( 'NONE', *, *, #54951, .F. ) ;
#8104=CARTESIAN_POINT ( 'NONE',  ( 7.313705784284628031, 14.63606873438734901, -13.09617149020746751 ) ) ;
#8108=CARTESIAN_POINT ( 'NONE',  ( -5.440088680355558814, -7.769647989178493752, -9.422509992056136596 ) ) ;
#8110=CARTESIAN_POINT ( 'NONE',  ( 13.78891971893208357, 0.5000000000000004441, -5.904717858191528279 ) ) ;
#8112=DIRECTION ( 'NONE',  ( -0.000000000000000000, -1.000000000000000000, -0.000000000000000000 ) ) ;
#8113=FACE_OUTER_BOUND ( 'NONE', #54263, .T. ) ;
#8119=CARTESIAN_POINT ( 'NONE',  ( -7.002992508388866888, -2.668153783851045279E-15, -12.84003923133027492 ) ) ;
#8122=CARTESIAN_POINT ( 'NONE',  ( 9.876730923139225737, 0.5000000000000004441, 11.28938378619069560 ) ) ;
#8135=DIRECTION ( 'NONE',  ( 0.000000000000000000, 1.000000000000000000, 0.000000000000000000 ) ) ;
#8137=ADVANCED_FACE ( 'NONE', ( #10513 ), #13613, .T. ) ;
#8139=CARTESIAN_POINT ( 'NONE',  ( 3.469446951953614189E-15, 5.938309369127516391, 11.92686044187656513 ) ) ;
#8156=CARTESIAN_POINT ( 'NONE',  ( -9.846743663894594434, -18.99106884899921255, 3.469446951953614189E-15 ) ) ;
#8159=VERTEX_POINT ( 'NONE', #72481 ) ;
#8161=VERTEX_POINT ( 'NONE', #4015 ) ;
#8162=AXIS2_PLACEMENT_3D ( 'NONE', #83103, #73616, #88622 ) ;
#8163=DIRECTION ( 'NONE',  ( 0.000000000000000000, 1.000000000000000000, 0.000000000000000000 ) ) ;
#8168=DIRECTION ( 'NONE',  ( 0.9953961983671798519, 0.000000000000000000, -0.09584575252021386438 ) ) ;
#8172=CARTESIAN_POINT ( 'NONE',  ( -12.81628187352647252, 24.33196800326376064, 3.434112377981066722 ) ) ;
#8185=CARTESIAN_POINT ( 'NONE',  ( 1.180296924652914470, 0.000000000000000000, -5.323975374878053834 ) ) ;
#8186=AXIS2_PLACEMENT_3D ( 'NONE', #21844, #45823, #30301 ) ;
#8187=DIRECTION ( 'NONE',  ( 0.000000000000000000, 1.000000000000000000, 0.000000000000000000 ) ) ;
#8193=CARTESIAN_POINT ( 'NONE',  ( 6.761335002693003027, 14.76984993307862482, 13.32315948060042743 ) ) ;
#8198=ORIENTED_EDGE ( 'NONE', *, *, #14233, .F. ) ;
#8200=CARTESIAN_POINT ( 'NONE',  ( 0.000000000000000000, 15.00000000000000000, 0.000000000000000000 ) ) ;
#8204=DIRECTION ( 'NONE',  ( -0.000000000000000000, -1.000000000000000000, -0.000000000000000000 ) ) ;
#8210=EDGE_CURVE ( 'NONE', #67800, #37192, #74579, .T. ) ;
#8212=CARTESIAN_POINT ( 'NONE',  ( -0.1034006766821533585, 15.00000000000000000, -14.49963131600461175 ) ) ;
#8224=MANIFOLD_SOLID_BREP ( 'CirPattern1', #25068 ) ;
#8227=CARTESIAN_POINT ( 'NONE',  ( 10.36894250292379027, 23.67874883491397142, 10.36894250292378672 ) ) ;
#8237=ORIENTED_EDGE ( 'NONE', *, *, #9740, .F. ) ;
#8246=VERTEX_POINT ( 'NONE', #33491 ) ;
#8248=CARTESIAN_POINT ( 'NONE',  ( 14.56311970191028138, 14.76984991344722253, -3.337330457605880873 ) ) ;
#8255=EDGE_CURVE ( 'NONE', #60677, #94458, #49001, .T. ) ;
#8261=CARTESIAN_POINT ( 'NONE',  ( 6.767445849361160448, 14.49999999999999112, 13.38662304974508110 ) ) ;
#8276=ORIENTED_EDGE ( 'NONE', *, *, #58455, .T. ) ;
#8277=DIRECTION ( 'NONE',  ( -0.6360782202777751637, -0.000000000000000000, 0.7716245833877106719 ) ) ;
#8282=ORIENTED_EDGE ( 'NONE', *, *, #19548, .T. ) ;
#8296=DIRECTION ( 'NONE',  ( 0.000000000000000000, 0.000000000000000000, 1.000000000000000000 ) ) ;
#8301=EDGE_LOOP ( 'NONE', ( #15157, #94152, #5535, #44717, #58647, #34551 ) ) ;
#8318=CARTESIAN_POINT ( 'NONE',  ( -10.84451454131299997, 15.00000000000000000, 9.625305416633544553 ) ) ;
#8334=CARTESIAN_POINT ( 'NONE',  ( 9.876730923139286134, 14.49999999999999112, 11.28938378619072935 ) ) ;
#8338=CARTESIAN_POINT ( 'NONE',  ( -10.19513985507817821, 15.00000000000000000, -11.00268709613231088 ) ) ;
#8347=DIRECTION ( 'NONE',  ( 0.000000000000000000, 0.000000000000000000, 1.000000000000000000 ) ) ;
#8368=DIRECTION ( 'NONE',  ( 0.000000000000000000, 0.000000000000000000, 1.000000000000000000 ) ) ;
#8372=EDGE_CURVE ( 'NONE', #43197, #7097, #74450, .T. ) ;
#8386=ORIENTED_EDGE ( 'NONE', *, *, #78748, .T. ) ;
#8396=CARTESIAN_POINT ( 'NONE',  ( -14.04391541078760675, 15.00000000000000000, -3.608107528143027043 ) ) ;
#8400=CARTESIAN_POINT ( 'NONE',  ( 0.000000000000000000, 14.49999999999999822, 0.000000000000000000 ) ) ;
#8401=AXIS2_PLACEMENT_3D ( 'NONE', #87395, #9933, #41433 ) ;
#8404=ADVANCED_FACE ( 'NONE', ( #36470 ), #65968, .F. ) ;
#8411=CARTESIAN_POINT ( 'NONE',  ( -12.34086200392831678, 15.00000000000000000, 7.124999999999885425 ) ) ;
#8422=ORIENTED_EDGE ( 'NONE', *, *, #311, .F. ) ;
#8423=AXIS2_PLACEMENT_3D ( 'NONE', #66964, #49986, #12480 ) ;
#8432=CARTESIAN_POINT ( 'NONE',  ( -14.48718990079891888, 15.00000000000000000, -0.6093675230842395818 ) ) ;
#8435=VERTEX_POINT ( 'NONE', #42983 ) ;
#8437=CARTESIAN_POINT ( 'NONE',  ( 3.014428414850129911, 3.659700295649314761, -11.25000000000000000 ) ) ;
#8447=CARTESIAN_POINT ( 'NONE',  ( -3.014428414850141458, 9.076366962315983500, -11.25000000000000000 ) ) ;
#8452=DIRECTION ( 'NONE',  ( -0.3826834323650877834, 0.000000000000000000, -0.9238795325112876267 ) ) ;
#8454=ADVANCED_FACE ( 'NONE', ( #72977 ), #5225, .T. ) ;
#8458=CARTESIAN_POINT ( 'NONE',  ( -3.795296366450300773, -12.15458449841936250, 14.16423886937410437 ) ) ;
#8474=LINE ( 'NONE', #38980, #65951 ) ;
#8477=LINE ( 'NONE', #32935, #27224 ) ;
#8485=EDGE_CURVE ( 'NONE', #50974, #88806, #26987, .T. ) ;
#8496=CARTESIAN_POINT ( 'NONE',  ( 0.000000000000000000, 15.00000000000000000, 0.000000000000000000 ) ) ;
#8497=( BOUNDED_CURVE ( )  B_SPLINE_CURVE ( 2, ( #81723, #27739, #36740, #29220, #89238, #50239, #43731, #57743, #88246, #88742, #59220, #73732, #66228 ),
 .UNSPECIFIED., .F., .T. ) 
 B_SPLINE_CURVE_WITH_KNOTS ( ( 3, 2, 2, 2, 2, 2, 3 ),
 ( 0.5999999999999999778, 0.6055555555555555136, 0.6111111111111111605, 0.6166666666666666963, 0.6222222222222222321, 0.6277777777777777679, 0.6333333333333333037 ),
 .UNSPECIFIED. ) 
 CURVE ( )  GEOMETRIC_REPRESENTATION_ITEM ( )  RATIONAL_B_SPLINE_CURVE ( ( 1.000000000000000000, 0.9659258262890684232, 1.000000000000000000, 0.9659258262890684232, 1.000000000000000000, 0.9659258262890684232, 1.000000000000000000, 0.9659258262890684232, 1.000000000000000000, 0.9659258262890684232, 1.000000000000000000, 0.9659258262890684232, 1.000000000000000000 ) ) 
 REPRESENTATION_ITEM ( '' )  );
#8499=ORIENTED_EDGE ( 'NONE', *, *, #48768, .F. ) ;
#8506=DIRECTION ( 'NONE',  ( 0.000000000000000000, 0.000000000000000000, -1.000000000000000000 ) ) ;
#8512=LINE ( 'NONE', #39015, #96684 ) ;
#8521=CARTESIAN_POINT ( 'NONE',  ( -10.17198128013151326, 14.76930270348881002, 10.94389562857658760 ) ) ;
#8526=EDGE_CURVE ( 'NONE', #20839, #98896, #12969, .T. ) ;
#8530=EDGE_CURVE ( 'NONE', #54264, #43197, #50476, .T. ) ;
#8532=CARTESIAN_POINT ( 'NONE',  ( -7.208316651077764980, 30.38393115100079456, -7.208316651077759651 ) ) ;
#8535=ORIENTED_EDGE ( 'NONE', *, *, #73858, .F. ) ;
#8543=VECTOR ( 'NONE', #93323, 1000.000000000000227 ) ;
#8546=TOROIDAL_SURFACE ( 'NONE', #78767, 14.49999999999999822, 0.5000000000000000000 ) ;
#8557=CARTESIAN_POINT ( 'NONE',  ( -10.04796213703165186, 9.757819552369537934E-16, -10.62905469192480723 ) ) ;
#8560=VERTEX_POINT ( 'NONE', #82453 ) ;
#8567=CARTESIAN_POINT ( 'NONE',  ( -7.595945211628415628, 4.258289072137175049E-16, 12.35117874301636398 ) ) ;
#8568=LINE ( 'NONE', #78044, #67357 ) ;
#8571=ORIENTED_EDGE ( 'NONE', *, *, #2248, .F. ) ;
#8593=CARTESIAN_POINT ( 'NONE',  ( 3.469446951953614189E-15, -0.6863146558451562740, 10.88017736071110342 ) ) ;
#8598=CARTESIAN_POINT ( 'NONE',  ( -9.898881779040801021, -0.03417435944610275333, 10.25059215482569641 ) ) ;
#8608=CARTESIAN_POINT ( 'NONE',  ( -10.64017930668213374, 0.3640475087720987379, 10.57291749337208842 ) ) ;
#8610=ORIENTED_EDGE ( 'NONE', *, *, #45037, .F. ) ;
#8612=AXIS2_PLACEMENT_3D ( 'NONE', #58116, #5141, #20132 ) ;
#8620=CARTESIAN_POINT ( 'NONE',  ( 0.9082943533636183009, 15.00000000000000000, 14.47152380945585648 ) ) ;
#8622=DIRECTION ( 'NONE',  ( 0.07845909572783234254, 0.000000000000000000, 0.9969173337331289630 ) ) ;
#8636=CARTESIAN_POINT ( 'NONE',  ( 12.60589901313222327, 0.3640475087720989600, -8.129656208642053627 ) ) ;
#8638=CARTESIAN_POINT ( 'NONE',  ( 9.846743663894590881, -11.28273551566587685, -2.638427012816833894 ) ) ;
#8639=ORIENTED_EDGE ( 'NONE', *, *, #15606, .T. ) ;
#8643=ORIENTED_EDGE ( 'NONE', *, *, #4333, .T. ) ;
#8664=DIRECTION ( 'NONE',  ( 0.000000000000000000, -1.000000000000000000, 0.000000000000000000 ) ) ;
#8665=ORIENTED_EDGE ( 'NONE', *, *, #57584, .T. ) ;
#8667=AXIS2_PLACEMENT_3D ( 'NONE', #62403, #44947, #75452 ) ;
#8676=DIRECTION ( 'NONE',  ( 0.02617694830788287394, 0.000000000000000000, -0.9996573249755570378 ) ) ;
#8687=EDGE_CURVE ( 'NONE', #26584, #48509, #53933, .T. ) ;
#8689=CARTESIAN_POINT ( 'NONE',  ( -8.731067818237029599, 8.287123368507817389, 8.731067818237043809 ) ) ;
#8691=ORIENTED_EDGE ( 'NONE', *, *, #78213, .T. ) ;
#8692=FACE_OUTER_BOUND ( 'NONE', #73450, .T. ) ;
#8696=CARTESIAN_POINT ( 'NONE',  ( -14.97687855664608847, 15.00000000000000000, 0.8325315005899532883 ) ) ;
#8698=CARTESIAN_POINT ( 'NONE',  ( 13.78891971893209245, 14.49999999999999112, 5.904717858191670388 ) ) ;
#8703=CARTESIAN_POINT ( 'NONE',  ( -9.422509992056145478, -37.35298132251182324, -5.440088680355541939 ) ) ;
#8718=DIRECTION ( 'NONE',  ( 0.000000000000000000, 1.000000000000000000, 0.000000000000000000 ) ) ;
#8723=ORIENTED_EDGE ( 'NONE', *, *, #39252, .F. ) ;
#8732=CARTESIAN_POINT ( 'NONE',  ( -7.674241358950697922, 14.76984990496856831, -12.81905807005896136 ) ) ;
#8737=ORIENTED_EDGE ( 'NONE', *, *, #29591, .F. ) ;
#8745=DIRECTION ( 'NONE',  ( -0.8788171126619678253, 0.000000000000000000, 0.4771587602596037425 ) ) ;
#8746=B_SPLINE_CURVE_WITH_KNOTS ( 'NONE', 3,
 ( #93816, #16848, #78318, #33301, #26298, #86817 ),
 .UNSPECIFIED., .F., .F.,
 ( 4, 2, 4 ),
 ( 3.409110551494476605E-05, 0.0004400426677367900953, 0.0008459942299586354448 ),
 .UNSPECIFIED. ) ;
#8751=DIRECTION ( 'NONE',  ( 0.000000000000000000, 0.000000000000000000, 1.000000000000000000 ) ) ;
#8759=CIRCLE ( 'NONE', #85405, 15.00000000000000000 ) ;
#8760=EDGE_LOOP ( 'NONE', ( #62169, #18141, #85288, #16881 ) ) ;
#8762=VERTEX_POINT ( 'NONE', #21974 ) ;
#8766=EDGE_CURVE ( 'NONE', #50677, #65059, #97465, .T. ) ;
#8768=ORIENTED_EDGE ( 'NONE', *, *, #76445, .F. ) ;
#8770=CARTESIAN_POINT ( 'NONE',  ( 12.07856007377819907, 15.00000000000000000, 8.022367888854917695 ) ) ;
#8771=AXIS2_PLACEMENT_3D ( 'NONE', #36382, #74361, #96407 ) ;
#8772=ORIENTED_EDGE ( 'NONE', *, *, #81136, .T. ) ;
#8774=VERTEX_POINT ( 'NONE', #8432 ) ;
#8777=CARTESIAN_POINT ( 'NONE',  ( 0.000000000000000000, 15.00000000000000000, 0.000000000000000000 ) ) ;
#8783=CARTESIAN_POINT ( 'NONE',  ( 0.000000000000000000, 0.000000000000000000, 0.000000000000000000 ) ) ;
#8785=CARTESIAN_POINT ( 'NONE',  ( -1.354709868695722852, 0.5000000000000004441, 14.93870011653150698 ) ) ;
#8790=ORIENTED_EDGE ( 'NONE', *, *, #36598, .T. ) ;
#8797=AXIS2_PLACEMENT_3D ( 'NONE', #83805, #60794, #85282 ) ;
#8802=FACE_OUTER_BOUND ( 'NONE', #69291, .T. ) ;
#8810=FACE_OUTER_BOUND ( 'NONE', #6338, .T. ) ;
#8812=EDGE_CURVE ( 'NONE', #62525, #77069, #79564, .T. ) ;
#8813=VECTOR ( 'NONE', #47781, 1000.000000000000000 ) ;
#8823=CARTESIAN_POINT ( 'NONE',  ( -0.3093388210927633386, 14.63723947401114067, -14.99680997725065978 ) ) ;
#8824=CARTESIAN_POINT ( 'NONE',  ( -13.07907619356921636, 0.2301500790491314286, -7.222187741820853546 ) ) ;
#8830=EDGE_CURVE ( 'NONE', #67262, #10027, #31410, .T. ) ;
#8833=LINE ( 'NONE', #75858, #49853 ) ;
#8834=CARTESIAN_POINT ( 'NONE',  ( 13.14228782657341732, 14.49999999999999112, 7.230509711182337540 ) ) ;
#8841=VERTEX_POINT ( 'NONE', #36965 ) ;
#8848=CARTESIAN_POINT ( 'NONE',  ( 8.375939845167756914, 15.00000000000000000, -11.52849216984298941 ) ) ;
#8849=LINE ( 'NONE', #38871, #33638 ) ;
#8853=CARTESIAN_POINT ( 'NONE',  ( 5.419894505350611347, 14.63606864254977502, -13.98659156302462314 ) ) ;
#8856=AXIS2_PLACEMENT_3D ( 'NONE', #1346, #55296, #94274 ) ;
#8861=DIRECTION ( 'NONE',  ( 0.3007057995042701770, -0.000000000000000000, 0.9537169507482278208 ) ) ;
#8873=ADVANCED_FACE ( 'NONE', ( #23942, #67461 ), #97982, .T. ) ;
#8875=CIRCLE ( 'NONE', #48764, 14.49999999999999822 ) ;
#8880=CARTESIAN_POINT ( 'NONE',  ( -14.47650479471822393, 14.49999999999999112, -3.928206833722243108 ) ) ;
#8883=ORIENTED_EDGE ( 'NONE', *, *, #24810, .F. ) ;
#8885=VECTOR ( 'NONE', #1000, 1000.000000000000114 ) ;
#8899=DIRECTION ( 'NONE',  ( -0.000000000000000000, -1.000000000000000000, -0.000000000000000000 ) ) ;
#8900=ORIENTED_EDGE ( 'NONE', *, *, #86042, .T. ) ;
#8906=CARTESIAN_POINT ( 'NONE',  ( 3.115783986955464435, 4.832823856176936692E-16, 14.16128137375399731 ) ) ;
#8910=CARTESIAN_POINT ( 'NONE',  ( 10.64017930668211598, 14.49999999999999112, -10.57291749337218256 ) ) ;
#8914=TOROIDAL_SURFACE ( 'NONE', #98320, 14.49999999999999822, 0.5000000000000000000 ) ;
#8919=EDGE_CURVE ( 'NONE', #23491, #54920, #44942, .T. ) ;
#8921=EDGE_LOOP ( 'NONE', ( #20040, #85019, #6689, #74280 ) ) ;
#8924=ADVANCED_FACE ( 'NONE', ( #30429 ), #45098, .T. ) ;
#8928=CARTESIAN_POINT ( 'NONE',  ( -0.9940297508535884674, -0.03417435944610275333, -14.21528771620250886 ) ) ;
#8934=CARTESIAN_POINT ( 'NONE',  ( -3.881909499400240104, 15.00000000000000178, -14.10103859407600169 ) ) ;
#8940=CARTESIAN_POINT ( 'NONE',  ( 14.71525861348293063, 0.3639310978437776956, -2.908807992686601285 ) ) ;
#8943=CARTESIAN_POINT ( 'NONE',  ( -14.16423886937410082, -13.19625116508602680, 4.336808689942017736E-15 ) ) ;
#8953=LINE ( 'NONE', #75108, #32798 ) ;
#8962=DIRECTION ( 'NONE',  ( 0.000000000000000000, 1.000000000000000000, 0.000000000000000000 ) ) ;
#8970=ORIENTED_EDGE ( 'NONE', *, *, #78248, .F. ) ;
#8981=VERTEX_POINT ( 'NONE', #33857 ) ;
#8990=DIRECTION ( 'NONE',  ( 0.000000000000000000, 1.000000000000000000, 0.000000000000000000 ) ) ;
#8992=ORIENTED_EDGE ( 'NONE', *, *, #52734, .F. ) ;
#8993=VECTOR ( 'NONE', #41411, 1000.000000000000000 ) ;
#8996=EDGE_LOOP ( 'NONE', ( #98076, #95760, #52171, #44849, #12868, #43804 ) ) ;
#8997=ORIENTED_EDGE ( 'NONE', *, *, #63713, .F. ) ;
#9003=CARTESIAN_POINT ( 'NONE',  ( 0.000000000000000000, 15.00000000000000000, 0.000000000000000000 ) ) ;
#9011=CARTESIAN_POINT ( 'NONE',  ( 7.208316651077764980, 27.88393115100078745, 7.208316651077762316 ) ) ;
#9024=VERTEX_POINT ( 'NONE', #62901 ) ;
#9025=VECTOR ( 'NONE', #76551, 1000.000000000000114 ) ;
#9036=EDGE_CURVE ( 'NONE', #59690, #23318, #47308, .T. ) ;
#9039=CARTESIAN_POINT ( 'NONE',  ( -12.84737282370062061, 15.00000000000000000, -9.530079116402557560 ) ) ;
#9040=CIRCLE ( 'NONE', #36157, 15.00000000000000000 ) ;
#9046=TOROIDAL_SURFACE ( 'NONE', #77698, 14.49999999999999822, 0.5000000000000000000 ) ;
#9077=CARTESIAN_POINT ( 'NONE',  ( 14.62617646268087768, 0.5000000000000004441, -3.327906561566883692 ) ) ;
#9083=CARTESIAN_POINT ( 'NONE',  ( 5.440088680355556150, 4.730352010821510689, 9.422509992056138373 ) ) ;
#9088=CARTESIAN_POINT ( 'NONE',  ( 8.209432707284774366, 14.49999999999999822, 12.55409154915492032 ) ) ;
#9092=LINE ( 'NONE', #70096, #42535 ) ;
#9093=LINE ( 'NONE', #56563, #33146 ) ;
#9094=VECTOR ( 'NONE', #93648, 1000.000000000000000 ) ;
#9098=CARTESIAN_POINT ( 'NONE',  ( -10.27191093752570339, 9.232659125071871724E-16, 10.41278984915619432 ) ) ;
#9100=ORIENTED_EDGE ( 'NONE', *, *, #47309, .T. ) ;
#9127=CARTESIAN_POINT ( 'NONE',  ( 4.923371831947295441, -15.65773551566587685, -8.527530157486179263 ) ) ;
#9129=ORIENTED_EDGE ( 'NONE', *, *, #54687, .F. ) ;
#9140=EDGE_CURVE ( 'NONE', #22285, #41784, #72464, .T. ) ;
#9150=LINE ( 'NONE', #42004, #21850 ) ;
#9157=CARTESIAN_POINT ( 'NONE',  ( 0.1558200433086288639, 4.218224077326415689E-16, -14.62618286184525829 ) ) ;
#9159=EDGE_CURVE ( 'NONE', #81080, #44839, #52195, .T. ) ;
#9161=CARTESIAN_POINT ( 'NONE',  ( 0.000000000000000000, 0.5000000000000004441, 0.000000000000000000 ) ) ;
#9162=ORIENTED_EDGE ( 'NONE', *, *, #368, .T. ) ;
#9163=FACE_OUTER_BOUND ( 'NONE', #30817, .T. ) ;
#9166=ADVANCED_FACE ( 'NONE', ( #21209 ), #51707, .F. ) ;
#9168=CARTESIAN_POINT ( 'NONE',  ( 8.375939845167682307, 15.00000000000000000, 11.52849216984304448 ) ) ;
#9170=CARTESIAN_POINT ( 'NONE',  ( 14.42525372082711144, 0.2301507929055687240, -3.890283033989180517 ) ) ;
#9175=VERTEX_POINT ( 'NONE', #36708 ) ;
#9176=CARTESIAN_POINT ( 'NONE',  ( -11.62719953690051788, 0.5000000000000004441, -9.476720473301954328 ) ) ;
#9178=CIRCLE ( 'NONE', #23623, 15.00000000000000000 ) ;
#9184=CIRCLE ( 'NONE', #69868, 14.49999999999999822 ) ;
#9186=EDGE_LOOP ( 'NONE', ( #64457, #92181, #23407, #74927, #76119, #26006 ) ) ;
#9192=CARTESIAN_POINT ( 'NONE',  ( -8.549759589250339076, 0.2301501389895029837, 12.25250350990691572 ) ) ;
#9200=CARTESIAN_POINT ( 'NONE',  ( -7.082119434687044190, 32.63708216824731778, 12.26659068614894998 ) ) ;
#9208=ORIENTED_EDGE ( 'NONE', *, *, #80937, .T. ) ;
#9214=CARTESIAN_POINT ( 'NONE',  ( -5.803070148808410877, 4.629725225344712954E-16, 13.28812917035384267 ) ) ;
#9219=EDGE_LOOP ( 'NONE', ( #85513, #98030, #66562, #84543 ) ) ;
#9230=DIRECTION ( 'NONE',  ( -0.09584575252022721481, 0.000000000000000000, 0.9953961983671785196 ) ) ;
#9232=DIRECTION ( 'NONE',  ( 0.3665012267243070720, 0.000000000000000000, -0.9304175679820205769 ) ) ;
#9235=ORIENTED_EDGE ( 'NONE', *, *, #71364, .T. ) ;
#9236=ORIENTED_EDGE ( 'NONE', *, *, #2869, .F. ) ;
#9246=CARTESIAN_POINT ( 'NONE',  ( -4.265913727722004722, 0.04962886353675339396, -14.12300574719584034 ) ) ;
#9250=AXIS2_PLACEMENT_3D ( 'NONE', #42219, #96708, #95197 ) ;
#9254=EDGE_LOOP ( 'NONE', ( #24691, #37207, #46599, #14551 ) ) ;
#9255=AXIS2_PLACEMENT_3D ( 'NONE', #2829, #86308, #10800 ) ;
#9257=EDGE_LOOP ( 'NONE', ( #55525, #43373, #18459, #31335, #56607, #35813 ) ) ;
#9263=ORIENTED_EDGE ( 'NONE', *, *, #80380, .F. ) ;
#9264=AXIS2_PLACEMENT_3D ( 'NONE', #69635, #53642, #1159 ) ;
#9277=B_SPLINE_CURVE_WITH_KNOTS ( 'NONE', 3,
 ( #60245, #74244, #97283, #82748, #58759, #74753 ),
 .UNSPECIFIED., .F., .F.,
 ( 4, 2, 4 ),
 ( 3.409110551495907074E-05, 0.0004400426677367846201, 0.0008459942299586101829 ),
 .UNSPECIFIED. ) ;
#9278=EDGE_LOOP ( 'NONE', ( #51801, #68106, #89158, #16682, #86655, #76300 ) ) ;
#9279=EDGE_CURVE ( 'NONE', #70392, #70139, #65862, .T. ) ;
#9280=FACE_OUTER_BOUND ( 'NONE', #72739, .T. ) ;
#9282=CARTESIAN_POINT ( 'NONE',  ( -14.69266224296346479, 14.95037104324862476, 1.335284760096034695 ) ) ;
#9285=VERTEX_POINT ( 'NONE', #74522 ) ;
#9286=CARTESIAN_POINT ( 'NONE',  ( 11.94665733272772812, 0.2301501672491274575, 8.972157519073714838 ) ) ;
#9292=DIRECTION ( 'NONE',  ( 0.000000000000000000, 0.000000000000000000, 1.000000000000000000 ) ) ;
#9303=CARTESIAN_POINT ( 'NONE',  ( 0.000000000000000000, 14.49999999999999822, 0.000000000000000000 ) ) ;
#9313=LINE ( 'NONE', #62801, #36207 ) ;
#9314=CARTESIAN_POINT ( 'NONE',  ( -0.7117905103454820193, 0.000000000000000000, -5.406585696355432624 ) ) ;
#9316=AXIS2_PLACEMENT_3D ( 'NONE', #9412, #67952, #83932 ) ;
#9317=CARTESIAN_POINT ( 'NONE',  ( -12.07856007377814223, 15.00000000000000000, -8.022367888855001183 ) ) ;
#9318=VECTOR ( 'NONE', #69524, 1000.000000000000114 ) ;
#9327=LINE ( 'NONE', #40819, #2371 ) ;
#9330=EDGE_LOOP ( 'NONE', ( #54598, #67961, #80216, #59564 ) ) ;
#9335=ORIENTED_EDGE ( 'NONE', *, *, #9159, .F. ) ;
#9371=EDGE_CURVE ( 'NONE', #37098, #39036, #14117, .T. ) ;
#9373=ORIENTED_EDGE ( 'NONE', *, *, #19468, .F. ) ;
#9377=CARTESIAN_POINT ( 'NONE',  ( 4.391347328462916089, 0.2301508954901538839, 14.28069739540083738 ) ) ;
#9396=EDGE_CURVE ( 'NONE', #71843, #16281, #39879, .T. ) ;
#9404=CARTESIAN_POINT ( 'NONE',  ( 0.000000000000000000, 0.000000000000000000, 0.000000000000000000 ) ) ;
#9412=CARTESIAN_POINT ( 'NONE',  ( 0.000000000000000000, 0.000000000000000000, 0.000000000000000000 ) ) ;
#9421=DIRECTION ( 'NONE',  ( -0.1650476058606676066, 0.000000000000000000, -0.9862856015372331031 ) ) ;
#9424=DIRECTION ( 'NONE',  ( 6.661338147750940505E-14, 0.000000000000000000, 1.000000000000000000 ) ) ;
#9430=CARTESIAN_POINT ( 'NONE',  ( 13.75503023589407015, 14.95077488074853456, 5.333408231410830425 ) ) ;
#9434=ORIENTED_EDGE ( 'NONE', *, *, #94306, .F. ) ;
#9436=CARTESIAN_POINT ( 'NONE',  ( 3.866352809136213597, 0.04962897115651117991, -14.23757791217069801 ) ) ;
#9441=CARTESIAN_POINT ( 'NONE',  ( 14.16423886937410259, -5.696251165086027690, -2.602085213965210642E-15 ) ) ;
#9448=DIRECTION ( 'NONE',  ( 0.5519369853120561498, -0.000000000000000000, 0.8338858220671695465 ) ) ;
#9456=DIRECTION ( 'NONE',  ( -0.000000000000000000, -1.000000000000000000, -0.000000000000000000 ) ) ;
#9487=ORIENTED_EDGE ( 'NONE', *, *, #82436, .T. ) ;
#9492=ORIENTED_EDGE ( 'NONE', *, *, #6319, .F. ) ;
#9493=ORIENTED_EDGE ( 'NONE', *, *, #66589, .F. ) ;
#9503=ADVANCED_FACE ( 'NONE', ( #78857 ), #32386, .T. ) ;
#9508=CARTESIAN_POINT ( 'NONE',  ( -12.81628187352647608, -40.87636533006958217, 3.903127820947815962E-15 ) ) ;
#9509=VERTEX_POINT ( 'NONE', #40381 ) ;
#9510=TOROIDAL_SURFACE ( 'NONE', #15876, 14.49999999999999822, 0.5000000000000000000 ) ;
#9513=EDGE_CURVE ( 'NONE', #26946, #50486, #62866, .T. ) ;
#9529=CARTESIAN_POINT ( 'NONE',  ( 3.468686501387114429, 0.000000000000000000, 4.207853202970351703 ) ) ;
#9536=ORIENTED_EDGE ( 'NONE', *, *, #79976, .F. ) ;
#9538=VERTEX_POINT ( 'NONE', #2887 ) ;
#9544=AXIS2_PLACEMENT_3D ( 'NONE', #67886, #30355, #77336 ) ;
#9546=DIRECTION ( 'NONE',  ( 0.000000000000000000, 1.000000000000000000, 0.000000000000000000 ) ) ;
#9555=CARTESIAN_POINT ( 'NONE',  ( 14.24131928502211331, -0.03417435944610275333, 0.4973178280106892446 ) ) ;
#9558=CARTESIAN_POINT ( 'NONE',  ( 4.792102989642838651, -0.03417435944610275333, 15.26149223938176291 ) ) ;
#9561=ORIENTED_EDGE ( 'NONE', *, *, #55802, .T. ) ;
#9576=CARTESIAN_POINT ( 'NONE',  ( 10.88017736071110164, -4.644647989178486647, 2.915334737309921209 ) ) ;
#9578=CARTESIAN_POINT ( 'NONE',  ( 14.88585913059882948, 0.2301501830257872971, 1.278057234793960939 ) ) ;
#9582=CARTESIAN_POINT ( 'NONE',  ( -7.313705784284419309, 0.5000000000000004441, -13.09617149020753502 ) ) ;
#9585=FACE_OUTER_BOUND ( 'NONE', #11194, .T. ) ;
#9586=CARTESIAN_POINT ( 'NONE',  ( 11.92686044187656336, 12.18830936912751461, -2.602085213965210642E-15 ) ) ;
#9607=VECTOR ( 'NONE', #9230, 1000.000000000000000 ) ;
#9609=VERTEX_POINT ( 'NONE', #56840 ) ;
#9610=ORIENTED_EDGE ( 'NONE', *, *, #67392, .F. ) ;
#9622=EDGE_CURVE ( 'NONE', #46867, #18218, #79834, .T. ) ;
#9626=CARTESIAN_POINT ( 'NONE',  ( -8.527530157486182816, -9.407735515665871517, -4.923371831947288335 ) ) ;
#9639=EDGE_CURVE ( 'NONE', #57707, #65696, #17751, .T. ) ;
#9640=FACE_OUTER_BOUND ( 'NONE', #73323, .T. ) ;
#9642=CARTESIAN_POINT ( 'NONE',  ( 3.469446951953614189E-15, 30.37363466993042849, 12.81628187352647608 ) ) ;
#9643=ORIENTED_EDGE ( 'NONE', *, *, #28800, .F. ) ;
#9645=ORIENTED_EDGE ( 'NONE', *, *, #26323, .T. ) ;
#9646=EDGE_CURVE ( 'NONE', #11601, #15080, #27200, .T. ) ;
#9648=EDGE_LOOP ( 'NONE', ( #53660, #81650, #31401, #10037 ) ) ;
#9656=EDGE_CURVE ( 'NONE', #75294, #60216, #49822, .T. ) ;
#9659=CIRCLE ( 'NONE', #86310, 14.49999999999999822 ) ;
#9664=CARTESIAN_POINT ( 'NONE',  ( -14.26139399674453578, 3.905478766663822759E-16, -2.619664342929995282 ) ) ;
#9672=ORIENTED_EDGE ( 'NONE', *, *, #28883, .T. ) ;
#9687=CARTESIAN_POINT ( 'NONE',  ( -8.564643372776702179, 0.5000000000000004441, 12.31449893000734797 ) ) ;
#9690=PLANE ( 'NONE',  #87115 ) ;
#9693=CARTESIAN_POINT ( 'NONE',  ( 1.915564264621337554, 4.132324795315745510E-16, 14.37291249357991774 ) ) ;
#9694=CARTESIAN_POINT ( 'NONE',  ( 14.16423886937410437, 29.09541550158064638, 3.795296366450304770 ) ) ;
#9697=ADVANCED_FACE ( 'NONE', ( #43798 ), #5820, .F. ) ;
#9704=ORIENTED_EDGE ( 'NONE', *, *, #63333, .T. ) ;
#9710=CARTESIAN_POINT ( 'NONE',  ( 10.64017930668198453, 15.00000000000000000, 10.57291749337222875 ) ) ;
#9714=ORIENTED_EDGE ( 'NONE', *, *, #74034, .T. ) ;
#9715=DIRECTION ( 'NONE',  ( -0.2840153447039170387, 0.000000000000000000, -0.9588197348681947174 ) ) ;
#9728=ORIENTED_EDGE ( 'NONE', *, *, #15044, .T. ) ;
#9731=LINE ( 'NONE', #24739, #85269 ) ;
#9732=CARTESIAN_POINT ( 'NONE',  ( 14.99847009497950800, 14.49999999999999112, 0.2142307401081135487 ) ) ;
#9739=CARTESIAN_POINT ( 'NONE',  ( 13.82192141328807011, 15.00000000000000000, 4.382292601468777526 ) ) ;
#9740=EDGE_CURVE ( 'NONE', #23897, #81593, #72814, .T. ) ;
#9748=DIRECTION ( 'NONE',  ( 0.000000000000000000, 1.000000000000000000, 0.000000000000000000 ) ) ;
#9752=VERTEX_POINT ( 'NONE', #34820 ) ;
#9757=ORIENTED_EDGE ( 'NONE', *, *, #1205, .T. ) ;
#9760=DIRECTION ( 'NONE',  ( 0.000000000000000000, 0.000000000000000000, -1.000000000000000000 ) ) ;
#9763=CARTESIAN_POINT ( 'NONE',  ( -11.09922568453595382, -11.29303199673624469, -6.408140936763226492 ) ) ;
#9764=ORIENTED_EDGE ( 'NONE', *, *, #31800, .T. ) ;
#9769=ADVANCED_FACE ( 'NONE', ( #32739 ), #24770, .T. ) ;
#9779=CARTESIAN_POINT ( 'NONE',  ( 9.402796353261051010, 0.5000000000000004441, 11.68706210897763320 ) ) ;
#9780=CARTESIAN_POINT ( 'NONE',  ( 0.000000000000000000, 14.49999999999999822, 0.000000000000000000 ) ) ;
#9783=CARTESIAN_POINT ( 'NONE',  ( -15.86177583122253765, 15.00000000000000000, 2.069169861586545700 ) ) ;
#9789=CARTESIAN_POINT ( 'NONE',  ( 0.000000000000000000, 0.5000000000000004441, 0.000000000000000000 ) ) ;
#9793=AXIS2_PLACEMENT_3D ( 'NONE', #1848, #55312, #32305 ) ;
#9795=CARTESIAN_POINT ( 'NONE',  ( 9.641087339108921128, 0.04922511925147053657, -11.16671550067049878 ) ) ;
#9800=CARTESIAN_POINT ( 'NONE',  ( 13.21236992757673789, 0.000000000000000000, -5.338143956176714333 ) ) ;
#9801=VECTOR ( 'NONE', #32931, 1000.000000000000000 ) ;
#9805=CARTESIAN_POINT ( 'NONE',  ( 4.698669664746458530, 0.000000000000000000, 2.767727949825354195 ) ) ;
#9817=EDGE_CURVE ( 'NONE', #57516, #86312, #10256, .T. ) ;
#9819=CARTESIAN_POINT ( 'NONE',  ( -12.54397927573557681, 14.76930270348881002, -8.117058495689191133 ) ) ;
#9824=EDGE_LOOP ( 'NONE', ( #17145, #10361, #38287, #96638, #48377 ) ) ;
#9827=CARTESIAN_POINT ( 'NONE',  ( -4.873787042390880231, -0.03417435944610275333, 13.39061984619915791 ) ) ;
#9830=PLANE ( 'NONE',  #59567 ) ;
#9832=VECTOR ( 'NONE', #87552, 1000.000000000000000 ) ;
#9836=ORIENTED_EDGE ( 'NONE', *, *, #37057, .F. ) ;
#9838=CARTESIAN_POINT ( 'NONE',  ( -14.67697702673046933, 15.00000000000000000, 6.361111679013309761 ) ) ;
#9850=CARTESIAN_POINT ( 'NONE',  ( -12.34086200392831678, 0.000000000000000000, 7.124999999999885425 ) ) ;
#9854=B_SPLINE_CURVE_WITH_KNOTS ( 'NONE', 3,
 ( #40438, #46928, #47911, #15955, #38468, #55427 ),
 .UNSPECIFIED., .F., .F.,
 ( 4, 2, 4 ),
 ( 3.409110551435918168E-05, 0.0004400426677361854357, 0.0008459942299580117033 ),
 .UNSPECIFIED. ) ;
#9865=EDGE_CURVE ( 'NONE', #1556, #25275, #41580, .T. ) ;
#9872=ORIENTED_EDGE ( 'NONE', *, *, #18920, .F. ) ;
#9875=VERTEX_POINT ( 'NONE', #23799 ) ;
#9877=DIRECTION ( 'NONE',  ( 0.09584575252022037306, 0.000000000000000000, 0.9953961983671790748 ) ) ;
#9881=CARTESIAN_POINT ( 'NONE',  ( 10.58981376305288613, -0.03417435944610275333, -9.535111140613709679 ) ) ;
#9882=DIRECTION ( 'NONE',  ( 0.000000000000000000, 1.000000000000000000, 0.000000000000000000 ) ) ;
#9889=VERTEX_POINT ( 'NONE', #55248 ) ;
#9899=EDGE_CURVE ( 'NONE', #77971, #37161, #35525, .T. ) ;
#9901=DIRECTION ( 'NONE',  ( 0.000000000000000000, 0.000000000000000000, -1.000000000000000000 ) ) ;
#9906=ORIENTED_EDGE ( 'NONE', *, *, #4415, .F. ) ;
#9913=CARTESIAN_POINT ( 'NONE',  ( -6.715867195167532167, 15.00000000000000000, 12.85095824508320028 ) ) ;
#9921=CARTESIAN_POINT ( 'NONE',  ( 13.74385066382883913, 14.76930270348882779, -5.860428621090359336 ) ) ;
#9927=LINE ( 'NONE', #62912, #66400 ) ;
#9933=DIRECTION ( 'NONE',  ( 0.000000000000000000, 1.000000000000000000, 0.000000000000000000 ) ) ;
#9937=FACE_OUTER_BOUND ( 'NONE', #84895, .T. ) ;
#9941=DIRECTION ( 'NONE',  ( -0.8038568606172123987, 0.000000000000000000, -0.5948227867513479206 ) ) ;
#9942=CARTESIAN_POINT ( 'NONE',  ( -10.36894250292379205, -8.821251165086028578, -10.36894250292378672 ) ) ;
#9946=ORIENTED_EDGE ( 'NONE', *, *, #67793, .F. ) ;
#9948=CARTESIAN_POINT ( 'NONE',  ( -12.50534872682722565, 15.00000000000000000, -7.339363270777700343 ) ) ;
#9955=LINE ( 'NONE', #47450, #45176 ) ;
#9961=B_SPLINE_CURVE_WITH_KNOTS ( 'NONE', 3,
 ( #76475, #67503, #68983, #30964, #89508, #14014 ),
 .UNSPECIFIED., .F., .F.,
 ( 4, 2, 4 ),
 ( 3.409110551494635847E-05, 0.0004400426677367929142, 0.0008459942299586394564 ),
 .UNSPECIFIED. ) ;
#9965=ORIENTED_EDGE ( 'NONE', *, *, #17637, .T. ) ;
#9968=DIRECTION ( 'NONE',  ( 0.000000000000000000, 0.000000000000000000, 1.000000000000000000 ) ) ;
#9969=TOROIDAL_SURFACE ( 'NONE', #68997, 14.49999999999999822, 0.5000000000000000000 ) ;
#9977=TOROIDAL_SURFACE ( 'NONE', #56292, 14.49999999999999822, 0.5000000000000000000 ) ;
#9980=DIRECTION ( 'NONE',  ( -0.000000000000000000, -1.000000000000000000, -0.000000000000000000 ) ) ;
#9982=EDGE_CURVE ( 'NONE', #37318, #79695, #37208, .T. ) ;
#9989=B_SPLINE_CURVE_WITH_KNOTS ( 'NONE', 3,
 ( #34851, #58837, #89344, #30675, #88851, #83699 ),
 .UNSPECIFIED., .F., .F.,
 ( 4, 2, 4 ),
 ( 0.0002800206007755223943, 0.0006862260317143878017, 0.001092431462653253209 ),
 .UNSPECIFIED. ) ;
#9995=CARTESIAN_POINT ( 'NONE',  ( -5.056330833731550456, 15.00000000000000000, -13.58983143750704592 ) ) ;
#10010=VECTOR ( 'NONE', #98976, 1000.000000000000000 ) ;
#10012=CARTESIAN_POINT ( 'NONE',  ( -11.09922568453594316, -40.45969866340291077, 6.408140936763246920 ) ) ;
#10014=EDGE_CURVE ( 'NONE', #12471, #67320, #9955, .T. ) ;
#10021=ADVANCED_FACE ( 'NONE', ( #33414 ), #15980, .T. ) ;
#10024=ORIENTED_EDGE ( 'NONE', *, *, #49376, .F. ) ;
#10027=VERTEX_POINT ( 'NONE', #16970 ) ;
#10029=CARTESIAN_POINT ( 'NONE',  ( 10.93781366033347169, 0.5000000000000004441, -10.26470809774065351 ) ) ;
#10032=LINE ( 'NONE', #32016, #73039 ) ;
#10036=AXIS2_PLACEMENT_3D ( 'NONE', #59589, #50619, #43603 ) ;
#10037=ORIENTED_EDGE ( 'NONE', *, *, #18120, .F. ) ;
#10038=DIRECTION ( 'NONE',  ( 0.8788171126619711560, 0.000000000000000000, -0.4771587602595978028 ) ) ;
#10042=DIRECTION ( 'NONE',  ( 0.000000000000000000, 0.000000000000000000, -1.000000000000000000 ) ) ;
#10057=CARTESIAN_POINT ( 'NONE',  ( 0.000000000000000000, 15.00000000000000000, 0.000000000000000000 ) ) ;
#10058=EDGE_CURVE ( 'NONE', #23012, #13614, #66522, .T. ) ;
#10060=CARTESIAN_POINT ( 'NONE',  ( -6.715867195167276371, 15.00000000000000000, -12.85095824508335838 ) ) ;
#10070=DIRECTION ( 'NONE',  ( -0.1478094111296113511, 0.000000000000000000, 0.9890158633619168249 ) ) ;
#10075=CARTESIAN_POINT ( 'NONE',  ( 5.440088680355556150, -0.2696479891784869798, 9.422509992056138373 ) ) ;
#10077=CARTESIAN_POINT ( 'NONE',  ( 14.94699059465100888, 0.5000000000000004441, 1.259949270174915981 ) ) ;
#10080=VECTOR ( 'NONE', #35640, 1000.000000000000000 ) ;
#10087=CARTESIAN_POINT ( 'NONE',  ( 4.949168087017304707, 13.09799106954466019, -10.91454864610492059 ) ) ;
#10097=EDGE_CURVE ( 'NONE', #18033, #83367, #80605, .T. ) ;
#10106=DIRECTION ( 'NONE',  ( -0.04361938736532633420, 0.000000000000000000, -0.9990482215818581313 ) ) ;
#10108=CARTESIAN_POINT ( 'NONE',  ( -9.383624259804166812, 0.2301501999355076711, 11.62625599701874179 ) ) ;
#10121=TOROIDAL_SURFACE ( 'NONE', #27648, 14.49999999999999822, 0.5000000000000000000 ) ;
#10122=FACE_OUTER_BOUND ( 'NONE', #4375, .T. ) ;
#10125=CARTESIAN_POINT ( 'NONE',  ( -9.846743663894590881, -8.782735515665878623, 2.638427012816840111 ) ) ;
#10128=DIRECTION ( 'NONE',  ( -0.9170600743851211600, 0.000000000000000000, -0.3987490689252528031 ) ) ;
#10132=EDGE_LOOP ( 'NONE', ( #62322, #75282, #36985, #87582 ) ) ;
#10138=CARTESIAN_POINT ( 'NONE',  ( -13.55157833323626271, 14.76930270348881535, -6.292279346205571500 ) ) ;
#10144=ORIENTED_EDGE ( 'NONE', *, *, #38845, .T. ) ;
#10153=CARTESIAN_POINT ( 'NONE',  ( -11.22915323889586858, -0.03417435944610275333, 8.773176023390528044 ) ) ;
#10159=DIRECTION ( 'NONE',  ( -0.9999619230641711987, 0.000000000000000000, -0.008726535498381204903 ) ) ;
#10162=CARTESIAN_POINT ( 'NONE',  ( -1.847340224724643987, 0.04922511925147186884, -14.63671528203495065 ) ) ;
#10166=LINE ( 'NONE', #4638, #35512 ) ;
#10168=ORIENTED_EDGE ( 'NONE', *, *, #94472, .T. ) ;
#10169=CARTESIAN_POINT ( 'NONE',  ( -11.49638213510170104, 0.04922511925147123046, -9.245501498402102669 ) ) ;
#10175=CARTESIAN_POINT ( 'NONE',  ( 3.469446951953614189E-15, 8.912123368507815613, 11.92686044187656513 ) ) ;
#10176=B_SPLINE_CURVE_WITH_KNOTS ( 'NONE', 3,
 ( #61691, #54196, #6248, #36752, #21757, #9693 ),
 .UNSPECIFIED., .F., .F.,
 ( 4, 2, 4 ),
 ( 3.409110551496051408E-05, 0.0004400426677367857043, 0.0008459942299586108334 ),
 .UNSPECIFIED. ) ;
#10177=VECTOR ( 'NONE', #10229, 1000.000000000000114 ) ;
#10179=EDGE_CURVE ( 'NONE', #61376, #30551, #54941, .T. ) ;
#10180=ORIENTED_EDGE ( 'NONE', *, *, #94043, .F. ) ;
#10188=LINE ( 'NONE', #25205, #74699 ) ;
#10189=DIRECTION ( 'NONE',  ( 0.9170600743851183845, 0.000000000000000000, 0.3987490689252593534 ) ) ;
#10190=CARTESIAN_POINT ( 'NONE',  ( -13.96521320569128299, 14.95077488074852923, 4.755935267939069178 ) ) ;
#10192=CARTESIAN_POINT ( 'NONE',  ( 5.440088680355549045, -33.60298132251182324, -9.422509992056141925 ) ) ;
#10195=CARTESIAN_POINT ( 'NONE',  ( -14.03351048042399007, -0.03417435944610275333, 2.474486531753619989 ) ) ;
#10215=EDGE_CURVE ( 'NONE', #87579, #85555, #65889, .T. ) ;
#10216=DIRECTION ( 'NONE',  ( -0.3826834323650877279, 0.000000000000000000, -0.9238795325112876267 ) ) ;
#10224=CARTESIAN_POINT ( 'NONE',  ( 13.82671409943296226, -0.03417435944610275333, -3.447387012295225261 ) ) ;
#10225=CARTESIAN_POINT ( 'NONE',  ( 0.000000000000000000, 0.5000000000000004441, 0.000000000000000000 ) ) ;
#10227=VERTEX_POINT ( 'NONE', #66385 ) ;
#10229=DIRECTION ( 'NONE',  ( -0.5075383629606967650, 0.000000000000000000, -0.8616291604415300398 ) ) ;
#10234=CARTESIAN_POINT ( 'NONE',  ( 2.962741594152983993, 15.00000000000000000, 13.93860331045674883 ) ) ;
#10237=DIRECTION ( 'NONE',  ( 0.000000000000000000, 0.000000000000000000, 1.000000000000000000 ) ) ;
#10240=PLANE ( 'NONE',  #94503 ) ;
#10246=CARTESIAN_POINT ( 'NONE',  ( -1.114591949024829054, 4.106534489568945963E-16, -14.45709807627966015 ) ) ;
#10247=ORIENTED_EDGE ( 'NONE', *, *, #29623, .F. ) ;
#10256=LINE ( 'NONE', #807, #73938 ) ;
#10258=CARTESIAN_POINT ( 'NONE',  ( -6.408140936763246032, -11.70969866340290721, -11.09922568453594316 ) ) ;
#10261=ORIENTED_EDGE ( 'NONE', *, *, #42403, .T. ) ;
#10262=VECTOR ( 'NONE', #39214, 1000.000000000000000 ) ;
#10263=ORIENTED_EDGE ( 'NONE', *, *, #71711, .F. ) ;
#10266=CARTESIAN_POINT ( 'NONE',  ( 14.88232117145531141, 0.5000000000000004441, -1.875237731503139438 ) ) ;
#10271=CARTESIAN_POINT ( 'NONE',  ( 1.114591949024928752, 4.429576435485488210E-16, 14.45709807627965304 ) ) ;
#10273=CARTESIAN_POINT ( 'NONE',  ( 9.282040431732605512, 2.405573570202212963E-16, 11.30407325590345025 ) ) ;
#10277=CARTESIAN_POINT ( 'NONE',  ( -6.715867195167276371, 4.396228481599465503E-16, -12.85095824508335838 ) ) ;
#10283=DIRECTION ( 'NONE',  ( 0.8141155183563185682, 0.000000000000000000, -0.5807029557109406603 ) ) ;
#10288=CARTESIAN_POINT ( 'NONE',  ( 13.61802159414987479, 14.99999999999808509, -5.334603887713429415 ) ) ;
#10289=CIRCLE ( 'NONE', #94926, 15.00000000000000000 ) ;
#10295=EDGE_CURVE ( 'NONE', #70888, #57109, #96419, .T. ) ;
#10307=DIRECTION ( 'NONE',  ( 0.000000000000000000, 0.000000000000000000, 1.000000000000000000 ) ) ;
#10309=LINE ( 'NONE', #86798, #20217 ) ;
#10312=DIRECTION ( 'NONE',  ( 0.3173046564051031360, 0.000000000000000000, -0.9483236552061955482 ) ) ;
#10314=( GEOMETRIC_REPRESENTATION_CONTEXT ( 3 ) GLOBAL_UNCERTAINTY_ASSIGNED_CONTEXT ( ( #73472 ) ) GLOBAL_UNIT_ASSIGNED_CONTEXT ( ( #71293, #55288, #3283 ) ) REPRESENTATION_CONTEXT ( 'NONE', 'WORKASPACE' ) );
#10317=DIRECTION ( 'NONE',  ( -0.6087614290087131064, 0.000000000000000000, -0.7933533402912409382 ) ) ;
#10319=CARTESIAN_POINT ( 'NONE',  ( 5.148594389986208775, 15.00000000000000711, 13.69051944078650607 ) ) ;
#10324=VERTEX_POINT ( 'NONE', #65396 ) ;
#10336=CARTESIAN_POINT ( 'NONE',  ( -14.56368227077860844, 0.2306972965111897811, 3.337246381125087424 ) ) ;
#10361=ORIENTED_EDGE ( 'NONE', *, *, #12228, .T. ) ;
#10362=CIRCLE ( 'NONE', #55019, 15.00000000000000000 ) ;
#10363=DIRECTION ( 'NONE',  ( 0.000000000000000000, 1.000000000000000000, 0.000000000000000000 ) ) ;
#10376=VERTEX_POINT ( 'NONE', #5420 ) ;
#10387=DIRECTION ( 'NONE',  ( -0.000000000000000000, -1.000000000000000000, -0.000000000000000000 ) ) ;
#10392=ORIENTED_EDGE ( 'NONE', *, *, #63758, .T. ) ;
#10397=CARTESIAN_POINT ( 'NONE',  ( 14.03351048042395632, 15.00000000000000000, 2.474486531753810059 ) ) ;
#10405=EDGE_LOOP ( 'NONE', ( #78253, #83545, #80972, #3170 ) ) ;
#10406=DIRECTION ( 'NONE',  ( 0.8526401643540917341, 0.000000000000000000, -0.5224985647159496871 ) ) ;
#10413=ADVANCED_FACE ( 'NONE', ( #72793 ), #79332, .T. ) ;
#10422=LINE ( 'NONE', #93914, #85050 ) ;
#10427=DIRECTION ( 'NONE',  ( 0.000000000000000000, 1.000000000000000000, 0.000000000000000000 ) ) ;
#10430=CARTESIAN_POINT ( 'NONE',  ( 14.16423886937410259, 9.303748834913978527, -2.602085213965210642E-15 ) ) ;
#10433=ORIENTED_EDGE ( 'NONE', *, *, #12492, .T. ) ;
#10436=EDGE_CURVE ( 'NONE', #54278, #91250, #19320, .T. ) ;
#10437=DIRECTION ( 'NONE',  ( 3.197442310920450836E-14, 0.000000000000000000, 1.000000000000000000 ) ) ;
#10445=CARTESIAN_POINT ( 'NONE',  ( 14.04391541078763161, 4.402316570082688340E-16, 3.608107528142934228 ) ) ;
#10447=LINE ( 'NONE', #65892, #40025 ) ;
#10454=ORIENTED_EDGE ( 'NONE', *, *, #41583, .T. ) ;
#10466=ORIENTED_EDGE ( 'NONE', *, *, #46090, .F. ) ;
#10467=CARTESIAN_POINT ( 'NONE',  ( 0.000000000000000000, 14.49999999999999822, 0.000000000000000000 ) ) ;
#10478=EDGE_LOOP ( 'NONE', ( #12078, #74864, #52246, #33021 ) ) ;
#10479=ORIENTED_EDGE ( 'NONE', *, *, #48984, .F. ) ;
#10492=CARTESIAN_POINT ( 'NONE',  ( -12.81628187352647252, -25.66803199673624292, 3.434112377981066722 ) ) ;
#10493=ORIENTED_EDGE ( 'NONE', *, *, #77155, .F. ) ;
#10503=ORIENTED_EDGE ( 'NONE', *, *, #37300, .F. ) ;
#10506=ORIENTED_EDGE ( 'NONE', *, *, #18879, .T. ) ;
#10510=B_SPLINE_CURVE_WITH_KNOTS ( 'NONE', 3,
 ( #2135, #1143, #15650, #16622, #92121, #46133 ),
 .UNSPECIFIED., .F., .F.,
 ( 4, 2, 4 ),
 ( 0.0002800001862105968306, 0.0006862054174524884372, 0.001092410648694380152 ),
 .UNSPECIFIED. ) ;
#10513=FACE_OUTER_BOUND ( 'NONE', #1182, .T. ) ;
#10517=ORIENTED_EDGE ( 'NONE', *, *, #17240, .F. ) ;
#10518=AXIS2_PLACEMENT_3D ( 'NONE', #46159, #8163, #61146 ) ;
#10521=CARTESIAN_POINT ( 'NONE',  ( 5.093587308868497310, 15.00000000000000000, -15.16353404595997567 ) ) ;
#10525=ORIENTED_EDGE ( 'NONE', *, *, #5001, .T. ) ;
#10527=CIRCLE ( 'NONE', #63253, 15.00000000000000000 ) ;
#10533=DIRECTION ( 'NONE',  ( 0.9799247046208268141, 0.000000000000000000, 0.1993679344172108459 ) ) ;
#10542=DIRECTION ( 'NONE',  ( 0.000000000000000000, 1.000000000000000000, 0.000000000000000000 ) ) ;
#10545=CARTESIAN_POINT ( 'NONE',  ( 14.16423886937410259, -30.69625116508602858, -2.602085213965210642E-15 ) ) ;
#10547=AXIS2_PLACEMENT_3D ( 'NONE', #11908, #32436, #62936 ) ;
#10549=EDGE_LOOP ( 'NONE', ( #54737, #91566, #78747, #96781, #2068, #21875 ) ) ;
#10555=CARTESIAN_POINT ( 'NONE',  ( -5.795997163829992083, -0.03417435944610275333, -13.01802277140713926 ) ) ;
#10557=CARTESIAN_POINT ( 'NONE',  ( 7.595945211628243321, 4.245086020036709294E-16, 12.35117874301647056 ) ) ;
#10561=CARTESIAN_POINT ( 'NONE',  ( -10.88017736071110164, 7.855352010821508024, -2.915334737309917212 ) ) ;
#10562=LINE ( 'NONE', #72042, #61207 ) ;
#10567=EDGE_CURVE ( 'NONE', #79224, #4697, #13584, .T. ) ;
#10569=CARTESIAN_POINT ( 'NONE',  ( 5.056330833731659702, 4.503963689120695453E-16, 13.58983143750703348 ) ) ;
#10578=FACE_OUTER_BOUND ( 'NONE', #96129, .T. ) ;
#10580=ORIENTED_EDGE ( 'NONE', *, *, #74756, .F. ) ;
#10590=CARTESIAN_POINT ( 'NONE',  ( 12.98685442714197791, 15.00000000000000000, -6.449155920600934344 ) ) ;
#10592=CIRCLE ( 'NONE', #87233, 15.00000000000000000 ) ;
#10597=VERTEX_POINT ( 'NONE', #29277 ) ;
#10607=VECTOR ( 'NONE', #95232, 1000.000000000000000 ) ;
#10611=CARTESIAN_POINT ( 'NONE',  ( 9.846743663894590881, 8.717264484334116048, -2.638427012816833894 ) ) ;
#10612=ORIENTED_EDGE ( 'NONE', *, *, #71373, .T. ) ;
#10615=FACE_OUTER_BOUND ( 'NONE', #87677, .T. ) ;
#10628=ORIENTED_EDGE ( 'NONE', *, *, #77317, .T. ) ;
#10630=ORIENTED_EDGE ( 'NONE', *, *, #35460, .F. ) ;
#10632=ORIENTED_EDGE ( 'NONE', *, *, #69001, .T. ) ;
#10644=PLANE ( 'NONE',  #18117 ) ;
#10646=EDGE_CURVE ( 'NONE', #15318, #11601, #97815, .T. ) ;
#10647=ORIENTED_EDGE ( 'NONE', *, *, #10058, .T. ) ;
#10649=CARTESIAN_POINT ( 'NONE',  ( 14.82269085861168811, 15.00000000000000000, -2.299529454046961519 ) ) ;
#10654=CARTESIAN_POINT ( 'NONE',  ( 14.42525372082709012, 14.76984920709442051, 3.890283033989281769 ) ) ;
#10660=DIRECTION ( 'NONE',  ( 0.9426414910921783186, 0.000000000000000000, -0.3338068592337714025 ) ) ;
#10663=CARTESIAN_POINT ( 'NONE',  ( -11.92686044187656336, 7.870456701841145986, 3.195792623639540864 ) ) ;
#10672=CARTESIAN_POINT ( 'NONE',  ( -2.120353041430744323, 15.00000000000000000, 14.34413130794943925 ) ) ;
#10673=CARTESIAN_POINT ( 'NONE',  ( -14.16722289976693894, 14.49999999999999112, 4.928467845925465163 ) ) ;
#10676=CARTESIAN_POINT ( 'NONE',  ( -7.964842623401179544, -32.56131465584516604, -7.964842623401174215 ) ) ;
#10687=VECTOR ( 'NONE', #94572, 1000.000000000000114 ) ;
#10697=CARTESIAN_POINT ( 'NONE',  ( -13.74344568549552825, 14.76984872680916183, -5.860030649990871865 ) ) ;
#10701=ORIENTED_EDGE ( 'NONE', *, *, #23783, .T. ) ;
#10710=ORIENTED_EDGE ( 'NONE', *, *, #23751, .F. ) ;
#10713=CARTESIAN_POINT ( 'NONE',  ( 3.469446951953614189E-15, 9.171802177851546389, 11.25000000000000355 ) ) ;
#10715=DIRECTION ( 'NONE',  ( 0.000000000000000000, 0.000000000000000000, 1.000000000000000000 ) ) ;
#10725=CARTESIAN_POINT ( 'NONE',  ( -4.096035146093346846, 4.802464241948007172E-16, -13.90943910019264429 ) ) ;
#10726=EDGE_CURVE ( 'NONE', #52526, #10914, #21516, .T. ) ;
#10731=EDGE_LOOP ( 'NONE', ( #53157, #25749, #51971, #67230, #5826, #55023 ) ) ;
#10743=CIRCLE ( 'NONE', #28294, 15.00000000000000000 ) ;
#10744=ADVANCED_FACE ( 'NONE', ( #30292 ), #45813, .F. ) ;
#10745=CARTESIAN_POINT ( 'NONE',  ( 12.81628187352647608, -3.376365330069575066, -2.602085213965210642E-15 ) ) ;
#10754=CARTESIAN_POINT ( 'NONE',  ( 12.25993886608609351, 14.49999999999999112, -8.642563219313673883 ) ) ;
#10762=DIRECTION ( 'NONE',  ( 0.000000000000000000, 0.000000000000000000, 1.000000000000000000 ) ) ;
#10764=CARTESIAN_POINT ( 'NONE',  ( 14.02068044289378967, 0.3639308153356252129, 5.331089937175756077 ) ) ;
#10777=DIRECTION ( 'NONE',  ( 0.3665012267243070720, 0.000000000000000000, -0.9304175679820205769 ) ) ;
#10782=CARTESIAN_POINT ( 'NONE',  ( -0.8218345515126993517, 0.04922511925147192435, -14.72992491912911639 ) ) ;
#10784=CIRCLE ( 'NONE', #47465, 15.00000000000000000 ) ;
#10798=CARTESIAN_POINT ( 'NONE',  ( 1.909764518474428519, 0.000000000000000000, 5.107897229450606424 ) ) ;
#10799=CARTESIAN_POINT ( 'NONE',  ( -0.2078280073304304698, 14.95041468192699696, -14.75174119393810557 ) ) ;
#10800=DIRECTION ( 'NONE',  ( 0.000000000000000000, 0.000000000000000000, 1.000000000000000000 ) ) ;
#10805=CARTESIAN_POINT ( 'NONE',  ( 11.62719953690061558, 14.49999999999999112, 9.476720473301933012 ) ) ;
#10809=CARTESIAN_POINT ( 'NONE',  ( -14.71525861348292175, 14.49999999999999822, 2.908807992686482713 ) ) ;
#10829=CARTESIAN_POINT ( 'NONE',  ( -11.62006642627369146, 15.00000000000000533, 8.881585844847059263 ) ) ;
#10834=VECTOR ( 'NONE', #39641, 1000.000000000000000 ) ;
#10857=ADVANCED_FACE ( 'NONE', ( #9280 ), #90227, .F. ) ;
#10859=DIRECTION ( 'NONE',  ( -0.000000000000000000, 1.000000000000000000, -0.000000000000000000 ) ) ;
#10862=EDGE_CURVE ( 'NONE', #18218, #75294, #52286, .T. ) ;
#10873=DIRECTION ( 'NONE',  ( 0.000000000000000000, 0.000000000000000000, 1.000000000000000000 ) ) ;
#10877=CARTESIAN_POINT ( 'NONE',  ( -5.817157072110893168, 15.00000000000000000, 13.82608706751082828 ) ) ;
#10881=EDGE_CURVE ( 'NONE', #72857, #14939, #90597, .T. ) ;
#10887=CARTESIAN_POINT ( 'NONE',  ( -1.354709868695722852, 15.00000000000000000, 14.93870011653150698 ) ) ;
#10890=CARTESIAN_POINT ( 'NONE',  ( 14.35840480524201013, 0.3640475087720984604, -4.340070442838850795 ) ) ;
#10896=ORIENTED_EDGE ( 'NONE', *, *, #75848, .T. ) ;
#10902=CARTESIAN_POINT ( 'NONE',  ( -13.48255862861931043, 15.00000000000000000, 5.335786055104065895 ) ) ;
#10912=DIRECTION ( 'NONE',  ( -0.000000000000000000, -1.000000000000000000, -0.000000000000000000 ) ) ;
#10914=VERTEX_POINT ( 'NONE', #98836 ) ;
#10916=DIRECTION ( 'NONE',  ( 0.000000000000000000, 0.000000000000000000, 1.000000000000000000 ) ) ;
#10918=CARTESIAN_POINT ( 'NONE',  ( -10.36894250292378317, 2.428748834913970089, 10.36894250292379560 ) ) ;
#10920=DIRECTION ( 'NONE',  ( -0.9890158633619157147, 0.000000000000000000, -0.1478094111296180124 ) ) ;
#10921=ORIENTED_EDGE ( 'NONE', *, *, #23303, .F. ) ;
#10927=CARTESIAN_POINT ( 'NONE',  ( -3.822225673302219739, 0.000000000000000000, -3.889525102760289066 ) ) ;
#10931=EDGE_CURVE ( 'NONE', #74605, #48230, #83355, .T. ) ;
#10934=CARTESIAN_POINT ( 'NONE',  ( 4.096035146093531587, 4.098443466602401877E-16, -13.90943910019259278 ) ) ;
#10942=ADVANCED_FACE ( 'NONE', ( #73086 ), #31506, .T. ) ;
#10963=B_SPLINE_CURVE_WITH_KNOTS ( 'NONE', 3,
 ( #98567, #28552, #37051, #82539, #74040, #74538 ),
 .UNSPECIFIED., .F., .F.,
 ( 4, 2, 4 ),
 ( 0.0002800630492131261874, 0.0006862688956284150425, 0.001092474742043704006 ),
 .UNSPECIFIED. ) ;
#10966=ORIENTED_EDGE ( 'NONE', *, *, #94485, .F. ) ;
#10967=CARTESIAN_POINT ( 'NONE',  ( 13.07907619356926610, 0.2301500790491319004, 7.222187741820762064 ) ) ;
#10971=DIRECTION ( 'NONE',  ( -0.000000000000000000, -1.000000000000000000, -0.000000000000000000 ) ) ;
#10973=CARTESIAN_POINT ( 'NONE',  ( -3.927832320392339316, -0.03417435944610275333, 13.69797916712101404 ) ) ;
#10981=LINE ( 'NONE', #41502, #4780 ) ;
#10983=CARTESIAN_POINT ( 'NONE',  ( 3.434112377981060948, -29.41803199673624292, 12.81628187352647430 ) ) ;
#10985=VECTOR ( 'NONE', #44694, 999.9999999999998863 ) ;
#10993=CARTESIAN_POINT ( 'NONE',  ( -14.48718990079891888, 4.171500096121077077E-16, -0.6093675230842403590 ) ) ;
#10994=EDGE_CURVE ( 'NONE', #32864, #85555, #28455, .T. ) ;
#10998=DIRECTION ( 'NONE',  ( 0.02617694830788287394, 0.000000000000000000, -0.9996573249755571489 ) ) ;
#11000=EDGE_CURVE ( 'NONE', #5711, #8841, #53600, .T. ) ;
#11004=CARTESIAN_POINT ( 'NONE',  ( 10.32896413005679825, 7.604976035794179801, -5.963430220938286119 ) ) ;
#11010=CARTESIAN_POINT ( 'NONE',  ( -5.240693273018903753, 0.04962883216462592173, -13.79102773477921140 ) ) ;
#11014=LINE ( 'NONE', #10521, #15112 ) ;
#11020=CARTESIAN_POINT ( 'NONE',  ( -14.94699059465099822, 0.5000000000000004441, -1.259949270175015013 ) ) ;
#11025=DIRECTION ( 'NONE',  ( 0.000000000000000000, 1.000000000000000000, -0.000000000000000000 ) ) ;
#11033=CARTESIAN_POINT ( 'NONE',  ( -13.82671409943298357, 0.000000000000000000, 3.447387012295131115 ) ) ;
#11036=CARTESIAN_POINT ( 'NONE',  ( -14.16423886937409726, -37.98791783175268932, 3.795296366450320757 ) ) ;
#11047=CYLINDRICAL_SURFACE ( 'NONE', #73578, 15.00000000000000000 ) ;
#11053=CARTESIAN_POINT ( 'NONE',  ( 5.440088680355556150, 9.730352010821514241, 9.422509992056138373 ) ) ;
#11057=EDGE_CURVE ( 'NONE', #20937, #77207, #66625, .T. ) ;
#11058=CARTESIAN_POINT ( 'NONE',  ( -13.07751017357375112, 4.831904710033835254E-16, -6.263284095430687870 ) ) ;
#11059=DIRECTION ( 'NONE',  ( -0.9483236552062001001, 0.000000000000000000, 0.3173046564050899798 ) ) ;
#11062=CARTESIAN_POINT ( 'NONE',  ( 0.000000000000000000, 14.49999999999999822, 0.000000000000000000 ) ) ;
#11068=CARTESIAN_POINT ( 'NONE',  ( -9.065164099344377391, 14.63595249122790598, -11.95084933600779920 ) ) ;
#11074=DIRECTION ( 'NONE',  ( 0.000000000000000000, 1.000000000000000000, 0.000000000000000000 ) ) ;
#11078=AXIS2_PLACEMENT_3D ( 'NONE', #14655, #7139, #13642 ) ;
#11083=VECTOR ( 'NONE', #33540, 1000.000000000000000 ) ;
#11084=CARTESIAN_POINT ( 'NONE',  ( -10.14667048435152097, 4.576487713787624877E-16, 10.35833375027034542 ) ) ;
#11085=DIRECTION ( 'NONE',  ( -0.8526401643540953978, 0.000000000000000000, 0.5224985647159435809 ) ) ;
#11086=VERTEX_POINT ( 'NONE', #4622 ) ;
#11094=CARTESIAN_POINT ( 'NONE',  ( -14.88232117145528655, 15.00000000000000000, -1.875237731503337946 ) ) ;
#11098=EDGE_CURVE ( 'NONE', #87486, #22095, #58585, .T. ) ;
#11100=CARTESIAN_POINT ( 'NONE',  ( 2.638427012816829897, -0.4494021823325435872, -9.846743663894592657 ) ) ;
#11102=DIRECTION ( 'NONE',  ( 0.000000000000000000, 0.000000000000000000, 1.000000000000000000 ) ) ;
#11111=CARTESIAN_POINT ( 'NONE',  ( -13.75801628063875803, 15.00000000000000000, -4.578972376164643698 ) ) ;
#11113=ORIENTED_EDGE ( 'NONE', *, *, #73178, .T. ) ;
#11117=ORIENTED_EDGE ( 'NONE', *, *, #69915, .F. ) ;
#11119=AXIS2_PLACEMENT_3D ( 'NONE', #4436, #4921, #13897 ) ;
#11128=ORIENTED_EDGE ( 'NONE', *, *, #5230, .T. ) ;
#11135=CARTESIAN_POINT ( 'NONE',  ( -3.420591144908350589, 0.5000000000000004441, -14.60477854057960556 ) ) ;
#11137=DIRECTION ( 'NONE',  ( -0.000000000000000000, -1.000000000000000000, -0.000000000000000000 ) ) ;
#11138=EDGE_LOOP ( 'NONE', ( #71022, #22328, #43098, #88809 ) ) ;
#11144=CARTESIAN_POINT ( 'NONE',  ( 0.000000000000000000, 0.5000000000000004441, 0.000000000000000000 ) ) ;
#11147=DIRECTION ( 'NONE',  ( 0.000000000000000000, 0.000000000000000000, 1.000000000000000000 ) ) ;
#11153=CARTESIAN_POINT ( 'NONE',  ( 8.490309438743736337, 12.94122572292852347, -8.044354728829526735 ) ) ;
#11155=FACE_OUTER_BOUND ( 'NONE', #52594, .T. ) ;
#11159=CARTESIAN_POINT ( 'NONE',  ( 3.469446951953614189E-15, -20.68631465584515539, 10.88017736071110342 ) ) ;
#11161=CARTESIAN_POINT ( 'NONE',  ( -14.43100913236851568, 4.866596497322921311E-16, 1.412789942453065883 ) ) ;
#11180=ORIENTED_EDGE ( 'NONE', *, *, #32623, .F. ) ;
#11181=CARTESIAN_POINT ( 'NONE',  ( 0.000000000000000000, 0.5000000000000004441, 0.000000000000000000 ) ) ;
#11189=DIRECTION ( 'NONE',  ( -0.000000000000000000, -1.000000000000000000, -0.000000000000000000 ) ) ;
#11193=ORIENTED_EDGE ( 'NONE', *, *, #56947, .F. ) ;
#11194=EDGE_LOOP ( 'NONE', ( #45264, #6200, #82683, #40983 ) ) ;
#11196=CARTESIAN_POINT ( 'NONE',  ( 11.24999999999999822, 10.63013551118487143, -3.014428414850134796 ) ) ;
#11203=DIRECTION ( 'NONE',  ( -0.7132504491541847846, 0.000000000000000000, 0.7009092642998475675 ) ) ;
#11210=CARTESIAN_POINT ( 'NONE',  ( 0.9082943533637206635, 15.00000000000000000, -14.47152380945584760 ) ) ;
#11214=CARTESIAN_POINT ( 'NONE',  ( 7.208316651077762316, -30.86606884899920900, -7.208316651077764980 ) ) ;
#11223=CARTESIAN_POINT ( 'NONE',  ( 14.66196617519557677, 0.2306972965111900586, 2.874856965127918773 ) ) ;
#11227=CARTESIAN_POINT ( 'NONE',  ( 3.469446951953614189E-15, -4.626365330069575954, 12.81628187352647608 ) ) ;
#11228=ORIENTED_EDGE ( 'NONE', *, *, #19347, .T. ) ;
#11236=DIRECTION ( 'NONE',  ( 0.000000000000000000, 0.000000000000000000, -1.000000000000000000 ) ) ;
#11241=CARTESIAN_POINT ( 'NONE',  ( -14.43100913236851568, 15.00000000000000000, 1.412789942453067216 ) ) ;
#11249=LINE ( 'NONE', #56274, #53697 ) ;
#11254=LINE ( 'NONE', #55786, #60833 ) ;
#11265=EDGE_LOOP ( 'NONE', ( #51939, #25976, #8900, #62737 ) ) ;
#11270=DIRECTION ( 'NONE',  ( -0.000000000000000000, -1.000000000000000000, -0.000000000000000000 ) ) ;
#11273=CARTESIAN_POINT ( 'NONE',  ( -2.120353041430445895, 3.806229657360874111E-16, -14.34413130794948543 ) ) ;
#11274=FACE_OUTER_BOUND ( 'NONE', #56138, .T. ) ;
#11277=CARTESIAN_POINT ( 'NONE',  ( -11.94720539484415944, 0.2306972965111586116, 8.972309510150065393 ) ) ;
#11279=CARTESIAN_POINT ( 'NONE',  ( 0.000000000000000000, 15.00000000000000000, 0.000000000000000000 ) ) ;
#11284=DIRECTION ( 'NONE',  ( 0.000000000000000000, 0.000000000000000000, 1.000000000000000000 ) ) ;
#11285=EDGE_LOOP ( 'NONE', ( #44064, #73161, #81306, #10506 ) ) ;
#11289=PLANE ( 'NONE',  #57925 ) ;
#11292=CARTESIAN_POINT ( 'NONE',  ( -8.439016546559740206, 3.923478264313957572E-16, -11.79122553964984910 ) ) ;
#11304=CARTESIAN_POINT ( 'NONE',  ( -13.07751017358212131, 15.00000000000000000, 6.263284095430918796 ) ) ;
#11308=CARTESIAN_POINT ( 'NONE',  ( -14.64885433386000635, 14.95077488074853456, 1.748475581354107300 ) ) ;
#11312=ADVANCED_FACE ( 'NONE', ( #53055 ), #21092, .T. ) ;
#11325=CARTESIAN_POINT ( 'NONE',  ( -2.393480905993250918, 0.5000000000000004441, 14.80781041047749724 ) ) ;
#11331=ORIENTED_EDGE ( 'NONE', *, *, #50459, .F. ) ;
#11340=CARTESIAN_POINT ( 'NONE',  ( 14.42956166533737417, 15.00000000000000533, -2.386684097925001247 ) ) ;
#11349=ORIENTED_EDGE ( 'NONE', *, *, #37081, .T. ) ;
#11350=CARTESIAN_POINT ( 'NONE',  ( -12.07856007377833407, 15.00000000000000000, 8.022367888854752493 ) ) ;
#11354=DIRECTION ( 'NONE',  ( -0.000000000000000000, -1.000000000000000000, -0.000000000000000000 ) ) ;
#11358=AXIS2_PLACEMENT_3D ( 'NONE', #21497, #24457, #85439 ) ;
#11359=ADVANCED_FACE ( 'NONE', ( #45563 ), #13587, .F. ) ;
#11366=VERTEX_POINT ( 'NONE', #52084 ) ;
#11367=DIRECTION ( 'NONE',  ( 0.000000000000000000, 1.000000000000000000, 0.000000000000000000 ) ) ;
#11368=VERTEX_POINT ( 'NONE', #82577 ) ;
#11373=AXIS2_PLACEMENT_3D ( 'NONE', #11749, #86775, #3274 ) ;
#11381=ORIENTED_EDGE ( 'NONE', *, *, #3476, .F. ) ;
#11398=DIRECTION ( 'NONE',  ( -0.000000000000000000, -1.000000000000000000, -0.000000000000000000 ) ) ;
#11400=EDGE_LOOP ( 'NONE', ( #95918, #52061, #40696, #77815, #41110 ) ) ;
#11405=EDGE_CURVE ( 'NONE', #1162, #31031, #6579, .T. ) ;
#11410=DIRECTION ( 'NONE',  ( 0.000000000000000000, 0.000000000000000000, 1.000000000000000000 ) ) ;
#11440=CARTESIAN_POINT ( 'NONE',  ( -4.856044144387799300, 15.00000000000000888, 13.79699902221156371 ) ) ;
#11446=EDGE_CURVE ( 'NONE', #83367, #22095, #11730, .T. ) ;
#11453=EDGE_CURVE ( 'NONE', #83674, #39649, #10032, .T. ) ;
#11454=LINE ( 'NONE', #96953, #7401 ) ;
#11456=ORIENTED_EDGE ( 'NONE', *, *, #8812, .T. ) ;
#11471=CARTESIAN_POINT ( 'NONE',  ( 6.408140936763243367, -34.20969866340291077, 11.09922568453594494 ) ) ;
#11472=VERTEX_POINT ( 'NONE', #92048 ) ;
#11473=AXIS2_PLACEMENT_3D ( 'NONE', #66093, #21106, #44080 ) ;
#11482=EDGE_LOOP ( 'NONE', ( #38481, #88483, #86375, #21689, #80007, #90829 ) ) ;
#11489=CARTESIAN_POINT ( 'NONE',  ( 14.99847009497944406, 0.5000000000000004441, 0.2142307401081381124 ) ) ;
#11493=EDGE_CURVE ( 'NONE', #43585, #18004, #46544, .T. ) ;
#11500=PLANE ( 'NONE',  #11880 ) ;
#11502=ORIENTED_EDGE ( 'NONE', *, *, #67189, .F. ) ;
#11518=DIRECTION ( 'NONE',  ( 0.000000000000000000, 1.000000000000000000, 0.000000000000000000 ) ) ;
#11520=CARTESIAN_POINT ( 'NONE',  ( 14.16423886937410437, -35.90458449841936783, 3.795296366450304770 ) ) ;
#11526=ORIENTED_EDGE ( 'NONE', *, *, #9656, .T. ) ;
#11527=EDGE_CURVE ( 'NONE', #1561, #20489, #38565, .T. ) ;
#11533=AXIS2_PLACEMENT_3D ( 'NONE', #87619, #41656, #86654 ) ;
#11534=CARTESIAN_POINT ( 'NONE',  ( -2.815433093576914736, 14.49999999999999112, -14.73340885523760413 ) ) ;
#11539=CARTESIAN_POINT ( 'NONE',  ( 10.88017736071109987, 15.77201867748817854, -2.915334737309928315 ) ) ;
#11544=FACE_OUTER_BOUND ( 'NONE', #37227, .T. ) ;
#11548=CARTESIAN_POINT ( 'NONE',  ( 5.073789285385978509, 0.000000000000000000, -1.998618750576372838 ) ) ;
#11553=CARTESIAN_POINT ( 'NONE',  ( -0.9940297508538862292, 15.00000000000000000, 14.21528771620248932 ) ) ;
#11560=EDGE_CURVE ( 'NONE', #57214, #57542, #32520, .T. ) ;
#11568=CARTESIAN_POINT ( 'NONE',  ( 0.000000000000000000, 0.000000000000000000, 0.000000000000000000 ) ) ;
#11579=DIRECTION ( 'NONE',  ( -0.000000000000000000, -1.000000000000000000, -0.000000000000000000 ) ) ;
#11581=CARTESIAN_POINT ( 'NONE',  ( -13.55255535720598026, -0.03417435944610275333, 4.403492169842870396 ) ) ;
#11584=CARTESIAN_POINT ( 'NONE',  ( -4.856092091437838043, 14.99999999999808686, -13.79590085421244439 ) ) ;
#11586=CARTESIAN_POINT ( 'NONE',  ( 2.638427012816835227, -2.532735515665880843, 9.846743663894590881 ) ) ;
#11587=VERTEX_POINT ( 'NONE', #48504 ) ;
#11601=VERTEX_POINT ( 'NONE', #69060 ) ;
#11604=VERTEX_POINT ( 'NONE', #31040 ) ;
#11608=AXIS2_PLACEMENT_3D ( 'NONE', #63296, #72276, #79299 ) ;
#11611=EDGE_CURVE ( 'NONE', #5083, #1372, #37957, .T. ) ;
#11620=VECTOR ( 'NONE', #28950, 1000.000000000000000 ) ;
#11622=VERTEX_POINT ( 'NONE', #19007 ) ;
#11624=DIRECTION ( 'NONE',  ( -0.7009092642998523415, 0.000000000000000000, 0.7132504491541801217 ) ) ;
#11628=CARTESIAN_POINT ( 'NONE',  ( 12.11353679309432785, 14.95037110518055812, 8.421373815019714826 ) ) ;
#11629=ORIENTED_EDGE ( 'NONE', *, *, #8255, .T. ) ;
#11634=CARTESIAN_POINT ( 'NONE',  ( -10.58223187590993497, 14.76930270348881002, -10.54772123337545509 ) ) ;
#11642=EDGE_CURVE ( 'NONE', #14221, #37192, #46274, .T. ) ;
#11648=CARTESIAN_POINT ( 'NONE',  ( 6.779815635997717749, 13.03986625811624833, -9.668860777447443766 ) ) ;
#11651=CARTESIAN_POINT ( 'NONE',  ( -13.86186289918447478, 15.00000000000000888, 4.667665767314873371 ) ) ;
#11654=CARTESIAN_POINT ( 'NONE',  ( -7.964842623401172439, -31.31131465584515539, 7.964842623401183097 ) ) ;
#11670=B_SPLINE_CURVE_WITH_KNOTS ( 'NONE', 3,
 ( #25580, #32060, #56072, #9578, #62070, #10077 ),
 .UNSPECIFIED., .F., .F.,
 ( 4, 2, 4 ),
 ( 0.0002800098398849620428, 0.0006862151655504652656, 0.001092420491215968488 ),
 .UNSPECIFIED. ) ;
#11673=AXIS2_PLACEMENT_3D ( 'NONE', #89364, #74344, #19878 ) ;
#11677=ORIENTED_EDGE ( 'NONE', *, *, #51375, .T. ) ;
#11687=DIRECTION ( 'NONE',  ( -3.375077994860475883E-14, 0.000000000000000000, 1.000000000000000000 ) ) ;
#11688=CARTESIAN_POINT ( 'NONE',  ( 3.469446951953614189E-15, 10.93830936912750573, 11.92686044187656513 ) ) ;
#11689=ORIENTED_EDGE ( 'NONE', *, *, #23751, .T. ) ;
#11691=ORIENTED_EDGE ( 'NONE', *, *, #45037, .T. ) ;
#11692=EDGE_LOOP ( 'NONE', ( #12195, #84969, #93478, #57693, #53918, #14624 ) ) ;
#11705=CARTESIAN_POINT ( 'NONE',  ( 0.000000000000000000, 14.49999999999999822, 0.000000000000000000 ) ) ;
#11706=CARTESIAN_POINT ( 'NONE',  ( 7.208316651077764980, -32.11606884899921255, 7.208316651077762316 ) ) ;
#11707=ORIENTED_EDGE ( 'NONE', *, *, #53507, .T. ) ;
#11708=ORIENTED_EDGE ( 'NONE', *, *, #78248, .T. ) ;
#11710=ORIENTED_EDGE ( 'NONE', *, *, #77235, .T. ) ;
#11718=CARTESIAN_POINT ( 'NONE',  ( -5.204170427930421283E-15, 2.873634669930423602, -12.81628187352647608 ) ) ;
#11722=ORIENTED_EDGE ( 'NONE', *, *, #83097, .T. ) ;
#11728=FACE_OUTER_BOUND ( 'NONE', #76292, .T. ) ;
#11730=B_SPLINE_CURVE_WITH_KNOTS ( 'NONE', 3,
 ( #93023, #1566, #70536, #24058, #8557, #40533 ),
 .UNSPECIFIED., .F., .F.,
 ( 4, 2, 4 ),
 ( 3.409110551496096132E-05, 0.0004400426677367851079, 0.0008459942299586093156 ),
 .UNSPECIFIED. ) ;
#11732=CARTESIAN_POINT ( 'NONE',  ( 10.19513985507825993, 0.3640475087720984049, 11.00268709613225049 ) ) ;
#11733=EDGE_LOOP ( 'NONE', ( #92608, #17537, #45978, #27383 ) ) ;
#11734=VECTOR ( 'NONE', #62323, 1000.000000000000000 ) ;
#11737=CARTESIAN_POINT ( 'NONE',  ( 0.000000000000000000, 0.000000000000000000, 0.000000000000000000 ) ) ;
#11741=CIRCLE ( 'NONE', #19733, 15.00000000000000000 ) ;
#11749=CARTESIAN_POINT ( 'NONE',  ( 0.000000000000000000, 15.00000000000000000, 0.000000000000000000 ) ) ;
#11757=CARTESIAN_POINT ( 'NONE',  ( -13.14228782657349370, 14.63606917158947418, 7.230509711182151023 ) ) ;
#11758=EDGE_CURVE ( 'NONE', #8161, #43087, #57064, .T. ) ;
#11768=DIRECTION ( 'NONE',  ( 0.6755902076156591329, 0.000000000000000000, -0.7372773368101250835 ) ) ;
#11769=DIRECTION ( 'NONE',  ( -0.000000000000000000, 1.000000000000000000, -0.000000000000000000 ) ) ;
#11788=ORIENTED_EDGE ( 'NONE', *, *, #70147, .F. ) ;
#11789=CARTESIAN_POINT ( 'NONE',  ( -12.50534872682722565, 4.101355178835516792E-16, -7.339363270777700343 ) ) ;
#11795=ADVANCED_FACE ( 'NONE', ( #55748 ), #5968, .T. ) ;
#11811=CARTESIAN_POINT ( 'NONE',  ( 0.000000000000000000, 0.5000000000000004441, 0.000000000000000000 ) ) ;
#11816=LINE ( 'NONE', #73301, #36311 ) ;
#11824=ORIENTED_EDGE ( 'NONE', *, *, #33966, .F. ) ;
#11826=FACE_OUTER_BOUND ( 'NONE', #97583, .T. ) ;
#11828=ORIENTED_EDGE ( 'NONE', *, *, #97691, .T. ) ;
#11831=DIRECTION ( 'NONE',  ( -0.000000000000000000, -1.000000000000000000, -0.000000000000000000 ) ) ;
#11841=ORIENTED_EDGE ( 'NONE', *, *, #31140, .F. ) ;
#11842=CARTESIAN_POINT ( 'NONE',  ( -10.39692778084925173, 0.04962893796709067634, -10.46714871971213334 ) ) ;
#11863=EDGE_CURVE ( 'NONE', #16892, #82266, #12964, .T. ) ;
#11864=CARTESIAN_POINT ( 'NONE',  ( 11.81378540890930751, -0.03417435944610275333, 7.968498874458199488 ) ) ;
#11869=CARTESIAN_POINT ( 'NONE',  ( -1.180296924652950663, 0.000000000000000000, 5.323975374878045841 ) ) ;
#11880=AXIS2_PLACEMENT_3D ( 'NONE', #25054, #94019, #25542 ) ;
#11884=EDGE_CURVE ( 'NONE', #64703, #70287, #92748, .T. ) ;
#11886=ADVANCED_FACE ( 'NONE', ( #25748 ), #56241, .F. ) ;
#11889=CARTESIAN_POINT ( 'NONE',  ( 7.640985187756247576, 0.04962896822202483849, -12.62032702733652734 ) ) ;
#11896=CARTESIAN_POINT ( 'NONE',  ( -7.881609424765860794, -3.319945636763228996E-15, -12.32025747423903894 ) ) ;
#11904=CARTESIAN_POINT ( 'NONE',  ( -0.2851577207221824284, 0.2306972965111893648, 14.93843163678290153 ) ) ;
#11905=ORIENTED_EDGE ( 'NONE', *, *, #29234, .T. ) ;
#11908=CARTESIAN_POINT ( 'NONE',  ( 0.000000000000000000, 15.00000000000000000, 0.000000000000000000 ) ) ;
#11911=CARTESIAN_POINT ( 'NONE',  ( -14.29541133317239243, 14.76930270348881002, -4.345028136609722758 ) ) ;
#11914=VERTEX_POINT ( 'NONE', #69276 ) ;
#11918=DIRECTION ( 'NONE',  ( -0.000000000000000000, -1.000000000000000000, -0.000000000000000000 ) ) ;
#11924=DIRECTION ( 'NONE',  ( 0.000000000000000000, 0.000000000000000000, -1.000000000000000000 ) ) ;
#11926=CARTESIAN_POINT ( 'NONE',  ( 13.14228782657334804, 0.5000000000000004441, 7.230509711182329546 ) ) ;
#11929=EDGE_CURVE ( 'NONE', #59079, #63992, #797, .T. ) ;
#11950=ORIENTED_EDGE ( 'NONE', *, *, #91444, .F. ) ;
#11964=CARTESIAN_POINT ( 'NONE',  ( -6.408140936763246032, -31.70969866340291077, -11.09922568453594316 ) ) ;
#11975=ADVANCED_FACE ( 'NONE', ( #18237 ), #39593, .T. ) ;
#11998=ORIENTED_EDGE ( 'NONE', *, *, #75508, .F. ) ;
#12001=LINE ( 'NONE', #80000, #15247 ) ;
#12002=EDGE_CURVE ( 'NONE', #54148, #16083, #49693, .T. ) ;
#12008=CARTESIAN_POINT ( 'NONE',  ( -14.40939250469967448, 4.171366831970869137E-16, 1.618458416365661012 ) ) ;
#12019=CARTESIAN_POINT ( 'NONE',  ( -7.082119434687058401, -29.02958449841936073, -12.26659068614894110 ) ) ;
#12023=FACE_OUTER_BOUND ( 'NONE', #4858, .T. ) ;
#12024=CIRCLE ( 'NONE', #61479, 14.49999999999999822 ) ;
#12034=CARTESIAN_POINT ( 'NONE',  ( 5.440088680355556150, 19.73035201082151602, 9.422509992056138373 ) ) ;
#12040=DIRECTION ( 'NONE',  ( 0.3665012267242946375, -0.000000000000000000, 0.9304175679820254619 ) ) ;
#12041=COLOUR_RGB ( '', 0.66274510, 0.83137255, 0.94901961) ;
#12048=ORIENTED_EDGE ( 'NONE', *, *, #50125, .F. ) ;
#12051=CARTESIAN_POINT ( 'NONE',  ( -12.60874940350953111, 15.00000000000000000, 7.160268045226944267 ) ) ;
#12063=ORIENTED_EDGE ( 'NONE', *, *, #83219, .F. ) ;
#12068=AXIS2_PLACEMENT_3D ( 'NONE', #16233, #14768, #37271 ) ;
#12070=CARTESIAN_POINT ( 'NONE',  ( 0.000000000000000000, 0.000000000000000000, 0.000000000000000000 ) ) ;
#12071=DIRECTION ( 'NONE',  ( -0.000000000000000000, -1.000000000000000000, -0.000000000000000000 ) ) ;
#12075=CARTESIAN_POINT ( 'NONE',  ( -7.208316651077764980, 0.3839311510007899497, -7.208316651077759651 ) ) ;
#12078=ORIENTED_EDGE ( 'NONE', *, *, #67276, .F. ) ;
#12079=DIRECTION ( 'NONE',  ( -0.000000000000000000, -1.000000000000000000, -0.000000000000000000 ) ) ;
#12089=ADVANCED_FACE ( 'NONE', ( #20193 ), #58173, .T. ) ;
#12090=CIRCLE ( 'NONE', #59975, 15.00000000000000000 ) ;
#12091=VECTOR ( 'NONE', #75498, 1000.000000000000000 ) ;
#12093=EDGE_CURVE ( 'NONE', #14429, #43985, #12690, .T. ) ;
#12099=ORIENTED_EDGE ( 'NONE', *, *, #23783, .F. ) ;
#12105=CARTESIAN_POINT ( 'NONE',  ( 0.000000000000000000, 14.49999999999999822, 0.000000000000000000 ) ) ;
#12115=CARTESIAN_POINT ( 'NONE',  ( -1.175527996596911873, 15.00000000000000711, -14.57931687975697344 ) ) ;
#12119=DIRECTION ( 'NONE',  ( 0.000000000000000000, 0.000000000000000000, 1.000000000000000000 ) ) ;
#12121=CARTESIAN_POINT ( 'NONE',  ( -7.003840667633812522, 2.083701050245578834E-16, 12.84073839985649812 ) ) ;
#12127=LINE ( 'NONE', #42150, #55373 ) ;
#12130=ADVANCED_FACE ( 'NONE', ( #19211 ), #35690, .F. ) ;
#12132=ORIENTED_EDGE ( 'NONE', *, *, #67277, .T. ) ;
#12137=CARTESIAN_POINT ( 'NONE',  ( -12.35505582470280572, -0.03417435944610275333, 10.16021613965622095 ) ) ;
#12139=CARTESIAN_POINT ( 'NONE',  ( 8.838651438279566008, 0.04922511925147201456, -11.81204219878339323 ) ) ;
#12143=CARTESIAN_POINT ( 'NONE',  ( 5.440088680355556150, -25.26964798917849109, 9.422509992056138373 ) ) ;
#12147=CARTESIAN_POINT ( 'NONE',  ( -9.402796353260967521, 0.5000000000000004441, -11.68706210897770248 ) ) ;
#12148=DIRECTION ( 'NONE',  ( 0.000000000000000000, 1.000000000000000000, 0.000000000000000000 ) ) ;
#12154=CIRCLE ( 'NONE', #10518, 14.49999999999999822 ) ;
#12158=FACE_OUTER_BOUND ( 'NONE', #64512, .T. ) ;
#12162=ORIENTED_EDGE ( 'NONE', *, *, #97691, .F. ) ;
#12176=ORIENTED_EDGE ( 'NONE', *, *, #24423, .F. ) ;
#12178=CARTESIAN_POINT ( 'NONE',  ( 11.25000000000000355, 10.42180217785154639, -2.602085213965210642E-15 ) ) ;
#12192=CARTESIAN_POINT ( 'NONE',  ( -2.638427012816824124, -32.94940218233254825, 9.846743663894596210 ) ) ;
#12195=ORIENTED_EDGE ( 'NONE', *, *, #21286, .T. ) ;
#12197=CIRCLE ( 'NONE', #66518, 15.00000000000000000 ) ;
#12206=CARTESIAN_POINT ( 'NONE',  ( -6.408140936763246032, 3.290301336597092785, -11.09922568453594316 ) ) ;
#12207=EDGE_CURVE ( 'NONE', #9538, #27610, #59352, .T. ) ;
#12208=ORIENTED_EDGE ( 'NONE', *, *, #96632, .T. ) ;
#12210=ORIENTED_EDGE ( 'NONE', *, *, #368, .F. ) ;
#12219=CARTESIAN_POINT ( 'NONE',  ( -12.50534872682736065, 15.00000000000000000, 7.339363270777414350 ) ) ;
#12222=CARTESIAN_POINT ( 'NONE',  ( -9.240973841163453883, 4.157471065789850032E-16, -11.17382667070385160 ) ) ;
#12224=DIRECTION ( 'NONE',  ( 0.000000000000000000, 0.000000000000000000, 1.000000000000000000 ) ) ;
#12227=CARTESIAN_POINT ( 'NONE',  ( -1.983216688681034068, -0.03417435944610275333, 14.11131997956736406 ) ) ;
#12228=EDGE_CURVE ( 'NONE', #74162, #87326, #60154, .T. ) ;
#12238=CARTESIAN_POINT ( 'NONE',  ( -13.40508947812791796, 15.00000000000000000, -5.527528931052510863 ) ) ;
#12246=CARTESIAN_POINT ( 'NONE',  ( -2.258648100792393532, 0.04922511925146987738, 14.57890972981271993 ) ) ;
#12248=ORIENTED_EDGE ( 'NONE', *, *, #58466, .T. ) ;
#12249=DIRECTION ( 'NONE',  ( 0.000000000000000000, 1.000000000000000000, 0.000000000000000000 ) ) ;
#12253=FACE_OUTER_BOUND ( 'NONE', #50627, .T. ) ;
#12262=CARTESIAN_POINT ( 'NONE',  ( 11.22915323889580463, -0.03417435944610275333, -8.773176023390609757 ) ) ;
#12270=DIRECTION ( 'NONE',  ( 0.000000000000000000, 0.000000000000000000, 1.000000000000000000 ) ) ;
#12272=B_SPLINE_CURVE_WITH_KNOTS ( 'NONE', 3,
 ( #14396, #44867, #75370, #41342, #2852, #24365 ),
 .UNSPECIFIED., .F., .F.,
 ( 4, 2, 4 ),
 ( 3.409110551496111039E-05, 0.0004400426677367860295, 0.0008459942299586109419 ),
 .UNSPECIFIED. ) ;
#12274=CIRCLE ( 'NONE', #90495, 14.49999999999999822 ) ;
#12282=CARTESIAN_POINT ( 'NONE',  ( -11.29168986245485051, 0.2301502372707046606, -9.783658503027551134 ) ) ;
#12288=DIRECTION ( 'NONE',  ( 0.000000000000000000, 0.000000000000000000, 1.000000000000000000 ) ) ;
#12295=ADVANCED_FACE ( 'NONE', ( #89675 ), #30141, .F. ) ;
#12305=TOROIDAL_SURFACE ( 'NONE', #69777, 14.49999999999999822, 0.5000000000000000000 ) ;
#12313=DIRECTION ( 'NONE',  ( 0.000000000000000000, 0.000000000000000000, 1.000000000000000000 ) ) ;
#12314=ORIENTED_EDGE ( 'NONE', *, *, #53053, .T. ) ;
#12318=ORIENTED_EDGE ( 'NONE', *, *, #40561, .T. ) ;
#12319=DIRECTION ( 'NONE',  ( 0.000000000000000000, 0.000000000000000000, -1.000000000000000000 ) ) ;
#12321=DIRECTION ( 'NONE',  ( 0.8038568606172163955, 0.000000000000000000, 0.5948227867513425915 ) ) ;
#12323=AXIS2_PLACEMENT_3D ( 'NONE', #5178, #35663, #60625 ) ;
#12327=CARTESIAN_POINT ( 'NONE',  ( -8.731067818237040257, 12.03712336850782094, -8.731067818237033151 ) ) ;
#12335=EDGE_LOOP ( 'NONE', ( #6302, #79950, #17675, #81704, #27044, #80866 ) ) ;
#12350=CARTESIAN_POINT ( 'NONE',  ( 14.02068044289375415, 0.5000000000000004441, 5.331089937175756965 ) ) ;
#12355=CARTESIAN_POINT ( 'NONE',  ( 0.000000000000000000, 0.000000000000000000, 0.000000000000000000 ) ) ;
#12357=CARTESIAN_POINT ( 'NONE',  ( -14.04391541078767958, 4.832815575535569023E-16, 3.608107528142744602 ) ) ;
#12362=DIRECTION ( 'NONE',  ( -0.1822355254921514123, 0.000000000000000000, 0.9832549075639539504 ) ) ;
#12364=ORIENTED_EDGE ( 'NONE', *, *, #86264, .T. ) ;
#12365=CARTESIAN_POINT ( 'NONE',  ( 7.313705784284509903, 14.63595249122788999, 13.09617149020749061 ) ) ;
#12368=LINE ( 'NONE', #95887, #40938 ) ;
#12373=CARTESIAN_POINT ( 'NONE',  ( 7.674241358950872005, 0.2301500950314220029, -12.81905807005885123 ) ) ;
#12376=AXIS2_PLACEMENT_3D ( 'NONE', #47625, #85629, #17146 ) ;
#12379=CARTESIAN_POINT ( 'NONE',  ( 7.674241358951006120, 14.76984990496591621, 12.81905807006024922 ) ) ;
#12382=EDGE_LOOP ( 'NONE', ( #5896, #26599, #22069, #58151, #28062, #90487 ) ) ;
#12385=CIRCLE ( 'NONE', #20325, 14.49999999999999822 ) ;
#12386=CARTESIAN_POINT ( 'NONE',  ( -7.313705784284419309, 15.00000000000000000, -13.09617149020753502 ) ) ;
#12387=AXIS2_PLACEMENT_3D ( 'NONE', #91998, #77479, #83523 ) ;
#12390=ORIENTED_EDGE ( 'NONE', *, *, #55445, .T. ) ;
#12392=DIRECTION ( 'NONE',  ( 0.000000000000000000, 0.000000000000000000, 1.000000000000000000 ) ) ;
#12396=CARTESIAN_POINT ( 'NONE',  ( -7.313705784284471711, 14.49999999999999112, -13.09617149020757942 ) ) ;
#12398=ORIENTED_EDGE ( 'NONE', *, *, #62351, .F. ) ;
#12399=DIRECTION ( 'NONE',  ( 0.000000000000000000, 1.000000000000000000, 0.000000000000000000 ) ) ;
#12405=CARTESIAN_POINT ( 'NONE',  ( 0.000000000000000000, 14.49999999999999822, 0.000000000000000000 ) ) ;
#12420=EDGE_LOOP ( 'NONE', ( #10024, #12398, #12820, #46629 ) ) ;
#12432=CARTESIAN_POINT ( 'NONE',  ( -12.34597252984343640, 14.95037103437615755, 8.076773567935736864 ) ) ;
#12435=ORIENTED_EDGE ( 'NONE', *, *, #36367, .T. ) ;
#12440=ADVANCED_FACE ( 'NONE', ( #37190 ), #52658, .T. ) ;
#12450=ORIENTED_EDGE ( 'NONE', *, *, #13305, .F. ) ;
#12453=CARTESIAN_POINT ( 'NONE',  ( -9.382169495545422677, -26.50136533006957151, -9.382169495545417348 ) ) ;
#12454=AXIS2_PLACEMENT_3D ( 'NONE', #443, #44909, #83908 ) ;
#12463=AXIS2_PLACEMENT_3D ( 'NONE', #70588, #64042, #25104 ) ;
#12464=AXIS2_PLACEMENT_3D ( 'NONE', #11705, #48713, #57690 ) ;
#12471=VERTEX_POINT ( 'NONE', #66683 ) ;
#12480=DIRECTION ( 'NONE',  ( -0.09584575252022721481, 0.000000000000000000, 0.9953961983671785196 ) ) ;
#12486=ORIENTED_EDGE ( 'NONE', *, *, #21475, .T. ) ;
#12492=EDGE_CURVE ( 'NONE', #58402, #44777, #18629, .T. ) ;
#12499=ORIENTED_EDGE ( 'NONE', *, *, #6958, .F. ) ;
#12508=CARTESIAN_POINT ( 'NONE',  ( -5.204170427930421283E-15, -34.44625116508602503, -14.16423886937410082 ) ) ;
#12511=EDGE_LOOP ( 'NONE', ( #97985, #71298, #56134, #38783 ) ) ;
#12523=CARTESIAN_POINT ( 'NONE',  ( -7.964842623401172439, 13.68868534415483573, 7.964842623401183097 ) ) ;
#12526=VERTEX_POINT ( 'NONE', #59665 ) ;
#12527=VECTOR ( 'NONE', #91253, 1000.000000000000000 ) ;
#12531=VECTOR ( 'NONE', #95074, 1000.000000000000000 ) ;
#12534=CARTESIAN_POINT ( 'NONE',  ( 0.000000000000000000, 14.49999999999999822, 0.000000000000000000 ) ) ;
#12540=CARTESIAN_POINT ( 'NONE',  ( 3.469446951953614189E-15, 8.912123368507815613, 11.92686044187656513 ) ) ;
#12543=ORIENTED_EDGE ( 'NONE', *, *, #30838, .T. ) ;
#12547=DIRECTION ( 'NONE',  ( 0.000000000000000000, 1.000000000000000000, 0.000000000000000000 ) ) ;
#12567=DIRECTION ( 'NONE',  ( -0.6087614290087131064, 0.000000000000000000, -0.7933533402912409382 ) ) ;
#12569=EDGE_CURVE ( 'NONE', #73387, #58242, #32107, .T. ) ;
#12570=CARTESIAN_POINT ( 'NONE',  ( 8.527530157486179263, 3.092264484334125818, 4.923371831947292776 ) ) ;
#12571=ORIENTED_EDGE ( 'NONE', *, *, #69001, .F. ) ;
#12575=VERTEX_POINT ( 'NONE', #31130 ) ;
#12593=CARTESIAN_POINT ( 'NONE',  ( -6.090257717040695518, 15.00000000000000178, 13.29726560978565075 ) ) ;
#12598=ORIENTED_EDGE ( 'NONE', *, *, #32120, .T. ) ;
#12608=ORIENTED_EDGE ( 'NONE', *, *, #85248, .F. ) ;
#12609=FACE_OUTER_BOUND ( 'NONE', #54185, .T. ) ;
#12614=VECTOR ( 'NONE', #25875, 1000.000000000000000 ) ;
#12618=DIRECTION ( 'NONE',  ( 0.000000000000000000, 0.000000000000000000, -1.000000000000000000 ) ) ;
#12626=CARTESIAN_POINT ( 'NONE',  ( -13.78891971893212443, 0.5000000000000004441, 5.904717858191433244 ) ) ;
#12628=CARTESIAN_POINT ( 'NONE',  ( 9.065164099344530158, 0.5000000000000004441, -11.95084933600767307 ) ) ;
#12632=CARTESIAN_POINT ( 'NONE',  ( 7.964842623401181321, -25.06131465584515894, 7.964842623401174215 ) ) ;
#12635=ADVANCED_FACE ( 'NONE', ( #1163 ), #70628, .F. ) ;
#12638=CARTESIAN_POINT ( 'NONE',  ( -10.09792486685175916, 14.95037105583725534, -10.75589247084427136 ) ) ;
#12642=EDGE_CURVE ( 'NONE', #61749, #68154, #31624, .T. ) ;
#12648=ADVANCED_FACE ( 'NONE', ( #86124 ), #1658, .T. ) ;
#12654=DIRECTION ( 'NONE',  ( -0.000000000000000000, -1.000000000000000000, -0.000000000000000000 ) ) ;
#12664=LINE ( 'NONE', #4695, #76077 ) ;
#12670=DIRECTION ( 'NONE',  ( 0.000000000000000000, 1.000000000000000000, 0.000000000000000000 ) ) ;
#12684=CARTESIAN_POINT ( 'NONE',  ( 0.000000000000000000, 0.5000000000000004441, 0.000000000000000000 ) ) ;
#12688=CARTESIAN_POINT ( 'NONE',  ( 9.846743663894594434, -31.49106884899921610, -2.168404344971008868E-15 ) ) ;
#12690=LINE ( 'NONE', #71726, #20379 ) ;
#12698=ADVANCED_FACE ( 'NONE', ( #48106 ), #40128, .F. ) ;
#12701=CARTESIAN_POINT ( 'NONE',  ( 12.81628187352647608, 6.623634669930426710, -2.602085213965210642E-15 ) ) ;
#12702=VERTEX_POINT ( 'NONE', #40625 ) ;
#12706=ORIENTED_EDGE ( 'NONE', *, *, #87259, .F. ) ;
#12714=VECTOR ( 'NONE', #54334, 1000.000000000000000 ) ;
#12715=DIRECTION ( 'NONE',  ( -0.000000000000000000, -1.000000000000000000, -0.000000000000000000 ) ) ;
#12722=ORIENTED_EDGE ( 'NONE', *, *, #54641, .F. ) ;
#12724=CARTESIAN_POINT ( 'NONE',  ( -9.820682251645251881, 0.2306972965111889484, 11.26020669458352685 ) ) ;
#12730=CARTESIAN_POINT ( 'NONE',  ( 0.000000000000000000, 0.5000000000000004441, 0.000000000000000000 ) ) ;
#12737=VERTEX_POINT ( 'NONE', #70138 ) ;
#12748=CARTESIAN_POINT ( 'NONE',  ( 0.000000000000000000, 0.000000000000000000, 0.000000000000000000 ) ) ;
#12749=CARTESIAN_POINT ( 'NONE',  ( 10.36894250292378850, 9.928748834913969645, -10.36894250292379027 ) ) ;
#12753=CARTESIAN_POINT ( 'NONE',  ( -11.62112565934162767, 2.541098841762901017E-16, 8.881879596174677260 ) ) ;
#12755=CIRCLE ( 'NONE', #55888, 14.49999999999999822 ) ;
#12760=ORIENTED_EDGE ( 'NONE', *, *, #6319, .T. ) ;
#12767=CARTESIAN_POINT ( 'NONE',  ( -11.22915323889586858, 15.00000000000000000, 8.773176023390528044 ) ) ;
#12791=DIRECTION ( 'NONE',  ( 3.907985046680550391E-14, 0.000000000000000000, 1.000000000000000000 ) ) ;
#12796=CARTESIAN_POINT ( 'NONE',  ( 12.84737282370068812, -0.03417435944610275333, 9.530079116402468742 ) ) ;
#12798=ADVANCED_FACE ( 'NONE', ( #41125 ), #97125, .T. ) ;
#12801=EDGE_LOOP ( 'NONE', ( #2767, #54205, #2648, #81023 ) ) ;
#12805=ORIENTED_EDGE ( 'NONE', *, *, #44754, .F. ) ;
#12818=ORIENTED_EDGE ( 'NONE', *, *, #24306, .T. ) ;
#12820=ORIENTED_EDGE ( 'NONE', *, *, #98965, .F. ) ;
#12825=DIRECTION ( 'NONE',  ( 0.000000000000000000, 1.000000000000000000, 0.000000000000000000 ) ) ;
#12827=VECTOR ( 'NONE', #29188, 1000.000000000000000 ) ;
#12829=ORIENTED_EDGE ( 'NONE', *, *, #10436, .T. ) ;
#12840=LINE ( 'NONE', #82322, #43579 ) ;
#12841=CARTESIAN_POINT ( 'NONE',  ( -7.109031286574947650, 14.95037114371795894, 12.92745085449634246 ) ) ;
#12844=CARTESIAN_POINT ( 'NONE',  ( -14.47650479471824880, 0.5000000000000004441, 3.928206833721914482 ) ) ;
#12849=ORIENTED_EDGE ( 'NONE', *, *, #87380, .F. ) ;
#12850=CARTESIAN_POINT ( 'NONE',  ( 9.383624259804008716, 14.76984980006448822, 11.62625599701886792 ) ) ;
#12865=LINE ( 'NONE', #88874, #74945 ) ;
#12868=ORIENTED_EDGE ( 'NONE', *, *, #73420, .F. ) ;
#12872=DIRECTION ( 'NONE',  ( -0.6225146366376237417, 0.000000000000000000, 0.7826081568524104748 ) ) ;
#12874=CARTESIAN_POINT ( 'NONE',  ( 0.000000000000000000, 0.5000000000000004441, 0.000000000000000000 ) ) ;
#12888=CARTESIAN_POINT ( 'NONE',  ( -3.715841784917612856, 15.00000000000000000, -15.55859621770273193 ) ) ;
#12889=ORIENTED_EDGE ( 'NONE', *, *, #6776, .F. ) ;
#12897=CARTESIAN_POINT ( 'NONE',  ( 14.47650479471819551, 15.00000000000000000, 3.928206833722108549 ) ) ;
#12901=CARTESIAN_POINT ( 'NONE',  ( 0.000000000000000000, 14.49999999999999822, 0.000000000000000000 ) ) ;
#12902=FACE_OUTER_BOUND ( 'NONE', #40109, .T. ) ;
#12913=CARTESIAN_POINT ( 'NONE',  ( 0.000000000000000000, 0.5000000000000004441, 0.000000000000000000 ) ) ;
#12914=CARTESIAN_POINT ( 'NONE',  ( -11.96291822454885612, 15.00000000000000000, 8.193813980848972278 ) ) ;
#12921=ORIENTED_EDGE ( 'NONE', *, *, #10931, .T. ) ;
#12922=AXIS2_PLACEMENT_3D ( 'NONE', #87531, #10070, #26057 ) ;
#12924=ADVANCED_FACE ( 'NONE', ( #65560 ), #56605, .F. ) ;
#12926=CARTESIAN_POINT ( 'NONE',  ( -13.74385066382875920, 0.2306972965111898921, -5.860428621090559176 ) ) ;
#12928=ORIENTED_EDGE ( 'NONE', *, *, #88860, .T. ) ;
#12932=CIRCLE ( 'NONE', #96024, 14.49999999999999822 ) ;
#12933=CARTESIAN_POINT ( 'NONE',  ( 14.16722289976685012, 0.5000000000000004441, -4.928467845925517565 ) ) ;
#12939=CARTESIAN_POINT ( 'NONE',  ( 8.502721643904001425, 14.95037103750703622, 12.05657636697107904 ) ) ;
#12943=CARTESIAN_POINT ( 'NONE',  ( 11.09922568453594671, -12.95969866340290721, -6.408140936763241591 ) ) ;
#12951=TOROIDAL_SURFACE ( 'NONE', #28930, 14.49999999999999822, 0.5000000000000000000 ) ;
#12952=CARTESIAN_POINT ( 'NONE',  ( -13.34343830728411184, 0.3639313252796100850, 6.852200678592532235 ) ) ;
#12953=VERTEX_POINT ( 'NONE', #27568 ) ;
#12964=B_SPLINE_CURVE_WITH_KNOTS ( 'NONE', 3,
 ( #10246, #70758, #85752, #69764, #17750, #31746 ),
 .UNSPECIFIED., .F., .F.,
 ( 4, 2, 4 ),
 ( 0.0002800267093086770119, 0.0006862322000164198209, 0.001092437690724162467 ),
 .UNSPECIFIED. ) ;
#12969=LINE ( 'NONE', #73964, #11620 ) ;
#12973=CARTESIAN_POINT ( 'NONE',  ( 0.1034006766821532752, 4.444999227851523509E-16, 14.49963131600461175 ) ) ;
#12977=CARTESIAN_POINT ( 'NONE',  ( 2.962741594153077251, -0.03417435944610275333, -13.93860331045673107 ) ) ;
#12985=VERTEX_POINT ( 'NONE', #14937 ) ;
#12994=CARTESIAN_POINT ( 'NONE',  ( 3.469446951953614189E-15, -21.94625116508602858, 14.16423886937410259 ) ) ;
#13011=CARTESIAN_POINT ( 'NONE',  ( -7.964842623401172439, 18.68868534415485172, 7.964842623401183097 ) ) ;
#13015=EDGE_LOOP ( 'NONE', ( #32019, #87831, #74247, #2168 ) ) ;
#13019=CIRCLE ( 'NONE', #92885, 14.49999999999999822 ) ;
#13031=VERTEX_POINT ( 'NONE', #68915 ) ;
#13044=EDGE_CURVE ( 'NONE', #51389, #21190, #84343, .T. ) ;
#13053=DIRECTION ( 'NONE',  ( -0.8870108331782244893, 0.000000000000000000, 0.4617486132350284711 ) ) ;
#13059=EDGE_CURVE ( 'NONE', #98886, #87109, #49593, .T. ) ;
#13061=CARTESIAN_POINT ( 'NONE',  ( -9.846743663894590881, 11.21726448433411605, 2.638427012816840111 ) ) ;
#13064=VERTEX_POINT ( 'NONE', #98944 ) ;
#13078=EDGE_LOOP ( 'NONE', ( #50318, #15577, #90776, #94491 ) ) ;
#13080=ORIENTED_EDGE ( 'NONE', *, *, #16997, .F. ) ;
#13085=CARTESIAN_POINT ( 'NONE',  ( 1.175527996597151903, 2.337810934421868936E-16, -14.57931687975703205 ) ) ;
#13088=AXIS2_PLACEMENT_3D ( 'NONE', #97950, #22927, #75908 ) ;
#13094=EDGE_CURVE ( 'NONE', #26759, #17506, #55647, .T. ) ;
#13095=CARTESIAN_POINT ( 'NONE',  ( 14.47650479471823637, 14.63595249122792907, -3.928206833722017510 ) ) ;
#13096=AXIS2_PLACEMENT_3D ( 'NONE', #58310, #52310, #82802 ) ;
#13097=AXIS2_PLACEMENT_3D ( 'NONE', #45527, #60028, #84028 ) ;
#13099=CARTESIAN_POINT ( 'NONE',  ( -10.15753629091561550, 13.12143304556736112, 6.250710446193390446 ) ) ;
#13101=CARTESIAN_POINT ( 'NONE',  ( 0.000000000000000000, 14.49999999999999822, 0.000000000000000000 ) ) ;
#13103=CARTESIAN_POINT ( 'NONE',  ( 13.82192141328812518, 4.718101003023380916E-16, -4.382292601468683380 ) ) ;
#13104=ORIENTED_EDGE ( 'NONE', *, *, #11453, .F. ) ;
#13105=CARTESIAN_POINT ( 'NONE',  ( 14.03351048042395632, 0.000000000000000000, 2.474486531753810059 ) ) ;
#13106=TOROIDAL_SURFACE ( 'NONE', #64202, 14.49999999999999822, 0.5000000000000000000 ) ;
#13108=LINE ( 'NONE', #21615, #21163 ) ;
#13114=DIRECTION ( 'NONE',  ( 0.000000000000000000, 1.000000000000000000, 0.000000000000000000 ) ) ;
#13116=VERTEX_POINT ( 'NONE', #31172 ) ;
#13128=CARTESIAN_POINT ( 'NONE',  ( 7.964842623401177768, -23.81131465584515539, -7.964842623401181321 ) ) ;
#13135=AXIS2_PLACEMENT_3D ( 'NONE', #95354, #3877, #39899 ) ;
#13144=ORIENTED_EDGE ( 'NONE', *, *, #81629, .T. ) ;
#13153=DIRECTION ( 'NONE',  ( 0.000000000000000000, 1.000000000000000000, 0.000000000000000000 ) ) ;
#13154=DIRECTION ( 'NONE',  ( 0.000000000000000000, 1.000000000000000000, 0.000000000000000000 ) ) ;
#13155=EDGE_CURVE ( 'NONE', #64180, #86629, #55149, .T. ) ;
#13157=VECTOR ( 'NONE', #97414, 1000.000000000000000 ) ;
#13158=DIRECTION ( 'NONE',  ( -0.000000000000000000, 1.000000000000000000, 0.000000000000000000 ) ) ;
#13160=ORIENTED_EDGE ( 'NONE', *, *, #95536, .F. ) ;
#13161=ORIENTED_EDGE ( 'NONE', *, *, #78495, .F. ) ;
#13162=CARTESIAN_POINT ( 'NONE',  ( 6.689969769698871360, 15.00000000000000000, 12.58200319823975022 ) ) ;
#13176=CARTESIAN_POINT ( 'NONE',  ( -2.888614318722246832, 2.439454888092384977E-16, -14.33855829812827665 ) ) ;
#13181=CARTESIAN_POINT ( 'NONE',  ( -4.923371831947302546, -39.82440218233254825, -8.527530157486173934 ) ) ;
#13184=VECTOR ( 'NONE', #55820, 1000.000000000000000 ) ;
#13185=EDGE_LOOP ( 'NONE', ( #92107, #29061, #203, #66150, #22609, #18544 ) ) ;
#13190=CARTESIAN_POINT ( 'NONE',  ( 0.000000000000000000, 15.00000000000000000, 0.000000000000000000 ) ) ;
#13191=VECTOR ( 'NONE', #83248, 1000.000000000000227 ) ;
#13194=CARTESIAN_POINT ( 'NONE',  ( 9.382169495545415572, 12.24863466993041961, -9.382169495545422677 ) ) ;
#13198=EDGE_LOOP ( 'NONE', ( #27813, #38653, #74289, #83034 ) ) ;
#13200=ORIENTED_EDGE ( 'NONE', *, *, #91835, .F. ) ;
#13209=CARTESIAN_POINT ( 'NONE',  ( 0.000000000000000000, 15.00000000000000000, 0.000000000000000000 ) ) ;
#13213=CARTESIAN_POINT ( 'NONE',  ( -2.120353041430744323, 4.696395766537044518E-16, 14.34413130794943925 ) ) ;
#13218=VERTEX_POINT ( 'NONE', #23708 ) ;
#13231=CARTESIAN_POINT ( 'NONE',  ( 14.49440716394870954, 15.00000000000000000, 0.4026921475167317688 ) ) ;
#13237=CARTESIAN_POINT ( 'NONE',  ( -3.836325488035988052, 0.5000000000000004441, -14.50112432709427424 ) ) ;
#13241=CARTESIAN_POINT ( 'NONE',  ( 9.402796353261051010, 15.00000000000000000, 11.68706210897763320 ) ) ;
#13248=LINE ( 'NONE', #96274, #44114 ) ;
#13249=CIRCLE ( 'NONE', #94694, 14.49999999999999822 ) ;
#13250=CARTESIAN_POINT ( 'NONE',  ( -3.795296366450322534, 10.76208216824729647, -14.16423886937409904 ) ) ;
#13261=CARTESIAN_POINT ( 'NONE',  ( -13.64884605730320644, 15.00000000000000000, 8.341846182955681144 ) ) ;
#13262=DIRECTION ( 'NONE',  ( -0.000000000000000000, -1.000000000000000000, -0.000000000000000000 ) ) ;
#13266=ORIENTED_EDGE ( 'NONE', *, *, #43152, .F. ) ;
#13269=CARTESIAN_POINT ( 'NONE',  ( -12.22506292814009576, 0.2306972965111887819, -8.589871424854882420 ) ) ;
#13273=CARTESIAN_POINT ( 'NONE',  ( 8.470640952597564777, -3.685863869977086348E-15, -11.92295067084766380 ) ) ;
#13283=ADVANCED_FACE ( 'NONE', ( #53196 ), #24188, .T. ) ;
#13285=ORIENTED_EDGE ( 'NONE', *, *, #49353, .F. ) ;
#13305=EDGE_CURVE ( 'NONE', #35666, #48192, #22180, .T. ) ;
#13312=AXIS2_PLACEMENT_3D ( 'NONE', #53354, #66382, #98897 ) ;
#13321=AXIS2_PLACEMENT_3D ( 'NONE', #3273, #16803, #10283 ) ;
#13327=DIRECTION ( 'NONE',  ( 0.000000000000000000, 0.000000000000000000, 1.000000000000000000 ) ) ;
#13337=EDGE_CURVE ( 'NONE', #17685, #28441, #92649, .T. ) ;
#13339=CARTESIAN_POINT ( 'NONE',  ( -4.862001128006866679, 15.00000000000000000, 13.66056166602454347 ) ) ;
#13346=DIRECTION ( 'NONE',  ( -0.000000000000000000, -1.000000000000000000, -0.000000000000000000 ) ) ;
#13361=EDGE_CURVE ( 'NONE', #30230, #43585, #55661, .T. ) ;
#13365=DIRECTION ( 'NONE',  ( 0.000000000000000000, 1.000000000000000000, 0.000000000000000000 ) ) ;
#13368=ORIENTED_EDGE ( 'NONE', *, *, #32527, .T. ) ;
#13370=CARTESIAN_POINT ( 'NONE',  ( -2.815433093576927170, 15.00000000000000000, -14.73340885523753663 ) ) ;
#13376=ORIENTED_EDGE ( 'NONE', *, *, #78245, .T. ) ;
#13379=ORIENTED_EDGE ( 'NONE', *, *, #47254, .T. ) ;
#13400=DIRECTION ( 'NONE',  ( -4.085620730620576069E-14, 0.000000000000000000, 1.000000000000000000 ) ) ;
#13401=CARTESIAN_POINT ( 'NONE',  ( 2.933660812629996339, 15.00000000000000000, -15.72485391577589731 ) ) ;
#13418=ORIENTED_EDGE ( 'NONE', *, *, #35938, .F. ) ;
#13423=CARTESIAN_POINT ( 'NONE',  ( 7.551349515323185990, -0.03417435944610275333, -12.08468537022906020 ) ) ;
#13425=ORIENTED_EDGE ( 'NONE', *, *, #93354, .F. ) ;
#13439=CARTESIAN_POINT ( 'NONE',  ( 11.09922568453594671, -17.95969866340290721, -6.408140936763241591 ) ) ;
#13454=ADVANCED_FACE ( 'NONE', ( #19616 ), #49606, .F. ) ;
#13457=CIRCLE ( 'NONE', #69354, 14.49999999999999822 ) ;
#13460=CARTESIAN_POINT ( 'NONE',  ( -12.54397927573574378, 0.2306972965111899199, 8.117058495688928232 ) ) ;
#13467=CARTESIAN_POINT ( 'NONE',  ( 14.76100041229769744, 14.76930270348882068, 2.313205896730931244 ) ) ;
#13475=LINE ( 'NONE', #43467, #58182 ) ;
#13477=CARTESIAN_POINT ( 'NONE',  ( 0.000000000000000000, 14.49999999999999822, 0.000000000000000000 ) ) ;
#13489=CARTESIAN_POINT ( 'NONE',  ( -5.056330833731841778, 4.586016791640643039E-16, 13.58983143750696421 ) ) ;
#13490=ORIENTED_EDGE ( 'NONE', *, *, #11929, .T. ) ;
#13497=DIRECTION ( 'NONE',  ( -0.000000000000000000, -1.000000000000000000, -0.000000000000000000 ) ) ;
#13500=CARTESIAN_POINT ( 'NONE',  ( 3.795296366450314540, -16.73791783175269998, 14.16423886937410082 ) ) ;
#13510=DIRECTION ( 'NONE',  ( -0.000000000000000000, -1.000000000000000000, -0.000000000000000000 ) ) ;
#13515=CARTESIAN_POINT ( 'NONE',  ( 10.88017736071110164, 30.35535201082151957, 2.915334737309921209 ) ) ;
#13520=ORIENTED_EDGE ( 'NONE', *, *, #70897, .F. ) ;
#13523=DIRECTION ( 'NONE',  ( 0.000000000000000000, 0.000000000000000000, 1.000000000000000000 ) ) ;
#13530=DIRECTION ( 'NONE',  ( -0.000000000000000000, 1.000000000000000000, -0.000000000000000000 ) ) ;
#13532=ORIENTED_EDGE ( 'NONE', *, *, #75556, .F. ) ;
#13543=CARTESIAN_POINT ( 'NONE',  ( 14.17193700899789022, 15.00000000000000000, 1.489530601564113654 ) ) ;
#13557=CARTESIAN_POINT ( 'NONE',  ( 12.11331110855140736, 14.95077488074852923, -8.421032842869449198 ) ) ;
#13560=CARTESIAN_POINT ( 'NONE',  ( -2.638427012816824124, 12.05059781766744997, 9.846743663894596210 ) ) ;
#13561=ORIENTED_EDGE ( 'NONE', *, *, #38726, .F. ) ;
#13570=VECTOR ( 'NONE', #79110, 999.9999999999998863 ) ;
#13574=ORIENTED_EDGE ( 'NONE', *, *, #40068, .F. ) ;
#13578=ORIENTED_EDGE ( 'NONE', *, *, #70114, .T. ) ;
#13584=CIRCLE ( 'NONE', #67836, 14.49999999999999822 ) ;
#13587=PLANE ( 'NONE',  #34707 ) ;
#13589=CARTESIAN_POINT ( 'NONE',  ( -5.625000000000007994, 9.284700295649319202, -9.742785792574931492 ) ) ;
#13596=ORIENTED_EDGE ( 'NONE', *, *, #10179, .F. ) ;
#13602=CARTESIAN_POINT ( 'NONE',  ( 5.845017550302928022, 15.00000000000000000, 14.89003580495037582 ) ) ;
#13603=ORIENTED_EDGE ( 'NONE', *, *, #81198, .T. ) ;
#13604=CARTESIAN_POINT ( 'NONE',  ( 9.240973841163597768, 15.00000000000000000, -11.17382667070370061 ) ) ;
#13609=EDGE_CURVE ( 'NONE', #58939, #10027, #4633, .T. ) ;
#13613=TOROIDAL_SURFACE ( 'NONE', #51951, 14.49999999999999822, 0.5000000000000000000 ) ;
#13614=VERTEX_POINT ( 'NONE', #74083 ) ;
#13622=CARTESIAN_POINT ( 'NONE',  ( 13.16767742306549493, 14.95037115937769912, 6.653539137818540006 ) ) ;
#13625=CARTESIAN_POINT ( 'NONE',  ( -10.88017736071109987, -11.72798132251182501, 2.915334737309934532 ) ) ;
#13627=CARTESIAN_POINT ( 'NONE',  ( 13.40508947812166873, 4.119406375368599477E-16, -5.527528931046103544 ) ) ;
#13629=CARTESIAN_POINT ( 'NONE',  ( 13.14228782657344219, 14.63606917158947418, -7.230509711182243393 ) ) ;
#13631=CARTESIAN_POINT ( 'NONE',  ( 1.847237859018642459, 14.95037103927854538, 14.63711110085122158 ) ) ;
#13636=VECTOR ( 'NONE', #51143, 1000.000000000000000 ) ;
#13642=DIRECTION ( 'NONE',  ( 0.000000000000000000, 0.000000000000000000, -1.000000000000000000 ) ) ;
#13649=AXIS2_PLACEMENT_3D ( 'NONE', #97606, #29067, #23078 ) ;
#13651=DIRECTION ( 'NONE',  ( -0.5664062369248259454, 0.000000000000000000, -0.8241261886220204724 ) ) ;
#13652=EDGE_CURVE ( 'NONE', #87109, #76776, #7694, .T. ) ;
#13655=CARTESIAN_POINT ( 'NONE',  ( 8.209432707284774366, 0.5000000000000004441, 12.55409154915492032 ) ) ;
#13658=ORIENTED_EDGE ( 'NONE', *, *, #88708, .T. ) ;
#13676=CARTESIAN_POINT ( 'NONE',  ( 7.208316651077764980, -27.11606884899921255, 7.208316651077762316 ) ) ;
#13679=ORIENTED_EDGE ( 'NONE', *, *, #25432, .T. ) ;
#13680=ORIENTED_EDGE ( 'NONE', *, *, #61404, .F. ) ;
#13686=CYLINDRICAL_SURFACE ( 'NONE', #55806, 15.00000000000000000 ) ;
#13689=EDGE_CURVE ( 'NONE', #65696, #4144, #24889, .T. ) ;
#13691=CARTESIAN_POINT ( 'NONE',  ( 12.81628187352647252, 26.83196800326376419, -3.434112377981059172 ) ) ;
#13701=CARTESIAN_POINT ( 'NONE',  ( 9.065164099344453774, 0.5000000000000004441, 11.95084933600773169 ) ) ;
#13705=DIRECTION ( 'NONE',  ( -0.9537169507482278208, 0.000000000000000000, 0.3007057995042701770 ) ) ;
#13706=ORIENTED_EDGE ( 'NONE', *, *, #66616, .T. ) ;
#13709=CYLINDRICAL_SURFACE ( 'NONE', #23786, 15.00000000000000000 ) ;
#13710=DIRECTION ( 'NONE',  ( 0.000000000000000000, 0.000000000000000000, 1.000000000000000000 ) ) ;
#13715=CARTESIAN_POINT ( 'NONE',  ( 10.70613742633613796, 15.00000000000000000, 9.778988772292906972 ) ) ;
#13722=CARTESIAN_POINT ( 'NONE',  ( 12.60589901313222505, 14.49999999999999112, 8.129656208642151327 ) ) ;
#13725=CARTESIAN_POINT ( 'NONE',  ( 12.83294900548058415, 0.5000000000000004441, 7.766300266068450142 ) ) ;
#13731=PRODUCT_CONTEXT ( 'NONE', #52544, 'mechanical' ) ;
#13732=CARTESIAN_POINT ( 'NONE',  ( -10.32896413005680536, 7.245456701841145097, -5.963430220938272797 ) ) ;
#13733=AXIS2_PLACEMENT_3D ( 'NONE', #86856, #4355, #93858 ) ;
#13741=CARTESIAN_POINT ( 'NONE',  ( 12.84737282370068812, 15.00000000000000000, 9.530079116402468742 ) ) ;
#13743=CARTESIAN_POINT ( 'NONE',  ( -13.74344568549460455, 0.2301512731879738205, 5.860030649989552920 ) ) ;
#13745=FACE_OUTER_BOUND ( 'NONE', #68575, .T. ) ;
#13748=DIRECTION ( 'NONE',  ( 0.000000000000000000, 0.000000000000000000, 1.000000000000000000 ) ) ;
#13749=CARTESIAN_POINT ( 'NONE',  ( -12.26659068614894110, 12.22041550158064283, 7.082119434687058401 ) ) ;
#13755=VERTEX_POINT ( 'NONE', #59584 ) ;
#13759=CARTESIAN_POINT ( 'NONE',  ( 15.08495336817614607, -0.03417435944610275333, -5.321802168063438643 ) ) ;
#13761=CARTESIAN_POINT ( 'NONE',  ( 0.000000000000000000, 0.5000000000000004441, 0.000000000000000000 ) ) ;
#13765=VERTEX_POINT ( 'NONE', #42616 ) ;
#13769=DIRECTION ( 'NONE',  ( 0.000000000000000000, 0.000000000000000000, 1.000000000000000000 ) ) ;
#13779=AXIS2_PLACEMENT_3D ( 'NONE', #27530, #26547, #72528 ) ;
#13791=EDGE_CURVE ( 'NONE', #95455, #75433, #63881, .T. ) ;
#13802=ORIENTED_EDGE ( 'NONE', *, *, #49376, .T. ) ;
#13806=EDGE_LOOP ( 'NONE', ( #57212, #74554, #80511, #59788 ) ) ;
#13811=ORIENTED_EDGE ( 'NONE', *, *, #2089, .F. ) ;
#13814=EDGE_CURVE ( 'NONE', #32242, #29178, #47535, .T. ) ;
#13819=ORIENTED_EDGE ( 'NONE', *, *, #88208, .F. ) ;
#13824=FACE_OUTER_BOUND ( 'NONE', #98594, .T. ) ;
#13830=TOROIDAL_SURFACE ( 'NONE', #61772, 14.49999999999999822, 0.5000000000000000000 ) ;
#13839=DIRECTION ( 'NONE',  ( 0.7009092642998574485, 0.000000000000000000, -0.7132504491541751257 ) ) ;
#13850=EDGE_CURVE ( 'NONE', #7375, #32515, #70213, .T. ) ;
#13853=CARTESIAN_POINT ( 'NONE',  ( -10.76493118081697276, 15.00000000000000711, 9.902252441915640802 ) ) ;
#13860=VECTOR ( 'NONE', #49916, 1000.000000000000000 ) ;
#13864=DIRECTION ( 'NONE',  ( 0.000000000000000000, 0.000000000000000000, 1.000000000000000000 ) ) ;
#13875=CARTESIAN_POINT ( 'NONE',  ( 8.731067818237031375, 2.813309369127509285, -8.731067818237036704 ) ) ;
#13885=CARTESIAN_POINT ( 'NONE',  ( -11.25000000000000178, 7.921802177851544613, 3.951965214266261022E-15 ) ) ;
#13892=CARTESIAN_POINT ( 'NONE',  ( -14.26139399674456776, 15.00000000000000000, 2.619664342929695966 ) ) ;
#13897=DIRECTION ( 'NONE',  ( 0.9999619230641714207, 0.000000000000000000, -0.008726535498360278933 ) ) ;
#13902=CARTESIAN_POINT ( 'NONE',  ( 0.000000000000000000, 2.500000000000005773, 0.000000000000000000 ) ) ;
#13903=CARTESIAN_POINT ( 'NONE',  ( -14.29730467489535428, 3.987535082655999417E-16, 2.416004766803123260 ) ) ;
#13908=VECTOR ( 'NONE', #3110, 1000.000000000000000 ) ;
#13914=EDGE_CURVE ( 'NONE', #25080, #83450, #39734, .T. ) ;
#13934=EDGE_LOOP ( 'NONE', ( #95048, #38925, #90566, #3895, #10493, #91293 ) ) ;
#13937=FACE_OUTER_BOUND ( 'NONE', #41254, .T. ) ;
#13938=DIRECTION ( 'NONE',  ( 0.000000000000000000, 1.000000000000000000, 0.000000000000000000 ) ) ;
#13942=TOROIDAL_SURFACE ( 'NONE', #28337, 14.49999999999999822, 0.5000000000000000000 ) ;
#13950=CARTESIAN_POINT ( 'NONE',  ( -11.09922568453595382, -16.29303199673624292, -6.408140936763226492 ) ) ;
#13968=ORIENTED_EDGE ( 'NONE', *, *, #86479, .T. ) ;
#13976=TOROIDAL_SURFACE ( 'NONE', #95397, 14.49999999999999822, 0.5000000000000000000 ) ;
#13980=VERTEX_POINT ( 'NONE', #94459 ) ;
#13986=CARTESIAN_POINT ( 'NONE',  ( 11.36220558718857099, 4.586546245355948473E-16, 9.008345252845320061 ) ) ;
#13989=EDGE_CURVE ( 'NONE', #62860, #26361, #59386, .T. ) ;
#13994=CARTESIAN_POINT ( 'NONE',  ( 14.88232117145529720, 0.5000000000000004441, 1.875237731503240024 ) ) ;
#14003=CARTESIAN_POINT ( 'NONE',  ( -10.36894250292378317, -17.57125116508602503, 10.36894250292379560 ) ) ;
#14012=CARTESIAN_POINT ( 'NONE',  ( -12.34086200392816757, 15.00000000000000000, -7.125000000000143885 ) ) ;
#14014=CARTESIAN_POINT ( 'NONE',  ( -0.9082943533638283551, 15.00000000000000000, 14.47152380945581918 ) ) ;
#14017=CARTESIAN_POINT ( 'NONE',  ( -2.915334737309917656, 24.10535201082151247, 10.88017736071110164 ) ) ;
#14023=ORIENTED_EDGE ( 'NONE', *, *, #98651, .F. ) ;
#14026=CARTESIAN_POINT ( 'NONE',  ( -13.40508947812168827, 15.00000000000000000, 5.527528931045992522 ) ) ;
#14028=AXIS2_PLACEMENT_3D ( 'NONE', #84152, #15658, #46141 ) ;
#14035=CARTESIAN_POINT ( 'NONE',  ( 11.92686044187657224, 9.953790035174483464, 3.195792623639526209 ) ) ;
#14037=EDGE_LOOP ( 'NONE', ( #18427, #52784, #70332, #4044 ) ) ;
#14046=CARTESIAN_POINT ( 'NONE',  ( -14.97653319723434073, 15.00000000000000000, -5.619684139539446122 ) ) ;
#14063=LINE ( 'NONE', #51560, #66782 ) ;
#14066=FACE_OUTER_BOUND ( 'NONE', #83762, .T. ) ;
#14067=CARTESIAN_POINT ( 'NONE',  ( -7.208316651077756099, 16.63393115100079100, 7.208316651077766757 ) ) ;
#14068=EDGE_LOOP ( 'NONE', ( #75499, #37847, #35216, #45589 ) ) ;
#14084=VERTEX_POINT ( 'NONE', #26923 ) ;
#14091=DIRECTION ( 'NONE',  ( -0.8433914458128813907, 0.000000000000000000, -0.5372996083468306594 ) ) ;
#14096=DIRECTION ( 'NONE',  ( 0.9366721892483971246, 0.000000000000000000, 0.3502073812594685975 ) ) ;
#14099=ORIENTED_EDGE ( 'NONE', *, *, #97807, .F. ) ;
#14101=CARTESIAN_POINT ( 'NONE',  ( -9.997910040112678587, 4.195612547371048347E-16, 10.50199004140710812 ) ) ;
#14108=CARTESIAN_POINT ( 'NONE',  ( 6.767445849361252819, 14.49999999999999112, -13.38662304974503492 ) ) ;
#14112=AXIS2_PLACEMENT_3D ( 'NONE', #21290, #34289, #95304 ) ;
#14117=B_SPLINE_CURVE_WITH_KNOTS ( 'NONE', 3,
 ( #81920, #15904, #67421, #32854, #64325, #77368 ),
 .UNSPECIFIED., .F., .F.,
 ( 4, 2, 4 ),
 ( 3.409110551496146276E-05, 0.0004400426677367891737, 0.0008459942299586169050 ),
 .UNSPECIFIED. ) ;
#14118=ORIENTED_EDGE ( 'NONE', *, *, #44340, .T. ) ;
#14127=CARTESIAN_POINT ( 'NONE',  ( -8.813102413619921194, -0.03417435944610275333, -13.34940531570976496 ) ) ;
#14131=CARTESIAN_POINT ( 'NONE',  ( 2.915334737309921209, -8.394647989178491088, -10.88017736071110164 ) ) ;
#14135=CARTESIAN_POINT ( 'NONE',  ( 12.60874940350947959, 4.146618495107105809E-16, -7.160268045227032196 ) ) ;
#14136=DIRECTION ( 'NONE',  ( -0.9723699203976758909, 0.000000000000000000, -0.2334453638559087496 ) ) ;
#14137=B_SPLINE_CURVE_WITH_KNOTS ( 'NONE', 3,
 ( #22011, #14511, #83977, #97034, #37999, #15502 ),
 .UNSPECIFIED., .F., .F.,
 ( 4, 2, 4 ),
 ( 0.0002800039672440436710, 0.0006862092354666161648, 0.001092414503689188550 ),
 .UNSPECIFIED. ) ;
#14148=ORIENTED_EDGE ( 'NONE', *, *, #28799, .F. ) ;
#14150=B_SPLINE_CURVE_WITH_KNOTS ( 'NONE', 3,
 ( #44305, #35324, #43321, #89324, #20832, #29303 ),
 .UNSPECIFIED., .F., .F.,
 ( 4, 2, 4 ),
 ( 0.0002800364959418023825, 0.0006862420824208962733, 0.001092447668899990164 ),
 .UNSPECIFIED. ) ;
#14151=CARTESIAN_POINT ( 'NONE',  ( -13.82671409943291785, -0.03417435944610275333, -3.447387012295409114 ) ) ;
#14157=AXIS2_PLACEMENT_3D ( 'NONE', #96794, #80290, #50781 ) ;
#14164=ORIENTED_EDGE ( 'NONE', *, *, #63561, .T. ) ;
#14180=CARTESIAN_POINT ( 'NONE',  ( -8.527530157486173934, -23.57440218233254470, 4.923371831947302546 ) ) ;
#14182=CARTESIAN_POINT ( 'NONE',  ( 1.460619146402132233E-15, 35.00000000000000000, 11.92686044187656513 ) ) ;
#14197=CARTESIAN_POINT ( 'NONE',  ( 12.81628187352647608, 16.62363466993042849, -2.602085213965210642E-15 ) ) ;
#14207=DIRECTION ( 'NONE',  ( -0.7489557207890037427, 0.000000000000000000, 0.6626200482157358351 ) ) ;
#14214=CARTESIAN_POINT ( 'NONE',  ( 0.000000000000000000, 14.49999999999999822, 0.000000000000000000 ) ) ;
#14215=CARTESIAN_POINT ( 'NONE',  ( 0.000000000000000000, 0.5000000000000004441, 0.000000000000000000 ) ) ;
#14221=VERTEX_POINT ( 'NONE', #6431 ) ;
#14228=CARTESIAN_POINT ( 'NONE',  ( 9.065164099344483972, 0.3639310782753644169, 11.95084933600775301 ) ) ;
#14233=EDGE_CURVE ( 'NONE', #86850, #56243, #87180, .T. ) ;
#14235=CARTESIAN_POINT ( 'NONE',  ( 0.000000000000000000, 15.00000000000000000, 0.000000000000000000 ) ) ;
#14238=CARTESIAN_POINT ( 'NONE',  ( -12.83294900548052730, 15.00000000000000000, -7.766300266068542513 ) ) ;
#14249=CARTESIAN_POINT ( 'NONE',  ( -1.881370533971388870, 15.00000000000000888, 14.50512983964824620 ) ) ;
#14250=CARTESIAN_POINT ( 'NONE',  ( -14.16423886937409726, 17.01208216824730357, 3.795296366450320757 ) ) ;
#14259=B_SPLINE_CURVE_WITH_KNOTS ( 'NONE', 3,
 ( #87322, #35800, #66287, #28298, #20809, #51297 ),
 .UNSPECIFIED., .F., .F.,
 ( 4, 2, 4 ),
 ( 3.409110551496091388E-05, 0.0004400426677367852164, 0.0008459942299586095324 ),
 .UNSPECIFIED. ) ;
#14262=EDGE_CURVE ( 'NONE', #62525, #25445, #65158, .T. ) ;
#14267=CARTESIAN_POINT ( 'NONE',  ( -11.36220558718869711, 4.706058445226104967E-16, 9.008345252845160189 ) ) ;
#14276=CARTESIAN_POINT ( 'NONE',  ( -12.25993886608593897, 0.3640475087720980163, -8.642563219313796452 ) ) ;
#14281=DIRECTION ( 'NONE',  ( 0.000000000000000000, 1.000000000000000000, 0.000000000000000000 ) ) ;
#14285=CARTESIAN_POINT ( 'NONE',  ( 0.000000000000000000, 0.000000000000000000, 0.000000000000000000 ) ) ;
#14287=VECTOR ( 'NONE', #18955, 1000.000000000000114 ) ;
#14302=DIRECTION ( 'NONE',  ( 0.5075383629606904368, 0.000000000000000000, 0.8616291604415338146 ) ) ;
#14320=LINE ( 'NONE', #92277, #72819 ) ;
#14326=CARTESIAN_POINT ( 'NONE',  ( -4.873787042390612001, 0.000000000000000000, -13.39061984619925916 ) ) ;
#14343=VECTOR ( 'NONE', #51819, 1000.000000000000000 ) ;
#14348=ADVANCED_FACE ( 'NONE', ( #42768 ), #73250, .T. ) ;
#14350=ORIENTED_EDGE ( 'NONE', *, *, #62428, .T. ) ;
#14360=CARTESIAN_POINT ( 'NONE',  ( 3.927832320392247389, 15.00000000000000000, -13.69797916712104602 ) ) ;
#14370=EDGE_CURVE ( 'NONE', #18862, #77856, #28583, .T. ) ;
#14372=ORIENTED_EDGE ( 'NONE', *, *, #44400, .F. ) ;
#14373=PLANE ( 'NONE',  #19358 ) ;
#14375=CARTESIAN_POINT ( 'NONE',  ( 11.92686044187655980, 2.396642702460846319, -3.195792623639533314 ) ) ;
#14379=ORIENTED_EDGE ( 'NONE', *, *, #76214, .T. ) ;
#14383=PLANE ( 'NONE',  #83423 ) ;
#14391=CARTESIAN_POINT ( 'NONE',  ( -11.22915323889586858, -0.03417435944610275333, 8.773176023390528044 ) ) ;
#14396=CARTESIAN_POINT ( 'NONE',  ( -13.14228782657345107, 0.5000000000000004441, 7.230509711182143917 ) ) ;
#14414=DIRECTION ( 'NONE',  ( 0.000000000000000000, 1.000000000000000000, 0.000000000000000000 ) ) ;
#14422=AXIS2_PLACEMENT_3D ( 'NONE', #51338, #11367, #34346 ) ;
#14429=VERTEX_POINT ( 'NONE', #4339 ) ;
#14443=CARTESIAN_POINT ( 'NONE',  ( -11.09922568453595382, -21.29303199673624292, -6.408140936763226492 ) ) ;
#14452=B_SPLINE_CURVE_WITH_KNOTS ( 'NONE', 3,
 ( #29207, #44206, #21226, #84207, #51730, #97744 ),
 .UNSPECIFIED., .F., .F.,
 ( 4, 2, 4 ),
 ( 0.0002800630492218076652, 0.0006862688956327564049, 0.001092474742043705090 ),
 .UNSPECIFIED. ) ;
#14453=CARTESIAN_POINT ( 'NONE',  ( -14.37657372141817724, 15.00000000000000888, 2.693041920167245529 ) ) ;
#14459=VERTEX_POINT ( 'NONE', #3845 ) ;
#14471=VECTOR ( 'NONE', #83756, 1000.000000000000000 ) ;
#14474=DIRECTION ( 'NONE',  ( -0.000000000000000000, -1.000000000000000000, -0.000000000000000000 ) ) ;
#14489=CARTESIAN_POINT ( 'NONE',  ( -3.897244926436033374, 15.00000000000000000, -13.96644127841335958 ) ) ;
#14501=CARTESIAN_POINT ( 'NONE',  ( -5.204170427930421283E-15, -14.44625116508602858, -14.16423886937410082 ) ) ;
#14505=VERTEX_POINT ( 'NONE', #30264 ) ;
#14506=LINE ( 'NONE', #74489, #77903 ) ;
#14508=CARTESIAN_POINT ( 'NONE',  ( -0.9940297508535884674, 15.00000000000000000, -14.21528771620250886 ) ) ;
#14511=CARTESIAN_POINT ( 'NONE',  ( 2.888814634336697829, 15.00000000000000711, 14.33747749179070752 ) ) ;
#14516=CARTESIAN_POINT ( 'NONE',  ( 7.964842623401181321, 29.93868534415484461, 7.964842623401174215 ) ) ;
#14522=ORIENTED_EDGE ( 'NONE', *, *, #90421, .F. ) ;
#14526=FACE_OUTER_BOUND ( 'NONE', #14613, .T. ) ;
#14546=CARTESIAN_POINT ( 'NONE',  ( 0.000000000000000000, 1.823139558123437975, 0.000000000000000000 ) ) ;
#14551=ORIENTED_EDGE ( 'NONE', *, *, #79762, .T. ) ;
#14556=CARTESIAN_POINT ( 'NONE',  ( 0.000000000000000000, 12.49999999999999112, 0.000000000000000000 ) ) ;
#14561=FACE_OUTER_BOUND ( 'NONE', #11692, .T. ) ;
#14564=AXIS2_PLACEMENT_3D ( 'NONE', #2411, #55884, #2902 ) ;
#14566=CARTESIAN_POINT ( 'NONE',  ( 4.923371831947301658, 17.67559781766744820, 8.527530157486175710 ) ) ;
#14580=ORIENTED_EDGE ( 'NONE', *, *, #37493, .T. ) ;
#14583=VERTEX_POINT ( 'NONE', #79218 ) ;
#14591=VECTOR ( 'NONE', #60843, 1000.000000000000114 ) ;
#14592=AXIS2_PLACEMENT_3D ( 'NONE', #69454, #84462, #6988 ) ;
#14594=LINE ( 'NONE', #83074, #20032 ) ;
#14595=B_SPLINE_CURVE_WITH_KNOTS ( 'NONE', 3,
 ( #98507, #83961, #45970, #77428, #8940, #4 ),
 .UNSPECIFIED., .F., .F.,
 ( 4, 2, 4 ),
 ( 0.0002800421825936745958, 0.0006862478247299499869, 0.001092453466866225541 ),
 .UNSPECIFIED. ) ;
#14599=AXIS2_PLACEMENT_3D ( 'NONE', #51506, #74494, #22503 ) ;
#14602=DIRECTION ( 'NONE',  ( 0.000000000000000000, 0.000000000000000000, 1.000000000000000000 ) ) ;
#14603=B_SPLINE_CURVE_WITH_KNOTS ( 'NONE', 3,
 ( #30729, #14276, #13269, #90744, #67265, #45753 ),
 .UNSPECIFIED., .F., .F.,
 ( 4, 2, 4 ),
 ( 3.409110551496050731E-05, 0.0004400426677367859753, 0.0008459942299586113755 ),
 .UNSPECIFIED. ) ;
#14613=EDGE_LOOP ( 'NONE', ( #38153, #53182, #97519, #57704, #48297, #3714 ) ) ;
#14620=DIRECTION ( 'NONE',  ( 0.000000000000000000, 1.000000000000000000, 0.000000000000000000 ) ) ;
#14622=DIRECTION ( 'NONE',  ( -0.000000000000000000, -1.000000000000000000, -0.000000000000000000 ) ) ;
#14623=VECTOR ( 'NONE', #83009, 1000.000000000000227 ) ;
#14624=ORIENTED_EDGE ( 'NONE', *, *, #29685, .F. ) ;
#14625=ORIENTED_EDGE ( 'NONE', *, *, #91225, .F. ) ;
#14633=EDGE_CURVE ( 'NONE', #97319, #89788, #73180, .T. ) ;
#14638=CARTESIAN_POINT ( 'NONE',  ( 9.422509992056141925, -14.01964798917848576, -5.440088680355554374 ) ) ;
#14640=CARTESIAN_POINT ( 'NONE',  ( 3.927832320392247389, -0.03417435944610275333, -13.69797916712104602 ) ) ;
#14643=CARTESIAN_POINT ( 'NONE',  ( 0.7375392941518293943, 14.49999999999999822, -14.98185688723470932 ) ) ;
#14645=CARTESIAN_POINT ( 'NONE',  ( -0.1552420861355162940, 14.99999999999805489, 14.62478754979945705 ) ) ;
#14655=CARTESIAN_POINT ( 'NONE',  ( 0.000000000000000000, 15.00000000000000000, 0.000000000000000000 ) ) ;
#14663=CIRCLE ( 'NONE', #1897, 15.00000000000000000 ) ;
#14664=ORIENTED_EDGE ( 'NONE', *, *, #79282, .F. ) ;
#14665=LINE ( 'NONE', #28654, #84859 ) ;
#14667=VERTEX_POINT ( 'NONE', #19700 ) ;
#14683=CARTESIAN_POINT ( 'NONE',  ( -9.846743663894596210, -19.19940218233254114, -2.638427012816824124 ) ) ;
#14684=ORIENTED_EDGE ( 'NONE', *, *, #92676, .F. ) ;
#14688=DIRECTION ( 'NONE',  ( 0.000000000000000000, 0.000000000000000000, 1.000000000000000000 ) ) ;
#14690=DIRECTION ( 'NONE',  ( 0.000000000000000000, 1.000000000000000000, 0.000000000000000000 ) ) ;
#14696=EDGE_CURVE ( 'NONE', #7648, #43985, #58914, .T. ) ;
#14699=CARTESIAN_POINT ( 'NONE',  ( 3.434112377981054287, 17.66530133659708568, -12.81628187352647608 ) ) ;
#14709=DIRECTION ( 'NONE',  ( 0.9935718556765863463, 0.000000000000000000, 0.1132032137679171435 ) ) ;
#14713=ORIENTED_EDGE ( 'NONE', *, *, #31526, .T. ) ;
#14715=CARTESIAN_POINT ( 'NONE',  ( -3.115783986955657614, 15.00000000000000000, 14.16128137375395468 ) ) ;
#14716=LINE ( 'NONE', #45191, #64177 ) ;
#14718=EDGE_LOOP ( 'NONE', ( #12, #40130, #88494, #24667 ) ) ;
#14723=ADVANCED_FACE ( 'NONE', ( #56716 ), #17167, .F. ) ;
#14726=DIRECTION ( 'NONE',  ( 4.440892098500626162E-15, 0.000000000000000000, 1.000000000000000000 ) ) ;
#14730=CARTESIAN_POINT ( 'NONE',  ( 7.313705784284593392, 0.5000000000000004441, -13.09617149020743732 ) ) ;
#14731=CARTESIAN_POINT ( 'NONE',  ( -6.689969769699040114, -0.03417435944610275333, 12.58200319823965785 ) ) ;
#14739=B_SPLINE_CURVE_WITH_KNOTS ( 'NONE', 3,
 ( #55337, #84381, #23881, #38875, #30862, #1873 ),
 .UNSPECIFIED., .F., .F.,
 ( 4, 2, 4 ),
 ( 0.0002800808511812530191, 0.0006862868719358964590, 0.001092492892690540007 ),
 .UNSPECIFIED. ) ;
#14741=EDGE_CURVE ( 'NONE', #29043, #15233, #22928, .T. ) ;
#14742=ORIENTED_EDGE ( 'NONE', *, *, #42281, .F. ) ;
#14747=DIRECTION ( 'NONE',  ( -0.000000000000000000, -1.000000000000000000, -0.000000000000000000 ) ) ;
#14749=B_SPLINE_CURVE_WITH_KNOTS ( 'NONE', 3,
 ( #18372, #79847, #11842, #64825, #25395, #71858 ),
 .UNSPECIFIED., .F., .F.,
 ( 4, 2, 4 ),
 ( 0.0002800206007755498788, 0.0006862260317144059079, 0.001092431462653262100 ),
 .UNSPECIFIED. ) ;
#14754=CARTESIAN_POINT ( 'NONE',  ( 3.795296366450306547, 15.34541550158064460, -14.16423886937410259 ) ) ;
#14756=B_SPLINE_CURVE_WITH_KNOTS ( 'NONE', 3,
 ( #97760, #29716, #98258, #53705, #75222, #8698 ),
 .UNSPECIFIED., .F., .F.,
 ( 4, 2, 4 ),
 ( 0.0002800912045164338977, 0.0006862973266905296552, 0.001092503448864625250 ),
 .UNSPECIFIED. ) ;
#14758=CARTESIAN_POINT ( 'NONE',  ( 3.115783986955557694, 15.00000000000000000, -14.16128137375397955 ) ) ;
#14768=DIRECTION ( 'NONE',  ( 0.000000000000000000, 1.000000000000000000, 0.000000000000000000 ) ) ;
#14777=CARTESIAN_POINT ( 'NONE',  ( -14.48718990079892954, 4.238615592650390652E-16, 0.6093675230839495915 ) ) ;
#14782=CARTESIAN_POINT ( 'NONE',  ( 8.564643372776536978, 0.5000000000000004441, 12.31449893000746343 ) ) ;
#14783=B_SPLINE_CURVE_WITH_KNOTS ( 'NONE', 3,
 ( #69947, #94407, #56423, #77426, #62421, #92925 ),
 .UNSPECIFIED., .F., .F.,
 ( 4, 2, 4 ),
 ( 0.0002800047503720886136, 0.0006862100262544192433, 0.001092415302136749873 ),
 .UNSPECIFIED. ) ;
#14793=CARTESIAN_POINT ( 'NONE',  ( 3.469446951953614189E-15, 4.171802177851546389, 11.25000000000000355 ) ) ;
#14798=CARTESIAN_POINT ( 'NONE',  ( -8.209432707284950226, 0.5000000000000004441, 12.55409154915480485 ) ) ;
#14799=DIRECTION ( 'NONE',  ( 0.000000000000000000, 0.000000000000000000, 1.000000000000000000 ) ) ;
#14800=B_SPLINE_CURVE_WITH_KNOTS ( 'NONE', 3,
 ( #11111, #33111, #32119, #3133, #85637, #62616 ),
 .UNSPECIFIED., .F., .F.,
 ( 4, 2, 4 ),
 ( 0.0002800715030460627138, 0.0006862774322447868407, 0.001092483361443510968 ),
 .UNSPECIFIED. ) ;
#14809=VERTEX_POINT ( 'NONE', #51769 ) ;
#14823=ORIENTED_EDGE ( 'NONE', *, *, #6586, .F. ) ;
#14827=LINE ( 'NONE', #53292, #1587 ) ;
#14831=EDGE_LOOP ( 'NONE', ( #60474, #5384, #19440, #34341 ) ) ;
#14832=ADVANCED_FACE ( 'NONE', ( #29741 ), #51271, .F. ) ;
#14836=EDGE_CURVE ( 'NONE', #6506, #73794, #14603, .T. ) ;
#14848=CARTESIAN_POINT ( 'NONE',  ( 14.94699059465102309, 0.3640475087720504432, -1.259949270174814284 ) ) ;
#14862=DIRECTION ( 'NONE',  ( -0.1650476058606810958, 0.000000000000000000, 0.9862856015372308827 ) ) ;
#14870=EDGE_CURVE ( 'NONE', #40514, #20839, #7614, .T. ) ;
#14875=ADVANCED_FACE ( 'NONE', ( #74250 ), #20366, .T. ) ;
#14881=DIRECTION ( 'NONE',  ( -0.000000000000000000, -1.000000000000000000, -0.000000000000000000 ) ) ;
#14885=DIRECTION ( 'NONE',  ( -0.000000000000000000, -1.000000000000000000, -0.000000000000000000 ) ) ;
#14893=CARTESIAN_POINT ( 'NONE',  ( -14.99847009497944406, 0.5000000000000004441, -0.2142307401082361173 ) ) ;
#14897=DIRECTION ( 'NONE',  ( -0.000000000000000000, -1.000000000000000000, -0.000000000000000000 ) ) ;
#14921=VERTEX_POINT ( 'NONE', #14777 ) ;
#14922=AXIS2_PLACEMENT_3D ( 'NONE', #5557, #66536, #90507 ) ;
#14929=VERTEX_POINT ( 'NONE', #52258 ) ;
#14937=CARTESIAN_POINT ( 'NONE',  ( 3.115783986955448892, 15.00000000000000000, 14.16128137375397600 ) ) ;
#14939=VERTEX_POINT ( 'NONE', #20780 ) ;
#14941=CARTESIAN_POINT ( 'NONE',  ( -11.09922568453594316, -15.45969866340291077, 6.408140936763246920 ) ) ;
#14951=VECTOR ( 'NONE', #89463, 1000.000000000000114 ) ;
#14953=CARTESIAN_POINT ( 'NONE',  ( -9.876730923139175999, 0.3639310091266617642, -11.28938378619078264 ) ) ;
#14958=ADVANCED_FACE ( 'NONE', ( #91239 ), #89026, .T. ) ;
#14959=ORIENTED_EDGE ( 'NONE', *, *, #71380, .F. ) ;
#14965=CARTESIAN_POINT ( 'NONE',  ( 13.61464873478162829, 14.49999999999999822, 6.296136897217933459 ) ) ;
#14969=CARTESIAN_POINT ( 'NONE',  ( 11.96291822454875842, 4.834832779786913688E-16, 8.193813980849165901 ) ) ;
#14973=LINE ( 'NONE', #40913, #91681 ) ;
#14984=CARTESIAN_POINT ( 'NONE',  ( -2.888814634336603238, 15.00000000000000178, -14.33747749179072883 ) ) ;
#14993=CARTESIAN_POINT ( 'NONE',  ( -9.876730923139204421, 14.49999999999999112, -11.28938378619079863 ) ) ;
#14997=CARTESIAN_POINT ( 'NONE',  ( 3.795296366450306547, -24.65458449841936428, -14.16423886937410259 ) ) ;
#15004=DIRECTION ( 'NONE',  ( 0.000000000000000000, 1.000000000000000000, 0.000000000000000000 ) ) ;
#15007=CARTESIAN_POINT ( 'NONE',  ( -3.836325488035982278, 14.49999999999999112, -14.50112432709434351 ) ) ;
#15009=LINE ( 'NONE', #45479, #82110 ) ;
#15013=CARTESIAN_POINT ( 'NONE',  ( 9.422509992056141925, 30.14701867748817321, 5.440088680355547268 ) ) ;
#15019=ORIENTED_EDGE ( 'NONE', *, *, #24095, .T. ) ;
#15031=ORIENTED_EDGE ( 'NONE', *, *, #7055, .T. ) ;
#15044=EDGE_CURVE ( 'NONE', #92547, #14921, #53844, .T. ) ;
#15054=CARTESIAN_POINT ( 'NONE',  ( 3.836325488036075981, 14.49999999999999112, 14.50112432709431687 ) ) ;
#15059=ADVANCED_FACE ( 'NONE', ( #77221 ), #44267, .T. ) ;
#15061=CARTESIAN_POINT ( 'NONE',  ( -4.020549461440751315, 0.000000000000000000, 3.684154808197060316 ) ) ;
#15064=B_SPLINE_CURVE_WITH_KNOTS ( 'NONE', 3,
 ( #84651, #40633, #10138, #93620, #54623, #55118 ),
 .UNSPECIFIED., .F., .F.,
 ( 4, 2, 4 ),
 ( 3.409110551494654820E-05, 0.0004400426677367934021, 0.0008459942299586403237 ),
 .UNSPECIFIED. ) ;
#15065=LINE ( 'NONE', #92999, #86529 ) ;
#15066=CARTESIAN_POINT ( 'NONE',  ( -2.638427012816840111, 14.96726448433411605, -9.846743663894590881 ) ) ;
#15080=VERTEX_POINT ( 'NONE', #71212 ) ;
#15083=ORIENTED_EDGE ( 'NONE', *, *, #64565, .T. ) ;
#15084=EDGE_CURVE ( 'NONE', #97132, #16779, #1507, .T. ) ;
#15096=PLANE ( 'NONE',  #55435 ) ;
#15103=ORIENTED_EDGE ( 'NONE', *, *, #19629, .F. ) ;
#15104=PLANE ( 'NONE',  #1759 ) ;
#15112=VECTOR ( 'NONE', #87984, 1000.000000000000114 ) ;
#15113=ORIENTED_EDGE ( 'NONE', *, *, #29705, .T. ) ;
#15127=CARTESIAN_POINT ( 'NONE',  ( -9.422509992056145478, -7.352981322511817019, -5.440088680355541939 ) ) ;
#15131=CARTESIAN_POINT ( 'NONE',  ( 14.48718990079892066, 4.852832169489322230E-16, 0.6093675230841453239 ) ) ;
#15154=VECTOR ( 'NONE', #92253, 999.9999999999998863 ) ;
#15157=ORIENTED_EDGE ( 'NONE', *, *, #2782, .T. ) ;
#15174=CARTESIAN_POINT ( 'NONE',  ( 9.846743663894590881, -21.28273551566588395, -2.638427012816833894 ) ) ;
#15180=EDGE_LOOP ( 'NONE', ( #78896, #4154, #35824, #1052 ) ) ;
#15181=DIRECTION ( 'NONE',  ( -0.9762960071199346945, 0.000000000000000000, 0.2164396139380971307 ) ) ;
#15187=CARTESIAN_POINT ( 'NONE',  ( -12.81628187352647608, 24.12363466993042138, 3.903127820947815962E-15 ) ) ;
#15203=CARTESIAN_POINT ( 'NONE',  ( 12.98685442714775640, 15.00000000000000000, 6.449155920607609893 ) ) ;
#15205=VECTOR ( 'NONE', #20483, 1000.000000000000000 ) ;
#15208=CARTESIAN_POINT ( 'NONE',  ( -8.721827932831688557, -2.980708941387882104E-15, -11.74045266257187592 ) ) ;
#15209=ORIENTED_EDGE ( 'NONE', *, *, #66706, .T. ) ;
#15215=CARTESIAN_POINT ( 'NONE',  ( 0.000000000000000000, 0.5000000000000004441, 0.000000000000000000 ) ) ;
#15216=ORIENTED_EDGE ( 'NONE', *, *, #53671, .T. ) ;
#15217=CARTESIAN_POINT ( 'NONE',  ( 0.000000000000000000, 15.00000000000000000, 0.000000000000000000 ) ) ;
#15222=DIRECTION ( 'NONE',  ( -0.7604059656000257128, 0.000000000000000000, -0.6494480483301898754 ) ) ;
#15225=TOROIDAL_SURFACE ( 'NONE', #82287, 14.49999999999999822, 0.5000000000000000000 ) ;
#15231=AXIS2_PLACEMENT_3D ( 'NONE', #13761, #20277, #90240 ) ;
#15233=VERTEX_POINT ( 'NONE', #63586 ) ;
#15234=CARTESIAN_POINT ( 'NONE',  ( 0.000000000000000000, 14.49999999999999822, 0.000000000000000000 ) ) ;
#15238=DIRECTION ( 'NONE',  ( 0.3826834323650877834, -0.000000000000000000, 0.9238795325112876267 ) ) ;
#15239=B_SPLINE_CURVE_WITH_KNOTS ( 'NONE', 3,
 ( #1854, #47811, #78311, #57280, #72279, #11292 ),
 .UNSPECIFIED., .F., .F.,
 ( 4, 2, 4 ),
 ( 3.409110551496119171E-05, 0.0004400426677367866800, 0.0008459942299586122429 ),
 .UNSPECIFIED. ) ;
#15240=LINE ( 'NONE', #23728, #23624 ) ;
#15246=EDGE_CURVE ( 'NONE', #50110, #51389, #17623, .T. ) ;
#15247=VECTOR ( 'NONE', #57980, 1000.000000000000114 ) ;
#15249=CARTESIAN_POINT ( 'NONE',  ( -1.780824192092602010, 14.63595249122789177, 14.89391369643512952 ) ) ;
#15250=CARTESIAN_POINT ( 'NONE',  ( -12.26659068614894110, 17.22041550158065348, 7.082119434687058401 ) ) ;
#15253=DIRECTION ( 'NONE',  ( -0.9099612708765455471, 0.000000000000000000, 0.4146932426562339180 ) ) ;
#15254=EDGE_CURVE ( 'NONE', #4847, #54861, #34763, .T. ) ;
#15263=DIRECTION ( 'NONE',  ( -0.000000000000000000, -1.000000000000000000, -0.000000000000000000 ) ) ;
#15265=VECTOR ( 'NONE', #45487, 1000.000000000000000 ) ;
#15269=ORIENTED_EDGE ( 'NONE', *, *, #84673, .F. ) ;
#15275=CARTESIAN_POINT ( 'NONE',  ( -11.96291822454887033, 4.341775326899288507E-16, 8.193813980848993594 ) ) ;
#15283=EDGE_CURVE ( 'NONE', #56877, #59079, #90662, .T. ) ;
#15285=VERTEX_POINT ( 'NONE', #64069 ) ;
#15287=AXIS2_PLACEMENT_3D ( 'NONE', #55685, #92688, #71668 ) ;
#15302=ORIENTED_EDGE ( 'NONE', *, *, #33284, .T. ) ;
#15304=ORIENTED_EDGE ( 'NONE', *, *, #76212, .F. ) ;
#15308=CARTESIAN_POINT ( 'NONE',  ( 7.109031286574768238, 0.04962885628204084798, 12.92745085449643128 ) ) ;
#15316=ORIENTED_EDGE ( 'NONE', *, *, #94125, .F. ) ;
#15318=VERTEX_POINT ( 'NONE', #73546 ) ;
#15328=VERTEX_POINT ( 'NONE', #56595 ) ;
#15337=LINE ( 'NONE', #38320, #47943 ) ;
#15352=DIRECTION ( 'NONE',  ( 0.9990482215818582423, 0.000000000000000000, -0.04361938736532634114 ) ) ;
#15353=VECTOR ( 'NONE', #28623, 999.9999999999998863 ) ;
#15357=ORIENTED_EDGE ( 'NONE', *, *, #20916, .T. ) ;
#15362=CARTESIAN_POINT ( 'NONE',  ( 11.22915323889574601, 0.000000000000000000, 8.773176023390684364 ) ) ;
#15367=VECTOR ( 'NONE', #1619, 1000.000000000000000 ) ;
#15368=CARTESIAN_POINT ( 'NONE',  ( 6.761335002693093621, 0.2301500669213601691, -13.32315948060037059 ) ) ;
#15369=ADVANCED_FACE ( 'NONE', ( #35559 ), #86603, .F. ) ;
#15375=VERTEX_POINT ( 'NONE', #73056 ) ;
#15384=ORIENTED_EDGE ( 'NONE', *, *, #72713, .F. ) ;
#15386=CARTESIAN_POINT ( 'NONE',  ( 11.62112565934141095, 15.00000000000000711, 8.881879596174812264 ) ) ;
#15391=DIRECTION ( 'NONE',  ( -0.8526401643540953978, 0.000000000000000000, 0.5224985647159435809 ) ) ;
#15392=DIRECTION ( 'NONE',  ( -0.000000000000000000, -1.000000000000000000, -0.000000000000000000 ) ) ;
#15400=B_SPLINE_CURVE_WITH_KNOTS ( 'NONE', 3,
 ( #3926, #95411, #11911, #27395, #56911, #18929 ),
 .UNSPECIFIED., .F., .F.,
 ( 4, 2, 4 ),
 ( 3.409110551494637202E-05, 0.0004400426677367945405, 0.0008459942299586427090 ),
 .UNSPECIFIED. ) ;
#15413=EDGE_CURVE ( 'NONE', #17506, #21360, #79467, .T. ) ;
#15415=DIRECTION ( 'NONE',  ( 0.1650476058606878405, 0.000000000000000000, -0.9862856015372296614 ) ) ;
#15427=PLANE ( 'NONE',  #76045 ) ;
#15429=ORIENTED_EDGE ( 'NONE', *, *, #48758, .T. ) ;
#15440=CARTESIAN_POINT ( 'NONE',  ( -9.382169495545413795, -0.2513653300695748993, 9.382169495545428006 ) ) ;
#15444=CARTESIAN_POINT ( 'NONE',  ( -14.88232117145534517, 14.49999999999999112, -1.875237731503371030 ) ) ;
#15452=VERTEX_POINT ( 'NONE', #4093 ) ;
#15456=ORIENTED_EDGE ( 'NONE', *, *, #60444, .T. ) ;
#15465=CARTESIAN_POINT ( 'NONE',  ( -7.882504294823764468, 15.00000000000000888, -12.32089577884801379 ) ) ;
#15469=VERTEX_POINT ( 'NONE', #3604 ) ;
#15481=CARTESIAN_POINT ( 'NONE',  ( 3.469446951953614189E-15, 11.36803362898265135, 11.25000000000000178 ) ) ;
#15485=DIRECTION ( 'NONE',  ( -0.8433914458128884961, 0.000000000000000000, 0.5372996083468194461 ) ) ;
#15490=CARTESIAN_POINT ( 'NONE',  ( 12.26659068614894821, -1.112917831752692432, 7.082119434687044190 ) ) ;
#15491=CIRCLE ( 'NONE', #12323, 14.49999999999999822 ) ;
#15502=CARTESIAN_POINT ( 'NONE',  ( 2.815433093577012880, 14.49999999999999112, 14.73340885523758281 ) ) ;
#15508=CARTESIAN_POINT ( 'NONE',  ( 3.469446951953614189E-15, 29.31368534415484817, 10.88017736071110342 ) ) ;
#15514=DIRECTION ( 'NONE',  ( 0.000000000000000000, 0.000000000000000000, 1.000000000000000000 ) ) ;
#15518=CARTESIAN_POINT ( 'NONE',  ( -13.78891971893213331, 14.63595249122791842, 5.904717858191443014 ) ) ;
#15519=ADVANCED_FACE ( 'NONE', ( #87573 ), #64560, .F. ) ;
#15525=CARTESIAN_POINT ( 'NONE',  ( 0.000000000000000000, 15.00000000000000000, -14.25000000000000000 ) ) ;
#15534=DIRECTION ( 'NONE',  ( -1.776356839400250465E-15, 0.000000000000000000, 1.000000000000000000 ) ) ;
#15552=VECTOR ( 'NONE', #87123, 1000.000000000000000 ) ;
#15556=CARTESIAN_POINT ( 'NONE',  ( -8.527530157486173934, 26.42559781766745530, 4.923371831947302546 ) ) ;
#15568=AXIS2_PLACEMENT_3D ( 'NONE', #96871, #13346, #30183 ) ;
#15571=ORIENTED_EDGE ( 'NONE', *, *, #4880, .F. ) ;
#15574=EDGE_LOOP ( 'NONE', ( #58874, #93353, #72209, #86364 ) ) ;
#15577=ORIENTED_EDGE ( 'NONE', *, *, #20131, .T. ) ;
#15586=VERTEX_POINT ( 'NONE', #20567 ) ;
#15600=EDGE_CURVE ( 'NONE', #16779, #18519, #39581, .T. ) ;
#15606=EDGE_CURVE ( 'NONE', #5928, #70551, #83760, .T. ) ;
#15607=B_SPLINE_CURVE_WITH_KNOTS ( 'NONE', 3,
 ( #43219, #66720, #12724, #27229, #96743, #67217 ),
 .UNSPECIFIED., .F., .F.,
 ( 4, 2, 4 ),
 ( 3.409110551496041244E-05, 0.0004400426677367855958, 0.0008459942299586108334 ),
 .UNSPECIFIED. ) ;
#15621=CARTESIAN_POINT ( 'NONE',  ( 7.964842623401181321, -10.06131465584515716, 7.964842623401174215 ) ) ;
#15627=FACE_OUTER_BOUND ( 'NONE', #48697, .T. ) ;
#15633=CARTESIAN_POINT ( 'NONE',  ( -7.313705784284419309, 0.5000000000000004441, -13.09617149020753502 ) ) ;
#15650=CARTESIAN_POINT ( 'NONE',  ( 5.810213597521796558, 0.04962897357397456216, -13.56092647078870606 ) ) ;
#15658=DIRECTION ( 'NONE',  ( -0.000000000000000000, -1.000000000000000000, -0.000000000000000000 ) ) ;
#15668=CARTESIAN_POINT ( 'NONE',  ( -9.846743663894594434, -28.99106884899921255, 3.469446951953614189E-15 ) ) ;
#15672=CARTESIAN_POINT ( 'NONE',  ( -7.313705784284471711, 14.49999999999999112, -13.09617149020757942 ) ) ;
#15674=CARTESIAN_POINT ( 'NONE',  ( -12.25993886608615568, 14.49999999999999112, 8.642563219313586842 ) ) ;
#15683=CARTESIAN_POINT ( 'NONE',  ( -3.434112377981047626, 20.16530133659709634, 12.81628187352647963 ) ) ;
#15687=ORIENTED_EDGE ( 'NONE', *, *, #66846, .T. ) ;
#15699=CARTESIAN_POINT ( 'NONE',  ( -5.204170427930421283E-15, 3.438309369127513726, -11.92686044187656513 ) ) ;
#15705=DIRECTION ( 'NONE',  ( 0.000000000000000000, 1.000000000000000000, 0.000000000000000000 ) ) ;
#15708=EDGE_LOOP ( 'NONE', ( #28578, #8997, #20589, #12760, #46420, #17894 ) ) ;
#15709=CARTESIAN_POINT ( 'NONE',  ( 14.04391541078765471, 3.833537969851530006E-16, -3.608107528142839637 ) ) ;
#15710=CARTESIAN_POINT ( 'NONE',  ( -8.606322355891181886, 15.00000000000000000, -11.66967075398817322 ) ) ;
#15714=DIRECTION ( 'NONE',  ( 0.000000000000000000, 0.000000000000000000, 1.000000000000000000 ) ) ;
#15716=B_SPLINE_CURVE_WITH_KNOTS ( 'NONE', 3,
 ( #8906, #63380, #23932, #54401, #39422, #25412 ),
 .UNSPECIFIED., .F., .F.,
 ( 4, 2, 4 ),
 ( 0.0002800484630364014570, 0.0006862541666483245543, 0.001092459870260247814 ),
 .UNSPECIFIED. ) ;
#15727=ADVANCED_FACE ( 'NONE', ( #58548 ), #98703, .F. ) ;
#15729=CARTESIAN_POINT ( 'NONE',  ( 6.767445849361155119, 0.3640475087720991820, 13.38662304974502071 ) ) ;
#15738=FACE_OUTER_BOUND ( 'NONE', #75596, .T. ) ;
#15739=CARTESIAN_POINT ( 'NONE',  ( 12.26659068614894821, 13.88708216824730712, 7.082119434687044190 ) ) ;
#15769=ORIENTED_EDGE ( 'NONE', *, *, #17550, .F. ) ;
#15771=CARTESIAN_POINT ( 'NONE',  ( 5.624999999999998224, 6.255135511184880315, -9.742785792574936821 ) ) ;
#15780=DIRECTION ( 'NONE',  ( 0.000000000000000000, 0.000000000000000000, 1.000000000000000000 ) ) ;
#15789=VERTEX_POINT ( 'NONE', #51052 ) ;
#15794=ORIENTED_EDGE ( 'NONE', *, *, #17316, .F. ) ;
#15805=B_SPLINE_CURVE_WITH_KNOTS ( 'NONE', 3,
 ( #7002, #53469, #82498, #59985, #37006, #90478 ),
 .UNSPECIFIED., .F., .F.,
 ( 4, 2, 4 ),
 ( 3.409110551494641268E-05, 0.0004400426677367923721, 0.0008459942299586382638 ),
 .UNSPECIFIED. ) ;
#15810=EDGE_CURVE ( 'NONE', #48181, #92979, #10963, .T. ) ;
#15814=CARTESIAN_POINT ( 'NONE',  ( 0.000000000000000000, 0.5000000000000004441, 0.000000000000000000 ) ) ;
#15818=VECTOR ( 'NONE', #20191, 1000.000000000000000 ) ;
#15833=AXIS2_PLACEMENT_3D ( 'NONE', #77163, #61654, #93642 ) ;
#15856=LINE ( 'NONE', #38850, #46477 ) ;
#15860=PLANE ( 'NONE',  #46655 ) ;
#15861=CARTESIAN_POINT ( 'NONE',  ( 12.60874940350940321, 15.00000000000000000, 7.160268045227115685 ) ) ;
#15875=CARTESIAN_POINT ( 'NONE',  ( -14.99847009497945116, 14.63595249122789177, -0.2142307401082309548 ) ) ;
#15876=AXIS2_PLACEMENT_3D ( 'NONE', #50545, #11074, #19556 ) ;
#15881=CARTESIAN_POINT ( 'NONE',  ( 5.056330833737696651, 15.00000000000000000, -13.58983143751348521 ) ) ;
#15882=DIRECTION ( 'NONE',  ( 0.000000000000000000, 0.000000000000000000, -1.000000000000000000 ) ) ;
#15896=EDGE_LOOP ( 'NONE', ( #93097, #92273, #15316, #45080 ) ) ;
#15903=CARTESIAN_POINT ( 'NONE',  ( -15.96747533562963994, -0.03417435944610275333, 0.9576679184939570488 ) ) ;
#15904=CARTESIAN_POINT ( 'NONE',  ( 14.82269085861169167, 0.3640475087720976832, -2.299529454046960630 ) ) ;
#15908=CARTESIAN_POINT ( 'NONE',  ( -14.29484424893248473, 14.76984993772165744, 4.345072767107034828 ) ) ;
#15921=EDGE_CURVE ( 'NONE', #19669, #37030, #34745, .T. ) ;
#15923=CYLINDRICAL_SURFACE ( 'NONE', #78670, 15.00000000000000000 ) ;
#15924=VERTEX_POINT ( 'NONE', #77490 ) ;
#15933=CARTESIAN_POINT ( 'NONE',  ( -14.02068044289371684, 0.5000000000000004441, -5.331089937175857330 ) ) ;
#15938=CARTESIAN_POINT ( 'NONE',  ( -7.993154516100878126, 14.95077488074853456, -12.39982181464625022 ) ) ;
#15941=ORIENTED_EDGE ( 'NONE', *, *, #57670, .F. ) ;
#15946=EDGE_CURVE ( 'NONE', #16892, #95455, #67, .T. ) ;
#15955=CARTESIAN_POINT ( 'NONE',  ( -3.270119481323782828, 0.04922511925147937673, 14.38584091150419653 ) ) ;
#15958=FACE_OUTER_BOUND ( 'NONE', #30140, .T. ) ;
#15963=CARTESIAN_POINT ( 'NONE',  ( 12.26659068614894466, -0.2795844984193537885, -7.082119434687053960 ) ) ;
#15967=VERTEX_POINT ( 'NONE', #47977 ) ;
#15973=DIRECTION ( 'NONE',  ( 0.6883545756937550220, 0.000000000000000000, 0.7253743710122867450 ) ) ;
#15980=CYLINDRICAL_SURFACE ( 'NONE', #47047, 15.00000000000000000 ) ;
#15982=CARTESIAN_POINT ( 'NONE',  ( 6.382347221874473675, 14.49999999999999112, -13.57444820018232079 ) ) ;
#16012=ORIENTED_EDGE ( 'NONE', *, *, #58593, .T. ) ;
#16013=ORIENTED_EDGE ( 'NONE', *, *, #46442, .F. ) ;
#16025=B_SPLINE_CURVE_WITH_KNOTS ( 'NONE', 3,
 ( #90160, #190, #68177, #98696, #45661, #21690 ),
 .UNSPECIFIED., .F., .F.,
 ( 4, 2, 4 ),
 ( 0.0002800124554034236863, 0.0006862178066545029931, 0.001092423157905582191 ),
 .UNSPECIFIED. ) ;
#16028=CARTESIAN_POINT ( 'NONE',  ( 8.722765153436254693, 15.00000000000000888, 11.74102699209690392 ) ) ;
#16029=CARTESIAN_POINT ( 'NONE',  ( -6.408140936763246032, -41.70969866340291077, -11.09922568453594316 ) ) ;
#16039=EDGE_CURVE ( 'NONE', #8246, #4144, #72904, .T. ) ;
#16040=VECTOR ( 'NONE', #41709, 1000.000000000000000 ) ;
#16045=ORIENTED_EDGE ( 'NONE', *, *, #82737, .F. ) ;
#16046=AXIS2_PLACEMENT_3D ( 'NONE', #97913, #89882, #36896 ) ;
#16062=VERTEX_POINT ( 'NONE', #64933 ) ;
#16073=VERTEX_POINT ( 'NONE', #27442 ) ;
#16075=VECTOR ( 'NONE', #16091, 1000.000000000000114 ) ;
#16083=VERTEX_POINT ( 'NONE', #33943 ) ;
#16091=DIRECTION ( 'NONE',  ( 0.8038568606172243891, 0.000000000000000000, -0.5948227867513316003 ) ) ;
#16093=CARTESIAN_POINT ( 'NONE',  ( -0.9940297508535884674, -0.03417435944610275333, -14.21528771620250886 ) ) ;
#16097=CARTESIAN_POINT ( 'NONE',  ( 2.915334737309921209, -3.394647989178489311, -10.88017736071110164 ) ) ;
#16103=CARTESIAN_POINT ( 'NONE',  ( -14.22792531055116783, -3.140798168418944474E-15, -3.387425595041295256 ) ) ;
#16111=CARTESIAN_POINT ( 'NONE',  ( -10.64017930668212664, 0.5000000000000004441, 10.57291749337208309 ) ) ;
#16129=VERTEX_POINT ( 'NONE', #49952 ) ;
#16142=CARTESIAN_POINT ( 'NONE',  ( -4.923371831947302546, -4.824402182332542921, -8.527530157486173934 ) ) ;
#16143=ORIENTED_EDGE ( 'NONE', *, *, #91022, .F. ) ;
#16147=ORIENTED_EDGE ( 'NONE', *, *, #59478, .F. ) ;
#16157=EDGE_CURVE ( 'NONE', #44682, #71137, #48964, .T. ) ;
#16159=EDGE_CURVE ( 'NONE', #88013, #89546, #49192, .T. ) ;
#16161=CARTESIAN_POINT ( 'NONE',  ( -6.408140936763246032, 28.29030133659709989, -11.09922568453594316 ) ) ;
#16174=LINE ( 'NONE', #8185, #82390 ) ;
#16175=VECTOR ( 'NONE', #54954, 1000.000000000000114 ) ;
#16176=ORIENTED_EDGE ( 'NONE', *, *, #19935, .T. ) ;
#16178=DIRECTION ( 'NONE',  ( -0.000000000000000000, -1.000000000000000000, -0.000000000000000000 ) ) ;
#16186=AXIS2_PLACEMENT_3D ( 'NONE', #52508, #91501, #76001 ) ;
#16187=ADVANCED_FACE ( 'NONE', ( #34938 ), #80457, .T. ) ;
#16188=DIRECTION ( 'NONE',  ( 0.9996573249755570378, 0.000000000000000000, 0.02617694830788287394 ) ) ;
#16189=ORIENTED_EDGE ( 'NONE', *, *, #16876, .T. ) ;
#16191=CARTESIAN_POINT ( 'NONE',  ( -11.62719953690053742, 14.63606895804558583, -9.476720473301991632 ) ) ;
#16195=CARTESIAN_POINT ( 'NONE',  ( -11.42945456197606724, 2.337810934421868936E-16, -9.127207413380881817 ) ) ;
#16196=CIRCLE ( 'NONE', #41754, 14.49999999999999822 ) ;
#16204=CARTESIAN_POINT ( 'NONE',  ( -12.80781515976318907, 15.00000000000000000, 6.246788841744232990 ) ) ;
#16210=CARTESIAN_POINT ( 'NONE',  ( 11.92686044187656869, 5.370456701841152203, -3.195792623639533758 ) ) ;
#16212=DIRECTION ( 'NONE',  ( 0.000000000000000000, 0.000000000000000000, -1.000000000000000000 ) ) ;
#16214=CARTESIAN_POINT ( 'NONE',  ( -10.36894250292378317, 27.42874883491397853, 10.36894250292379560 ) ) ;
#16218=CARTESIAN_POINT ( 'NONE',  ( -10.04755927614759869, -3.159856409732166232E-15, 10.62803196998849486 ) ) ;
#16233=CARTESIAN_POINT ( 'NONE',  ( 0.000000000000000000, 14.49999999999999822, 0.000000000000000000 ) ) ;
#16266=AXIS2_PLACEMENT_3D ( 'NONE', #97946, #4469, #4952 ) ;
#16267=CARTESIAN_POINT ( 'NONE',  ( 0.000000000000000000, 14.49999999999999822, 0.000000000000000000 ) ) ;
#16272=CARTESIAN_POINT ( 'NONE',  ( -14.42571047809463636, 14.76930270348881002, 3.890621016587766601 ) ) ;
#16274=ORIENTED_EDGE ( 'NONE', *, *, #93009, .F. ) ;
#16281=VERTEX_POINT ( 'NONE', #32975 ) ;
#16283=EDGE_CURVE ( 'NONE', #96556, #97330, #34859, .T. ) ;
#16285=ORIENTED_EDGE ( 'NONE', *, *, #43351, .F. ) ;
#16287=ORIENTED_EDGE ( 'NONE', *, *, #5973, .F. ) ;
#16296=VERTEX_POINT ( 'NONE', #5942 ) ;
#16300=CARTESIAN_POINT ( 'NONE',  ( 0.000000000000000000, 0.5000000000000004441, 0.000000000000000000 ) ) ;
#16305=CARTESIAN_POINT ( 'NONE',  ( 10.80773140175846159, 12.34856811493710715, 3.780460097596739288 ) ) ;
#16314=CARTESIAN_POINT ( 'NONE',  ( 12.07856007377822394, 4.551077920620485022E-16, 8.022367888854921247 ) ) ;
#16324=VECTOR ( 'NONE', #59090, 1000.000000000000000 ) ;
#16330=CARTESIAN_POINT ( 'NONE',  ( 9.520529577030400148, 15.00000000000000888, 11.10395710204425868 ) ) ;
#16365=FACE_OUTER_BOUND ( 'NONE', #35722, .T. ) ;
#16372=AXIS2_PLACEMENT_3D ( 'NONE', #90417, #96980, #97968 ) ;
#16375=CARTESIAN_POINT ( 'NONE',  ( 11.96291822454879750, 15.00000000000000000, -8.193813980849057543 ) ) ;
#16385=EDGE_CURVE ( 'NONE', #88245, #43121, #85971, .T. ) ;
#16390=AXIS2_PLACEMENT_3D ( 'NONE', #78829, #31838, #23882 ) ;
#16394=DIRECTION ( 'NONE',  ( 0.000000000000000000, 0.000000000000000000, 1.000000000000000000 ) ) ;
#16403=CARTESIAN_POINT ( 'NONE',  ( -14.75001642003106994, 14.95037105299814506, 0.3071237627328327058 ) ) ;
#16405=ORIENTED_EDGE ( 'NONE', *, *, #51871, .T. ) ;
#16406=VECTOR ( 'NONE', #90913, 1000.000000000000114 ) ;
#16423=ORIENTED_EDGE ( 'NONE', *, *, #87764, .F. ) ;
#16428=CARTESIAN_POINT ( 'NONE',  ( -12.07856007377814223, 15.00000000000000000, -8.022367888855001183 ) ) ;
#16432=CARTESIAN_POINT ( 'NONE',  ( 12.11331110855135762, 0.04922511925147226436, 8.421032842869534463 ) ) ;
#16436=ADVANCED_FACE ( 'NONE', ( #59413 ), #36427, .T. ) ;
#16453=DIRECTION ( 'NONE',  ( 0.000000000000000000, 1.000000000000000000, 0.000000000000000000 ) ) ;
#16458=CARTESIAN_POINT ( 'NONE',  ( -12.26659068614894110, -12.77958449841935717, 7.082119434687058401 ) ) ;
#16464=CARTESIAN_POINT ( 'NONE',  ( -6.382347221874270282, 0.3639313913011587021, -13.57444820018238829 ) ) ;
#16466=LINE ( 'NONE', #77942, #59999 ) ;
#16498=CARTESIAN_POINT ( 'NONE',  ( 0.000000000000000000, 15.00000000000000000, 0.000000000000000000 ) ) ;
#16499=EDGE_LOOP ( 'NONE', ( #43750, #65975, #90272, #26402, #61335, #42109 ) ) ;
#16510=ORIENTED_EDGE ( 'NONE', *, *, #38726, .T. ) ;
#16516=CIRCLE ( 'NONE', #64370, 15.00000000000000000 ) ;
#16523=CARTESIAN_POINT ( 'NONE',  ( -10.04796213703186503, 15.00000000000000888, 10.62905469192457986 ) ) ;
#16528=EDGE_CURVE ( 'NONE', #98433, #58154, #44481, .T. ) ;
#16529=DIRECTION ( 'NONE',  ( 0.000000000000000000, 0.000000000000000000, 1.000000000000000000 ) ) ;
#16532=CARTESIAN_POINT ( 'NONE',  ( -9.846743663894596210, 25.80059781766745530, -2.638427012816824124 ) ) ;
#16541=ORIENTED_EDGE ( 'NONE', *, *, #79517, .T. ) ;
#16544=ORIENTED_EDGE ( 'NONE', *, *, #79929, .T. ) ;
#16549=ORIENTED_EDGE ( 'NONE', *, *, #17647, .F. ) ;
#16552=CARTESIAN_POINT ( 'NONE',  ( 10.32896413005680181, 6.771642702460840546, 5.963430220938278126 ) ) ;
#16561=EDGE_LOOP ( 'NONE', ( #38202, #33764, #49099 ) ) ;
#16587=CARTESIAN_POINT ( 'NONE',  ( 14.36343418943213912, 0.04922511925147082107, -3.367173657400652775 ) ) ;
#16592=CARTESIAN_POINT ( 'NONE',  ( -7.964842623401172439, 3.688685344154841061, 7.964842623401183097 ) ) ;
#16599=DIRECTION ( 'NONE',  ( -0.000000000000000000, -1.000000000000000000, -0.000000000000000000 ) ) ;
#16612=VECTOR ( 'NONE', #18913, 1000.000000000000000 ) ;
#16620=CARTESIAN_POINT ( 'NONE',  ( 4.020549461440776184, 0.000000000000000000, -3.684154808197036335 ) ) ;
#16622=CARTESIAN_POINT ( 'NONE',  ( 5.815488105659760265, 0.2301500539507717324, -13.76235181012718023 ) ) ;
#16624=ORIENTED_EDGE ( 'NONE', *, *, #68918, .F. ) ;
#16625=ORIENTED_EDGE ( 'NONE', *, *, #75537, .T. ) ;
#16640=CARTESIAN_POINT ( 'NONE',  ( 12.34557190004681360, 0.04922511925147205619, -8.076692058882494862 ) ) ;
#16642=CARTESIAN_POINT ( 'NONE',  ( 7.208316651077762316, -15.86606884899921610, -7.208316651077764980 ) ) ;
#16643=ORIENTED_EDGE ( 'NONE', *, *, #43631, .F. ) ;
#16644=CARTESIAN_POINT ( 'NONE',  ( -13.03370038005733456, 15.00000000000000000, 9.273621236547603175 ) ) ;
#16645=ORIENTED_EDGE ( 'NONE', *, *, #90441, .T. ) ;
#16647=VERTEX_POINT ( 'NONE', #37926 ) ;
#16652=DIRECTION ( 'NONE',  ( -0.000000000000000000, -1.000000000000000000, -0.000000000000000000 ) ) ;
#16653=DIRECTION ( 'NONE',  ( -0.000000000000000000, 1.000000000000000000, -0.000000000000000000 ) ) ;
#16655=CARTESIAN_POINT ( 'NONE',  ( -12.81628187352647608, 29.12363466993042493, 3.903127820947815962E-15 ) ) ;
#16656=VERTEX_POINT ( 'NONE', #70386 ) ;
#16662=EDGE_CURVE ( 'NONE', #72594, #72857, #33609, .T. ) ;
#16666=CARTESIAN_POINT ( 'NONE',  ( 10.64017930668199874, 14.63595249122789177, 10.57291749337223052 ) ) ;
#16669=EDGE_CURVE ( 'NONE', #23582, #35712, #59824, .T. ) ;
#16678=CARTESIAN_POINT ( 'NONE',  ( 12.25993886608603489, 14.49999999999999112, 8.642563219313760925 ) ) ;
#16679=AXIS2_PLACEMENT_3D ( 'NONE', #82609, #45097, #32558 ) ;
#16682=ORIENTED_EDGE ( 'NONE', *, *, #73651, .T. ) ;
#16695=ORIENTED_EDGE ( 'NONE', *, *, #89095, .T. ) ;
#16697=CARTESIAN_POINT ( 'NONE',  ( -14.19749592853509768, -0.03417435944610275333, 7.369430493279844008 ) ) ;
#16702=CARTESIAN_POINT ( 'NONE',  ( -3.866352809136307744, 0.04962897115650977131, 14.23757791217067314 ) ) ;
#16703=CARTESIAN_POINT ( 'NONE',  ( 0.000000000000000000, 15.00000000000000000, 0.000000000000000000 ) ) ;
#16708=CARTESIAN_POINT ( 'NONE',  ( 3.795296366450306547, 30.34541550158064283, -14.16423886937410259 ) ) ;
#16732=CARTESIAN_POINT ( 'NONE',  ( 0.000000000000000000, 0.5000000000000004441, 0.000000000000000000 ) ) ;
#16735=DIRECTION ( 'NONE',  ( -0.9170600743851212711, 0.000000000000000000, -0.3987490689252527476 ) ) ;
#16740=AXIS2_PLACEMENT_3D ( 'NONE', #70288, #84789, #77273 ) ;
#16743=EDGE_LOOP ( 'NONE', ( #16643, #68066, #82751, #57406 ) ) ;
#16745=CARTESIAN_POINT ( 'NONE',  ( -9.240973841163672375, 15.00000000000000000, 11.17382667070363667 ) ) ;
#16757=FACE_OUTER_BOUND ( 'NONE', #35704, .T. ) ;
#16764=ORIENTED_EDGE ( 'NONE', *, *, #52290, .T. ) ;
#16768=EDGE_LOOP ( 'NONE', ( #46530, #41818, #70642, #24286, #20469, #89803 ) ) ;
#16773=ORIENTED_EDGE ( 'NONE', *, *, #51139, .F. ) ;
#16775=AXIS2_PLACEMENT_3D ( 'NONE', #50388, #14885, #45354 ) ;
#16779=VERTEX_POINT ( 'NONE', #68415 ) ;
#16784=CARTESIAN_POINT ( 'NONE',  ( 3.243710765982329214, 0.000000000000000000, -4.383623511354890034 ) ) ;
#16788=EDGE_CURVE ( 'NONE', #36938, #87330, #7430, .T. ) ;
#16789=ORIENTED_EDGE ( 'NONE', *, *, #8372, .F. ) ;
#16796=CARTESIAN_POINT ( 'NONE',  ( -4.289191146912808207E-15, 3.868033628982651795, -11.25000000000000178 ) ) ;
#16803=DIRECTION ( 'NONE',  ( 0.5807029557109406603, 0.000000000000000000, 0.8141155183563185682 ) ) ;
#16807=DIRECTION ( 'NONE',  ( 0.000000000000000000, 0.000000000000000000, -1.000000000000000000 ) ) ;
#16812=DIRECTION ( 'NONE',  ( 0.000000000000000000, 0.000000000000000000, 1.000000000000000000 ) ) ;
#16834=AXIS2_PLACEMENT_3D ( 'NONE', #19773, #80777, #12270 ) ;
#16836=EDGE_CURVE ( 'NONE', #44051, #40499, #7327, .T. ) ;
#16837=EDGE_CURVE ( 'NONE', #55655, #39990, #97185, .T. ) ;
#16839=CARTESIAN_POINT ( 'NONE',  ( -1.457314710996554519, 0.000000000000000000, 5.254907083456953565 ) ) ;
#16846=ORIENTED_EDGE ( 'NONE', *, *, #31510, .F. ) ;
#16848=CARTESIAN_POINT ( 'NONE',  ( 2.815433093577121682, 14.63595249122789177, -14.73340885523751354 ) ) ;
#16861=TOROIDAL_SURFACE ( 'NONE', #8856, 14.49999999999999822, 0.5000000000000000000 ) ;
#16869=PLANE ( 'NONE',  #31041 ) ;
#16876=EDGE_CURVE ( 'NONE', #45246, #27971, #83967, .T. ) ;
#16881=ORIENTED_EDGE ( 'NONE', *, *, #76973, .T. ) ;
#16884=VECTOR ( 'NONE', #17006, 1000.000000000000000 ) ;
#16892=VERTEX_POINT ( 'NONE', #55375 ) ;
#16904=CARTESIAN_POINT ( 'NONE',  ( 0.000000000000000000, 14.49999999999999822, 0.000000000000000000 ) ) ;
#16908=ADVANCED_FACE ( 'NONE', ( #2398 ), #7403, .T. ) ;
#16915=ORIENTED_EDGE ( 'NONE', *, *, #28276, .T. ) ;
#16919=DIRECTION ( 'NONE',  ( -0.9799247046208282574, 0.000000000000000000, -0.1993679344172039347 ) ) ;
#16920=CARTESIAN_POINT ( 'NONE',  ( 0.000000000000000000, 0.5000000000000004441, 0.000000000000000000 ) ) ;
#16924=CARTESIAN_POINT ( 'NONE',  ( 0.000000000000000000, 14.49999999999999822, 0.000000000000000000 ) ) ;
#16934=DIRECTION ( 'NONE',  ( 0.000000000000000000, 0.000000000000000000, 1.000000000000000000 ) ) ;
#16940=PLANE ( 'NONE',  #91476 ) ;
#16941=EDGE_CURVE ( 'NONE', #89575, #72583, #44057, .T. ) ;
#16946=CARTESIAN_POINT ( 'NONE',  ( 12.00809552683962700, 14.63606912728062959, -8.989195838243558612 ) ) ;
#16949=CARTESIAN_POINT ( 'NONE',  ( -10.36894250292378317, -12.57125116508602325, 10.36894250292379560 ) ) ;
#16952=CARTESIAN_POINT ( 'NONE',  ( 13.55255535720595184, 15.00000000000000000, -4.403492169842965431 ) ) ;
#16954=EDGE_CURVE ( 'NONE', #45188, #42998, #41860, .T. ) ;
#16959=EDGE_CURVE ( 'NONE', #89913, #39436, #31273, .T. ) ;
#16960=CARTESIAN_POINT ( 'NONE',  ( -12.83294900548056994, 14.49999999999999112, -7.766300266068596692 ) ) ;
#16961=CARTESIAN_POINT ( 'NONE',  ( 14.03351048042395632, -0.03417435944610275333, 2.474486531753810059 ) ) ;
#16968=CARTESIAN_POINT ( 'NONE',  ( 0.9940297508536876103, 15.00000000000000000, 14.21528771620250353 ) ) ;
#16970=CARTESIAN_POINT ( 'NONE',  ( 12.80781515976314822, 15.00000000000000000, -6.246788841744324472 ) ) ;
#16972=CARTESIAN_POINT ( 'NONE',  ( -3.541595367958631169, 0.000000000000000000, -4.146675399920641603 ) ) ;
#16983=DIRECTION ( 'NONE',  ( 0.000000000000000000, 1.000000000000000000, 0.000000000000000000 ) ) ;
#16989=CARTESIAN_POINT ( 'NONE',  ( 14.03351048042397231, 15.00000000000000000, -2.474486531753715024 ) ) ;
#16990=CYLINDRICAL_SURFACE ( 'NONE', #56153, 15.00000000000000000 ) ;
#16993=CARTESIAN_POINT ( 'NONE',  ( 0.000000000000000000, 15.00000000000000000, 0.000000000000000000 ) ) ;
#16994=LINE ( 'NONE', #47473, #92553 ) ;
#16997=EDGE_CURVE ( 'NONE', #78552, #6506, #63249, .T. ) ;
#17002=ORIENTED_EDGE ( 'NONE', *, *, #42681, .F. ) ;
#17006=DIRECTION ( 'NONE',  ( -0.3826834323650877279, 0.000000000000000000, 0.9238795325112876267 ) ) ;
#17013=DIRECTION ( 'NONE',  ( 0.000000000000000000, 1.000000000000000000, 0.000000000000000000 ) ) ;
#17019=DIRECTION ( 'NONE',  ( -0.6755902076156540259, 0.000000000000000000, -0.7372773368101297464 ) ) ;
#17023=CARTESIAN_POINT ( 'NONE',  ( 8.527530157486179263, 23.09226448433413026, 4.923371831947292776 ) ) ;
#17025=CARTESIAN_POINT ( 'NONE',  ( -13.55255535720589322, 15.00000000000000000, -4.403492169843143067 ) ) ;
#17031=VECTOR ( 'NONE', #40688, 1000.000000000000000 ) ;
#17035=ORIENTED_EDGE ( 'NONE', *, *, #82411, .F. ) ;
#17045=EDGE_CURVE ( 'NONE', #78351, #42731, #86368, .T. ) ;
#17049=EDGE_CURVE ( 'NONE', #89452, #59664, #63354, .T. ) ;
#17052=ORIENTED_EDGE ( 'NONE', *, *, #65798, .T. ) ;
#17053=TOROIDAL_SURFACE ( 'NONE', #1074, 14.49999999999999822, 0.5000000000000000000 ) ;
#17054=TOROIDAL_SURFACE ( 'NONE', #96857, 14.49999999999999822, 0.5000000000000000000 ) ;
#17063=CARTESIAN_POINT ( 'NONE',  ( 3.115783986955559470, 4.823715477197806954E-16, -14.16128137375397777 ) ) ;
#17074=CARTESIAN_POINT ( 'NONE',  ( -13.21236992757677164, 0.000000000000000000, 5.338143956176621074 ) ) ;
#17080=VERTEX_POINT ( 'NONE', #40871 ) ;
#17088=CARTESIAN_POINT ( 'NONE',  ( 0.000000000000000000, 0.5000000000000004441, 0.000000000000000000 ) ) ;
#17093=CARTESIAN_POINT ( 'NONE',  ( 7.964842623401177768, 6.188685344154841061, -7.964842623401181321 ) ) ;
#17095=CARTESIAN_POINT ( 'NONE',  ( 4.850115630859686888, 14.95077488074853456, -13.93278430610806495 ) ) ;
#17099=FACE_OUTER_BOUND ( 'NONE', #98057, .T. ) ;
#17102=DIRECTION ( 'NONE',  ( 0.000000000000000000, 0.000000000000000000, -1.000000000000000000 ) ) ;
#17141=CARTESIAN_POINT ( 'NONE',  ( -8.721827932831924812, 15.00000000000000178, 11.74045266257169473 ) ) ;
#17143=B_SPLINE_CURVE_WITH_KNOTS ( 'NONE', 3,
 ( #22889, #83868, #7883, #38375, #68876, #26797 ),
 .UNSPECIFIED., .F., .F.,
 ( 4, 2, 4 ),
 ( 0.0002800225282622548998, 0.0006862279780598551935, 0.001092433427857455487 ),
 .UNSPECIFIED. ) ;
#17144=CARTESIAN_POINT ( 'NONE',  ( -3.469446951953614189E-15, -15.24106884899921077, -9.846743663894594434 ) ) ;
#17145=ORIENTED_EDGE ( 'NONE', *, *, #78846, .T. ) ;
#17146=DIRECTION ( 'NONE',  ( 0.000000000000000000, 0.000000000000000000, -1.000000000000000000 ) ) ;
#17154=FACE_OUTER_BOUND ( 'NONE', #84879, .T. ) ;
#17160=ORIENTED_EDGE ( 'NONE', *, *, #54038, .T. ) ;
#17162=VERTEX_POINT ( 'NONE', #67178 ) ;
#17165=CARTESIAN_POINT ( 'NONE',  ( -5.419894505350674407, 0.5000000000000004441, 13.98659156302455031 ) ) ;
#17167=( BOUNDED_SURFACE ( )  B_SPLINE_SURFACE ( 1, 2, ( 
 ( #3731, #4219, #13181, #74161, #42216, #34690, #66173, #96706, #87693, #35688, #87206, #18730, #34192, #65183, #20693, #50187, #95705, #27687, #80698, #50693, #42701, #5695, #49211, #27188, #28184, #72683, #57691, #49691, #51185, #65680, #88189, #79714, #64685, #57196, #81667, #12192, #81187, #96204, #35179, #11706, #72203, #58171, #12688, #58680, #43674, #11214, #41732, #98690, #52170, #36683, #68655, #60647, #184, #84163, #15668, #98187, #53151, #46153, #7675, #97696, #45152, #29160, #21185, #13676, #59663, #83657, #51685, #29645, #75657, #7168, #38168, #21685, #6669, #82664, #91649, #90154, #37188, #67172, #60152, #76637, #14180, #90649, #67678, #30632, #82163, #44663, #91146, #6180, #37671, #97206, #22672, #15174, #61141, #75158, #22175, #23167, #53645, #52656, #68171, #83159, #74670, #14683, #8156, #66681, #30139, #45655, #28674, #59167, #76151, #89673, #44160, #61623, #77129, #17632, #47115, #56115, #63595, #16642, #9127, #32105, #17144, #86121, #63106, #48594, #79098, #77615, #62604, #18122, #47622, #39643, #55107, #55623, #1161, #70136, #1656, #93112, #48103, #78118, #24145, #8638, #38648, #92141, #39148, #78616, #24639, #86612, #94101, #85627, #9626, #40125, #70625, #10125, #93609, #69153, #678, #2153, #32610, #31127, #25146, #40622, #71120, #2647, #31622, #33101, #25624, #23666, #54127, #84640, #54613, #69637, #16142, #46628, #62114, #92623, #85133, #42581, #65058, #4596, #57571, #89062, #3124, #11586, #50572, #57084, #19091, #3609, #66058, #80580, #49571, #64076, #79598, #11100, #96585, #87578, #65558, #12075, #19581, #18605, #87093, #72565, #34564, #27566, #49095, #95585, #4102, #73063, #95077, #41618, #12570, #35059, #43071, #28060, #58556, #42102, #96084, #20577, #81068, #72084, #88068, #34074, #94592, #56603, #64568, #58061, #26109, #27071, #50078, #88565, #73556, #26583, #80081, #20068, #35566, #5079, #51061, #10611, #41123, #71613, #33582, #6551, #52057, #22559, #36060, #29042, #75542, #21067, #60037, #13061, #7058, #30028, #76033, #13560, #59550, #38053, #83543, #44047, #52541, #37062, #89560, #90046, #77, #61025, #21568, #82550, #53028, #15066, #74550, #91029, #74049, #51564, #82049, #45536, #98578, #14067, #44548, #6067, #91537, #75043, #14566, #23053, #67560, #5584, #83047, #98071, #68544, #30524, #90533, #36567, #7566, #67055, #97581, #29531, #22067, #45033, #37560, #68050, #60536, #81552, #43553, #66561, #97090, #28560, #59055, #54994, #17023, #31990, #32986, #25024, #93992, #70512, #46517, #55509, #24534, #62496, #2036, #92021, #86009, #16532, #77499, #47500, #15556, #63489, #24035, #93000, #47008, #39032, #40513, #9011, #32497, #47988, #46042, #2532, #92505, #39527, #78003, #70021, #1545, #71010, #1042, #8532, #17521, #78498, #54022, #85512, #54505, #53524, #84036, #23552, #62995 ),
 ( #8042, #571, #16029, #93499, #38542, #85018, #9508, #40010, #10012, #69527, #76526, #31505, #69037, #84531, #31017, #77018, #61513, #62007, #94475, #49460, #94964, #65445, #78985, #71972, #19470, #63962, #3984, #56001, #49961, #72951, #19954, #56488, #3495, #80955, #27453, #86976, #95470, #79966, #11471, #56965, #87467, #25993, #80465, #42468, #18487, #41989, #86505, #4479, #73440, #57461, #11964, #18003, #87954, #3016, #18982, #33953, #72453, #33465, #79483, #57946, #48975, #10983, #95969, #34946, #64456, #34451, #41504, #4966, #64943, #88453, #65943, #26961, #48483, #50448, #26465, #12453, #35447, #42959, #25515, #10492, #41003, #71503, #28443, #81931, #5952, #66436, #44424, #6428, #43926, #7439, #98453, #59918, #81441, #89928, #97957, #90406, #74929, #75915, #67933, #37936, #14443, #89441, #29909, #67436, #36940, #44913, #35940, #60415, #59425, #21443, #21948, #58434, #96470, #66936, #29413, #51941, #13439, #83422, #82425, #75420, #90910, #88949, #45410, #36443, #13950, #52426, #82925, #6935, #14941, #74424, #51442, #22438, #52909, #96971, #37442, #97457, #27942, #20456, #58941, #50947, #12943, #20954, #28922, #43439, #73940, #5468, #10258, #40262, #9763, #94728, #40751, #7924, #25278, #87219, #30403, #49227, #70769, #79232, #55758, #32743, #79728, #71737, #60906, #71255, #45920, #17763, #98948, #63726, #18249, #64212, #1789, #47750, #26234, #3246, #32244, #2778, #93743, #76408, #78247, #18743, #11227, #17275, #2284, #41263, #33713, #62747, #10745, #91408, #22935, #39774, #48728, #63239, #68425, #56729, #86251, #48240, #78752, #33233, #53403, #94227, #83912, #15440, #25759, #56252, #70272, #86745, #93249, #24773, #55249, #85764, #50200, #73195, #65695, #58691, #20203, #27203, #11718, #41747, #12206, #66693, #96218, #80711, #73683, #27699, #35699, #88695, #21200, #34207, #42713, #81679, #88203, #4727, #34702, #97220, #12701, #35191, #95209, #42231, #72697, #28687, #19713, #96719, #43196, #50707, #49704, #19223, #58183, #81200, #89194, #80212, #5219, #66184, #28195, #57703, #4232, #43688, #20705, #74174, #59180, #89684, #51198, #13194, #51698, #5707, #65196, #36195, #95718, #26715, #87708, #82180, #72216, #57211, #3747, #64697, #53167, #84176, #67692, #52672, #29661, #38664, #44678, #83174, #14197, #45169, #92155, #82678, #37688, #14699, #53659, #67188, #60170, #7687, #52184, #91161, #68185, #75671, #45670, #98204, #75173, #15683, #38185, #46168, #31145, #61635, #7184, #198, #23680, #76652, #6683, #22687, #37201, #97712, #59677, #90666, #30648, #29177, #98706, #83672, #15187, #8172, #22193, #30156, #60660, #69168, #76167, #68671, #61156, #91665, #54144, #23182, #691, #13691, #44175, #90168, #74684, #6196, #36700, #21700, #16161, #78632, #33113, #79114, #16655, #62618, #41139, #86625, #47129, #55635, #9642 ) ),
 .UNSPECIFIED., .F., .F., .F. ) 
 B_SPLINE_SURFACE_WITH_KNOTS ( ( 2, 2 ),
 ( 3, 2, 2, 2, 2, 2, 2, 2, 2, 2, 2, 2, 2, 2, 2, 2, 2, 2, 2, 2, 2, 2, 2, 2, 2, 2, 2, 2, 2, 2, 2, 2, 2, 2, 2, 2, 2, 2, 2, 2, 2, 2, 2, 2, 2, 2, 2, 2, 2, 2, 2, 2, 2, 2, 2, 2, 2, 2, 2, 2, 2, 2, 2, 2, 2, 2, 2, 2, 2, 2, 2, 2, 2, 2, 2, 2, 2, 2, 2, 2, 2, 2, 2, 2, 2, 2, 2, 2, 2, 2, 2, 2, 2, 2, 2, 2, 2, 2, 2, 2, 2, 2, 2, 2, 2, 2, 2, 2, 2, 2, 2, 2, 2, 2, 2, 2, 2, 2, 2, 2, 2, 2, 2, 2, 2, 2, 2, 2, 2, 2, 2, 2, 2, 2, 2, 2, 2, 2, 2, 2, 2, 2, 2, 2, 2, 2, 2, 2, 2, 2, 2, 2, 2, 2, 2, 2, 2, 2, 2, 2, 2, 2, 2, 2, 2, 2, 2, 2, 2, 2, 2, 2, 2, 2, 3 ),
 ( 0.000000000000000000, 1.000000000000000000 ),
 ( 0.000000000000000000, 0.005555555555555555768, 0.01111111111111111154, 0.01666666666666666644, 0.02222222222222222307, 0.02777777777777777624, 0.03333333333333333287, 0.03888888888888888951, 0.04444444444444444614, 0.05000000000000000278, 0.05555555555555555247, 0.06111111111111110911, 0.06666666666666666574, 0.07222222222222221544, 0.07777777777777777901, 0.08333333333333332871, 0.08888888888888889228, 0.09444444444444444198, 0.1000000000000000056, 0.1055555555555555552, 0.1111111111111111049, 0.1166666666666666685, 0.1222222222222222182, 0.1277777777777777679, 0.1333333333333333315, 0.1388888888888888951, 0.1444444444444444309, 0.1499999999999999944, 0.1555555555555555580, 0.1611111111111111216, 0.1666666666666666574, 0.1722222222222222210, 0.1777777777777777846, 0.1833333333333333204, 0.1888888888888888840, 0.1944444444444444475, 0.2000000000000000111, 0.2055555555555555469, 0.2111111111111111105, 0.2166666666666666741, 0.2222222222222222099, 0.2277777777777777735, 0.2333333333333333370, 0.2388888888888889006, 0.2444444444444444364, 0.2500000000000000000, 0.2555555555555555358, 0.2611111111111111271, 0.2666666666666666630, 0.2722222222222221988, 0.2777777777777777901, 0.2833333333333333259, 0.2888888888888888618, 0.2944444444444444531, 0.2999999999999999889, 0.3055555555555555802, 0.3111111111111111160, 0.3166666666666666519, 0.3222222222222222432, 0.3277777777777777790, 0.3333333333333333148, 0.3388888888888889062, 0.3444444444444444420, 0.3499999999999999778, 0.3555555555555555691, 0.3611111111111111049, 0.3666666666666666408, 0.3722222222222222321, 0.3777777777777777679, 0.3833333333333333592, 0.3888888888888888951, 0.3944444444444444309, 0.4000000000000000222, 0.4055555555555555580, 0.4111111111111110938, 0.4166666666666666852, 0.4222222222222222210, 0.4277777777777777568, 0.4333333333333333481, 0.4388888888888888840, 0.4444444444444444198, 0.4500000000000000111, 0.4555555555555555469, 0.4611111111111111382, 0.4666666666666666741, 0.4722222222222222099, 0.4777777777777778012, 0.4833333333333333370, 0.4888888888888888729, 0.4944444444444444642, 0.5000000000000000000, 0.5055555555555555358, 0.5111111111111110716, 0.5166666666666667185, 0.5222222222222222543, 0.5277777777777777901, 0.5333333333333333259, 0.5388888888888888618, 0.5444444444444443976, 0.5500000000000000444, 0.5555555555555555802, 0.5611111111111111160, 0.5666666666666666519, 0.5722222222222221877, 0.5777777777777777235, 0.5833333333333333703, 0.5888888888888889062, 0.5944444444444444420, 0.5999999999999999778, 0.6055555555555555136, 0.6111111111111111605, 0.6166666666666666963, 0.6222222222222222321, 0.6277777777777777679, 0.6333333333333333037, 0.6388888888888888395, 0.6444444444444444864, 0.6500000000000000222, 0.6555555555555555580, 0.6611111111111110938, 0.6666666666666666297, 0.6722222222222222765, 0.6777777777777778123, 0.6833333333333333481, 0.6888888888888888840, 0.6944444444444444198, 0.6999999999999999556, 0.7055555555555556024, 0.7111111111111111382, 0.7166666666666666741, 0.7222222222222222099, 0.7277777777777777457, 0.7333333333333332815, 0.7388888888888889284, 0.7444444444444444642, 0.7500000000000000000, 0.7555555555555555358, 0.7611111111111110716, 0.7666666666666667185, 0.7722222222222222543, 0.7777777777777777901, 0.7833333333333333259, 0.7888888888888888618, 0.7944444444444443976, 0.8000000000000000444, 0.8055555555555555802, 0.8111111111111111160, 0.8166666666666666519, 0.8222222222222221877, 0.8277777777777777235, 0.8333333333333333703, 0.8388888888888889062, 0.8444444444444444420, 0.8499999999999999778, 0.8555555555555555136, 0.8611111111111111605, 0.8666666666666666963, 0.8722222222222222321, 0.8777777777777777679, 0.8833333333333333037, 0.8888888888888888395, 0.8944444444444444864, 0.9000000000000000222, 0.9055555555555555580, 0.9111111111111110938, 0.9166666666666666297, 0.9222222222222222765, 0.9277777777777778123, 0.9333333333333333481, 0.9388888888888888840, 0.9444444444444444198, 0.9499999999999999556, 0.9555555555555556024, 0.9611111111111111382, 0.9666666666666666741 ),
 .UNSPECIFIED. ) 
 GEOMETRIC_REPRESENTATION_ITEM ( )  RATIONAL_B_SPLINE_SURFACE ( (
 ( 1.000000000000000000, 0.9659258262890683122, 1.000000000000000000, 0.9659258262890683122, 1.000000000000000000, 0.9659258262890683122, 1.000000000000000000, 0.9659258262890683122, 1.000000000000000000, 0.9659258262890683122, 1.000000000000000000, 0.9659258262890683122, 1.000000000000000000, 0.9659258262890683122, 1.000000000000000000, 0.9659258262890683122, 1.000000000000000000, 0.9659258262890683122, 1.000000000000000000, 0.9659258262890683122, 1.000000000000000000, 0.9659258262890683122, 1.000000000000000000, 0.9659258262890683122, 1.000000000000000000, 0.9659258262890683122, 1.000000000000000000, 0.9659258262890683122, 1.000000000000000000, 0.9659258262890683122, 1.000000000000000000, 0.9659258262890683122, 1.000000000000000000, 0.9659258262890683122, 1.000000000000000000, 0.9659258262890683122, 1.000000000000000000, 0.9659258262890683122, 1.000000000000000000, 0.9659258262890683122, 1.000000000000000000, 0.9659258262890683122, 1.000000000000000000, 0.9659258262890683122, 1.000000000000000000, 0.9659258262890683122, 1.000000000000000000, 0.9659258262890683122, 1.000000000000000000, 0.9659258262890683122, 1.000000000000000000, 0.9659258262890683122, 1.000000000000000000, 0.9659258262890683122, 1.000000000000000000, 0.9659258262890683122, 1.000000000000000000, 0.9659258262890683122, 1.000000000000000000, 0.9659258262890683122, 1.000000000000000000, 0.9659258262890683122, 1.000000000000000000, 0.9659258262890683122, 1.000000000000000000, 0.9659258262890683122, 1.000000000000000000, 0.9659258262890683122, 1.000000000000000000, 0.9659258262890683122, 1.000000000000000000, 0.9659258262890683122, 1.000000000000000000, 0.9659258262890683122, 1.000000000000000000, 0.9659258262890683122, 1.000000000000000000, 0.9659258262890683122, 1.000000000000000000, 0.9659258262890683122, 1.000000000000000000, 0.9659258262890683122, 1.000000000000000000, 0.9659258262890683122, 1.000000000000000000, 0.9659258262890683122, 1.000000000000000000, 0.9659258262890683122, 1.000000000000000000, 0.9659258262890683122, 1.000000000000000000, 0.9659258262890683122, 1.000000000000000000, 0.9659258262890683122, 1.000000000000000000, 0.9659258262890683122, 1.000000000000000000, 0.9659258262890683122, 1.000000000000000000, 0.9659258262890683122, 1.000000000000000000, 0.9659258262890683122, 1.000000000000000000, 0.9659258262890683122, 1.000000000000000000, 0.9659258262890683122, 1.000000000000000000, 0.9659258262890683122, 1.000000000000000000, 0.9659258262890683122, 1.000000000000000000, 0.9659258262890683122, 1.000000000000000000, 0.9659258262890683122, 1.000000000000000000, 0.9659258262890683122, 1.000000000000000000, 0.9659258262890683122, 1.000000000000000000, 0.9659258262890683122, 1.000000000000000000, 0.9659258262890683122, 1.000000000000000000, 0.9659258262890683122, 1.000000000000000000, 0.9659258262890683122, 1.000000000000000000, 0.9659258262890683122, 1.000000000000000000, 0.9659258262890683122, 1.000000000000000000, 0.9659258262890683122, 1.000000000000000000, 0.9659258262890683122, 1.000000000000000000, 0.9659258262890683122, 1.000000000000000000, 0.9659258262890683122, 1.000000000000000000, 0.9659258262890683122, 1.000000000000000000, 0.9659258262890683122, 1.000000000000000000, 0.9659258262890683122, 1.000000000000000000, 0.9659258262890683122, 1.000000000000000000, 0.9659258262890683122, 1.000000000000000000, 0.9659258262890683122, 1.000000000000000000, 0.9659258262890683122, 1.000000000000000000, 0.9659258262890683122, 1.000000000000000000, 0.9659258262890683122, 1.000000000000000000, 0.9659258262890683122, 1.000000000000000000, 0.9659258262890683122, 1.000000000000000000, 0.9659258262890683122, 1.000000000000000000, 0.9659258262890683122, 1.000000000000000000, 0.9659258262890683122, 1.000000000000000000, 0.9659258262890683122, 1.000000000000000000, 0.9659258262890683122, 1.000000000000000000, 0.9659258262890683122, 1.000000000000000000, 0.9659258262890683122, 1.000000000000000000, 0.9659258262890683122, 1.000000000000000000, 0.9659258262890683122, 1.000000000000000000, 0.9659258262890683122, 1.000000000000000000, 0.9659258262890683122, 1.000000000000000000, 0.9659258262890683122, 1.000000000000000000, 0.9659258262890683122, 1.000000000000000000, 0.9659258262890683122, 1.000000000000000000, 0.9659258262890683122, 1.000000000000000000, 0.9659258262890683122, 1.000000000000000000, 0.9659258262890683122, 1.000000000000000000, 0.9659258262890683122, 1.000000000000000000, 0.9659258262890683122, 1.000000000000000000, 0.9659258262890683122, 1.000000000000000000, 0.9659258262890683122, 1.000000000000000000, 0.9659258262890683122, 1.000000000000000000, 0.9659258262890683122, 1.000000000000000000, 0.9659258262890683122, 1.000000000000000000, 0.9659258262890683122, 1.000000000000000000, 0.9659258262890683122, 1.000000000000000000, 0.9659258262890683122, 1.000000000000000000, 0.9659258262890683122, 1.000000000000000000, 0.9659258262890683122, 1.000000000000000000, 0.9659258262890683122, 1.000000000000000000, 0.9659258262890683122, 1.000000000000000000, 0.9659258262890683122, 1.000000000000000000, 0.9659258262890683122, 1.000000000000000000, 0.9659258262890683122, 1.000000000000000000, 0.9659258262890683122, 1.000000000000000000, 0.9659258262890683122, 1.000000000000000000, 0.9659258262890683122, 1.000000000000000000, 0.9659258262890683122, 1.000000000000000000, 0.9659258262890683122, 1.000000000000000000, 0.9659258262890683122, 1.000000000000000000, 0.9659258262890683122, 1.000000000000000000, 0.9659258262890683122, 1.000000000000000000, 0.9659258262890683122, 1.000000000000000000, 0.9659258262890683122, 1.000000000000000000, 0.9659258262890683122, 1.000000000000000000, 0.9659258262890683122, 1.000000000000000000, 0.9659258262890683122, 1.000000000000000000, 0.9659258262890683122, 1.000000000000000000, 0.9659258262890683122, 1.000000000000000000, 0.9659258262890683122, 1.000000000000000000, 0.9659258262890683122, 1.000000000000000000, 0.9659258262890683122, 1.000000000000000000, 0.9659258262890683122, 1.000000000000000000, 0.9659258262890683122, 1.000000000000000000, 0.9659258262890683122, 1.000000000000000000, 0.9659258262890683122, 1.000000000000000000, 0.9659258262890683122, 1.000000000000000000, 0.9659258262890683122, 1.000000000000000000, 0.9659258262890683122, 1.000000000000000000, 0.9659258262890683122, 1.000000000000000000, 0.9659258262890683122, 1.000000000000000000, 0.9659258262890683122, 1.000000000000000000, 0.9659258262890683122, 1.000000000000000000, 0.9659258262890683122, 1.000000000000000000, 0.9659258262890683122, 1.000000000000000000, 0.9659258262890683122, 1.000000000000000000, 0.9659258262890683122, 1.000000000000000000, 0.9659258262890683122, 1.000000000000000000, 0.9659258262890683122, 1.000000000000000000, 0.9659258262890683122, 1.000000000000000000, 0.9659258262890683122, 1.000000000000000000, 0.9659258262890683122, 1.000000000000000000, 0.9659258262890683122, 1.000000000000000000, 0.9659258262890683122, 1.000000000000000000, 0.9659258262890683122, 1.000000000000000000, 0.9659258262890683122, 1.000000000000000000, 0.9659258262890683122, 1.000000000000000000, 0.9659258262890683122, 1.000000000000000000, 0.9659258262890683122, 1.000000000000000000, 0.9659258262890683122, 1.000000000000000000, 0.9659258262890683122, 1.000000000000000000, 0.9659258262890683122, 1.000000000000000000, 0.9659258262890683122, 1.000000000000000000, 0.9659258262890683122, 1.000000000000000000, 0.9659258262890683122, 1.000000000000000000, 0.9659258262890683122, 1.000000000000000000, 0.9659258262890683122, 1.000000000000000000, 0.9659258262890683122, 1.000000000000000000, 0.9659258262890683122, 1.000000000000000000, 0.9659258262890683122, 1.000000000000000000, 0.9659258262890683122, 1.000000000000000000, 0.9659258262890683122, 1.000000000000000000, 0.9659258262890683122, 1.000000000000000000, 0.9659258262890683122, 1.000000000000000000),
 ( 1.000000000000000000, 0.9659258262890683122, 1.000000000000000000, 0.9659258262890683122, 1.000000000000000000, 0.9659258262890683122, 1.000000000000000000, 0.9659258262890683122, 1.000000000000000000, 0.9659258262890683122, 1.000000000000000000, 0.9659258262890683122, 1.000000000000000000, 0.9659258262890683122, 1.000000000000000000, 0.9659258262890683122, 1.000000000000000000, 0.9659258262890683122, 1.000000000000000000, 0.9659258262890683122, 1.000000000000000000, 0.9659258262890683122, 1.000000000000000000, 0.9659258262890683122, 1.000000000000000000, 0.9659258262890683122, 1.000000000000000000, 0.9659258262890683122, 1.000000000000000000, 0.9659258262890683122, 1.000000000000000000, 0.9659258262890683122, 1.000000000000000000, 0.9659258262890683122, 1.000000000000000000, 0.9659258262890683122, 1.000000000000000000, 0.9659258262890683122, 1.000000000000000000, 0.9659258262890683122, 1.000000000000000000, 0.9659258262890683122, 1.000000000000000000, 0.9659258262890683122, 1.000000000000000000, 0.9659258262890683122, 1.000000000000000000, 0.9659258262890683122, 1.000000000000000000, 0.9659258262890683122, 1.000000000000000000, 0.9659258262890683122, 1.000000000000000000, 0.9659258262890683122, 1.000000000000000000, 0.9659258262890683122, 1.000000000000000000, 0.9659258262890683122, 1.000000000000000000, 0.9659258262890683122, 1.000000000000000000, 0.9659258262890683122, 1.000000000000000000, 0.9659258262890683122, 1.000000000000000000, 0.9659258262890683122, 1.000000000000000000, 0.9659258262890683122, 1.000000000000000000, 0.9659258262890683122, 1.000000000000000000, 0.9659258262890683122, 1.000000000000000000, 0.9659258262890683122, 1.000000000000000000, 0.9659258262890683122, 1.000000000000000000, 0.9659258262890683122, 1.000000000000000000, 0.9659258262890683122, 1.000000000000000000, 0.9659258262890683122, 1.000000000000000000, 0.9659258262890683122, 1.000000000000000000, 0.9659258262890683122, 1.000000000000000000, 0.9659258262890683122, 1.000000000000000000, 0.9659258262890683122, 1.000000000000000000, 0.9659258262890683122, 1.000000000000000000, 0.9659258262890683122, 1.000000000000000000, 0.9659258262890683122, 1.000000000000000000, 0.9659258262890683122, 1.000000000000000000, 0.9659258262890683122, 1.000000000000000000, 0.9659258262890683122, 1.000000000000000000, 0.9659258262890683122, 1.000000000000000000, 0.9659258262890683122, 1.000000000000000000, 0.9659258262890683122, 1.000000000000000000, 0.9659258262890683122, 1.000000000000000000, 0.9659258262890683122, 1.000000000000000000, 0.9659258262890683122, 1.000000000000000000, 0.9659258262890683122, 1.000000000000000000, 0.9659258262890683122, 1.000000000000000000, 0.9659258262890683122, 1.000000000000000000, 0.9659258262890683122, 1.000000000000000000, 0.9659258262890683122, 1.000000000000000000, 0.9659258262890683122, 1.000000000000000000, 0.9659258262890683122, 1.000000000000000000, 0.9659258262890683122, 1.000000000000000000, 0.9659258262890683122, 1.000000000000000000, 0.9659258262890683122, 1.000000000000000000, 0.9659258262890683122, 1.000000000000000000, 0.9659258262890683122, 1.000000000000000000, 0.9659258262890683122, 1.000000000000000000, 0.9659258262890683122, 1.000000000000000000, 0.9659258262890683122, 1.000000000000000000, 0.9659258262890683122, 1.000000000000000000, 0.9659258262890683122, 1.000000000000000000, 0.9659258262890683122, 1.000000000000000000, 0.9659258262890683122, 1.000000000000000000, 0.9659258262890683122, 1.000000000000000000, 0.9659258262890683122, 1.000000000000000000, 0.9659258262890683122, 1.000000000000000000, 0.9659258262890683122, 1.000000000000000000, 0.9659258262890683122, 1.000000000000000000, 0.9659258262890683122, 1.000000000000000000, 0.9659258262890683122, 1.000000000000000000, 0.9659258262890683122, 1.000000000000000000, 0.9659258262890683122, 1.000000000000000000, 0.9659258262890683122, 1.000000000000000000, 0.9659258262890683122, 1.000000000000000000, 0.9659258262890683122, 1.000000000000000000, 0.9659258262890683122, 1.000000000000000000, 0.9659258262890683122, 1.000000000000000000, 0.9659258262890683122, 1.000000000000000000, 0.9659258262890683122, 1.000000000000000000, 0.9659258262890683122, 1.000000000000000000, 0.9659258262890683122, 1.000000000000000000, 0.9659258262890683122, 1.000000000000000000, 0.9659258262890683122, 1.000000000000000000, 0.9659258262890683122, 1.000000000000000000, 0.9659258262890683122, 1.000000000000000000, 0.9659258262890683122, 1.000000000000000000, 0.9659258262890683122, 1.000000000000000000, 0.9659258262890683122, 1.000000000000000000, 0.9659258262890683122, 1.000000000000000000, 0.9659258262890683122, 1.000000000000000000, 0.9659258262890683122, 1.000000000000000000, 0.9659258262890683122, 1.000000000000000000, 0.9659258262890683122, 1.000000000000000000, 0.9659258262890683122, 1.000000000000000000, 0.9659258262890683122, 1.000000000000000000, 0.9659258262890683122, 1.000000000000000000, 0.9659258262890683122, 1.000000000000000000, 0.9659258262890683122, 1.000000000000000000, 0.9659258262890683122, 1.000000000000000000, 0.9659258262890683122, 1.000000000000000000, 0.9659258262890683122, 1.000000000000000000, 0.9659258262890683122, 1.000000000000000000, 0.9659258262890683122, 1.000000000000000000, 0.9659258262890683122, 1.000000000000000000, 0.9659258262890683122, 1.000000000000000000, 0.9659258262890683122, 1.000000000000000000, 0.9659258262890683122, 1.000000000000000000, 0.9659258262890683122, 1.000000000000000000, 0.9659258262890683122, 1.000000000000000000, 0.9659258262890683122, 1.000000000000000000, 0.9659258262890683122, 1.000000000000000000, 0.9659258262890683122, 1.000000000000000000, 0.9659258262890683122, 1.000000000000000000, 0.9659258262890683122, 1.000000000000000000, 0.9659258262890683122, 1.000000000000000000, 0.9659258262890683122, 1.000000000000000000, 0.9659258262890683122, 1.000000000000000000, 0.9659258262890683122, 1.000000000000000000, 0.9659258262890683122, 1.000000000000000000, 0.9659258262890683122, 1.000000000000000000, 0.9659258262890683122, 1.000000000000000000, 0.9659258262890683122, 1.000000000000000000, 0.9659258262890683122, 1.000000000000000000, 0.9659258262890683122, 1.000000000000000000, 0.9659258262890683122, 1.000000000000000000, 0.9659258262890683122, 1.000000000000000000, 0.9659258262890683122, 1.000000000000000000, 0.9659258262890683122, 1.000000000000000000, 0.9659258262890683122, 1.000000000000000000, 0.9659258262890683122, 1.000000000000000000, 0.9659258262890683122, 1.000000000000000000, 0.9659258262890683122, 1.000000000000000000, 0.9659258262890683122, 1.000000000000000000, 0.9659258262890683122, 1.000000000000000000, 0.9659258262890683122, 1.000000000000000000, 0.9659258262890683122, 1.000000000000000000, 0.9659258262890683122, 1.000000000000000000, 0.9659258262890683122, 1.000000000000000000, 0.9659258262890683122, 1.000000000000000000, 0.9659258262890683122, 1.000000000000000000, 0.9659258262890683122, 1.000000000000000000, 0.9659258262890683122, 1.000000000000000000, 0.9659258262890683122, 1.000000000000000000, 0.9659258262890683122, 1.000000000000000000, 0.9659258262890683122, 1.000000000000000000, 0.9659258262890683122, 1.000000000000000000, 0.9659258262890683122, 1.000000000000000000, 0.9659258262890683122, 1.000000000000000000, 0.9659258262890683122, 1.000000000000000000, 0.9659258262890683122, 1.000000000000000000, 0.9659258262890683122, 1.000000000000000000, 0.9659258262890683122, 1.000000000000000000, 0.9659258262890683122, 1.000000000000000000, 0.9659258262890683122, 1.000000000000000000, 0.9659258262890683122, 1.000000000000000000, 0.9659258262890683122, 1.000000000000000000, 0.9659258262890683122, 1.000000000000000000, 0.9659258262890683122, 1.000000000000000000, 0.9659258262890683122, 1.000000000000000000, 0.9659258262890683122, 1.000000000000000000, 0.9659258262890683122, 1.000000000000000000) ) ) 
 REPRESENTATION_ITEM ( '' )  SURFACE ( )  );
#17173=CARTESIAN_POINT ( 'NONE',  ( -14.35840480524203144, 0.5000000000000004441, 4.340070442838751319 ) ) ;
#17174=ORIENTED_EDGE ( 'NONE', *, *, #17906, .F. ) ;
#17175=PLANE ( 'NONE',  #15833 ) ;
#17177=DIRECTION ( 'NONE',  ( 0.000000000000000000, 0.000000000000000000, 1.000000000000000000 ) ) ;
#17180=DIRECTION ( 'NONE',  ( 0.3173046564050899243, -0.000000000000000000, 0.9483236552061999891 ) ) ;
#17182=ORIENTED_EDGE ( 'NONE', *, *, #67760, .T. ) ;
#17188=ORIENTED_EDGE ( 'NONE', *, *, #36018, .F. ) ;
#17190=CIRCLE ( 'NONE', #98650, 15.00000000000000000 ) ;
#17197=EDGE_CURVE ( 'NONE', #4683, #78530, #44167, .T. ) ;
#17199=EDGE_CURVE ( 'NONE', #63596, #33570, #53158, .T. ) ;
#17207=DIRECTION ( 'NONE',  ( -0.9914448613738093830, 0.000000000000000000, -0.1305261922200583180 ) ) ;
#17208=CARTESIAN_POINT ( 'NONE',  ( 5.817157072110704874, 0.5000000000000004441, 13.82608706751090821 ) ) ;
#17211=CARTESIAN_POINT ( 'NONE',  ( 14.16423886937410082, 29.51208216824729291, -3.795296366450314096 ) ) ;
#17226=CARTESIAN_POINT ( 'NONE',  ( 9.972640495195376431, -0.03417435944610275333, -12.50695158660345818 ) ) ;
#17240=EDGE_CURVE ( 'NONE', #98676, #90778, #16025, .T. ) ;
#17244=ORIENTED_EDGE ( 'NONE', *, *, #92884, .F. ) ;
#17246=CARTESIAN_POINT ( 'NONE',  ( -5.817157072110618721, 15.00000000000000000, -13.82608706751094552 ) ) ;
#17247=LINE ( 'NONE', #29881, #46316 ) ;
#17254=CARTESIAN_POINT ( 'NONE',  ( 0.000000000000000000, 0.5000000000000004441, 0.000000000000000000 ) ) ;
#17257=CARTESIAN_POINT ( 'NONE',  ( -4.431036607602373500, 0.5000000000000004441, -14.33059365769916838 ) ) ;
#17258=CARTESIAN_POINT ( 'NONE',  ( -11.75209714983963849, 14.95077488074851502, -8.918201205062176840 ) ) ;
#17264=ORIENTED_EDGE ( 'NONE', *, *, #65835, .F. ) ;
#17271=CARTESIAN_POINT ( 'NONE',  ( -11.96291822454869802, 15.00000000000000000, -8.193813980849247613 ) ) ;
#17272=ORIENTED_EDGE ( 'NONE', *, *, #50576, .F. ) ;
#17273=AXIS2_PLACEMENT_3D ( 'NONE', #26219, #4218, #71720 ) ;
#17275=CARTESIAN_POINT ( 'NONE',  ( 3.434112377981060948, -4.418031996736250022, 12.81628187352647430 ) ) ;
#17280=ORIENTED_EDGE ( 'NONE', *, *, #54333, .T. ) ;
#17287=EDGE_CURVE ( 'NONE', #12526, #33705, #60654, .T. ) ;
#17289=CARTESIAN_POINT ( 'NONE',  ( -6.382347221874545617, 14.63606860869883164, 13.57444820018226217 ) ) ;
#17291=CARTESIAN_POINT ( 'NONE',  ( -14.49440716394870599, 15.00000000000000000, -0.4026921475168267484 ) ) ;
#17292=DIRECTION ( 'NONE',  ( 0.000000000000000000, 0.000000000000000000, 1.000000000000000000 ) ) ;
#17311=DIRECTION ( 'NONE',  ( -0.000000000000000000, -1.000000000000000000, -0.000000000000000000 ) ) ;
#17316=EDGE_CURVE ( 'NONE', #73495, #7776, #95837, .T. ) ;
#17321=AXIS2_PLACEMENT_3D ( 'NONE', #74925, #59420, #11102 ) ;
#17326=DIRECTION ( 'NONE',  ( 0.000000000000000000, 1.000000000000000000, 0.000000000000000000 ) ) ;
#17327=CARTESIAN_POINT ( 'NONE',  ( 11.62719953690058361, 0.5000000000000004441, 9.476720473301874392 ) ) ;
#17335=VERTEX_POINT ( 'NONE', #15674 ) ;
#17353=PLANE ( 'NONE',  #3208 ) ;
#17375=ADVANCED_FACE ( 'NONE', ( #60160 ), #93592, .T. ) ;
#17381=ORIENTED_EDGE ( 'NONE', *, *, #47163, .F. ) ;
#17393=EDGE_CURVE ( 'NONE', #12985, #24643, #12154, .T. ) ;
#17399=CARTESIAN_POINT ( 'NONE',  ( 8.209432707284918251, 14.49999999999999112, -12.55409154915490255 ) ) ;
#17403=CARTESIAN_POINT ( 'NONE',  ( 6.189644032515678518, 14.95077488074853456, 13.39157970158800204 ) ) ;
#17408=AXIS2_PLACEMENT_3D ( 'NONE', #11737, #26249, #95739 ) ;
#17410=DIRECTION ( 'NONE',  ( 0.000000000000000000, 0.000000000000000000, 1.000000000000000000 ) ) ;
#17415=ORIENTED_EDGE ( 'NONE', *, *, #4488, .T. ) ;
#17424=DIRECTION ( 'NONE',  ( 0.000000000000000000, 1.000000000000000000, 0.000000000000000000 ) ) ;
#17429=CARTESIAN_POINT ( 'NONE',  ( -2.849309504156474215, 0.000000000000000000, -4.649650521509827605 ) ) ;
#17432=CARTESIAN_POINT ( 'NONE',  ( -1.881645754503658452, 15.00000000000000533, -14.50406564081099603 ) ) ;
#17436=CARTESIAN_POINT ( 'NONE',  ( -12.50534872682737664, 4.247830340245585198E-16, 7.339363270777436554 ) ) ;
#17437=EDGE_CURVE ( 'NONE', #47708, #69540, #24883, .T. ) ;
#17444=AXIS2_PLACEMENT_3D ( 'NONE', #65032, #41094, #50052 ) ;
#17447=ORIENTED_EDGE ( 'NONE', *, *, #96429, .F. ) ;
#17453=CARTESIAN_POINT ( 'NONE',  ( 14.16423886937410259, -10.69625116508603213, -2.602085213965210642E-15 ) ) ;
#17456=ORIENTED_EDGE ( 'NONE', *, *, #53096, .T. ) ;
#17458=CARTESIAN_POINT ( 'NONE',  ( -10.93781366033333136, 15.00000000000000000, -10.26470809774080628 ) ) ;
#17488=DIRECTION ( 'NONE',  ( 0.000000000000000000, 0.000000000000000000, -1.000000000000000000 ) ) ;
#17490=ORIENTED_EDGE ( 'NONE', *, *, #28357, .F. ) ;
#17491=DIRECTION ( 'NONE',  ( 0.000000000000000000, 1.000000000000000000, 0.000000000000000000 ) ) ;
#17506=VERTEX_POINT ( 'NONE', #66299 ) ;
#17512=CARTESIAN_POINT ( 'NONE',  ( -13.07751017357388257, 4.569076162262063760E-16, 6.263284095430414311 ) ) ;
#17521=CARTESIAN_POINT ( 'NONE',  ( -8.527530157486182816, 30.59226448433413736, -4.923371831947288335 ) ) ;
#17531=EDGE_CURVE ( 'NONE', #59664, #77130, #21813, .T. ) ;
#17537=ORIENTED_EDGE ( 'NONE', *, *, #48650, .F. ) ;
#17540=DIRECTION ( 'NONE',  ( 0.000000000000000000, 1.000000000000000000, 0.000000000000000000 ) ) ;
#17547=ORIENTED_EDGE ( 'NONE', *, *, #76347, .T. ) ;
#17548=CARTESIAN_POINT ( 'NONE',  ( 5.817157072110708427, 14.49999999999999112, 13.82608706751097749 ) ) ;
#17550=EDGE_CURVE ( 'NONE', #48910, #4697, #81313, .T. ) ;
#17551=VERTEX_POINT ( 'NONE', #36309 ) ;
#17552=ORIENTED_EDGE ( 'NONE', *, *, #23066, .T. ) ;
#17556=ADVANCED_FACE ( 'NONE', ( #28311 ), #21312, .F. ) ;
#17562=ORIENTED_EDGE ( 'NONE', *, *, #40260, .T. ) ;
#17568=CARTESIAN_POINT ( 'NONE',  ( 0.000000000000000000, 14.49999999999999822, 0.000000000000000000 ) ) ;
#17570=DIRECTION ( 'NONE',  ( -0.9990482215818576872, 0.000000000000000000, -0.04361938736533987893 ) ) ;
#17582=CARTESIAN_POINT ( 'NONE',  ( -13.82192141328815715, 4.664367351173465489E-16, 4.382292601468585680 ) ) ;
#17586=CARTESIAN_POINT ( 'NONE',  ( 5.440088680355549045, 6.397018677488181204, -9.422509992056141925 ) ) ;
#17613=EDGE_CURVE ( 'NONE', #73208, #65699, #2560, .T. ) ;
#17623=LINE ( 'NONE', #23157, #73088 ) ;
#17629=DIRECTION ( 'NONE',  ( -0.000000000000000000, -1.000000000000000000, -0.000000000000000000 ) ) ;
#17631=VECTOR ( 'NONE', #46119, 999.9999999999998863 ) ;
#17632=CARTESIAN_POINT ( 'NONE',  ( 9.846743663894590881, -16.69940218233254470, 2.638427012816828565 ) ) ;
#17634=VERTEX_POINT ( 'NONE', #35311 ) ;
#17636=PLANE ( 'NONE',  #97215 ) ;
#17637=EDGE_CURVE ( 'NONE', #92892, #2722, #90280, .T. ) ;
#17638=AXIS2_PLACEMENT_3D ( 'NONE', #74696, #37698, #89696 ) ;
#17645=CARTESIAN_POINT ( 'NONE',  ( -14.24131928502210975, -0.03417435944610275333, -0.4973178280107823923 ) ) ;
#17647=EDGE_CURVE ( 'NONE', #71473, #36285, #79174, .T. ) ;
#17649=ADVANCED_FACE ( 'NONE', ( #82793 ), #91959, .T. ) ;
#17660=DIRECTION ( 'NONE',  ( 0.000000000000000000, 0.000000000000000000, -1.000000000000000000 ) ) ;
#17661=AXIS2_PLACEMENT_3D ( 'NONE', #34610, #5622, #64122 ) ;
#17664=ORIENTED_EDGE ( 'NONE', *, *, #83306, .F. ) ;
#17670=CARTESIAN_POINT ( 'NONE',  ( -1.881370533971078673, 6.047815243395702449E-16, -14.50512983964831371 ) ) ;
#17675=ORIENTED_EDGE ( 'NONE', *, *, #71490, .T. ) ;
#17684=CIRCLE ( 'NONE', #30432, 14.49999999999999822 ) ;
#17685=VERTEX_POINT ( 'NONE', #97326 ) ;
#17687=CARTESIAN_POINT ( 'NONE',  ( 6.869455772997054233, -0.03417435944610275333, 14.44603661281844431 ) ) ;
#17691=CARTESIAN_POINT ( 'NONE',  ( 5.084766917237454109, 13.12107973746817358, -10.74788037306357324 ) ) ;
#17692=CARTESIAN_POINT ( 'NONE',  ( 10.76445796112984787, -3.045506961852835686E-15, -9.901260316209842927 ) ) ;
#17693=CARTESIAN_POINT ( 'NONE',  ( -3.836325488036276266, 0.3639308251242951986, 14.50112432709423516 ) ) ;
#17698=CARTESIAN_POINT ( 'NONE',  ( 7.964842623401177768, -33.81131465584515894, -7.964842623401181321 ) ) ;
#17700=AXIS2_PLACEMENT_3D ( 'NONE', #13190, #43683, #59176 ) ;
#17709=ORIENTED_EDGE ( 'NONE', *, *, #37974, .F. ) ;
#17719=ORIENTED_EDGE ( 'NONE', *, *, #28572, .F. ) ;
#17727=CARTESIAN_POINT ( 'NONE',  ( -7.640985187756077046, 14.95037103177797633, -12.62032702733663392 ) ) ;
#17729=CIRCLE ( 'NONE', #59172, 15.00000000000000000 ) ;
#17731=CARTESIAN_POINT ( 'NONE',  ( -8.209432707284987529, 14.63606883728482622, 12.55409154915482972 ) ) ;
#17733=ORIENTED_EDGE ( 'NONE', *, *, #95494, .F. ) ;
#17750=CARTESIAN_POINT ( 'NONE',  ( -1.354709868695428421, 0.3639309939382821546, -14.93870011653156915 ) ) ;
#17751=( BOUNDED_CURVE ( )  B_SPLINE_CURVE ( 2, ( #87339, #27319, #81795, #12327, #88325, #88817, #42831, #81317, #4840, #36313, #41859 ),
 .UNSPECIFIED., .F., .T. ) 
 B_SPLINE_CURVE_WITH_KNOTS ( ( 3, 2, 2, 2, 2, 3 ),
 ( 0.6666666666666667407, 0.6722222222222223875, 0.6777777777777779233, 0.6833333333333333481, 0.6888888888888888840, 0.6902146981917277602 ),
 .UNSPECIFIED. ) 
 CURVE ( )  GEOMETRIC_REPRESENTATION_ITEM ( )  RATIONAL_B_SPLINE_CURVE ( ( 0.9999999999999993339, 0.9659258262890688673, 1.000000000000000000, 0.9659258262890682012, 1.000000000000000000, 0.9659258262890682012, 1.000000000000000000, 0.9659258262890682012, 1.000000000000000000, 0.9918683458313497514, 0.9876178598506348827 ) ) 
 REPRESENTATION_ITEM ( '' )  );
#17752=ORIENTED_EDGE ( 'NONE', *, *, #8025, .T. ) ;
#17755=ORIENTED_EDGE ( 'NONE', *, *, #21925, .T. ) ;
#17763=CARTESIAN_POINT ( 'NONE',  ( 9.382169495545415572, -7.751365330069575954, -9.382169495545422677 ) ) ;
#17765=ORIENTED_EDGE ( 'NONE', *, *, #50585, .F. ) ;
#17768=ORIENTED_EDGE ( 'NONE', *, *, #505, .T. ) ;
#17772=CARTESIAN_POINT ( 'NONE',  ( 6.382347221874334231, 0.5000000000000004441, 13.57444820018231724 ) ) ;
#17773=CARTESIAN_POINT ( 'NONE',  ( -8.375939845167836850, -0.03417435944610275333, 11.52849216984293257 ) ) ;
#17778=LINE ( 'NONE', #79250, #62745 ) ;
#17785=LINE ( 'NONE', #26740, #60113 ) ;
#17790=LINE ( 'NONE', #86281, #41736 ) ;
#17793=CARTESIAN_POINT ( 'NONE',  ( 13.48255862862752430, 15.00000000000000000, -5.335786055104087211 ) ) ;
#17812=( BOUNDED_CURVE ( )  B_SPLINE_CURVE ( 2, ( #46914, #45953, #39438, #53938, #45443, #76440, #69932, #8437, #69432 ),
 .UNSPECIFIED., .F., .F. ) 
 B_SPLINE_CURVE_WITH_KNOTS ( ( 3, 2, 2, 2, 3 ),
 ( 0.5817427861304426129, 0.5833333333333333703, 0.5888888888888889062, 0.5944444444444444420, 0.5999999999999999778 ),
 .UNSPECIFIED. ) 
 CURVE ( )  GEOMETRIC_REPRESENTATION_ITEM ( )  RATIONAL_B_SPLINE_CURVE ( ( 0.9860751345400187162, 0.9902446152963877424, 1.000000000000000000, 0.9659258262890684232, 1.000000000000000000, 0.9659258262890684232, 1.000000000000000000, 0.9659258262890684232, 1.000000000000000000 ) ) 
 REPRESENTATION_ITEM ( '' )  );
#17815=LINE ( 'NONE', #69837, #59235 ) ;
#17823=AXIS2_PLACEMENT_3D ( 'NONE', #27536, #96052, #97055 ) ;
#17828=DIRECTION ( 'NONE',  ( -0.9426414910921759871, 0.000000000000000000, -0.3338068592337775642 ) ) ;
#17838=CARTESIAN_POINT ( 'NONE',  ( 7.551349515323185990, 15.00000000000000000, -12.08468537022906020 ) ) ;
#17841=EDGE_CURVE ( 'NONE', #59148, #79187, #70926, .T. ) ;
#17858=ORIENTED_EDGE ( 'NONE', *, *, #82331, .T. ) ;
#17860=ORIENTED_EDGE ( 'NONE', *, *, #18879, .F. ) ;
#17863=B_SPLINE_CURVE_WITH_KNOTS ( 'NONE', 3,
 ( #83003, #52015, #44502, #21026, #51515, #67510 ),
 .UNSPECIFIED., .F., .F.,
 ( 4, 2, 4 ),
 ( 3.409110551496135434E-05, 0.0004400426677367878184, 0.0008459942299586143029 ),
 .UNSPECIFIED. ) ;
#17864=ORIENTED_EDGE ( 'NONE', *, *, #78014, .F. ) ;
#17866=AXIS2_PLACEMENT_3D ( 'NONE', #85251, #49206, #79214 ) ;
#17869=DIRECTION ( 'NONE',  ( -0.6755902076156541369, 0.000000000000000000, -0.7372773368101296354 ) ) ;
#17879=VERTEX_POINT ( 'NONE', #804 ) ;
#17883=CARTESIAN_POINT ( 'NONE',  ( -14.02068044289382875, 0.5000000000000004441, 5.331089937175565119 ) ) ;
#17887=CIRCLE ( 'NONE', #78629, 15.00000000000000000 ) ;
#17888=CIRCLE ( 'NONE', #89683, 15.00000000000000000 ) ;
#17890=EDGE_LOOP ( 'NONE', ( #22801, #7299, #65119, #43073, #9129, #6026 ) ) ;
#17893=AXIS2_PLACEMENT_3D ( 'NONE', #82302, #72828, #73325 ) ;
#17894=ORIENTED_EDGE ( 'NONE', *, *, #543, .F. ) ;
#17897=VECTOR ( 'NONE', #68488, 1000.000000000000227 ) ;
#17904=CARTESIAN_POINT ( 'NONE',  ( 0.000000000000000000, 0.5000000000000004441, 0.000000000000000000 ) ) ;
#17905=CARTESIAN_POINT ( 'NONE',  ( 13.21236992757670059, 15.00000000000000000, 5.338143956176803151 ) ) ;
#17906=EDGE_CURVE ( 'NONE', #94698, #21605, #66468, .T. ) ;
#17917=ORIENTED_EDGE ( 'NONE', *, *, #80043, .F. ) ;
#17919=CARTESIAN_POINT ( 'NONE',  ( -13.75801628063885040, 4.154966894009843400E-16, 4.578972376164368363 ) ) ;
#17930=CARTESIAN_POINT ( 'NONE',  ( 3.836325488036183451, 0.5000000000000004441, -14.50112432709422627 ) ) ;
#17933=CARTESIAN_POINT ( 'NONE',  ( -3.795296366450300773, 12.84541550158064283, 14.16423886937410437 ) ) ;
#17936=AXIS2_PLACEMENT_3D ( 'NONE', #76421, #8899, #62381 ) ;
#17947=DIRECTION ( 'NONE',  ( 0.000000000000000000, 1.000000000000000000, 0.000000000000000000 ) ) ;
#17950=PLANE ( 'NONE',  #20826 ) ;
#17959=EDGE_CURVE ( 'NONE', #90631, #8762, #48239, .T. ) ;
#17969=CARTESIAN_POINT ( 'NONE',  ( 0.000000000000000000, 14.49999999999999822, 0.000000000000000000 ) ) ;
#17970=VECTOR ( 'NONE', #89599, 1000.000000000000000 ) ;
#17972=EDGE_LOOP ( 'NONE', ( #43303, #574, #59057, #95117 ) ) ;
#17973=DIRECTION ( 'NONE',  ( 6.394884621840901673E-14, 0.000000000000000000, 1.000000000000000000 ) ) ;
#17977=TOROIDAL_SURFACE ( 'NONE', #446, 14.49999999999999822, 0.5000000000000000000 ) ;
#17993=CARTESIAN_POINT ( 'NONE',  ( 13.40508947812163143, 3.998652394537887614E-16, 5.527528931046191474 ) ) ;
#18000=EDGE_CURVE ( 'NONE', #91280, #15586, #71267, .T. ) ;
#18003=CARTESIAN_POINT ( 'NONE',  ( -9.382169495545422677, -31.50136533006957862, -9.382169495545417348 ) ) ;
#18004=VERTEX_POINT ( 'NONE', #17271 ) ;
#18014=ORIENTED_EDGE ( 'NONE', *, *, #32320, .F. ) ;
#18017=ORIENTED_EDGE ( 'NONE', *, *, #29705, .F. ) ;
#18023=EDGE_CURVE ( 'NONE', #24535, #60677, #71250, .T. ) ;
#18025=FILL_AREA_STYLE ('',( #3520 ) ) ;
#18032=ORIENTED_EDGE ( 'NONE', *, *, #45261, .F. ) ;
#18033=VERTEX_POINT ( 'NONE', #56724 ) ;
#18035=CIRCLE ( 'NONE', #22820, 14.49999999999999822 ) ;
#18038=TOROIDAL_SURFACE ( 'NONE', #8401, 14.49999999999999822, 0.5000000000000000000 ) ;
#18051=DIRECTION ( 'NONE',  ( 0.000000000000000000, 0.000000000000000000, 1.000000000000000000 ) ) ;
#18069=CARTESIAN_POINT ( 'NONE',  ( -10.88017736071110342, -1.936314655845157384, 3.903127820947815962E-15 ) ) ;
#18073=CARTESIAN_POINT ( 'NONE',  ( -13.34989199099671353, 0.04962897297196560559, -6.279943681065631722 ) ) ;
#18080=B_SPLINE_CURVE_WITH_KNOTS ( 'NONE', 3,
 ( #33894, #64399, #63428, #56907, #79903, #25459 ),
 .UNSPECIFIED., .F., .F.,
 ( 4, 2, 4 ),
 ( 0.0002800245631443565872, 0.0006862300328522100146, 0.001092435502560063550 ),
 .UNSPECIFIED. ) ;
#18081=CARTESIAN_POINT ( 'NONE',  ( 2.393480905993186969, 14.49999999999999112, -14.80781041047757185 ) ) ;
#18082=EDGE_CURVE ( 'NONE', #4700, #15469, #40258, .T. ) ;
#18083=EDGE_CURVE ( 'NONE', #7679, #49977, #24352, .T. ) ;
#18094=LINE ( 'NONE', #69123, #60538 ) ;
#18104=CARTESIAN_POINT ( 'NONE',  ( 2.849309504156442685, 0.000000000000000000, 4.649650521509849810 ) ) ;
#18117=AXIS2_PLACEMENT_3D ( 'NONE', #41649, #25177, #10159 ) ;
#18120=EDGE_CURVE ( 'NONE', #4498, #82904, #60573, .T. ) ;
#18122=CARTESIAN_POINT ( 'NONE',  ( -9.846743663894590881, -13.78273551566587862, 2.638427012816840111 ) ) ;
#18124=EDGE_LOOP ( 'NONE', ( #68296, #81325, #2818, #20406 ) ) ;
#18127=DIRECTION ( 'NONE',  ( 0.000000000000000000, 0.000000000000000000, 1.000000000000000000 ) ) ;
#18141=ORIENTED_EDGE ( 'NONE', *, *, #77829, .T. ) ;
#18143=ORIENTED_EDGE ( 'NONE', *, *, #97652, .F. ) ;
#18154=CARTESIAN_POINT ( 'NONE',  ( 11.48952521350018685, 4.805858850777305443E-16, 8.845383562533823962 ) ) ;
#18156=CARTESIAN_POINT ( 'NONE',  ( -11.81378540890925066, 15.00000000000000000, -7.968498874458281200 ) ) ;
#18157=CARTESIAN_POINT ( 'NONE',  ( 8.209432707284802788, 0.3639311627136676552, 12.55409154915494163 ) ) ;
#18159=LINE ( 'NONE', #42621, #78635 ) ;
#18169=ORIENTED_EDGE ( 'NONE', *, *, #33841, .T. ) ;
#18175=DIRECTION ( 'NONE',  ( 0.4461978131098069400, 0.000000000000000000, -0.8949343616020258851 ) ) ;
#18176=AXIS2_PLACEMENT_3D ( 'NONE', #84984, #92477, #76987 ) ;
#18177=CARTESIAN_POINT ( 'NONE',  ( -14.91886229468047986, 14.76984964723649973, -0.8060919667646749831 ) ) ;
#18181=CARTESIAN_POINT ( 'NONE',  ( -5.440088680355558814, -32.76964798917848753, -9.422509992056136596 ) ) ;
#18192=ADVANCED_FACE ( 'NONE', ( #57699 ), #96715, .F. ) ;
#18200=EDGE_CURVE ( 'NONE', #43658, #68070, #44799, .T. ) ;
#18216=ORIENTED_EDGE ( 'NONE', *, *, #11642, .T. ) ;
#18218=VERTEX_POINT ( 'NONE', #27696 ) ;
#18219=DIRECTION ( 'NONE',  ( -0.000000000000000000, -1.000000000000000000, -0.000000000000000000 ) ) ;
#18225=LINE ( 'NONE', #48214, #7183 ) ;
#18230=DIRECTION ( 'NONE',  ( 0.000000000000000000, 1.000000000000000000, 0.000000000000000000 ) ) ;
#18236=ORIENTED_EDGE ( 'NONE', *, *, #1305, .F. ) ;
#18237=FACE_OUTER_BOUND ( 'NONE', #85765, .T. ) ;
#18238=ORIENTED_EDGE ( 'NONE', *, *, #73708, .T. ) ;
#18247=ORIENTED_EDGE ( 'NONE', *, *, #29663, .T. ) ;
#18249=CARTESIAN_POINT ( 'NONE',  ( -5.204170427930421283E-15, -7.126365330069578619, -12.81628187352647608 ) ) ;
#18254=VECTOR ( 'NONE', #25206, 999.9999999999998863 ) ;
#18258=CARTESIAN_POINT ( 'NONE',  ( -8.134956207566176545, 15.00000000000000000, 13.77315809598633756 ) ) ;
#18260=CARTESIAN_POINT ( 'NONE',  ( -4.746257547686221656, 0.000000000000000000, 2.685303318749045154 ) ) ;
#18265=CARTESIAN_POINT ( 'NONE',  ( 11.22915323889574601, -0.03417435944610275333, 8.773176023390684364 ) ) ;
#18279=CARTESIAN_POINT ( 'NONE',  ( 9.876730923139225737, 15.00000000000000000, 11.28938378619069560 ) ) ;
#18280=CIRCLE ( 'NONE', #58366, 15.00000000000000000 ) ;
#18281=EDGE_CURVE ( 'NONE', #86312, #4683, #68578, .T. ) ;
#18296=CARTESIAN_POINT ( 'NONE',  ( 10.70613742633258170, 4.237152514796235822E-16, -9.778988772285240216 ) ) ;
#18301=CARTESIAN_POINT ( 'NONE',  ( -12.60589901313211492, 14.63595249122789177, -8.129656208642225934 ) ) ;
#18303=B_SPLINE_CURVE_WITH_KNOTS ( 'NONE', 3,
 ( #88437, #80939, #12432, #4947, #42940, #35428 ),
 .UNSPECIFIED., .F., .F.,
 ( 4, 2, 4 ),
 ( 0.0002800047503720793978, 0.0006862100262544194602, 0.001092415302136759414 ),
 .UNSPECIFIED. ) ;
#18305=CARTESIAN_POINT ( 'NONE',  ( 11.62719953690060137, 14.63606895804700514, 9.476720473301911696 ) ) ;
#18306=ORIENTED_EDGE ( 'NONE', *, *, #93228, .T. ) ;
#18312=CARTESIAN_POINT ( 'NONE',  ( 5.419894505350494107, 14.63595249122791664, 13.98659156302463025 ) ) ;
#18314=EDGE_CURVE ( 'NONE', #83450, #98073, #82173, .T. ) ;
#18319=ORIENTED_EDGE ( 'NONE', *, *, #42103, .T. ) ;
#18320=LINE ( 'NONE', #9838, #52613 ) ;
#18326=CARTESIAN_POINT ( 'NONE',  ( -7.684764310694707667, 0.5000000000000004441, -12.88194075009945472 ) ) ;
#18341=EDGE_CURVE ( 'NONE', #57109, #72221, #81556, .T. ) ;
#18347=FACE_OUTER_BOUND ( 'NONE', #73572, .T. ) ;
#18349=EDGE_CURVE ( 'NONE', #18961, #16062, #74681, .T. ) ;
#18352=VERTEX_POINT ( 'NONE', #28682 ) ;
#18356=CIRCLE ( 'NONE', #59881, 14.49999999999999822 ) ;
#18369=ORIENTED_EDGE ( 'NONE', *, *, #37323, .F. ) ;
#18371=ORIENTED_EDGE ( 'NONE', *, *, #25344, .F. ) ;
#18372=CARTESIAN_POINT ( 'NONE',  ( -10.14667048435130781, 4.359436697371537845E-16, -10.35833375027055148 ) ) ;
#18377=CARTESIAN_POINT ( 'NONE',  ( -13.55255535720598026, 15.00000000000000000, 4.403492169842870396 ) ) ;
#18381=PRODUCT_DEFINITION_FORMATION_WITH_SPECIFIED_SOURCE ( 'ANY', '', #5926, .NOT_KNOWN. ) ;
#18383=ORIENTED_EDGE ( 'NONE', *, *, #36481, .F. ) ;
#18387=VERTEX_POINT ( 'NONE', #81675 ) ;
#18392=CARTESIAN_POINT ( 'NONE',  ( -14.71525861348289510, 14.63606890215620915, -2.908807992686800237 ) ) ;
#18393=LINE ( 'NONE', #55407, #72679 ) ;
#18394=ADVANCED_FACE ( 'NONE', ( #19709 ), #35696, .T. ) ;
#18406=ORIENTED_EDGE ( 'NONE', *, *, #19779, .T. ) ;
#18407=DIRECTION ( 'NONE',  ( 0.000000000000000000, 0.000000000000000000, 1.000000000000000000 ) ) ;
#18414=CARTESIAN_POINT ( 'NONE',  ( -13.78891971893215107, 0.3639314269420583781, 5.904717858191459889 ) ) ;
#18423=CARTESIAN_POINT ( 'NONE',  ( 14.16423886937410082, 4.512082168247307123, -3.795296366450314096 ) ) ;
#18425=LINE ( 'NONE', #79424, #67319 ) ;
#18426=ADVANCED_FACE ( 'NONE', ( #66180 ), #13686, .T. ) ;
#18427=ORIENTED_EDGE ( 'NONE', *, *, #95849, .F. ) ;
#18436=CARTESIAN_POINT ( 'NONE',  ( 11.29168986245494644, 14.76984976272934169, -9.783658503027382380 ) ) ;
#18442=DIRECTION ( 'NONE',  ( -0.3665012267243009103, 0.000000000000000000, 0.9304175679820231304 ) ) ;
#18446=CARTESIAN_POINT ( 'NONE',  ( -13.03370038005733456, -0.03417435944610275333, 9.273621236547603175 ) ) ;
#18452=VECTOR ( 'NONE', #62589, 1000.000000000000000 ) ;
#18459=ORIENTED_EDGE ( 'NONE', *, *, #7012, .T. ) ;
#18487=CARTESIAN_POINT ( 'NONE',  ( 11.09922568453594671, -32.95969866340291077, -6.408140936763241591 ) ) ;
#18496=VECTOR ( 'NONE', #68717, 1000.000000000000000 ) ;
#18498=VERTEX_POINT ( 'NONE', #65193 ) ;
#18511=DIRECTION ( 'NONE',  ( 0.2334453638559024768, -0.000000000000000000, 0.9723699203976773342 ) ) ;
#18517=FACE_OUTER_BOUND ( 'NONE', #46570, .T. ) ;
#18519=VERTEX_POINT ( 'NONE', #96213 ) ;
#18540=CARTESIAN_POINT ( 'NONE',  ( 10.36894250292379027, -36.32125116508603213, 10.36894250292378672 ) ) ;
#18544=ORIENTED_EDGE ( 'NONE', *, *, #98083, .F. ) ;
#18551=FACE_OUTER_BOUND ( 'NONE', #86699, .T. ) ;
#18558=CARTESIAN_POINT ( 'NONE',  ( -10.88017736071109987, 13.27201867748817321, 2.915334737309934532 ) ) ;
#18562=CIRCLE ( 'NONE', #92001, 15.00000000000000000 ) ;
#18570=CIRCLE ( 'NONE', #37899, 14.49999999999999822 ) ;
#18574=DIRECTION ( 'NONE',  ( 0.000000000000000000, 0.000000000000000000, 1.000000000000000000 ) ) ;
#18576=ORIENTED_EDGE ( 'NONE', *, *, #49716, .F. ) ;
#18585=DIRECTION ( 'NONE',  ( 0.000000000000000000, 0.000000000000000000, 1.000000000000000000 ) ) ;
#18587=AXIS2_PLACEMENT_3D ( 'NONE', #78298, #17326, #857 ) ;
#18590=DIRECTION ( 'NONE',  ( 0.000000000000000000, 1.000000000000000000, 0.000000000000000000 ) ) ;
#18601=VECTOR ( 'NONE', #93768, 1000.000000000000000 ) ;
#18604=EDGE_CURVE ( 'NONE', #51781, #49599, #91128, .T. ) ;
#18605=CARTESIAN_POINT ( 'NONE',  ( -9.846743663894596210, 0.8005978176674529712, -2.638427012816824124 ) ) ;
#18610=EDGE_LOOP ( 'NONE', ( #28303, #20056, #41229, #20580 ) ) ;
#18617=VECTOR ( 'NONE', #37244, 1000.000000000000000 ) ;
#18620=VERTEX_POINT ( 'NONE', #38660 ) ;
#18622=ORIENTED_EDGE ( 'NONE', *, *, #55648, .F. ) ;
#18629=B_SPLINE_CURVE_WITH_KNOTS ( 'NONE', 3,
 ( #45657, #76153, #186, #20695, #81669, #36685 ),
 .UNSPECIFIED., .F., .F.,
 ( 4, 2, 4 ),
 ( 1.825722095103865762E-18, 0.0004057005074147820617, 0.0008114010148295622803 ),
 .UNSPECIFIED. ) ;
#18639=CARTESIAN_POINT ( 'NONE',  ( -14.37657372141814172, 2.117582368135750848E-16, -2.693041920167547065 ) ) ;
#18647=DIRECTION ( 'NONE',  ( 0.000000000000000000, 1.000000000000000000, 0.000000000000000000 ) ) ;
#18651=EDGE_CURVE ( 'NONE', #94563, #89588, #36193, .T. ) ;
#18653=VECTOR ( 'NONE', #29346, 999.9999999999998863 ) ;
#18659=CARTESIAN_POINT ( 'NONE',  ( 0.000000000000000000, 14.49999999999999822, 0.000000000000000000 ) ) ;
#18670=CARTESIAN_POINT ( 'NONE',  ( 0.000000000000000000, 14.49999999999999822, 0.000000000000000000 ) ) ;
#18671=CARTESIAN_POINT ( 'NONE',  ( 8.722765153436348839, 2.185345003916094875E-16, -11.74102699209685952 ) ) ;
#18674=CARTESIAN_POINT ( 'NONE',  ( -2.915334737309917656, -20.89464798917849109, 10.88017736071110164 ) ) ;
#18687=B_SPLINE_CURVE_WITH_KNOTS ( 'NONE', 3,
 ( #50852, #81345, #12841, #66332, #28344, #96868 ),
 .UNSPECIFIED., .F., .F.,
 ( 4, 2, 4 ),
 ( 0.0002800671705680389686, 0.0006862730573397217773, 0.001092478944111404749 ),
 .UNSPECIFIED. ) ;
#18697=ORIENTED_EDGE ( 'NONE', *, *, #64388, .F. ) ;
#18705=CARTESIAN_POINT ( 'NONE',  ( -10.19513985507843223, 14.49999999999999112, 11.00268709613216522 ) ) ;
#18708=EDGE_CURVE ( 'NONE', #36109, #17879, #25694, .T. ) ;
#18711=VERTEX_POINT ( 'NONE', #71623 ) ;
#18713=CARTESIAN_POINT ( 'NONE',  ( 6.336100170400826848, 0.2301512019179773050, 13.53056138701891875 ) ) ;
#18719=PLANE ( 'NONE',  #24333 ) ;
#18726=CARTESIAN_POINT ( 'NONE',  ( 0.000000000000000000, 0.000000000000000000, 0.000000000000000000 ) ) ;
#18727=DIRECTION ( 'NONE',  ( 0.000000000000000000, 0.000000000000000000, 1.000000000000000000 ) ) ;
#18730=CARTESIAN_POINT ( 'NONE',  ( -2.638427012816824124, -37.94940218233255536, 9.846743663894596210 ) ) ;
#18731=VERTEX_POINT ( 'NONE', #24157 ) ;
#18732=DIRECTION ( 'NONE',  ( -0.000000000000000000, 1.000000000000000000, 0.000000000000000000 ) ) ;
#18733=EDGE_LOOP ( 'NONE', ( #43787, #30943, #90788, #12390, #90064, #75776 ) ) ;
#18735=VERTEX_POINT ( 'NONE', #2166 ) ;
#18739=CARTESIAN_POINT ( 'NONE',  ( 4.746257547686200340, 0.000000000000000000, -2.685303318749077572 ) ) ;
#18743=CARTESIAN_POINT ( 'NONE',  ( -3.434112377981047626, -4.834698663402913432, 12.81628187352647963 ) ) ;
#18744=EDGE_LOOP ( 'NONE', ( #84254, #70225, #13266, #95093 ) ) ;
#18746=ORIENTED_EDGE ( 'NONE', *, *, #15413, .F. ) ;
#18747=VERTEX_POINT ( 'NONE', #25156 ) ;
#18749=AXIS2_PLACEMENT_3D ( 'NONE', #47738, #9748, #55237 ) ;
#18755=VECTOR ( 'NONE', #47662, 1000.000000000000000 ) ;
#18761=LINE ( 'NONE', #18265, #97892 ) ;
#18763=LINE ( 'NONE', #57229, #66843 ) ;
#18765=EDGE_CURVE ( 'NONE', #57516, #14429, #40635, .T. ) ;
#18774=CARTESIAN_POINT ( 'NONE',  ( 7.684764310694791156, 0.5000000000000004441, 12.88194075009940498 ) ) ;
#18789=EDGE_CURVE ( 'NONE', #7347, #21745, #14800, .T. ) ;
#18792=CYLINDRICAL_SURFACE ( 'NONE', #30739, 15.00000000000000000 ) ;
#18795=CARTESIAN_POINT ( 'NONE',  ( 0.000000000000000000, 14.49999999999999822, 0.000000000000000000 ) ) ;
#18799=CARTESIAN_POINT ( 'NONE',  ( 11.42891328973218279, 15.00000000000000533, 9.126250717928463985 ) ) ;
#18800=ORIENTED_EDGE ( 'NONE', *, *, #88065, .F. ) ;
#18803=CARTESIAN_POINT ( 'NONE',  ( -3.927832320392065313, 0.000000000000000000, -13.69797916712109398 ) ) ;
#18813=CARTESIAN_POINT ( 'NONE',  ( -0.3093388210927633941, 15.00000000000000000, -14.99680997725065978 ) ) ;
#18824=CARTESIAN_POINT ( 'NONE',  ( -14.88232117145532918, 14.63595249122789177, 1.875237731503045735 ) ) ;
#18829=CIRCLE ( 'NONE', #69931, 14.49999999999999822 ) ;
#18834=DIRECTION ( 'NONE',  ( 0.000000000000000000, 0.000000000000000000, 1.000000000000000000 ) ) ;
#18843=ORIENTED_EDGE ( 'NONE', *, *, #58466, .F. ) ;
#18854=CARTESIAN_POINT ( 'NONE',  ( -5.240693273019180864, 14.95037116783537456, 13.79102773477909949 ) ) ;
#18855=DIRECTION ( 'NONE',  ( 0.000000000000000000, 1.000000000000000000, 0.000000000000000000 ) ) ;
#18862=VERTEX_POINT ( 'NONE', #64091 ) ;
#18869=CARTESIAN_POINT ( 'NONE',  ( -6.699646882363181177, 1.931786074955269106, -9.748952036344858740 ) ) ;
#18872=ADVANCED_FACE ( 'NONE', ( #70638 ), #32621, .T. ) ;
#18879=EDGE_CURVE ( 'NONE', #47627, #59056, #63119, .T. ) ;
#18888=CARTESIAN_POINT ( 'NONE',  ( 13.82192141328812518, 4.718101003023380916E-16, -4.382292601468683380 ) ) ;
#18892=CARTESIAN_POINT ( 'NONE',  ( 0.8649609010932225450, -2.354751593366952970E-16, 14.60103384664012260 ) ) ;
#18895=ORIENTED_EDGE ( 'NONE', *, *, #13609, .F. ) ;
#18902=CARTESIAN_POINT ( 'NONE',  ( 8.235571585149870089, 6.993033628982647798, 8.235571585149868312 ) ) ;
#18905=DIRECTION ( 'NONE',  ( 0.000000000000000000, 1.000000000000000000, 0.000000000000000000 ) ) ;
#18912=CARTESIAN_POINT ( 'NONE',  ( 12.60589901313225702, 14.63606915354311155, -8.129656208642060733 ) ) ;
#18913=DIRECTION ( 'NONE',  ( -0.000000000000000000, -1.000000000000000000, -0.000000000000000000 ) ) ;
#18915=ORIENTED_EDGE ( 'NONE', *, *, #64585, .F. ) ;
#18919=DIRECTION ( 'NONE',  ( 0.3173046564051030805, 0.000000000000000000, -0.9483236552061955482 ) ) ;
#18920=EDGE_CURVE ( 'NONE', #78138, #42602, #55319, .T. ) ;
#18929=CARTESIAN_POINT ( 'NONE',  ( -13.82192141328803991, 15.00000000000000000, -4.382292601468865456 ) ) ;
#18937=DIRECTION ( 'NONE',  ( -0.9799247046208311440, 0.000000000000000000, 0.1993679344171901680 ) ) ;
#18952=CARTESIAN_POINT ( 'NONE',  ( -4.841283923550532720, 14.76930270348881002, 14.13506365971143808 ) ) ;
#18953=ORIENTED_EDGE ( 'NONE', *, *, #35093, .T. ) ;
#18954=DIRECTION ( 'NONE',  ( -0.7132504491541848957, 0.000000000000000000, 0.7009092642998474565 ) ) ;
#18955=DIRECTION ( 'NONE',  ( -0.7604059656000340395, 0.000000000000000000, 0.6494480483301798834 ) ) ;
#18961=VERTEX_POINT ( 'NONE', #79608 ) ;
#18971=FACE_OUTER_BOUND ( 'NONE', #35689, .T. ) ;
#18982=CARTESIAN_POINT ( 'NONE',  ( -12.81628187352647608, -30.87636533006957507, 3.903127820947815962E-15 ) ) ;
#18993=EDGE_CURVE ( 'NONE', #51268, #9175, #58569, .T. ) ;
#18995=ORIENTED_EDGE ( 'NONE', *, *, #22814, .T. ) ;
#19007=CARTESIAN_POINT ( 'NONE',  ( -4.096035146099030300, 15.00000000000000000, 13.90943910019935714 ) ) ;
#19012=ORIENTED_EDGE ( 'NONE', *, *, #50734, .T. ) ;
#19015=ORIENTED_EDGE ( 'NONE', *, *, #16283, .F. ) ;
#19016=ORIENTED_EDGE ( 'NONE', *, *, #27881, .F. ) ;
#19018=CARTESIAN_POINT ( 'NONE',  ( 2.258855624577543075, 0.04962891015807205375, 14.57926203528951881 ) ) ;
#19022=DIRECTION ( 'NONE',  ( 0.6626200482157461602, 0.000000000000000000, -0.7489557207889945278 ) ) ;
#19024=LINE ( 'NONE', #3540, #46644 ) ;
#19034=AXIS2_PLACEMENT_3D ( 'NONE', #75193, #74194, #81701 ) ;
#19035=CARTESIAN_POINT ( 'NONE',  ( -14.16423886937410437, -38.40458449841935362, -3.795296366450299885 ) ) ;
#19038=ORIENTED_EDGE ( 'NONE', *, *, #94988, .F. ) ;
#19045=CARTESIAN_POINT ( 'NONE',  ( 0.000000000000000000, 14.49999999999999822, 0.000000000000000000 ) ) ;
#19050=CARTESIAN_POINT ( 'NONE',  ( 7.964842623401177768, 21.18868534415484106, -7.964842623401181321 ) ) ;
#19062=CARTESIAN_POINT ( 'NONE',  ( -9.065164099344372062, 14.49999999999999822, -11.95084933600779742 ) ) ;
#19064=ORIENTED_EDGE ( 'NONE', *, *, #46893, .F. ) ;
#19073=CARTESIAN_POINT ( 'NONE',  ( 2.962741594152983993, -0.03417435944610275333, 13.93860331045674883 ) ) ;
#19077=CARTESIAN_POINT ( 'NONE',  ( -9.402796353261203777, 0.5000000000000004441, 11.68706210897750708 ) ) ;
#19079=ORIENTED_EDGE ( 'NONE', *, *, #48113, .T. ) ;
#19091=CARTESIAN_POINT ( 'NONE',  ( 8.527530157486179263, -1.907735515665878623, 4.923371831947292776 ) ) ;
#19092=EDGE_LOOP ( 'NONE', ( #69382, #6794, #62359, #921 ) ) ;
#19104=ORIENTED_EDGE ( 'NONE', *, *, #21862, .T. ) ;
#19108=CIRCLE ( 'NONE', #65421, 14.49999999999999822 ) ;
#19114=AXIS2_PLACEMENT_3D ( 'NONE', #96441, #58910, #20924 ) ;
#19116=ORIENTED_EDGE ( 'NONE', *, *, #68231, .F. ) ;
#19118=ORIENTED_EDGE ( 'NONE', *, *, #61724, .T. ) ;
#19134=B_SPLINE_CURVE_WITH_KNOTS ( 'NONE', 3,
 ( #36850, #12365, #73848, #34862, #58845, #5378 ),
 .UNSPECIFIED., .F., .F.,
 ( 4, 2, 4 ),
 ( 3.409110551494645334E-05, 0.0004400426677367917216, 0.0008459942299586370711 ),
 .UNSPECIFIED. ) ;
#19135=CARTESIAN_POINT ( 'NONE',  ( -0.4278561937607772148, 0.000000000000000000, -5.436428395565747529 ) ) ;
#19140=EDGE_CURVE ( 'NONE', #48484, #28000, #54220, .T. ) ;
#19144=CYLINDRICAL_SURFACE ( 'NONE', #20361, 11.92686044187656513 ) ;
#19151=CARTESIAN_POINT ( 'NONE',  ( 11.25483282072091384, 12.52949842971371908, 1.007928381667628326 ) ) ;
#19157=CARTESIAN_POINT ( 'NONE',  ( -2.915334737309917656, -30.89464798917849109, 10.88017736071110164 ) ) ;
#19161=CARTESIAN_POINT ( 'NONE',  ( 13.07907619356932827, 14.76984992095085758, -7.222187741820672358 ) ) ;
#19162=CARTESIAN_POINT ( 'NONE',  ( 0.000000000000000000, 14.49999999999999822, 0.000000000000000000 ) ) ;
#19172=PLANE ( 'NONE',  #74293 ) ;
#19177=CARTESIAN_POINT ( 'NONE',  ( 0.000000000000000000, 0.5000000000000004441, 0.000000000000000000 ) ) ;
#19184=DIRECTION ( 'NONE',  ( -0.000000000000000000, -1.000000000000000000, -0.000000000000000000 ) ) ;
#19186=VECTOR ( 'NONE', #33722, 1000.000000000000000 ) ;
#19188=ADVANCED_FACE ( 'NONE', ( #87905 ), #36895, .T. ) ;
#19191=ORIENTED_EDGE ( 'NONE', *, *, #71070, .F. ) ;
#19193=DIRECTION ( 'NONE',  ( 0.000000000000000000, 0.000000000000000000, 1.000000000000000000 ) ) ;
#19203=ADVANCED_FACE ( 'NONE', ( #35398 ), #89337, .T. ) ;
#19209=DIRECTION ( 'NONE',  ( 0.000000000000000000, 1.000000000000000000, 0.000000000000000000 ) ) ;
#19211=FACE_OUTER_BOUND ( 'NONE', #93001, .T. ) ;
#19214=ORIENTED_EDGE ( 'NONE', *, *, #16157, .T. ) ;
#19221=ADVANCED_FACE ( 'NONE', ( #57412 ), #50899, .F. ) ;
#19223=CARTESIAN_POINT ( 'NONE',  ( -12.81628187352647963, 8.915301336597083903, -3.434112377981046293 ) ) ;
#19236=AXIS2_PLACEMENT_3D ( 'NONE', #29136, #59641, #68146 ) ;
#19237=CARTESIAN_POINT ( 'NONE',  ( 14.66196617519559808, 14.76930270348881002, -2.874856965127823294 ) ) ;
#19240=CARTESIAN_POINT ( 'NONE',  ( 1.796645268984721877, 14.76930270348881180, -14.83273813124059082 ) ) ;
#19243=LINE ( 'NONE', #12227, #67426 ) ;
#19250=CARTESIAN_POINT ( 'NONE',  ( 7.595945211628243321, 4.245086020036709294E-16, 12.35117874301647056 ) ) ;
#19253=DIRECTION ( 'NONE',  ( -0.8870108331782182720, 0.000000000000000000, -0.4617486132350404615 ) ) ;
#19271=AXIS2_PLACEMENT_3D ( 'NONE', #29602, #44110, #68124 ) ;
#19276=CIRCLE ( 'NONE', #43252, 14.49999999999999822 ) ;
#19281=VECTOR ( 'NONE', #66098, 1000.000000000000000 ) ;
#19282=DIRECTION ( 'NONE',  ( 0.5948227867513318223, 0.000000000000000000, 0.8038568606172245001 ) ) ;
#19305=FACE_OUTER_BOUND ( 'NONE', #16743, .T. ) ;
#19308=AXIS2_PLACEMENT_3D ( 'NONE', #76314, #7832, #38328 ) ;
#19318=EDGE_CURVE ( 'NONE', #48243, #84680, #88409, .T. ) ;
#19320=LINE ( 'NONE', #27796, #3960 ) ;
#19333=DIRECTION ( 'NONE',  ( 0.000000000000000000, 1.000000000000000000, 0.000000000000000000 ) ) ;
#19339=CARTESIAN_POINT ( 'NONE',  ( 13.78891971893208357, 15.00000000000000000, -5.904717858191528279 ) ) ;
#19340=DIRECTION ( 'NONE',  ( 0.000000000000000000, 0.000000000000000000, 1.000000000000000000 ) ) ;
#19347=EDGE_CURVE ( 'NONE', #53389, #51268, #80910, .T. ) ;
#19349=VERTEX_POINT ( 'NONE', #96421 ) ;
#19354=CARTESIAN_POINT ( 'NONE',  ( -13.48255862861917009, 15.00000000000000000, -5.335786055104346559 ) ) ;
#19357=AXIS2_PLACEMENT_3D ( 'NONE', #97894, #14881, #82862 ) ;
#19358=AXIS2_PLACEMENT_3D ( 'NONE', #53333, #38842, #83842 ) ;
#19359=AXIS2_PLACEMENT_3D ( 'NONE', #67003, #44981, #67501 ) ;
#19363=B_SPLINE_CURVE_WITH_KNOTS ( 'NONE', 3,
 ( #88772, #97288, #89268, #79797, #66259, #11789 ),
 .UNSPECIFIED., .F., .F.,
 ( 4, 2, 4 ),
 ( 3.409110551495833213E-05, 0.0004400426677367820722, 0.0008459942299586057377 ),
 .UNSPECIFIED. ) ;
#19370=LINE ( 'NONE', #11864, #45227 ) ;
#19380=VERTEX_POINT ( 'NONE', #58384 ) ;
#19386=CARTESIAN_POINT ( 'NONE',  ( 8.549892366338843530, 14.76930270348882068, -12.25305656628354534 ) ) ;
#19392=DIRECTION ( 'NONE',  ( 0.000000000000000000, 1.000000000000000000, 0.000000000000000000 ) ) ;
#19395=DIRECTION ( 'NONE',  ( 0.000000000000000000, 0.000000000000000000, 1.000000000000000000 ) ) ;
#19398=EDGE_CURVE ( 'NONE', #18711, #76195, #86210, .T. ) ;
#19401=LINE ( 'NONE', #25924, #82555 ) ;
#19406=CARTESIAN_POINT ( 'NONE',  ( -14.73513795193454534, 14.95077488074854166, 0.7223639599945808065 ) ) ;
#19413=ORIENTED_EDGE ( 'NONE', *, *, #23514, .T. ) ;
#19420=CARTESIAN_POINT ( 'NONE',  ( 4.391700990647163572, 0.2306972965111900586, -14.28114200970190240 ) ) ;
#19432=AXIS2_PLACEMENT_3D ( 'NONE', #12874, #35384, #49889 ) ;
#19435=EDGE_CURVE ( 'NONE', #38291, #3216, #405, .T. ) ;
#19440=ORIENTED_EDGE ( 'NONE', *, *, #41900, .F. ) ;
#19448=ORIENTED_EDGE ( 'NONE', *, *, #44600, .F. ) ;
#19451=CARTESIAN_POINT ( 'NONE',  ( 6.382347221874430154, 0.3640475087720987935, -13.57444820018227638 ) ) ;
#19454=ORIENTED_EDGE ( 'NONE', *, *, #70118, .T. ) ;
#19460=DIRECTION ( 'NONE',  ( -0.000000000000000000, -1.000000000000000000, -0.000000000000000000 ) ) ;
#19467=AXIS2_PLACEMENT_3D ( 'NONE', #91791, #68310, #77266 ) ;
#19468=EDGE_CURVE ( 'NONE', #97173, #9609, #39889, .T. ) ;
#19470=CARTESIAN_POINT ( 'NONE',  ( -5.204170427930421283E-15, -37.12636533006957507, -12.81628187352647608 ) ) ;
#19471=CIRCLE ( 'NONE', #72126, 14.49999999999999822 ) ;
#19498=ORIENTED_EDGE ( 'NONE', *, *, #75080, .F. ) ;
#19503=DIRECTION ( 'NONE',  ( 0.8241261886220166977, 0.000000000000000000, 0.5664062369248314965 ) ) ;
#19506=EDGE_CURVE ( 'NONE', #28808, #23105, #67383, .T. ) ;
#19510=LINE ( 'NONE', #95511, #37183 ) ;
#19511=ORIENTED_EDGE ( 'NONE', *, *, #66083, .T. ) ;
#19518=EDGE_CURVE ( 'NONE', #72221, #73524, #30155, .T. ) ;
#19521=CARTESIAN_POINT ( 'NONE',  ( 7.082119434687047743, -34.86291783175269643, -12.26659068614894821 ) ) ;
#19522=VECTOR ( 'NONE', #55772, 1000.000000000000000 ) ;
#19536=CARTESIAN_POINT ( 'NONE',  ( 2.915334737309928315, 19.52201867748817676, 10.88017736071109987 ) ) ;
#19545=EDGE_CURVE ( 'NONE', #21360, #83033, #20608, .T. ) ;
#19548=EDGE_CURVE ( 'NONE', #68154, #57109, #62383, .T. ) ;
#19556=DIRECTION ( 'NONE',  ( 0.000000000000000000, 0.000000000000000000, 1.000000000000000000 ) ) ;
#19560=AXIS2_PLACEMENT_3D ( 'NONE', #90433, #37964, #52451 ) ;
#19564=CARTESIAN_POINT ( 'NONE',  ( -6.767445849361333643, 15.00000000000000000, 13.38662304974491946 ) ) ;
#19567=ORIENTED_EDGE ( 'NONE', *, *, #61050, .T. ) ;
#19574=PLANE ( 'NONE',  #29080 ) ;
#19577=EDGE_CURVE ( 'NONE', #89199, #14221, #95768, .T. ) ;
#19580=EDGE_CURVE ( 'NONE', #14459, #88316, #19108, .T. ) ;
#19581=CARTESIAN_POINT ( 'NONE',  ( -8.527530157486182816, 0.5922644843341234866, -4.923371831947288335 ) ) ;
#19584=CARTESIAN_POINT ( 'NONE',  ( 0.000000000000000000, 1.823139558123437975, -11.92686044187656513 ) ) ;
#19585=EDGE_LOOP ( 'NONE', ( #17280, #98562, #40593, #62034 ) ) ;
#19591=VECTOR ( 'NONE', #81400, 1000.000000000000000 ) ;
#19599=VECTOR ( 'NONE', #53910, 999.9999999999998863 ) ;
#19607=CARTESIAN_POINT ( 'NONE',  ( 1.354709868695624264, 0.3640475087720588809, -14.93870011653152297 ) ) ;
#19610=ORIENTED_EDGE ( 'NONE', *, *, #77114, .T. ) ;
#19616=FACE_OUTER_BOUND ( 'NONE', #34703, .T. ) ;
#19621=CARTESIAN_POINT ( 'NONE',  ( 12.25993886608601890, 14.63606888159244512, 8.642563219313739609 ) ) ;
#19623=CARTESIAN_POINT ( 'NONE',  ( 0.000000000000000000, 15.00000000000000000, 0.000000000000000000 ) ) ;
#19629=EDGE_CURVE ( 'NONE', #15586, #78552, #7881, .T. ) ;
#19630=CARTESIAN_POINT ( 'NONE',  ( -10.14667048435128294, 15.00000000000000000, -10.35833375027054082 ) ) ;
#19635=ORIENTED_EDGE ( 'NONE', *, *, #51144, .T. ) ;
#19641=CARTESIAN_POINT ( 'NONE',  ( 11.27492930200523880, 12.64336083852433035, -1.672692125565626631 ) ) ;
#19648=CARTESIAN_POINT ( 'NONE',  ( 10.88017736071110519, -19.43631465584515894, -2.602085213965210642E-15 ) ) ;
#19650=CARTESIAN_POINT ( 'NONE',  ( 14.99847009497945116, 0.3640475087720986824, -0.2142307401080281448 ) ) ;
#19663=DIRECTION ( 'NONE',  ( -0.000000000000000000, 1.000000000000000000, -0.000000000000000000 ) ) ;
#19669=VERTEX_POINT ( 'NONE', #90862 ) ;
#19680=ORIENTED_EDGE ( 'NONE', *, *, #3312, .F. ) ;
#19683=ORIENTED_EDGE ( 'NONE', *, *, #82536, .F. ) ;
#19685=LINE ( 'NONE', #3715, #42154 ) ;
#19700=CARTESIAN_POINT ( 'NONE',  ( -14.94699059465108881, 14.49999999999999112, 1.259949270174695268 ) ) ;
#19703=ORIENTED_EDGE ( 'NONE', *, *, #48173, .T. ) ;
#19709=FACE_OUTER_BOUND ( 'NONE', #8760, .T. ) ;
#19713=CARTESIAN_POINT ( 'NONE',  ( -5.204170427930421283E-15, 7.873634669930427599, -12.81628187352647608 ) ) ;
#19723=CARTESIAN_POINT ( 'NONE',  ( -12.67122524790595506, 14.95077488074853456, 7.555537761805664942 ) ) ;
#19726=CARTESIAN_POINT ( 'NONE',  ( 14.26139399674454822, 15.00000000000000000, -2.619664342929791445 ) ) ;
#19729=PLANE ( 'NONE',  #22867 ) ;
#19733=AXIS2_PLACEMENT_3D ( 'NONE', #10467, #9980, #17973 ) ;
#19741=CARTESIAN_POINT ( 'NONE',  ( -14.17193700899791153, 15.00000000000000000, 1.489530601563921808 ) ) ;
#19744=DIRECTION ( 'NONE',  ( 0.000000000000000000, 0.000000000000000000, 1.000000000000000000 ) ) ;
#19753=ORIENTED_EDGE ( 'NONE', *, *, #32943, .T. ) ;
#19754=CARTESIAN_POINT ( 'NONE',  ( -3.014428414850124138, 3.963468844518203138, 11.25000000000000178 ) ) ;
#19770=EDGE_CURVE ( 'NONE', #30654, #83990, #52376, .T. ) ;
#19773=CARTESIAN_POINT ( 'NONE',  ( 0.000000000000000000, 0.5000000000000004441, 0.000000000000000000 ) ) ;
#19775=CARTESIAN_POINT ( 'NONE',  ( 11.17717139118532010, 2.266418178063696498, 2.895237119026786043 ) ) ;
#19779=EDGE_CURVE ( 'NONE', #34423, #42615, #12272, .T. ) ;
#19786=CARTESIAN_POINT ( 'NONE',  ( -0.9082943533608713871, 15.00000000000000000, -14.47152380946376660 ) ) ;
#19798=VECTOR ( 'NONE', #83144, 1000.000000000000000 ) ;
#19804=CARTESIAN_POINT ( 'NONE',  ( 0.000000000000000000, 15.00000000000000000, 0.000000000000000000 ) ) ;
#19813=EDGE_LOOP ( 'NONE', ( #28331, #58590, #13561, #20299 ) ) ;
#19816=ORIENTED_EDGE ( 'NONE', *, *, #49456, .F. ) ;
#19823=CARTESIAN_POINT ( 'NONE',  ( -5.419894505350704605, 14.63606864255126538, 13.98659156302458229 ) ) ;
#19830=ORIENTED_EDGE ( 'NONE', *, *, #57231, .F. ) ;
#19838=CARTESIAN_POINT ( 'NONE',  ( 10.93781366033340063, 15.00000000000000000, 10.26470809774072634 ) ) ;
#19844=DIRECTION ( 'NONE',  ( 0.1822355254921578793, 0.000000000000000000, -0.9832549075639526182 ) ) ;
#19848=ORIENTED_EDGE ( 'NONE', *, *, #32622, .T. ) ;
#19849=CARTESIAN_POINT ( 'NONE',  ( 0.000000000000000000, 15.00000000000000000, 0.000000000000000000 ) ) ;
#19856=CARTESIAN_POINT ( 'NONE',  ( -7.313705784284680433, 15.00000000000000000, 13.09617149020738935 ) ) ;
#19860=ADVANCED_FACE ( 'NONE', ( #78823 ), #56803, .T. ) ;
#19865=AXIS2_PLACEMENT_3D ( 'NONE', #51471, #74959, #81960 ) ;
#19870=AXIS2_PLACEMENT_3D ( 'NONE', #1477, #84954, #1969 ) ;
#19871=VERTEX_POINT ( 'NONE', #3319 ) ;
#19874=CARTESIAN_POINT ( 'NONE',  ( 12.50534872682730914, 15.00000000000000000, -7.339363270777500503 ) ) ;
#19878=DIRECTION ( 'NONE',  ( 0.000000000000000000, 0.000000000000000000, 1.000000000000000000 ) ) ;
#19884=ORIENTED_EDGE ( 'NONE', *, *, #77005, .F. ) ;
#19895=CARTESIAN_POINT ( 'NONE',  ( -9.159723438033276821, 15.00000000000000000, 10.91613331444536250 ) ) ;
#19899=CARTESIAN_POINT ( 'NONE',  ( -7.003840667633538963, 15.00000000000000888, -12.84073839985662779 ) ) ;
#19901=CARTESIAN_POINT ( 'NONE',  ( -4.862001128006231632, 15.00000000000000000, -13.66056166603291189 ) ) ;
#19907=DIRECTION ( 'NONE',  ( 0.000000000000000000, 1.000000000000000000, 0.000000000000000000 ) ) ;
#19910=CARTESIAN_POINT ( 'NONE',  ( -14.99847009497944406, 0.5000000000000004441, -0.2142307401082361173 ) ) ;
#19915=CARTESIAN_POINT ( 'NONE',  ( 0.000000000000000000, 15.00000000000000000, 0.000000000000000000 ) ) ;
#19918=AXIS2_PLACEMENT_3D ( 'NONE', #32718, #63216, #46265 ) ;
#19926=DIRECTION ( 'NONE',  ( -0.000000000000000000, -1.000000000000000000, -0.000000000000000000 ) ) ;
#19933=VERTEX_POINT ( 'NONE', #1868 ) ;
#19935=EDGE_CURVE ( 'NONE', #1450, #41967, #65936, .T. ) ;
#19937=CARTESIAN_POINT ( 'NONE',  ( -13.59943737456451629, 0.04922511925147186190, -5.718514076973049143 ) ) ;
#19950=LINE ( 'NONE', #67427, #82830 ) ;
#19954=CARTESIAN_POINT ( 'NONE',  ( -12.81628187352647608, -35.87636533006957507, 3.903127820947815962E-15 ) ) ;
#19962=VECTOR ( 'NONE', #47199, 1000.000000000000000 ) ;
#19963=CARTESIAN_POINT ( 'NONE',  ( 2.962741594153077251, 15.00000000000000000, -13.93860331045673107 ) ) ;
#19969=ORIENTED_EDGE ( 'NONE', *, *, #37042, .F. ) ;
#19973=ADVANCED_FACE ( 'NONE', ( #85840 ), #17353, .F. ) ;
#19977=DIRECTION ( 'NONE',  ( 0.000000000000000000, 0.000000000000000000, 1.000000000000000000 ) ) ;
#19983=EDGE_CURVE ( 'NONE', #64886, #17335, #89413, .T. ) ;
#19990=EDGE_CURVE ( 'NONE', #42327, #62224, #37454, .T. ) ;
#19996=CARTESIAN_POINT ( 'NONE',  ( -5.419894505350674407, 0.5000000000000004441, 13.98659156302455031 ) ) ;
#20002=ADVANCED_FACE ( 'NONE', ( #95801 ), #4802, .F. ) ;
#20008=CARTESIAN_POINT ( 'NONE',  ( -10.36894250292379205, -28.82125116508602503, -10.36894250292378672 ) ) ;
#20011=ORIENTED_EDGE ( 'NONE', *, *, #11527, .F. ) ;
#20012=CARTESIAN_POINT ( 'NONE',  ( -3.843542995449753530, 0.2301500725087323451, 14.43777707752876438 ) ) ;
#20020=EDGE_CURVE ( 'NONE', #18735, #59535, #27858, .T. ) ;
#20024=CARTESIAN_POINT ( 'NONE',  ( 10.88017736071110519, 20.56368534415484106, -2.602085213965210642E-15 ) ) ;
#20027=DIRECTION ( 'NONE',  ( 0.000000000000000000, 1.000000000000000000, 0.000000000000000000 ) ) ;
#20032=VECTOR ( 'NONE', #92530, 1000.000000000000114 ) ;
#20040=ORIENTED_EDGE ( 'NONE', *, *, #47764, .T. ) ;
#20050=DIRECTION ( 'NONE',  ( 0.000000000000000000, 0.000000000000000000, 1.000000000000000000 ) ) ;
#20056=ORIENTED_EDGE ( 'NONE', *, *, #42417, .F. ) ;
#20067=LINE ( 'NONE', #29530, #46615 ) ;
#20068=CARTESIAN_POINT ( 'NONE',  ( 7.208316651077764980, 7.883931151000783011, 7.208316651077762316 ) ) ;
#20069=EDGE_CURVE ( 'NONE', #1023, #61713, #29660, .T. ) ;
#20073=ORIENTED_EDGE ( 'NONE', *, *, #82402, .F. ) ;
#20084=CIRCLE ( 'NONE', #31214, 14.49999999999999822 ) ;
#20086=EDGE_LOOP ( 'NONE', ( #55986, #11128, #9672, #52510 ) ) ;
#20090=ORIENTED_EDGE ( 'NONE', *, *, #15921, .T. ) ;
#20100=B_SPLINE_CURVE_WITH_KNOTS ( 'NONE', 3,
 ( #39895, #48368, #85889, #17403, #48857, #94360 ),
 .UNSPECIFIED., .F., .F.,
 ( 4, 2, 4 ),
 ( 3.409110551494643301E-05, 0.0004400426677367919384, 0.0008459942299586375048 ),
 .UNSPECIFIED. ) ;
#20103=DIRECTION ( 'NONE',  ( 0.000000000000000000, 0.000000000000000000, 1.000000000000000000 ) ) ;
#20107=CARTESIAN_POINT ( 'NONE',  ( -11.17418640071729818, 12.98409833943821567, 3.592726937080809257 ) ) ;
#20108=CARTESIAN_POINT ( 'NONE',  ( 9.722841580490404922, 15.00000000000000000, 12.70211588817942960 ) ) ;
#20109=CARTESIAN_POINT ( 'NONE',  ( -3.192513988407930547, -3.205596188883898450E-15, -14.27292421863754512 ) ) ;
#20111=DIRECTION ( 'NONE',  ( 0.000000000000000000, 0.000000000000000000, 1.000000000000000000 ) ) ;
#20115=CARTESIAN_POINT ( 'NONE',  ( 7.595945211629608451, 15.00000000000000000, 12.35117874302463292 ) ) ;
#20116=VECTOR ( 'NONE', #32572, 1000.000000000000227 ) ;
#20122=DIRECTION ( 'NONE',  ( -0.000000000000000000, 1.000000000000000000, -0.000000000000000000 ) ) ;
#20131=EDGE_CURVE ( 'NONE', #94488, #98433, #80296, .T. ) ;
#20132=DIRECTION ( 'NONE',  ( 0.000000000000000000, 0.000000000000000000, 1.000000000000000000 ) ) ;
#20137=CARTESIAN_POINT ( 'NONE',  ( 2.915334737309921209, -23.39464798917849464, -10.88017736071110164 ) ) ;
#20150=LINE ( 'NONE', #81632, #61524 ) ;
#20158=DIRECTION ( 'NONE',  ( 0.000000000000000000, 0.000000000000000000, 1.000000000000000000 ) ) ;
#20166=CARTESIAN_POINT ( 'NONE',  ( -5.361923921558584105, 0.000000000000000000, 0.9937738586171629418 ) ) ;
#20173=EDGE_LOOP ( 'NONE', ( #94577, #52042, #62448, #89610 ) ) ;
#20174=CARTESIAN_POINT ( 'NONE',  ( 8.235571585149873641, 9.796802177851539284, 8.235571585149866536 ) ) ;
#20189=DIRECTION ( 'NONE',  ( -0.9914448613738093830, 0.000000000000000000, -0.1305261922200583180 ) ) ;
#20190=B_SPLINE_CURVE_WITH_KNOTS ( 'NONE', 3,
 ( #46593, #69601, #25588, #94066, #79057, #1122 ),
 .UNSPECIFIED., .F., .F.,
 ( 4, 2, 4 ),
 ( 0.0002800518438701976435, 0.0006862575805781378786, 0.001092463317286078168 ),
 .UNSPECIFIED. ) ;
#20191=DIRECTION ( 'NONE',  ( -0.000000000000000000, 1.000000000000000000, -0.000000000000000000 ) ) ;
#20192=ORIENTED_EDGE ( 'NONE', *, *, #29887, .T. ) ;
#20193=FACE_OUTER_BOUND ( 'NONE', #6869, .T. ) ;
#20194=EDGE_LOOP ( 'NONE', ( #28548, #45034, #68105, #47595, #67681, #50931 ) ) ;
#20195=ORIENTED_EDGE ( 'NONE', *, *, #65117, .T. ) ;
#20203=CARTESIAN_POINT ( 'NONE',  ( 6.408140936763236262, 2.456968003263761080, -11.09922568453595026 ) ) ;
#20205=VERTEX_POINT ( 'NONE', #3821 ) ;
#20217=VECTOR ( 'NONE', #40317, 1000.000000000000114 ) ;
#20219=CARTESIAN_POINT ( 'NONE',  ( 0.000000000000000000, 0.000000000000000000, 0.000000000000000000 ) ) ;
#20221=ADVANCED_FACE ( 'NONE', ( #34785 ), #34276, .F. ) ;
#20224=TOROIDAL_SURFACE ( 'NONE', #39377, 14.49999999999999822, 0.5000000000000000000 ) ;
#20227=EDGE_CURVE ( 'NONE', #41669, #81607, #65273, .T. ) ;
#20229=FACE_OUTER_BOUND ( 'NONE', #82669, .T. ) ;
#20230=ORIENTED_EDGE ( 'NONE', *, *, #31276, .T. ) ;
#20232=CARTESIAN_POINT ( 'NONE',  ( -11.29222593019783538, 0.2306972965111817597, 9.783848334571175087 ) ) ;
#20236=CARTESIAN_POINT ( 'NONE',  ( -11.81378540890925066, 0.000000000000000000, -7.968498874458281200 ) ) ;
#20241=DIRECTION ( 'NONE',  ( 0.000000000000000000, 1.000000000000000000, 0.000000000000000000 ) ) ;
#20249=CIRCLE ( 'NONE', #50586, 15.00000000000000000 ) ;
#20251=ORIENTED_EDGE ( 'NONE', *, *, #17531, .F. ) ;
#20260=LINE ( 'NONE', #73247, #2019 ) ;
#20263=CARTESIAN_POINT ( 'NONE',  ( 12.26659068614894821, 3.887082168247312008, 7.082119434687044190 ) ) ;
#20268=ADVANCED_FACE ( 'NONE', ( #62084 ), #45620, .F. ) ;
#20277=DIRECTION ( 'NONE',  ( 0.000000000000000000, 1.000000000000000000, 0.000000000000000000 ) ) ;
#20283=PLANE ( 'NONE',  #14157 ) ;
#20290=DIRECTION ( 'NONE',  ( 0.000000000000000000, 1.000000000000000000, 0.000000000000000000 ) ) ;
#20294=CARTESIAN_POINT ( 'NONE',  ( 12.80781515976310203, 15.00000000000000000, 6.246788841744411513 ) ) ;
#20299=ORIENTED_EDGE ( 'NONE', *, *, #58058, .F. ) ;
#20306=CARTESIAN_POINT ( 'NONE',  ( 4.084234479374312166, 0.000000000000000000, -3.613425430272927397 ) ) ;
#20315=VECTOR ( 'NONE', #24559, 1000.000000000000000 ) ;
#20321=ORIENTED_EDGE ( 'NONE', *, *, #28594, .T. ) ;
#20324=EDGE_CURVE ( 'NONE', #12526, #33923, #53577, .T. ) ;
#20325=AXIS2_PLACEMENT_3D ( 'NONE', #25419, #71405, #40416 ) ;
#20328=VECTOR ( 'NONE', #84015, 999.9999999999998863 ) ;
#20330=CARTESIAN_POINT ( 'NONE',  ( -5.147851794455972296, 15.00000000000000533, 13.68970903997123401 ) ) ;
#20340=PLANE ( 'NONE',  #67081 ) ;
#20352=ORIENTED_EDGE ( 'NONE', *, *, #6684, .T. ) ;
#20360=CARTESIAN_POINT ( 'NONE',  ( 0.000000000000000000, 15.00000000000000000, 0.000000000000000000 ) ) ;
#20361=AXIS2_PLACEMENT_3D ( 'NONE', #98118, #68103, #66613 ) ;
#20363=PLANE ( 'NONE',  #88834 ) ;
#20366=TOROIDAL_SURFACE ( 'NONE', #76258, 14.49999999999999822, 0.5000000000000000000 ) ;
#20368=CARTESIAN_POINT ( 'NONE',  ( -10.93781366033333136, 0.5000000000000004441, -10.26470809774080628 ) ) ;
#20379=VECTOR ( 'NONE', #41250, 1000.000000000000114 ) ;
#20381=DIRECTION ( 'NONE',  ( -0.7604059656000340395, 0.000000000000000000, 0.6494480483301799945 ) ) ;
#20382=CARTESIAN_POINT ( 'NONE',  ( 7.618303901329630534, 14.99999999999807798, 12.48478900416944803 ) ) ;
#20383=ADVANCED_FACE ( 'NONE', ( #84610 ), #54584, .F. ) ;
#20387=VERTEX_POINT ( 'NONE', #83626 ) ;
#20392=DIRECTION ( 'NONE',  ( -0.000000000000000000, -1.000000000000000000, -0.000000000000000000 ) ) ;
#20395=FACE_OUTER_BOUND ( 'NONE', #95214, .T. ) ;
#20400=CARTESIAN_POINT ( 'NONE',  ( -9.742785792574931492, 8.338468844518212464, 5.625000000000008882 ) ) ;
#20403=CARTESIAN_POINT ( 'NONE',  ( -5.963430220938278126, 10.52164270246084499, 10.32896413005680358 ) ) ;
#20406=ORIENTED_EDGE ( 'NONE', *, *, #69340, .F. ) ;
#20407=CARTESIAN_POINT ( 'NONE',  ( 10.64017930668206446, 0.3640475087720991820, -10.57291749337215769 ) ) ;
#20414=CARTESIAN_POINT ( 'NONE',  ( 1.548803529118027100, 0.000000000000000000, -5.228673087012095877 ) ) ;
#20418=DIRECTION ( 'NONE',  ( 0.000000000000000000, 0.000000000000000000, 1.000000000000000000 ) ) ;
#20427=ORIENTED_EDGE ( 'NONE', *, *, #36389, .F. ) ;
#20431=CARTESIAN_POINT ( 'NONE',  ( 11.81378540890930751, 0.000000000000000000, 7.968498874458199488 ) ) ;
#20438=EDGE_CURVE ( 'NONE', #23897, #74408, #50042, .T. ) ;
#20440=CARTESIAN_POINT ( 'NONE',  ( -5.419894505350399072, 14.63595249122790598, -13.98659156302466222 ) ) ;
#20456=CARTESIAN_POINT ( 'NONE',  ( 12.81628187352647608, -13.58469866340290899, 3.434112377981052511 ) ) ;
#20468=CARTESIAN_POINT ( 'NONE',  ( -12.98685442714204008, 4.660809545892429844E-16, 6.449155920600864178 ) ) ;
#20469=ORIENTED_EDGE ( 'NONE', *, *, #56988, .T. ) ;
#20475=ORIENTED_EDGE ( 'NONE', *, *, #4415, .T. ) ;
#20477=CARTESIAN_POINT ( 'NONE',  ( -5.204170427930421283E-15, 8.438309369127518167, -11.92686044187656513 ) ) ;
#20483=DIRECTION ( 'NONE',  ( 0.4924235601034648302, 0.000000000000000000, 0.8703556959399010307 ) ) ;
#20486=ORIENTED_EDGE ( 'NONE', *, *, #13094, .F. ) ;
#20487=DIRECTION ( 'NONE',  ( 0.000000000000000000, 1.000000000000000000, 0.000000000000000000 ) ) ;
#20489=VERTEX_POINT ( 'NONE', #7646 ) ;
#20490=DIRECTION ( 'NONE',  ( 0.000000000000000000, 1.000000000000000000, 0.000000000000000000 ) ) ;
#20499=CARTESIAN_POINT ( 'NONE',  ( -11.62719953690072217, 14.63595249122789177, 9.476720473301721626 ) ) ;
#20508=CARTESIAN_POINT ( 'NONE',  ( 0.000000000000000000, 14.49999999999999822, 0.000000000000000000 ) ) ;
#20511=CARTESIAN_POINT ( 'NONE',  ( -12.26659068614895354, -23.61291783175269643, -7.082119434687038861 ) ) ;
#20521=CARTESIAN_POINT ( 'NONE',  ( 14.36343418943210892, 14.95077488074853456, 3.367173657400750031 ) ) ;
#20527=CARTESIAN_POINT ( 'NONE',  ( 9.422509992056141925, 15.98035201082151424, -5.440088680355554374 ) ) ;
#20530=DIRECTION ( 'NONE',  ( 0.5948227867513480316, 0.000000000000000000, -0.8038568606172125097 ) ) ;
#20542=CARTESIAN_POINT ( 'NONE',  ( -1.780824192092587577, 14.49999999999999112, 14.89391369643518637 ) ) ;
#20545=ORIENTED_EDGE ( 'NONE', *, *, #18000, .F. ) ;
#20551=CARTESIAN_POINT ( 'NONE',  ( -15.67879934938584263, -0.03417435944610275333, 3.170591017105712339 ) ) ;
#20560=VERTEX_POINT ( 'NONE', #8122 ) ;
#20561=ORIENTED_EDGE ( 'NONE', *, *, #25638, .F. ) ;
#20567=CARTESIAN_POINT ( 'NONE',  ( -12.00809552683946357, 14.49999999999999822, -8.989195838243713155 ) ) ;
#20568=CARTESIAN_POINT ( 'NONE',  ( -12.60589901313233874, 14.49999999999999112, 8.129656208641975468 ) ) ;
#20571=ADVANCED_FACE ( 'NONE', ( #68624 ), #75066, .T. ) ;
#20574=CARTESIAN_POINT ( 'NONE',  ( -14.71525861348295017, 0.3639310978437778066, 2.908807992686501809 ) ) ;
#20577=CARTESIAN_POINT ( 'NONE',  ( 2.638427012816829897, 4.550597817667449974, -9.846743663894592657 ) ) ;
#20580=ORIENTED_EDGE ( 'NONE', *, *, #43120, .F. ) ;
#20589=ORIENTED_EDGE ( 'NONE', *, *, #43226, .T. ) ;
#20602=AXIS2_PLACEMENT_3D ( 'NONE', #6928, #82919, #96966 ) ;
#20603=DIRECTION ( 'NONE',  ( -0.3007057995042635712, 0.000000000000000000, -0.9537169507482300412 ) ) ;
#20604=VERTEX_POINT ( 'NONE', #87551 ) ;
#20608=B_SPLINE_CURVE_WITH_KNOTS ( 'NONE', 3,
 ( #45877, #15875, #91863, #7393, #23381, #54340 ),
 .UNSPECIFIED., .F., .F.,
 ( 4, 2, 4 ),
 ( 3.409110551494648722E-05, 0.0004400426677367932937, 0.0008459942299586401069 ),
 .UNSPECIFIED. ) ;
#20613=CARTESIAN_POINT ( 'NONE',  ( -4.431036607602702126, 14.49999999999999112, 14.33059365769913462 ) ) ;
#20616=LINE ( 'NONE', #13602, #22755 ) ;
#20623=CARTESIAN_POINT ( 'NONE',  ( 0.000000000000000000, 0.5000000000000004441, 0.000000000000000000 ) ) ;
#20633=DIRECTION ( 'NONE',  ( 0.9426414910921736556, 0.000000000000000000, 0.3338068592337842255 ) ) ;
#20640=CARTESIAN_POINT ( 'NONE',  ( -9.422509992056145478, -27.35298132251182324, -5.440088680355541939 ) ) ;
#20644=FACE_OUTER_BOUND ( 'NONE', #84092, .T. ) ;
#20646=EDGE_CURVE ( 'NONE', #95164, #88686, #54810, .T. ) ;
#20656=VERTEX_POINT ( 'NONE', #11553 ) ;
#20674=ORIENTED_EDGE ( 'NONE', *, *, #13689, .T. ) ;
#20687=EDGE_CURVE ( 'NONE', #49977, #1901, #41539, .T. ) ;
#20690=LINE ( 'NONE', #83655, #33149 ) ;
#20693=CARTESIAN_POINT ( 'NONE',  ( 4.923371831947301658, -37.32440218233254114, 8.527530157486175710 ) ) ;
#20695=CARTESIAN_POINT ( 'NONE',  ( 0.2851878892742318872, 14.76937129508116264, -14.93850447011040927 ) ) ;
#20697=ORIENTED_EDGE ( 'NONE', *, *, #35991, .F. ) ;
#20702=DIRECTION ( 'NONE',  ( 0.000000000000000000, 1.000000000000000000, 0.000000000000000000 ) ) ;
#20705=CARTESIAN_POINT ( 'NONE',  ( 11.09922568453595026, 11.20696800326376241, 6.408140936763232709 ) ) ;
#20706=EDGE_LOOP ( 'NONE', ( #53087, #26994, #61274, #83480, #296, #68808 ) ) ;
#20708=ORIENTED_EDGE ( 'NONE', *, *, #30256, .T. ) ;
#20721=ORIENTED_EDGE ( 'NONE', *, *, #33440, .T. ) ;
#20724=DIRECTION ( 'NONE',  ( 0.000000000000000000, 1.000000000000000000, 0.000000000000000000 ) ) ;
#20725=DIRECTION ( 'NONE',  ( 0.9238795325112876267, 0.000000000000000000, 0.3826834323650877279 ) ) ;
#20731=CARTESIAN_POINT ( 'NONE',  ( -14.62232599144297929, 6.894848190650002788E-16, 0.3548652576987693097 ) ) ;
#20737=CARTESIAN_POINT ( 'NONE',  ( 6.689969769698871360, -0.03417435944610275333, 12.58200319823975022 ) ) ;
#20750=CARTESIAN_POINT ( 'NONE',  ( 14.24131928502211331, 0.000000000000000000, 0.4973178280106892446 ) ) ;
#20752=VECTOR ( 'NONE', #50088, 1000.000000000000114 ) ;
#20758=CARTESIAN_POINT ( 'NONE',  ( -12.26659068614895354, 1.387082168247309788, -7.082119434687038861 ) ) ;
#20780=CARTESIAN_POINT ( 'NONE',  ( 4.838527690343521925, 0.5000000000000004441, 14.19819177887730177 ) ) ;
#20786=VECTOR ( 'NONE', #52721, 1000.000000000000000 ) ;
#20799=CARTESIAN_POINT ( 'NONE',  ( 12.25993886608605443, 0.5000000000000004441, -8.642563219313617040 ) ) ;
#20809=CARTESIAN_POINT ( 'NONE',  ( -14.56195259121199115, 6.572975670693368659E-16, 1.374002722866616066 ) ) ;
#20812=EDGE_LOOP ( 'NONE', ( #50589, #57978, #50752, #81554, #29729, #35968 ) ) ;
#20818=DIRECTION ( 'NONE',  ( 5.506706202140776441E-14, 0.000000000000000000, 1.000000000000000000 ) ) ;
#20820=AXIS2_PLACEMENT_3D ( 'NONE', #6642, #82140, #81645 ) ;
#20824=ORIENTED_EDGE ( 'NONE', *, *, #26557, .F. ) ;
#20826=AXIS2_PLACEMENT_3D ( 'NONE', #58385, #63915, #18937 ) ;
#20832=CARTESIAN_POINT ( 'NONE',  ( 2.393480905993173646, 14.63606894034135308, -14.80781041047755053 ) ) ;
#20839=VERTEX_POINT ( 'NONE', #20542 ) ;
#20846=LINE ( 'NONE', #43337, #1661 ) ;
#20856=CARTESIAN_POINT ( 'NONE',  ( 1.829604203029677523, -0.03417435944610275333, -15.89119079541585755 ) ) ;
#20860=ORIENTED_EDGE ( 'NONE', *, *, #553, .T. ) ;
#20881=EDGE_CURVE ( 'NONE', #95321, #77887, #75507, .T. ) ;
#20885=CARTESIAN_POINT ( 'NONE',  ( -0.2076750170234879511, 0.04922511925147027984, 14.75137184266417201 ) ) ;
#20886=AXIS2_PLACEMENT_3D ( 'NONE', #94063, #3575, #70584 ) ;
#20887=EDGE_LOOP ( 'NONE', ( #15083, #42582, #23074, #67684, #63891, #98798 ) ) ;
#20889=LINE ( 'NONE', #49043, #89518 ) ;
#20912=CARTESIAN_POINT ( 'NONE',  ( -2.888814634336892784, -3.129363223631011419E-15, 14.33747749179066666 ) ) ;
#20916=EDGE_CURVE ( 'NONE', #31163, #31031, #71495, .T. ) ;
#20922=ORIENTED_EDGE ( 'NONE', *, *, #13337, .T. ) ;
#20924=DIRECTION ( 'NONE',  ( 0.000000000000000000, 0.000000000000000000, 1.000000000000000000 ) ) ;
#20935=CARTESIAN_POINT ( 'NONE',  ( -13.50249619331269102, 7.318364664277152957E-16, -5.623250243473677301 ) ) ;
#20937=VERTEX_POINT ( 'NONE', #74018 ) ;
#20947=FACE_OUTER_BOUND ( 'NONE', #10478, .T. ) ;
#20948=PLANE ( 'NONE',  #98860 ) ;
#20954=CARTESIAN_POINT ( 'NONE',  ( 9.382169495545415572, -12.75136533006957507, -9.382169495545422677 ) ) ;
#20964=ADVANCED_FACE ( 'NONE', ( #90011 ), #74516, .F. ) ;
#20966=AXIS2_PLACEMENT_3D ( 'NONE', #84491, #61476, #75502 ) ;
#20968=EDGE_LOOP ( 'NONE', ( #55828, #52059, #67309, #28237, #602, #29738 ) ) ;
#20974=ORIENTED_EDGE ( 'NONE', *, *, #45429, .T. ) ;
#20990=CARTESIAN_POINT ( 'NONE',  ( -14.88232117145535405, 0.3639310251205940538, 1.875237731503057281 ) ) ;
#20998=CARTESIAN_POINT ( 'NONE',  ( 5.377205135395962010, 0.2306972965111855067, -13.94000429068781877 ) ) ;
#21003=FACE_OUTER_BOUND ( 'NONE', #64322, .T. ) ;
#21007=CARTESIAN_POINT ( 'NONE',  ( -5.204170427930421283E-15, -24.44625116508603213, -14.16423886937410082 ) ) ;
#21017=CARTESIAN_POINT ( 'NONE',  ( 15.96747533562963639, 15.00000000000000000, -0.9576679184940652956 ) ) ;
#21022=CARTESIAN_POINT ( 'NONE',  ( 3.469446951953614189E-15, 34.31368534415485527, 10.88017736071110342 ) ) ;
#21026=CARTESIAN_POINT ( 'NONE',  ( -14.56332774647475858, 0.04922511925147020351, 2.357028871694085481 ) ) ;
#21027=ORIENTED_EDGE ( 'NONE', *, *, #36345, .T. ) ;
#21036=CARTESIAN_POINT ( 'NONE',  ( 13.86102707272219980, 15.00000000000000711, 4.666951904077296653 ) ) ;
#21037=CARTESIAN_POINT ( 'NONE',  ( 0.000000000000000000, 0.000000000000000000, 0.000000000000000000 ) ) ;
#21039=ORIENTED_EDGE ( 'NONE', *, *, #8530, .F. ) ;
#21041=EDGE_CURVE ( 'NONE', #64665, #24788, #68799, .T. ) ;
#21052=VECTOR ( 'NONE', #77538, 1000.000000000000114 ) ;
#21060=DIRECTION ( 'NONE',  ( 0.000000000000000000, 0.000000000000000000, 1.000000000000000000 ) ) ;
#21064=CARTESIAN_POINT ( 'NONE',  ( 10.84451454130500636, 4.196149184706192213E-16, 9.625305416630906663 ) ) ;
#21067=CARTESIAN_POINT ( 'NONE',  ( -9.846743663894596210, 10.80059781766745530, -2.638427012816824124 ) ) ;
#21069=EDGE_LOOP ( 'NONE', ( #74533, #5260, #60734, #39903 ) ) ;
#21079=AXIS2_PLACEMENT_3D ( 'NONE', #49688, #87691, #96201 ) ;
#21084=ORIENTED_EDGE ( 'NONE', *, *, #24016, .F. ) ;
#21092=CYLINDRICAL_SURFACE ( 'NONE', #41098, 15.00000000000000000 ) ;
#21094=AXIS2_PLACEMENT_3D ( 'NONE', #50726, #35715, #30175 ) ;
#21101=AXIS2_PLACEMENT_3D ( 'NONE', #53516, #75036, #563 ) ;
#21103=ORIENTED_EDGE ( 'NONE', *, *, #55564, .F. ) ;
#21106=DIRECTION ( 'NONE',  ( -0.000000000000000000, -1.000000000000000000, -0.000000000000000000 ) ) ;
#21109=VERTEX_POINT ( 'NONE', #81033 ) ;
#21110=CARTESIAN_POINT ( 'NONE',  ( 9.383795276901770066, 14.76930270348882601, -11.62679839395692305 ) ) ;
#21116=EDGE_CURVE ( 'NONE', #55876, #57707, #25043, .T. ) ;
#21135=CARTESIAN_POINT ( 'NONE',  ( -9.422509992056136596, -11.51964798917848931, 5.440088680355559703 ) ) ;
#21153=DIRECTION ( 'NONE',  ( -0.000000000000000000, -1.000000000000000000, -0.000000000000000000 ) ) ;
#21160=CARTESIAN_POINT ( 'NONE',  ( -0.04758788293964817673, 0.000000000000000000, -5.453031268574420665 ) ) ;
#21163=VECTOR ( 'NONE', #89603, 1000.000000000000000 ) ;
#21164=DIRECTION ( 'NONE',  ( -0.000000000000000000, -1.000000000000000000, -0.000000000000000000 ) ) ;
#21185=CARTESIAN_POINT ( 'NONE',  ( 4.923371831947301658, -27.32440218233254114, 8.527530157486175710 ) ) ;
#21190=VERTEX_POINT ( 'NONE', #39496 ) ;
#21200=CARTESIAN_POINT ( 'NONE',  ( -6.408140936763232709, 4.956968003263756195, 11.09922568453595026 ) ) ;
#21201=ORIENTED_EDGE ( 'NONE', *, *, #7939, .F. ) ;
#21209=FACE_OUTER_BOUND ( 'NONE', #55987, .T. ) ;
#21212=CIRCLE ( 'NONE', #61174, 13.74999999999999467 ) ;
#21214=DIRECTION ( 'NONE',  ( -7.105427357601001859E-15, 0.000000000000000000, 1.000000000000000000 ) ) ;
#21215=CARTESIAN_POINT ( 'NONE',  ( 0.3329122712635265713, 0.000000000000000000, 5.443067521379392204 ) ) ;
#21220=ORIENTED_EDGE ( 'NONE', *, *, #1410, .T. ) ;
#21226=CARTESIAN_POINT ( 'NONE',  ( -4.265913727725424209, 14.95037113646024096, 14.12300574719970392 ) ) ;
#21227=DIRECTION ( 'NONE',  ( -0.4461978131098131573, 0.000000000000000000, 0.8949343616020228875 ) ) ;
#21235=DIRECTION ( 'NONE',  ( 0.000000000000000000, 0.000000000000000000, 1.000000000000000000 ) ) ;
#21236=ADVANCED_FACE ( 'NONE', ( #53989 ), #30983, .T. ) ;
#21239=VECTOR ( 'NONE', #29199, 1000.000000000000000 ) ;
#21240=VERTEX_POINT ( 'NONE', #23519 ) ;
#21245=FACE_OUTER_BOUND ( 'NONE', #66359, .T. ) ;
#21251=CIRCLE ( 'NONE', #26039, 15.00000000000000000 ) ;
#21252=CARTESIAN_POINT ( 'NONE',  ( -14.16423886937410437, 11.59541550158063750, -3.795296366450299885 ) ) ;
#21255=EDGE_CURVE ( 'NONE', #74674, #89788, #31958, .T. ) ;
#21264=LINE ( 'NONE', #95787, #35876 ) ;
#21269=ORIENTED_EDGE ( 'NONE', *, *, #86840, .T. ) ;
#21282=CARTESIAN_POINT ( 'NONE',  ( 4.862001128006773421, 4.807100664002271835E-16, -13.66056166602460031 ) ) ;
#21286=EDGE_CURVE ( 'NONE', #97713, #80329, #28613, .T. ) ;
#21290=CARTESIAN_POINT ( 'NONE',  ( 0.000000000000000000, 0.5000000000000004441, 0.000000000000000000 ) ) ;
#21295=DIRECTION ( 'NONE',  ( 0.000000000000000000, 0.000000000000000000, -1.000000000000000000 ) ) ;
#21303=DIRECTION ( 'NONE',  ( 0.000000000000000000, 0.000000000000000000, -1.000000000000000000 ) ) ;
#21307=ORIENTED_EDGE ( 'NONE', *, *, #77475, .T. ) ;
#21312=PLANE ( 'NONE',  #45635 ) ;
#21313=VERTEX_POINT ( 'NONE', #15525 ) ;
#21317=ORIENTED_EDGE ( 'NONE', *, *, #59388, .T. ) ;
#21321=AXIS2_PLACEMENT_3D ( 'NONE', #86474, #78466, #46488 ) ;
#21323=ORIENTED_EDGE ( 'NONE', *, *, #36603, .F. ) ;
#21333=ADVANCED_FACE ( 'NONE', ( #47468 ), #29996, .T. ) ;
#21349=CARTESIAN_POINT ( 'NONE',  ( 13.14228782657334804, 15.00000000000000000, 7.230509711182329546 ) ) ;
#21353=CARTESIAN_POINT ( 'NONE',  ( -5.817157072110618721, 0.5000000000000004441, -13.82608706751094552 ) ) ;
#21360=VERTEX_POINT ( 'NONE', #53490 ) ;
#21361=LINE ( 'NONE', #82341, #32853 ) ;
#21363=CARTESIAN_POINT ( 'NONE',  ( 0.000000000000000000, 0.5000000000000004441, 0.000000000000000000 ) ) ;
#21367=CARTESIAN_POINT ( 'NONE',  ( 0.000000000000000000, 0.000000000000000000, 0.000000000000000000 ) ) ;
#21374=CYLINDRICAL_SURFACE ( 'NONE', #26804, 15.00000000000000000 ) ;
#21379=TOROIDAL_SURFACE ( 'NONE', #7047, 14.49999999999999822, 0.5000000000000000000 ) ;
#21394=CARTESIAN_POINT ( 'NONE',  ( -5.803070148808410877, 15.00000000000000000, 13.28812917035381780 ) ) ;
#21399=DIRECTION ( 'NONE',  ( -3.730349362740525976E-14, 0.000000000000000000, 1.000000000000000000 ) ) ;
#21409=DIRECTION ( 'NONE',  ( 0.9969173337331278528, 0.000000000000000000, 0.07845909572784537378 ) ) ;
#21436=CARTESIAN_POINT ( 'NONE',  ( -14.03351048042393856, -0.03417435944610275333, -2.474486531753901541 ) ) ;
#21437=FACE_OUTER_BOUND ( 'NONE', #2090, .T. ) ;
#21443=CARTESIAN_POINT ( 'NONE',  ( 3.434112377981060948, -19.41803199673624647, 12.81628187352647430 ) ) ;
#21453=EDGE_CURVE ( 'NONE', #14221, #23745, #96462, .T. ) ;
#21455=CARTESIAN_POINT ( 'NONE',  ( -14.71525861348292175, 14.63595249122790598, 2.908807992686487154 ) ) ;
#21456=ORIENTED_EDGE ( 'NONE', *, *, #29507, .T. ) ;
#21474=CARTESIAN_POINT ( 'NONE',  ( -6.689969769699040114, -0.03417435944610275333, 12.58200319823965785 ) ) ;
#21475=EDGE_CURVE ( 'NONE', #17879, #39344, #51094, .T. ) ;
#21479=ADVANCED_FACE ( 'NONE', ( #26931 ), #62960, .T. ) ;
#21488=CARTESIAN_POINT ( 'NONE',  ( 0.000000000000000000, 14.49999999999999822, 0.000000000000000000 ) ) ;
#21497=CARTESIAN_POINT ( 'NONE',  ( 0.000000000000000000, 14.49999999999999822, 0.000000000000000000 ) ) ;
#21499=CARTESIAN_POINT ( 'NONE',  ( 10.36894250292378850, -25.07125116508602858, -10.36894250292379027 ) ) ;
#21503=VERTEX_POINT ( 'NONE', #25486 ) ;
#21509=DIRECTION ( 'NONE',  ( -0.000000000000000000, 1.000000000000000000, -0.000000000000000000 ) ) ;
#21511=DIRECTION ( 'NONE',  ( 0.000000000000000000, 1.000000000000000000, -0.000000000000000000 ) ) ;
#21513=CARTESIAN_POINT ( 'NONE',  ( 7.964842623401177768, 26.18868534415484106, -7.964842623401181321 ) ) ;
#21516=CIRCLE ( 'NONE', #16740, 14.49999999999999822 ) ;
#21536=AXIS2_PLACEMENT_3D ( 'NONE', #40338, #86816, #79309 ) ;
#21553=ORIENTED_EDGE ( 'NONE', *, *, #88511, .T. ) ;
#21559=DIRECTION ( 'NONE',  ( 0.000000000000000000, 0.000000000000000000, 1.000000000000000000 ) ) ;
#21565=CARTESIAN_POINT ( 'NONE',  ( 13.40508947812163143, 15.00000000000000000, 5.527528931046191474 ) ) ;
#21567=CARTESIAN_POINT ( 'NONE',  ( 0.000000000000000000, 15.00000000000000000, 0.000000000000000000 ) ) ;
#21568=CARTESIAN_POINT ( 'NONE',  ( 4.923371831947295441, 14.34226448433412138, -8.527530157486179263 ) ) ;
#21571=LINE ( 'NONE', #37065, #60565 ) ;
#21572=ORIENTED_EDGE ( 'NONE', *, *, #16159, .T. ) ;
#21595=DIRECTION ( 'NONE',  ( 0.5372996083468306594, 0.000000000000000000, -0.8433914458128813907 ) ) ;
#21596=EDGE_CURVE ( 'NONE', #61713, #98693, #54362, .T. ) ;
#21601=VECTOR ( 'NONE', #10777, 1000.000000000000227 ) ;
#21602=DIRECTION ( 'NONE',  ( -2.131628207280300558E-14, 0.000000000000000000, 1.000000000000000000 ) ) ;
#21605=VERTEX_POINT ( 'NONE', #41475 ) ;
#21606=CARTESIAN_POINT ( 'NONE',  ( -10.02032951099770841, 12.52870482769689708, -5.208770347913566745 ) ) ;
#21607=FACE_OUTER_BOUND ( 'NONE', #68656, .T. ) ;
#21608=CARTESIAN_POINT ( 'NONE',  ( 13.14228782657346528, 14.49999999999999112, -7.230509711182246058 ) ) ;
#21611=CARTESIAN_POINT ( 'NONE',  ( 7.684764310694878198, 15.00000000000000000, -12.88194075009934991 ) ) ;
#21613=CARTESIAN_POINT ( 'NONE',  ( 3.469446951953614189E-15, 5.938309369127516391, 11.92686044187656513 ) ) ;
#21615=CARTESIAN_POINT ( 'NONE',  ( 13.21236992757673789, -0.03417435944610275333, -5.338143956176714333 ) ) ;
#21622=ORIENTED_EDGE ( 'NONE', *, *, #68762, .F. ) ;
#21624=EDGE_LOOP ( 'NONE', ( #91274, #41951, #55494, #74518 ) ) ;
#21635=CARTESIAN_POINT ( 'NONE',  ( -7.964842623401172439, -16.31131465584515539, 7.964842623401183097 ) ) ;
#21642=CARTESIAN_POINT ( 'NONE',  ( 14.09397099617992311, 14.95037102751076752, -4.360881834954174252 ) ) ;
#21652=ORIENTED_EDGE ( 'NONE', *, *, #4531, .F. ) ;
#21661=CARTESIAN_POINT ( 'NONE',  ( 9.065164099344563908, 14.63606892172321139, -11.95084933600769439 ) ) ;
#21663=ORIENTED_EDGE ( 'NONE', *, *, #38673, .F. ) ;
#21665=DIRECTION ( 'NONE',  ( 0.000000000000000000, 0.000000000000000000, 1.000000000000000000 ) ) ;
#21667=ORIENTED_EDGE ( 'NONE', *, *, #37571, .T. ) ;
#21685=CARTESIAN_POINT ( 'NONE',  ( 2.638427012816829897, -25.44940218233254825, -9.846743663894592657 ) ) ;
#21689=ORIENTED_EDGE ( 'NONE', *, *, #17049, .T. ) ;
#21690=CARTESIAN_POINT ( 'NONE',  ( -0.7375392941519317569, 0.5000000000000004441, 14.98185688723470044 ) ) ;
#21699=EDGE_CURVE ( 'NONE', #81069, #38526, #84779, .T. ) ;
#21700=CARTESIAN_POINT ( 'NONE',  ( -3.434112377981067610, 28.08196800326376774, -12.81628187352647252 ) ) ;
#21716=DIRECTION ( 'NONE',  ( -0.000000000000000000, -1.000000000000000000, -0.000000000000000000 ) ) ;
#21718=CYLINDRICAL_SURFACE ( 'NONE', #97227, 15.00000000000000000 ) ;
#21733=CARTESIAN_POINT ( 'NONE',  ( -14.97653319723434073, -0.03417435944610275333, -5.619684139539446122 ) ) ;
#21739=AXIS2_PLACEMENT_3D ( 'NONE', #35362, #59338, #28359 ) ;
#21741=CARTESIAN_POINT ( 'NONE',  ( -2.933660812630105141, -0.03417435944610275333, 15.72485391577587954 ) ) ;
#21744=AXIS2_PLACEMENT_3D ( 'NONE', #705, #22703, #67705 ) ;
#21745=VERTEX_POINT ( 'NONE', #92881 ) ;
#21746=CARTESIAN_POINT ( 'NONE',  ( -3.881785064875084235, 2.270048298641524909E-16, -14.10213074188660443 ) ) ;
#21750=FACE_OUTER_BOUND ( 'NONE', #51258, .T. ) ;
#21757=CARTESIAN_POINT ( 'NONE',  ( 1.881370533971186143, 2.354751593366954943E-16, 14.50512983964829772 ) ) ;
#21758=CARTESIAN_POINT ( 'NONE',  ( -10.36894250292379205, 16.17874883491396432, -10.36894250292378672 ) ) ;
#21764=EDGE_CURVE ( 'NONE', #71998, #47390, #24414, .T. ) ;
#21767=ORIENTED_EDGE ( 'NONE', *, *, #8526, .T. ) ;
#21771=DIRECTION ( 'NONE',  ( 0.000000000000000000, 0.000000000000000000, 1.000000000000000000 ) ) ;
#21773=CARTESIAN_POINT ( 'NONE',  ( 1.460619146402132233E-15, 13.17686044187655270, -11.92686044187656513 ) ) ;
#21776=ORIENTED_EDGE ( 'NONE', *, *, #55835, .F. ) ;
#21791=ORIENTED_EDGE ( 'NONE', *, *, #94605, .F. ) ;
#21806=ORIENTED_EDGE ( 'NONE', *, *, #54731, .F. ) ;
#21809=EDGE_LOOP ( 'NONE', ( #96877, #26854, #12450, #58338 ) ) ;
#21813=LINE ( 'NONE', #42827, #80824 ) ;
#21816=EDGE_CURVE ( 'NONE', #47923, #79627, #20100, .T. ) ;
#21820=ADVANCED_FACE ( 'NONE', ( #86382 ), #78873, .T. ) ;
#21821=ORIENTED_EDGE ( 'NONE', *, *, #94151, .T. ) ;
#21823=ORIENTED_EDGE ( 'NONE', *, *, #53278, .F. ) ;
#21824=EDGE_LOOP ( 'NONE', ( #77873, #7603, #22098, #60568 ) ) ;
#21826=B_SPLINE_CURVE_WITH_KNOTS ( 'NONE', 3,
 ( #28010, #4546, #27518, #58009, #49045, #50521 ),
 .UNSPECIFIED., .F., .F.,
 ( 4, 2, 4 ),
 ( 0.0002800011564896255026, 0.0006862063972211533995, 0.001092411637952681296 ),
 .UNSPECIFIED. ) ;
#21844=CARTESIAN_POINT ( 'NONE',  ( 0.000000000000000000, 0.000000000000000000, 0.000000000000000000 ) ) ;
#21850=VECTOR ( 'NONE', #93133, 1000.000000000000114 ) ;
#21856=EDGE_CURVE ( 'NONE', #13218, #9024, #64184, .T. ) ;
#21862=EDGE_CURVE ( 'NONE', #49345, #23295, #50327, .T. ) ;
#21864=CIRCLE ( 'NONE', #69756, 15.00000000000000000 ) ;
#21875=ORIENTED_EDGE ( 'NONE', *, *, #43513, .F. ) ;
#21877=CARTESIAN_POINT ( 'NONE',  ( 11.92686044187656336, 2.188309369127512838, -2.602085213965210642E-15 ) ) ;
#21881=EDGE_LOOP ( 'NONE', ( #10896, #41179, #79115, #85768, #19567, #37324 ) ) ;
#21886=LINE ( 'NONE', #19895, #85420 ) ;
#21899=CARTESIAN_POINT ( 'NONE',  ( 9.997910040112596874, 15.00000000000000000, -10.50199004140715253 ) ) ;
#21900=DIRECTION ( 'NONE',  ( -0.000000000000000000, -1.000000000000000000, -0.000000000000000000 ) ) ;
#21906=CARTESIAN_POINT ( 'NONE',  ( -9.509319644403765537, 13.17686044187662020, 7.198808227794258663 ) ) ;
#21908=TOROIDAL_SURFACE ( 'NONE', #44352, 14.49999999999999822, 0.5000000000000000000 ) ;
#21916=CARTESIAN_POINT ( 'NONE',  ( 4.873787042390789637, 15.00000000000000000, -13.39061984619918988 ) ) ;
#21925=EDGE_CURVE ( 'NONE', #81593, #7375, #89417, .T. ) ;
#21929=FACE_OUTER_BOUND ( 'NONE', #98439, .T. ) ;
#21946=ORIENTED_EDGE ( 'NONE', *, *, #72467, .F. ) ;
#21948=CARTESIAN_POINT ( 'NONE',  ( 6.408140936763243367, -19.20969866340291077, 11.09922568453594494 ) ) ;
#21957=CARTESIAN_POINT ( 'NONE',  ( -14.49120296996859558, 14.95077488074853456, 2.766068805437424949 ) ) ;
#21964=ORIENTED_EDGE ( 'NONE', *, *, #61050, .F. ) ;
#21965=VECTOR ( 'NONE', #71242, 1000.000000000000000 ) ;
#21973=CIRCLE ( 'NONE', #37900, 15.00000000000000000 ) ;
#21974=CARTESIAN_POINT ( 'NONE',  ( 3.897244926436223444, 15.00000000000000000, -13.96644127841327787 ) ) ;
#21975=CARTESIAN_POINT ( 'NONE',  ( 7.154372922009559765, 15.00000000000000000, -14.30707323420376831 ) ) ;
#21977=EDGE_LOOP ( 'NONE', ( #87211, #66920, #6096, #41851 ) ) ;
#21978=EDGE_CURVE ( 'NONE', #70649, #88318, #71296, .T. ) ;
#21981=CYLINDRICAL_SURFACE ( 'NONE', #27854, 15.00000000000000000 ) ;
#22001=CARTESIAN_POINT ( 'NONE',  ( 12.26659068614894821, -21.11291783175269643, 7.082119434687044190 ) ) ;
#22005=ORIENTED_EDGE ( 'NONE', *, *, #45495, .F. ) ;
#22011=CARTESIAN_POINT ( 'NONE',  ( 2.913501739333663743, 15.00000000000000000, 14.20427779279537184 ) ) ;
#22017=CARTESIAN_POINT ( 'NONE',  ( 10.88017736071110519, 25.56368534415484461, -2.602085213965210642E-15 ) ) ;
#22028=AXIS2_PLACEMENT_3D ( 'NONE', #14556, #5575, #21559 ) ;
#22036=ORIENTED_EDGE ( 'NONE', *, *, #67143, .T. ) ;
#22041=CARTESIAN_POINT ( 'NONE',  ( 3.420591144908446957, 15.00000000000000000, 14.60477854057958425 ) ) ;
#22046=CARTESIAN_POINT ( 'NONE',  ( -14.17193700899791153, 0.000000000000000000, 1.489530601563921808 ) ) ;
#22048=CARTESIAN_POINT ( 'NONE',  ( 9.402796353261066997, 14.49999999999999112, 11.68706210897770070 ) ) ;
#22052=ORIENTED_EDGE ( 'NONE', *, *, #63005, .T. ) ;
#22055=EDGE_CURVE ( 'NONE', #31483, #55265, #49838, .T. ) ;
#22066=DIRECTION ( 'NONE',  ( 0.000000000000000000, 1.000000000000000000, 0.000000000000000000 ) ) ;
#22067=CARTESIAN_POINT ( 'NONE',  ( -8.527530157486182816, 20.59226448433412671, -4.923371831947288335 ) ) ;
#22069=ORIENTED_EDGE ( 'NONE', *, *, #65811, .T. ) ;
#22070=LINE ( 'NONE', #30526, #52568 ) ;
#22080=ORIENTED_EDGE ( 'NONE', *, *, #3915, .T. ) ;
#22095=VERTEX_POINT ( 'NONE', #35328 ) ;
#22098=ORIENTED_EDGE ( 'NONE', *, *, #15413, .T. ) ;
#22099=CYLINDRICAL_SURFACE ( 'NONE', #80964, 15.00000000000000000 ) ;
#22108=CARTESIAN_POINT ( 'NONE',  ( 0.000000000000000000, 14.49999999999999822, 0.000000000000000000 ) ) ;
#22111=VECTOR ( 'NONE', #12567, 1000.000000000000114 ) ;
#22114=ORIENTED_EDGE ( 'NONE', *, *, #6089, .T. ) ;
#22122=B_SPLINE_CURVE_WITH_KNOTS ( 'NONE', 3,
 ( #92739, #84277, #55227, #24263, #93720, #9739 ),
 .UNSPECIFIED., .F., .F.,
 ( 4, 2, 4 ),
 ( 3.409110551494637202E-05, 0.0004400426677367930768, 0.0008459942299586397816 ),
 .UNSPECIFIED. ) ;
#22124=DIRECTION ( 'NONE',  ( -0.000000000000000000, -1.000000000000000000, -0.000000000000000000 ) ) ;
#22127=CARTESIAN_POINT ( 'NONE',  ( -10.88017736071110342, -11.93631465584515894, 3.903127820947815962E-15 ) ) ;
#22131=ADVANCED_FACE ( 'NONE', ( #58313 ), #20340, .F. ) ;
#22132=CARTESIAN_POINT ( 'NONE',  ( 14.11874224319630855, 0.2301510088455456793, -4.887061453530034072 ) ) ;
#22136=DIRECTION ( 'NONE',  ( 0.000000000000000000, 0.000000000000000000, 1.000000000000000000 ) ) ;
#22148=AXIS2_PLACEMENT_3D ( 'NONE', #63193, #55712, #86209 ) ;
#22150=CARTESIAN_POINT ( 'NONE',  ( 0.000000000000000000, 0.5000000000000004441, 0.000000000000000000 ) ) ;
#22153=LINE ( 'NONE', #59645, #32155 ) ;
#22155=ORIENTED_EDGE ( 'NONE', *, *, #6440, .T. ) ;
#22156=ORIENTED_EDGE ( 'NONE', *, *, #86479, .F. ) ;
#22160=EDGE_CURVE ( 'NONE', #53609, #71459, #79854, .T. ) ;
#22171=CARTESIAN_POINT ( 'NONE',  ( 7.551349515323100725, 0.000000000000000000, 12.08468537022911349 ) ) ;
#22175=CARTESIAN_POINT ( 'NONE',  ( 4.923371831947295441, -20.65773551566587685, -8.527530157486179263 ) ) ;
#22179=CARTESIAN_POINT ( 'NONE',  ( 6.689969769698956625, 15.00000000000000000, -12.58200319823970226 ) ) ;
#22180=B_SPLINE_CURVE_WITH_KNOTS ( 'NONE', 3,
 ( #15709, #47153, #77656, #9170, #39688, #1692 ),
 .UNSPECIFIED., .F., .F.,
 ( 4, 2, 4 ),
 ( 0.0002800553958269923053, 0.0006862611673083280749, 0.001092466938789663899 ),
 .UNSPECIFIED. ) ;
#22193=CARTESIAN_POINT ( 'NONE',  ( -11.09922568453594316, 24.54030133659709634, 6.408140936763246920 ) ) ;
#22210=ORIENTED_EDGE ( 'NONE', *, *, #14370, .T. ) ;
#22211=CARTESIAN_POINT ( 'NONE',  ( -3.270351084886894188, 14.95037111082768710, 14.38617789677959991 ) ) ;
#22212=DIRECTION ( 'NONE',  ( 0.000000000000000000, 1.000000000000000000, 0.000000000000000000 ) ) ;
#22220=ORIENTED_EDGE ( 'NONE', *, *, #64702, .T. ) ;
#22221=CIRCLE ( 'NONE', #63654, 15.00000000000000000 ) ;
#22223=DIRECTION ( 'NONE',  ( -0.000000000000000000, -1.000000000000000000, -0.000000000000000000 ) ) ;
#22233=CARTESIAN_POINT ( 'NONE',  ( -11.81378540890925066, 15.00000000000000000, -7.968498874458281200 ) ) ;
#22236=CARTESIAN_POINT ( 'NONE',  ( -10.58981376305295008, 15.00000000000000000, 9.535111140613638625 ) ) ;
#22248=CARTESIAN_POINT ( 'NONE',  ( 14.16423886937410259, 19.30374883491398208, -2.602085213965210642E-15 ) ) ;
#22252=CARTESIAN_POINT ( 'NONE',  ( 3.384479038598308343, 14.76984929998921636, -14.55223509985378350 ) ) ;
#22253=CIRCLE ( 'NONE', #54139, 13.75000000000001776 ) ;
#22255=EDGE_CURVE ( 'NONE', #7251, #33002, #83800, .T. ) ;
#22258=ORIENTED_EDGE ( 'NONE', *, *, #73127, .T. ) ;
#22265=CARTESIAN_POINT ( 'NONE',  ( 2.393480905993052854, 0.5000000000000004441, 14.80781041047752922 ) ) ;
#22272=CARTESIAN_POINT ( 'NONE',  ( 0.000000000000000000, 14.49999999999999822, 0.000000000000000000 ) ) ;
#22283=AXIS2_PLACEMENT_3D ( 'NONE', #8014, #76988, #23522 ) ;
#22285=VERTEX_POINT ( 'NONE', #30779 ) ;
#22287=DIRECTION ( 'NONE',  ( 0.8870108331782150524, 0.000000000000000000, 0.4617486132350466232 ) ) ;
#22293=CARTESIAN_POINT ( 'NONE',  ( 10.58521204051726627, 15.00000000000000000, 11.99294302885416563 ) ) ;
#22294=DIRECTION ( 'NONE',  ( -0.6755902076156641289, 0.000000000000000000, 0.7372773368101204206 ) ) ;
#22303=VERTEX_POINT ( 'NONE', #14326 ) ;
#22307=VERTEX_POINT ( 'NONE', #28812 ) ;
#22311=AXIS2_PLACEMENT_3D ( 'NONE', #1863, #79310, #3314 ) ;
#22312=CARTESIAN_POINT ( 'NONE',  ( 0.000000000000000000, 14.49999999999999822, 0.000000000000000000 ) ) ;
#22322=CARTESIAN_POINT ( 'NONE',  ( -8.606322355891443010, 3.794835101497137347E-16, 11.66967075398801335 ) ) ;
#22324=DIRECTION ( 'NONE',  ( -0.000000000000000000, -1.000000000000000000, -0.000000000000000000 ) ) ;
#22328=ORIENTED_EDGE ( 'NONE', *, *, #47764, .F. ) ;
#22345=DIRECTION ( 'NONE',  ( -0.000000000000000000, -1.000000000000000000, -0.000000000000000000 ) ) ;
#22355=ORIENTED_EDGE ( 'NONE', *, *, #24095, .F. ) ;
#22356=ADVANCED_FACE ( 'NONE', ( #30286 ), #90292, .F. ) ;
#22363=CARTESIAN_POINT ( 'NONE',  ( 9.876730923139232843, 14.63595249122789177, 11.28938378619070271 ) ) ;
#22368=FACE_OUTER_BOUND ( 'NONE', #42683, .T. ) ;
#22373=LINE ( 'NONE', #76345, #14591 ) ;
#22377=EDGE_CURVE ( 'NONE', #54264, #93214, #62219, .T. ) ;
#22379=DIRECTION ( 'NONE',  ( -0.9636304532086211738, 0.000000000000000000, -0.2672383760782636175 ) ) ;
#22380=CARTESIAN_POINT ( 'NONE',  ( -13.16767742306207545, 14.95037115938073491, -6.653539137814823867 ) ) ;
#22386=VERTEX_POINT ( 'NONE', #22811 ) ;
#22411=EDGE_CURVE ( 'NONE', #68868, #3541, #14827, .T. ) ;
#22415=ORIENTED_EDGE ( 'NONE', *, *, #13989, .T. ) ;
#22417=CIRCLE ( 'NONE', #78278, 14.49999999999999822 ) ;
#22438=CARTESIAN_POINT ( 'NONE',  ( -3.434112377981047626, -14.83469866340291610, 12.81628187352647963 ) ) ;
#22447=CARTESIAN_POINT ( 'NONE',  ( -9.399392868737665552, 3.795627280083113010E-16, -11.04089732309487104 ) ) ;
#22448=VERTEX_POINT ( 'NONE', #45805 ) ;
#22461=CARTESIAN_POINT ( 'NONE',  ( -7.771322705631315664, 15.00000000000000000, -12.24159072199926257 ) ) ;
#22481=ADVANCED_FACE ( 'NONE', ( #29305 ), #51324, .F. ) ;
#22482=CARTESIAN_POINT ( 'NONE',  ( 0.000000000000000000, 0.5000000000000004441, 0.000000000000000000 ) ) ;
#22491=CARTESIAN_POINT ( 'NONE',  ( 14.16423886937410259, -20.69625116508602858, -2.602085213965210642E-15 ) ) ;
#22503=DIRECTION ( 'NONE',  ( 0.000000000000000000, 0.000000000000000000, 1.000000000000000000 ) ) ;
#22505=LINE ( 'NONE', #52977, #26238 ) ;
#22508=CARTESIAN_POINT ( 'NONE',  ( -10.88017736071110342, 23.06368534415484461, 3.903127820947815962E-15 ) ) ;
#22514=EDGE_LOOP ( 'NONE', ( #43675, #11998, #10517, #90710 ) ) ;
#22523=( BOUNDED_CURVE ( )  B_SPLINE_CURVE ( 2, ( #44220, #74724, #42269, #72740, #4273, #34747, #65236, #95761, #27246, #19754, #80754 ),
 .UNSPECIFIED., .F., .F. ) 
 B_SPLINE_CURVE_WITH_KNOTS ( ( 3, 2, 2, 2, 2, 3 ),
 ( 0.5443736480827608970, 0.5444444444444443976, 0.5500000000000000444, 0.5555555555555555802, 0.5611111111111111160, 0.5666666666666666519 ),
 .UNSPECIFIED. ) 
 CURVE ( )  GEOMETRIC_REPRESENTATION_ITEM ( )  RATIONAL_B_SPLINE_CURVE ( ( 0.9991426288945820522, 0.9995657810453010272, 1.000000000000000000, 0.9659258262890683122, 1.000000000000000000, 0.9659258262890683122, 1.000000000000000000, 0.9659258262890683122, 1.000000000000000000, 0.9659258262890683122, 1.000000000000000000 ) ) 
 REPRESENTATION_ITEM ( '' )  );
#22527=CARTESIAN_POINT ( 'NONE',  ( -9.065164099344672266, 14.49999999999999112, 11.95084933600764820 ) ) ;
#22531=EDGE_CURVE ( 'NONE', #50677, #48484, #31269, .T. ) ;
#22534=CARTESIAN_POINT ( 'NONE',  ( 11.35178980618967337, 14.49999999999999822, 9.804941009311999522 ) ) ;
#22539=VECTOR ( 'NONE', #74206, 1000.000000000000000 ) ;
#22543=VERTEX_POINT ( 'NONE', #31766 ) ;
#22550=CARTESIAN_POINT ( 'NONE',  ( 3.897244926435189161, 15.00000000000000000, 13.96644127842154148 ) ) ;
#22555=DIRECTION ( 'NONE',  ( -0.7489557207889991908, 0.000000000000000000, -0.6626200482157409422 ) ) ;
#22559=CARTESIAN_POINT ( 'NONE',  ( -2.638427012816840111, 9.967264484334121377, -9.846743663894590881 ) ) ;
#22582=TOROIDAL_SURFACE ( 'NONE', #84807, 14.49999999999999822, 0.5000000000000000000 ) ;
#22586=ORIENTED_EDGE ( 'NONE', *, *, #89735, .F. ) ;
#22607=AXIS2_PLACEMENT_3D ( 'NONE', #76795, #7335, #83319 ) ;
#22609=ORIENTED_EDGE ( 'NONE', *, *, #54863, .F. ) ;
#22611=EDGE_CURVE ( 'NONE', #32046, #13614, #63246, .T. ) ;
#22616=CIRCLE ( 'NONE', #92825, 15.00000000000000000 ) ;
#22623=CARTESIAN_POINT ( 'NONE',  ( 9.422509992056141925, -14.85298132251182324, 5.440088680355547268 ) ) ;
#22628=CARTESIAN_POINT ( 'NONE',  ( 13.07964015051225104, 0.2306972965111895035, -7.222261988160741275 ) ) ;
#22629=CARTESIAN_POINT ( 'NONE',  ( -14.36383853300403501, 0.04962896932678149270, -3.367113227849129586 ) ) ;
#22639=ORIENTED_EDGE ( 'NONE', *, *, #17049, .F. ) ;
#22653=DIRECTION ( 'NONE',  ( 0.000000000000000000, 0.000000000000000000, 1.000000000000000000 ) ) ;
#22672=CARTESIAN_POINT ( 'NONE',  ( 9.846743663894594434, -21.49106884899921255, -2.168404344971008868E-15 ) ) ;
#22685=VECTOR ( 'NONE', #39106, 1000.000000000000000 ) ;
#22687=CARTESIAN_POINT ( 'NONE',  ( 9.382169495545415572, 22.24863466993043204, -9.382169495545422677 ) ) ;
#22688=ORIENTED_EDGE ( 'NONE', *, *, #94306, .T. ) ;
#22692=ORIENTED_EDGE ( 'NONE', *, *, #76212, .T. ) ;
#22698=CARTESIAN_POINT ( 'NONE',  ( 6.382347221874423937, 15.00000000000000000, -13.57444820018227638 ) ) ;
#22699=CARTESIAN_POINT ( 'NONE',  ( 0.9082943533636174127, 4.777657996272472852E-16, 14.47152380945585648 ) ) ;
#22703=DIRECTION ( 'NONE',  ( 0.000000000000000000, 1.000000000000000000, 0.000000000000000000 ) ) ;
#22704=CARTESIAN_POINT ( 'NONE',  ( -3.420591144908668557, 14.63606885998604490, 14.60477854057957003 ) ) ;
#22706=VERTEX_POINT ( 'NONE', #47259 ) ;
#22711=FACE_OUTER_BOUND ( 'NONE', #45134, .T. ) ;
#22712=DIRECTION ( 'NONE',  ( -0.000000000000000000, -1.000000000000000000, -0.000000000000000000 ) ) ;
#22713=DIRECTION ( 'NONE',  ( 0.000000000000000000, 0.000000000000000000, 1.000000000000000000 ) ) ;
#22717=DIRECTION ( 'NONE',  ( 0.9953961983671778535, 0.000000000000000000, 0.09584575252023383451 ) ) ;
#22723=DIRECTION ( 'NONE',  ( 0.3987490689252466414, 0.000000000000000000, 0.9170600743851238246 ) ) ;
#22724=AXIS2_PLACEMENT_3D ( 'NONE', #18726, #41242, #39756 ) ;
#22728=EDGE_CURVE ( 'NONE', #37192, #5083, #101, .T. ) ;
#22729=CARTESIAN_POINT ( 'NONE',  ( 6.715867195167361636, 4.143177415744058416E-16, 12.85095824508331930 ) ) ;
#22733=LINE ( 'NONE', #51743, #90337 ) ;
#22741=CARTESIAN_POINT ( 'NONE',  ( 3.469446951953614189E-15, 18.05374883491397853, 14.16423886937410259 ) ) ;
#22748=ORIENTED_EDGE ( 'NONE', *, *, #97611, .T. ) ;
#22755=VECTOR ( 'NONE', #88601, 999.9999999999998863 ) ;
#22763=DIRECTION ( 'NONE',  ( 0.000000000000000000, 1.000000000000000000, 0.000000000000000000 ) ) ;
#22770=VECTOR ( 'NONE', #7985, 1000.000000000000000 ) ;
#22771=DIRECTION ( 'NONE',  ( 4.263256414560601746E-14, 0.000000000000000000, 1.000000000000000000 ) ) ;
#22776=VERTEX_POINT ( 'NONE', #39784 ) ;
#22777=ORIENTED_EDGE ( 'NONE', *, *, #45451, .T. ) ;
#22779=DIRECTION ( 'NONE',  ( -0.9981347984218665870, 0.000000000000000000, -0.06104853953486361756 ) ) ;
#22793=ORIENTED_EDGE ( 'NONE', *, *, #66846, .F. ) ;
#22800=DIRECTION ( 'NONE',  ( 3.730349362740525976E-14, 0.000000000000000000, 1.000000000000000000 ) ) ;
#22801=ORIENTED_EDGE ( 'NONE', *, *, #47541, .T. ) ;
#22807=ORIENTED_EDGE ( 'NONE', *, *, #87764, .T. ) ;
#22808=ORIENTED_EDGE ( 'NONE', *, *, #704, .F. ) ;
#22811=CARTESIAN_POINT ( 'NONE',  ( 9.159723438033129383, 15.00000000000000000, 10.91613331444548507 ) ) ;
#22814=EDGE_CURVE ( 'NONE', #8560, #33923, #25285, .T. ) ;
#22815=AXIS2_PLACEMENT_3D ( 'NONE', #51402, #60372, #44388 ) ;
#22816=ORIENTED_EDGE ( 'NONE', *, *, #60765, .T. ) ;
#22820=AXIS2_PLACEMENT_3D ( 'NONE', #51619, #14622, #43610 ) ;
#22830=LINE ( 'NONE', #61787, #70498 ) ;
#22835=CARTESIAN_POINT ( 'NONE',  ( -7.595945211628163385, 15.00000000000000000, -12.35117874301652030 ) ) ;
#22838=CARTESIAN_POINT ( 'NONE',  ( 0.000000000000000000, 0.000000000000000000, 0.000000000000000000 ) ) ;
#22845=ADVANCED_FACE ( 'NONE', ( #86260 ), #47761, .F. ) ;
#22849=CARTESIAN_POINT ( 'NONE',  ( 0.9940297508537879745, -0.03417435944610275333, -14.21528771620249820 ) ) ;
#22867=AXIS2_PLACEMENT_3D ( 'NONE', #27220, #20725, #66205 ) ;
#22869=DIRECTION ( 'NONE',  ( 0.000000000000000000, 0.000000000000000000, 1.000000000000000000 ) ) ;
#22873=LINE ( 'NONE', #16839, #45155 ) ;
#22874=CARTESIAN_POINT ( 'NONE',  ( -13.34343830728397329, 14.63606867472037720, -6.852200678592815564 ) ) ;
#22889=CARTESIAN_POINT ( 'NONE',  ( 14.48718990079892599, 4.585916678612670543E-16, -0.6093675230840440715 ) ) ;
#22891=LINE ( 'NONE', #76370, #51330 ) ;
#22894=CARTESIAN_POINT ( 'NONE',  ( 5.795997163830076460, -0.03417435944610275333, 13.01802277140709663 ) ) ;
#22906=DIRECTION ( 'NONE',  ( 0.8526401643540846287, 0.000000000000000000, 0.5224985647159611224 ) ) ;
#22914=ORIENTED_EDGE ( 'NONE', *, *, #26120, .F. ) ;
#22920=ORIENTED_EDGE ( 'NONE', *, *, #66589, .T. ) ;
#22926=B_SPLINE_CURVE_WITH_KNOTS ( 'NONE', 3,
 ( #59117, #37136, #89134, #52612, #60605, #83616 ),
 .UNSPECIFIED., .F., .F.,
 ( 4, 2, 4 ),
 ( 3.409110551494638557E-05, 0.0004400426677367922637, 0.0008459942299586381553 ),
 .UNSPECIFIED. ) ;
#22927=DIRECTION ( 'NONE',  ( 0.000000000000000000, 1.000000000000000000, 0.000000000000000000 ) ) ;
#22928=B_SPLINE_CURVE_WITH_KNOTS ( 'NONE', 3,
 ( #30233, #43761, #36773, #83254, #28763, #67767 ),
 .UNSPECIFIED., .F., .F.,
 ( 4, 2, 4 ),
 ( 0.0002800056097852249184, 0.0006862108940693780260, 0.001092416178353531079 ),
 .UNSPECIFIED. ) ;
#22933=ORIENTED_EDGE ( 'NONE', *, *, #21856, .T. ) ;
#22935=CARTESIAN_POINT ( 'NONE',  ( 11.09922568453594671, -2.959698663402905883, -6.408140936763241591 ) ) ;
#22949=VERTEX_POINT ( 'NONE', #95219 ) ;
#22957=EDGE_CURVE ( 'NONE', #70902, #2423, #86755, .T. ) ;
#22964=DIRECTION ( 'NONE',  ( 0.8788171126619711560, 0.000000000000000000, -0.4771587602595978028 ) ) ;
#22966=ORIENTED_EDGE ( 'NONE', *, *, #31079, .F. ) ;
#22973=ADVANCED_FACE ( 'NONE', ( #11728 ), #73205, .T. ) ;
#22974=VECTOR ( 'NONE', #19926, 1000.000000000000000 ) ;
#22981=CARTESIAN_POINT ( 'NONE',  ( -11.25000000000000178, 10.11803362898265846, 3.674383000693412496E-15 ) ) ;
#22985=LINE ( 'NONE', #69451, #77001 ) ;
#22990=CARTESIAN_POINT ( 'NONE',  ( -10.36894250292379205, -3.821251165086027246, -10.36894250292378672 ) ) ;
#22994=ORIENTED_EDGE ( 'NONE', *, *, #19435, .F. ) ;
#23005=CARTESIAN_POINT ( 'NONE',  ( -7.964842623401172439, 33.68868534415485527, 7.964842623401183097 ) ) ;
#23012=VERTEX_POINT ( 'NONE', #41756 ) ;
#23016=FACE_OUTER_BOUND ( 'NONE', #76694, .T. ) ;
#23023=ORIENTED_EDGE ( 'NONE', *, *, #35057, .F. ) ;
#23032=LINE ( 'NONE', #38519, #20328 ) ;
#23036=DIRECTION ( 'NONE',  ( 0.000000000000000000, 0.000000000000000000, 1.000000000000000000 ) ) ;
#23037=ORIENTED_EDGE ( 'NONE', *, *, #63126, .F. ) ;
#23053=CARTESIAN_POINT ( 'NONE',  ( 7.208316651077764980, 17.88393115100078745, 7.208316651077762316 ) ) ;
#23055=CARTESIAN_POINT ( 'NONE',  ( 0.000000000000000000, 15.00000000000000000, 0.000000000000000000 ) ) ;
#23056=EDGE_CURVE ( 'NONE', #63858, #89913, #48737, .T. ) ;
#23057=ORIENTED_EDGE ( 'NONE', *, *, #51230, .T. ) ;
#23066=EDGE_CURVE ( 'NONE', #48953, #84655, #3255, .T. ) ;
#23069=ORIENTED_EDGE ( 'NONE', *, *, #75508, .T. ) ;
#23074=ORIENTED_EDGE ( 'NONE', *, *, #36622, .T. ) ;
#23078=DIRECTION ( 'NONE',  ( 0.7604059656000387024, 0.000000000000000000, -0.6494480483301745544 ) ) ;
#23084=ORIENTED_EDGE ( 'NONE', *, *, #60532, .T. ) ;
#23091=CARTESIAN_POINT ( 'NONE',  ( 3.897244926436124857, 3.990182060915936250E-16, 13.96644127841333294 ) ) ;
#23101=DIRECTION ( 'NONE',  ( 0.9914448613738086058, 0.000000000000000000, 0.1305261922200653124 ) ) ;
#23105=VERTEX_POINT ( 'NONE', #13701 ) ;
#23113=CARTESIAN_POINT ( 'NONE',  ( 0.000000000000000000, 0.5000000000000004441, 0.000000000000000000 ) ) ;
#23116=CARTESIAN_POINT ( 'NONE',  ( 0.000000000000000000, 15.00000000000000000, 0.000000000000000000 ) ) ;
#23119=CARTESIAN_POINT ( 'NONE',  ( -5.440088680355547268, -6.102981322511823237, 9.422509992056143702 ) ) ;
#23129=LINE ( 'NONE', #98149, #41175 ) ;
#23134=CARTESIAN_POINT ( 'NONE',  ( 9.402796353261136275, 0.3639308891339645968, -11.68706210897760833 ) ) ;
#23136=ORIENTED_EDGE ( 'NONE', *, *, #4848, .F. ) ;
#23139=DIRECTION ( 'NONE',  ( 0.1478094111295981949, 0.000000000000000000, 0.9890158633619187123 ) ) ;
#23148=ADVANCED_FACE ( 'NONE', ( #29672 ), #6206, .F. ) ;
#23149=PLANE ( 'NONE',  #28942 ) ;
#23151=EDGE_LOOP ( 'NONE', ( #52189, #38969, #25874, #80178 ) ) ;
#23157=CARTESIAN_POINT ( 'NONE',  ( 5.428133280998944876, 0.000000000000000000, -0.5226697871167509390 ) ) ;
#23164=CARTESIAN_POINT ( 'NONE',  ( -9.065164099344649173, 14.63606892172464136, 11.95084933600763399 ) ) ;
#23167=CARTESIAN_POINT ( 'NONE',  ( 2.638427012816829897, -20.44940218233254470, -9.846743663894592657 ) ) ;
#23168=EDGE_LOOP ( 'NONE', ( #13376, #4583, #316, #82008, #75846, #4304 ) ) ;
#23178=CARTESIAN_POINT ( 'NONE',  ( 0.000000000000000000, 15.00000000000000000, 0.000000000000000000 ) ) ;
#23182=CARTESIAN_POINT ( 'NONE',  ( 12.81628187352647608, 26.41530133659709989, 3.434112377981052511 ) ) ;
#23184=ORIENTED_EDGE ( 'NONE', *, *, #67276, .T. ) ;
#23188=ORIENTED_EDGE ( 'NONE', *, *, #90448, .T. ) ;
#23197=CARTESIAN_POINT ( 'NONE',  ( -3.897244926436316703, 15.00000000000000000, 13.96644127841325300 ) ) ;
#23200=CARTESIAN_POINT ( 'NONE',  ( -9.065164099344400483, 0.3639310782753642504, -11.95084933600781341 ) ) ;
#23201=ORIENTED_EDGE ( 'NONE', *, *, #71865, .T. ) ;
#23202=CARTESIAN_POINT ( 'NONE',  ( 10.19513985507835763, 14.49999999999999112, -11.00268709613223450 ) ) ;
#23204=DIRECTION ( 'NONE',  ( 3.552713678800500929E-14, 0.000000000000000000, 1.000000000000000000 ) ) ;
#23207=EDGE_CURVE ( 'NONE', #62480, #29582, #52683, .T. ) ;
#23211=FACE_OUTER_BOUND ( 'NONE', #12420, .T. ) ;
#23215=CARTESIAN_POINT ( 'NONE',  ( -14.03351048042399007, 0.000000000000000000, 2.474486531753619989 ) ) ;
#23223=CARTESIAN_POINT ( 'NONE',  ( 0.9082943533637201083, 4.650128654361622927E-16, -14.47152380945585115 ) ) ;
#23226=ORIENTED_EDGE ( 'NONE', *, *, #86995, .F. ) ;
#23227=DIRECTION ( 'NONE',  ( -0.000000000000000000, -1.000000000000000000, -0.000000000000000000 ) ) ;
#23231=CARTESIAN_POINT ( 'NONE',  ( -14.94699059465099822, 15.00000000000000000, -1.259949270175015013 ) ) ;
#23237=AXIS2_PLACEMENT_3D ( 'NONE', #81475, #50491, #42028 ) ;
#23240=CARTESIAN_POINT ( 'NONE',  ( -14.16423886937410437, 16.59541550158064283, -3.795296366450299885 ) ) ;
#23250=ORIENTED_EDGE ( 'NONE', *, *, #82865, .F. ) ;
#23260=ORIENTED_EDGE ( 'NONE', *, *, #23797, .F. ) ;
#23271=ADVANCED_FACE ( 'NONE', ( #37214 ), #44186, .F. ) ;
#23276=CARTESIAN_POINT ( 'NONE',  ( -14.97687855664612577, 0.3639309658595348829, 0.8325315005899682763 ) ) ;
#23277=CIRCLE ( 'NONE', #39259, 15.00000000000000000 ) ;
#23283=CARTESIAN_POINT ( 'NONE',  ( 10.84451454130507209, 4.631809541732465460E-16, -9.625305416630832056 ) ) ;
#23287=LINE ( 'NONE', #53765, #61855 ) ;
#23291=VERTEX_POINT ( 'NONE', #75681 ) ;
#23292=B_SPLINE_CURVE_WITH_KNOTS ( 'NONE', 3,
 ( #90115, #97163, #21642, #42175, #50146, #28631 ),
 .UNSPECIFIED., .F., .F.,
 ( 4, 2, 4 ),
 ( 0.0002800008091676911060, 0.0006862060465022900516, 0.001092411283836889051 ),
 .UNSPECIFIED. ) ;
#23295=VERTEX_POINT ( 'NONE', #7195 ) ;
#23296=AXIS2_PLACEMENT_3D ( 'NONE', #76221, #45719, #7734 ) ;
#23303=EDGE_CURVE ( 'NONE', #37161, #30649, #41623, .T. ) ;
#23304=AXIS2_PLACEMENT_3D ( 'NONE', #32342, #78340, #25845 ) ;
#23306=EDGE_LOOP ( 'NONE', ( #11193, #54128, #14522, #80202 ) ) ;
#23309=ORIENTED_EDGE ( 'NONE', *, *, #58713, .T. ) ;
#23312=CARTESIAN_POINT ( 'NONE',  ( 13.75801628063878645, 4.006593314786880238E-16, 4.578972376164555769 ) ) ;
#23317=CIRCLE ( 'NONE', #98340, 14.49999999999999822 ) ;
#23318=VERTEX_POINT ( 'NONE', #22699 ) ;
#23321=DIRECTION ( 'NONE',  ( -0.8038568606172125097, 0.000000000000000000, -0.5948227867513478095 ) ) ;
#23322=AXIS2_PLACEMENT_3D ( 'NONE', #73700, #13705, #65211 ) ;
#23326=PLANE ( 'NONE',  #24327 ) ;
#23329=DIRECTION ( 'NONE',  ( 0.000000000000000000, 1.000000000000000000, 0.000000000000000000 ) ) ;
#23347=CARTESIAN_POINT ( 'NONE',  ( -4.494156999534594021, 0.000000000000000000, -3.088748530746273868 ) ) ;
#23356=CARTESIAN_POINT ( 'NONE',  ( 6.767445849361247490, 0.5000000000000004441, -13.38662304974496564 ) ) ;
#23358=CARTESIAN_POINT ( 'NONE',  ( -13.14228782657333738, 0.3639308284105124414, -7.230509711182424581 ) ) ;
#23363=ORIENTED_EDGE ( 'NONE', *, *, #50335, .T. ) ;
#23375=B_SPLINE_CURVE_WITH_KNOTS ( 'NONE', 3,
 ( #42879, #65860, #11889, #12373, #27863, #42389 ),
 .UNSPECIFIED., .F., .F.,
 ( 4, 2, 4 ),
 ( 0.0002800032591452434271, 0.0006862085204419991757, 0.001092413781738754870 ),
 .UNSPECIFIED. ) ;
#23381=CARTESIAN_POINT ( 'NONE',  ( -14.62232599144295087, 15.00000000000000888, -0.3548652576990713459 ) ) ;
#23386=CARTESIAN_POINT ( 'NONE',  ( 14.40939250469963895, 15.00000000000000000, -1.618458416365745389 ) ) ;
#23390=EDGE_CURVE ( 'NONE', #38291, #42828, #65494, .T. ) ;
#23394=AXIS2_PLACEMENT_3D ( 'NONE', #22312, #85760, #26231 ) ;
#23401=( BOUNDED_CURVE ( )  B_SPLINE_CURVE ( 2, ( #73385, #25935, #49901, #50391, #35391, #58373, #65883, #56436, #96410, #88894, #20403, #50890, #40948 ),
 .UNSPECIFIED., .F., .F. ) 
 B_SPLINE_CURVE_WITH_KNOTS ( ( 3, 2, 2, 2, 2, 2, 3 ),
 ( 0.6666666666666667407, 0.6722222222222223875, 0.6777777777777779233, 0.6833333333333333481, 0.6888888888888888840, 0.6944444444444444198, 0.6999999999999999556 ),
 .UNSPECIFIED. ) 
 CURVE ( )  GEOMETRIC_REPRESENTATION_ITEM ( )  RATIONAL_B_SPLINE_CURVE ( ( 0.9999999999999993339, 0.9659258262890689783, 1.000000000000000000, 0.9659258262890683122, 1.000000000000000000, 0.9659258262890683122, 1.000000000000000000, 0.9659258262890683122, 1.000000000000000000, 0.9659258262890683122, 1.000000000000000000, 0.9659258262890683122, 1.000000000000000000 ) ) 
 REPRESENTATION_ITEM ( '' )  );
#23407=ORIENTED_EDGE ( 'NONE', *, *, #2058, .T. ) ;
#23413=VERTEX_POINT ( 'NONE', #97231 ) ;
#23416=DIRECTION ( 'NONE',  ( 0.000000000000000000, 0.000000000000000000, 1.000000000000000000 ) ) ;
#23449=CARTESIAN_POINT ( 'NONE',  ( -9.075906804202377387, -0.03417435944610275333, 13.17214151599831595 ) ) ;
#23453=CARTESIAN_POINT ( 'NONE',  ( 14.02068044289385718, 14.49999999999999112, -5.331089937175661930 ) ) ;
#23458=DIRECTION ( 'NONE',  ( 0.2334453638559024768, 0.000000000000000000, 0.9723699203976773342 ) ) ;
#23460=VERTEX_POINT ( 'NONE', #31154 ) ;
#23462=CARTESIAN_POINT ( 'NONE',  ( -1.457314710996519436, 0.000000000000000000, -5.254907083456964223 ) ) ;
#23465=AXIS2_PLACEMENT_3D ( 'NONE', #38695, #69194, #67716 ) ;
#23478=VECTOR ( 'NONE', #16735, 1000.000000000000227 ) ;
#23485=CARTESIAN_POINT ( 'NONE',  ( 3.469446951953614189E-15, -6.946251165086028578, 14.16423886937410259 ) ) ;
#23486=VECTOR ( 'NONE', #83637, 1000.000000000000000 ) ;
#23491=VERTEX_POINT ( 'NONE', #33972 ) ;
#23508=ORIENTED_EDGE ( 'NONE', *, *, #6093, .F. ) ;
#23510=EDGE_CURVE ( 'NONE', #24815, #64665, #77643, .T. ) ;
#23512=CARTESIAN_POINT ( 'NONE',  ( -13.74385066382887466, 14.76930270348882779, 5.860428621090259860 ) ) ;
#23514=EDGE_CURVE ( 'NONE', #39776, #81069, #37116, .T. ) ;
#23516=CIRCLE ( 'NONE', #81011, 14.49999999999999822 ) ;
#23519=CARTESIAN_POINT ( 'NONE',  ( 0.7375392941518293943, 0.5000000000000004441, -14.98185688723470932 ) ) ;
#23522=DIRECTION ( 'NONE',  ( 0.000000000000000000, 0.000000000000000000, -1.000000000000000000 ) ) ;
#23531=LINE ( 'NONE', #84998, #87286 ) ;
#23533=DIRECTION ( 'NONE',  ( -0.000000000000000000, -1.000000000000000000, -0.000000000000000000 ) ) ;
#23535=ORIENTED_EDGE ( 'NONE', *, *, #89345, .F. ) ;
#23542=CARTESIAN_POINT ( 'NONE',  ( -10.19513985507843223, 14.49999999999999112, 11.00268709613216522 ) ) ;
#23550=B_SPLINE_CURVE_WITH_KNOTS ( 'NONE', 3,
 ( #81135, #73628, #12638, #95145, #26655, #27141 ),
 .UNSPECIFIED., .F., .F.,
 ( 4, 2, 4 ),
 ( 0.0002800170536516727576, 0.0006862224498868463134, 0.001092427846122019869 ),
 .UNSPECIFIED. ) ;
#23552=CARTESIAN_POINT ( 'NONE',  ( -2.638427012816824124, 32.05059781766745886, 9.846743663894596210 ) ) ;
#23553=ORIENTED_EDGE ( 'NONE', *, *, #46190, .F. ) ;
#23554=DIRECTION ( 'NONE',  ( -0.000000000000000000, 1.000000000000000000, -0.000000000000000000 ) ) ;
#23568=VERTEX_POINT ( 'NONE', #54153 ) ;
#23576=CARTESIAN_POINT ( 'NONE',  ( -4.431036607602660382, 0.5000000000000004441, 14.33059365769907956 ) ) ;
#23579=ORIENTED_EDGE ( 'NONE', *, *, #72024, .F. ) ;
#23581=ORIENTED_EDGE ( 'NONE', *, *, #65000, .F. ) ;
#23582=VERTEX_POINT ( 'NONE', #26981 ) ;
#23583=CYLINDRICAL_SURFACE ( 'NONE', #74562, 15.00000000000000000 ) ;
#23586=CARTESIAN_POINT ( 'NONE',  ( -14.97687855664607248, 15.00000000000000000, -0.8325315005902533816 ) ) ;
#23588=AXIS2_PLACEMENT_3D ( 'NONE', #91198, #22723, #83711 ) ;
#23608=EDGE_CURVE ( 'NONE', #54278, #25526, #90760, .T. ) ;
#23613=DIRECTION ( 'NONE',  ( -0.000000000000000000, -1.000000000000000000, -0.000000000000000000 ) ) ;
#23614=VECTOR ( 'NONE', #18732, 1000.000000000000000 ) ;
#23618=CARTESIAN_POINT ( 'NONE',  ( -2.915334737309917656, -0.8946479891784895333, 10.88017736071110164 ) ) ;
#23623=AXIS2_PLACEMENT_3D ( 'NONE', #98386, #7369, #54315 ) ;
#23624=VECTOR ( 'NONE', #6733, 999.9999999999998863 ) ;
#23625=CARTESIAN_POINT ( 'NONE',  ( 13.75801628063881488, 4.740223025775510804E-16, -4.578972376164461622 ) ) ;
#23636=CARTESIAN_POINT ( 'NONE',  ( -10.14667048435152097, 4.576487713787624877E-16, 10.35833375027034542 ) ) ;
#23638=ORIENTED_EDGE ( 'NONE', *, *, #98139, .F. ) ;
#23647=LINE ( 'NONE', #16620, #23486 ) ;
#23651=ORIENTED_EDGE ( 'NONE', *, *, #67474, .F. ) ;
#23666=CARTESIAN_POINT ( 'NONE',  ( 7.208316651077762316, -5.866068848999215213, -7.208316651077764980 ) ) ;
#23668=DIRECTION ( 'NONE',  ( 0.9170600743851183845, 0.000000000000000000, 0.3987490689252593534 ) ) ;
#23680=CARTESIAN_POINT ( 'NONE',  ( 12.81628187352647608, 21.62363466993041783, -2.602085213965210642E-15 ) ) ;
#23694=EDGE_CURVE ( 'NONE', #54148, #37077, #20846, .T. ) ;
#23697=VERTEX_POINT ( 'NONE', #80853 ) ;
#23701=ORIENTED_EDGE ( 'NONE', *, *, #58102, .F. ) ;
#23704=CARTESIAN_POINT ( 'NONE',  ( 6.767445849361160448, 14.49999999999999112, 13.38662304974508110 ) ) ;
#23708=CARTESIAN_POINT ( 'NONE',  ( -9.705452947461587598, 2.500000000000008438, -5.689172442861014645 ) ) ;
#23713=CARTESIAN_POINT ( 'NONE',  ( -11.36220558718850882, 3.877685541201178108E-16, -9.008345252845398221 ) ) ;
#23728=CARTESIAN_POINT ( 'NONE',  ( -5.200846386093647133, 0.000000000000000000, 1.639820566680907588 ) ) ;
#23734=CARTESIAN_POINT ( 'NONE',  ( -10.36894250292379205, 21.17874883491397497, -10.36894250292378672 ) ) ;
#23736=EDGE_CURVE ( 'NONE', #73066, #74650, #61010, .T. ) ;
#23744=ADVANCED_FACE ( 'NONE', ( #57843 ), #54367, .T. ) ;
#23745=VERTEX_POINT ( 'NONE', #13339 ) ;
#23751=EDGE_CURVE ( 'NONE', #79627, #69540, #22417, .T. ) ;
#23769=VERTEX_POINT ( 'NONE', #12350 ) ;
#23778=CARTESIAN_POINT ( 'NONE',  ( 10.70613742633256926, 15.00000000000000000, -9.778988772285213571 ) ) ;
#23783=EDGE_CURVE ( 'NONE', #50106, #73111, #58829, .T. ) ;
#23786=AXIS2_PLACEMENT_3D ( 'NONE', #13209, #44191, #91177 ) ;
#23787=ORIENTED_EDGE ( 'NONE', *, *, #88420, .F. ) ;
#23791=ORIENTED_EDGE ( 'NONE', *, *, #58336, .F. ) ;
#23795=CARTESIAN_POINT ( 'NONE',  ( 3.881785064875274749, 15.00000000000000888, -14.10213074188652982 ) ) ;
#23796=EDGE_LOOP ( 'NONE', ( #80289, #5809, #63714, #61125, #83307, #12818, #20721, #26235, #17917, #30348, #93017, #16846 ) ) ;
#23797=EDGE_CURVE ( 'NONE', #43121, #72571, #15337, .T. ) ;
#23799=CARTESIAN_POINT ( 'NONE',  ( -7.684764310694971456, 0.5000000000000004441, 12.88194075009929840 ) ) ;
#23800=ORIENTED_EDGE ( 'NONE', *, *, #97888, .F. ) ;
#23802=ORIENTED_EDGE ( 'NONE', *, *, #33326, .T. ) ;
#23803=ORIENTED_EDGE ( 'NONE', *, *, #4755, .F. ) ;
#23806=CARTESIAN_POINT ( 'NONE',  ( 0.000000000000000000, 14.49999999999999822, 0.000000000000000000 ) ) ;
#23814=FACE_OUTER_BOUND ( 'NONE', #62761, .T. ) ;
#23817=CARTESIAN_POINT ( 'NONE',  ( 5.625000000000006217, 11.78470029564932098, 9.742785792574933268 ) ) ;
#23824=DIRECTION ( 'NONE',  ( -0.000000000000000000, -1.000000000000000000, -0.000000000000000000 ) ) ;
#23827=B_SPLINE_CURVE_WITH_KNOTS ( 'NONE', 3,
 ( #95226, #35209, #72716, #3262, #10764, #79746 ),
 .UNSPECIFIED., .F., .F.,
 ( 4, 2, 4 ),
 ( 0.0002800001171688649721, 0.0006862053477355121046, 0.001092410578302159237 ),
 .UNSPECIFIED. ) ;
#23831=CIRCLE ( 'NONE', #36596, 14.49999999999999822 ) ;
#23843=CARTESIAN_POINT ( 'NONE',  ( 9.820682251645100891, 14.76930270348881002, 11.26020669458365653 ) ) ;
#23854=PLANE ( 'NONE',  #72015 ) ;
#23858=LINE ( 'NONE', #69344, #3572 ) ;
#23859=CARTESIAN_POINT ( 'NONE',  ( 4.096035146093422341, 15.00000000000000000, 13.90943910019259810 ) ) ;
#23862=ADVANCED_FACE ( 'NONE', ( #29807 ), #23326, .F. ) ;
#23869=LINE ( 'NONE', #1373, #11734 ) ;
#23876=VECTOR ( 'NONE', #26559, 1000.000000000000000 ) ;
#23881=CARTESIAN_POINT ( 'NONE',  ( 5.240693273018990794, 0.04962883216462460334, 13.79102773477917232 ) ) ;
#23882=DIRECTION ( 'NONE',  ( 0.000000000000000000, 0.000000000000000000, 1.000000000000000000 ) ) ;
#23888=EDGE_CURVE ( 'NONE', #13765, #53769, #68815, .T. ) ;
#23889=LINE ( 'NONE', #69871, #44036 ) ;
#23897=VERTEX_POINT ( 'NONE', #37833 ) ;
#23906=CARTESIAN_POINT ( 'NONE',  ( 4.431036607602490740, 0.3639312379444061274, 14.33059365769916838 ) ) ;
#23910=CARTESIAN_POINT ( 'NONE',  ( -14.36383853300411140, 14.95037103067321560, 3.367113227848840040 ) ) ;
#23911=CARTESIAN_POINT ( 'NONE',  ( -14.62129639376012058, 15.00000000000000711, 0.3552502084984235919 ) ) ;
#23913=VERTEX_POINT ( 'NONE', #90306 ) ;
#23922=VECTOR ( 'NONE', #69499, 1000.000000000000000 ) ;
#23925=ORIENTED_EDGE ( 'NONE', *, *, #88430, .F. ) ;
#23932=CARTESIAN_POINT ( 'NONE',  ( 3.270351084886697457, 0.04962888917231522701, 14.38617789677964609 ) ) ;
#23942=FACE_OUTER_BOUND ( 'NONE', #58255, .T. ) ;
#23946=CARTESIAN_POINT ( 'NONE',  ( 11.36220558718861717, 15.00000000000000000, -9.008345252845218809 ) ) ;
#23964=CARTESIAN_POINT ( 'NONE',  ( 3.795296366450314540, -11.73791783175269821, 14.16423886937410082 ) ) ;
#23969=ORIENTED_EDGE ( 'NONE', *, *, #32257, .T. ) ;
#23976=ADVANCED_FACE ( 'NONE', ( #61295 ), #51832, .F. ) ;
#23982=CARTESIAN_POINT ( 'NONE',  ( 0.000000000000000000, 15.00000000000000000, 0.000000000000000000 ) ) ;
#23991=ORIENTED_EDGE ( 'NONE', *, *, #52463, .T. ) ;
#23992=AXIS2_PLACEMENT_3D ( 'NONE', #48973, #94473, #86974 ) ;
#24009=TOROIDAL_SURFACE ( 'NONE', #31967, 14.49999999999999822, 0.5000000000000000000 ) ;
#24012=CARTESIAN_POINT ( 'NONE',  ( 0.000000000000000000, 0.5000000000000004441, 0.000000000000000000 ) ) ;
#24016=EDGE_CURVE ( 'NONE', #71199, #67764, #93273, .T. ) ;
#24026=CARTESIAN_POINT ( 'NONE',  ( -3.014428414850141458, 11.88013551118487321, -11.24999999999999822 ) ) ;
#24027=CARTESIAN_POINT ( 'NONE',  ( -12.80781515976318907, 15.00000000000000000, 6.246788841744232990 ) ) ;
#24032=CARTESIAN_POINT ( 'NONE',  ( -1.514341385896341929, 15.00000000000000000, -15.92432625271835533 ) ) ;
#24034=CARTESIAN_POINT ( 'NONE',  ( 0.000000000000000000, 14.49999999999999822, 0.000000000000000000 ) ) ;
#24035=CARTESIAN_POINT ( 'NONE',  ( -4.923371831947292776, 26.84226448433413381, 8.527530157486181039 ) ) ;
#24036=ORIENTED_EDGE ( 'NONE', *, *, #54749, .T. ) ;
#24042=AXIS2_PLACEMENT_3D ( 'NONE', #79319, #41349, #79806 ) ;
#24045=VERTEX_POINT ( 'NONE', #10277 ) ;
#24053=AXIS2_PLACEMENT_3D ( 'NONE', #48563, #57049, #72534 ) ;
#24054=CARTESIAN_POINT ( 'NONE',  ( -5.419894505350392855, 0.5000000000000004441, -13.98659156302466045 ) ) ;
#24058=CARTESIAN_POINT ( 'NONE',  ( -10.09777502097869650, 0.04922511925147179945, -10.75551206493395107 ) ) ;
#24059=EDGE_CURVE ( 'NONE', #26051, #46052, #68102, .T. ) ;
#24065=ORIENTED_EDGE ( 'NONE', *, *, #63005, .F. ) ;
#24066=DIRECTION ( 'NONE',  ( -0.000000000000000000, -1.000000000000000000, -0.000000000000000000 ) ) ;
#24071=CARTESIAN_POINT ( 'NONE',  ( 0.000000000000000000, 14.49999999999999822, 0.000000000000000000 ) ) ;
#24072=DIRECTION ( 'NONE',  ( 0.000000000000000000, 0.000000000000000000, 1.000000000000000000 ) ) ;
#24087=VERTEX_POINT ( 'NONE', #16796 ) ;
#24093=LINE ( 'NONE', #54076, #16075 ) ;
#24095=EDGE_CURVE ( 'NONE', #91469, #29043, #92777, .T. ) ;
#24099=CARTESIAN_POINT ( 'NONE',  ( 7.964842623401177768, -3.811314655845160271, -7.964842623401181321 ) ) ;
#24103=DIRECTION ( 'NONE',  ( 0.000000000000000000, 0.000000000000000000, 1.000000000000000000 ) ) ;
#24105=CARTESIAN_POINT ( 'NONE',  ( -0.2849401152840977391, 14.76984969742594345, 14.93790629078302423 ) ) ;
#24127=DIRECTION ( 'NONE',  ( -0.000000000000000000, -1.000000000000000000, -0.000000000000000000 ) ) ;
#24129=ADVANCED_FACE ( 'NONE', ( #31286 ), #55272, .T. ) ;
#24143=CARTESIAN_POINT ( 'NONE',  ( -9.010802615327971665, 14.76984942314624227, 11.91753657575775271 ) ) ;
#24145=CARTESIAN_POINT ( 'NONE',  ( 9.846743663894594434, -11.49106884899921077, -2.168404344971008868E-15 ) ) ;
#24155=DIRECTION ( 'NONE',  ( 0.000000000000000000, 0.000000000000000000, 1.000000000000000000 ) ) ;
#24157=CARTESIAN_POINT ( 'NONE',  ( 2.120353041430647068, 15.00000000000000000, -14.34413130794945523 ) ) ;
#24158=B_SPLINE_CURVE_WITH_KNOTS ( 'NONE', 3,
 ( #4530, #95519, #26519, #78546, #56535, #64505 ),
 .UNSPECIFIED., .F., .F.,
 ( 4, 2, 4 ),
 ( 3.409110551496113072E-05, 0.0004400426677367864632, 0.0008459942299586118092 ),
 .UNSPECIFIED. ) ;
#24161=ORIENTED_EDGE ( 'NONE', *, *, #35008, .F. ) ;
#24175=DIRECTION ( 'NONE',  ( -0.000000000000000000, 1.000000000000000000, 0.000000000000000000 ) ) ;
#24179=ORIENTED_EDGE ( 'NONE', *, *, #97004, .T. ) ;
#24182=EDGE_CURVE ( 'NONE', #51377, #57773, #70294, .T. ) ;
#24183=DIRECTION ( 'NONE',  ( -0.9483236552061978797, 0.000000000000000000, -0.3173046564050965856 ) ) ;
#24187=EDGE_LOOP ( 'NONE', ( #84843, #35554, #25198, #17264 ) ) ;
#24188=CYLINDRICAL_SURFACE ( 'NONE', #4547, 15.00000000000000000 ) ;
#24200=ADVANCED_FACE ( 'NONE', ( #32761 ), #48748, .F. ) ;
#24208=CARTESIAN_POINT ( 'NONE',  ( 13.75801628063879711, 15.00000000000000000, -4.578972376164444746 ) ) ;
#24211=DIRECTION ( 'NONE',  ( 0.3502073812594748148, 0.000000000000000000, -0.9366721892483949041 ) ) ;
#24216=CARTESIAN_POINT ( 'NONE',  ( -5.440088680355547268, -36.10298132251183034, 9.422509992056143702 ) ) ;
#24232=CARTESIAN_POINT ( 'NONE',  ( 6.689969769698871360, -0.03417435944610275333, 12.58200319823975022 ) ) ;
#24238=ORIENTED_EDGE ( 'NONE', *, *, #31687, .T. ) ;
#24263=CARTESIAN_POINT ( 'NONE',  ( 14.09356342482593583, 14.95077488074853456, 4.360913911515476471 ) ) ;
#24266=CARTESIAN_POINT ( 'NONE',  ( -4.431036607602396593, 0.3639312379444145651, -14.33059365769920213 ) ) ;
#24272=CARTESIAN_POINT ( 'NONE',  ( 0.7117905103455572924, 0.000000000000000000, -5.406585696355421966 ) ) ;
#24274=EDGE_LOOP ( 'NONE', ( #25186, #62887, #13200, #17002 ) ) ;
#24280=DIRECTION ( 'NONE',  ( -0.000000000000000000, -1.000000000000000000, -0.000000000000000000 ) ) ;
#24286=ORIENTED_EDGE ( 'NONE', *, *, #90296, .F. ) ;
#24291=FACE_OUTER_BOUND ( 'NONE', #68423, .T. ) ;
#24299=ORIENTED_EDGE ( 'NONE', *, *, #80819, .T. ) ;
#24303=CARTESIAN_POINT ( 'NONE',  ( -14.88585913059898225, 14.76984981697404464, 1.278057234793719354 ) ) ;
#24306=EDGE_CURVE ( 'NONE', #18620, #3959, #25629, .T. ) ;
#24315=CARTESIAN_POINT ( 'NONE',  ( 1.114591949024928752, 4.429576435485488210E-16, 14.45709807627965304 ) ) ;
#24325=CARTESIAN_POINT ( 'NONE',  ( 11.48952521350825151, 15.00000000000000000, -8.845383562535966249 ) ) ;
#24327=AXIS2_PLACEMENT_3D ( 'NONE', #29315, #75315, #53807 ) ;
#24333=AXIS2_PLACEMENT_3D ( 'NONE', #49201, #79705, #11203 ) ;
#24340=CARTESIAN_POINT ( 'NONE',  ( -4.792102989642738287, 15.00000000000000000, -15.26149223938179134 ) ) ;
#24341=CARTESIAN_POINT ( 'NONE',  ( 0.000000000000000000, 14.49999999999999822, 0.000000000000000000 ) ) ;
#24347=ORIENTED_EDGE ( 'NONE', *, *, #9817, .F. ) ;
#24350=CARTESIAN_POINT ( 'NONE',  ( 14.94699059465107105, 14.49999999999999112, 1.259949270174897329 ) ) ;
#24352=B_SPLINE_CURVE_WITH_KNOTS ( 'NONE', 3,
 ( #79724, #32735, #11223, #39769, #70268, #63235 ),
 .UNSPECIFIED., .F., .F.,
 ( 4, 2, 4 ),
 ( 3.409110551495850831E-05, 0.0004400426677367822890, 0.0008459942299586060629 ),
 .UNSPECIFIED. ) ;
#24365=CARTESIAN_POINT ( 'NONE',  ( -12.60874940350953111, 3.965829894984375834E-16, 7.160268045226943379 ) ) ;
#24389=ORIENTED_EDGE ( 'NONE', *, *, #21816, .F. ) ;
#24390=EDGE_CURVE ( 'NONE', #35712, #28751, #89819, .T. ) ;
#24407=ORIENTED_EDGE ( 'NONE', *, *, #10097, .T. ) ;
#24414=LINE ( 'NONE', #8411, #57441 ) ;
#24417=EDGE_CURVE ( 'NONE', #89545, #24788, #72719, .T. ) ;
#24419=DIRECTION ( 'NONE',  ( 0.000000000000000000, 1.000000000000000000, 0.000000000000000000 ) ) ;
#24420=ORIENTED_EDGE ( 'NONE', *, *, #96003, .T. ) ;
#24423=EDGE_CURVE ( 'NONE', #91116, #89674, #71636, .T. ) ;
#24446=ADVANCED_FACE ( 'NONE', ( #72236 ), #64720, .T. ) ;
#24457=DIRECTION ( 'NONE',  ( 0.000000000000000000, 1.000000000000000000, 0.000000000000000000 ) ) ;
#24460=CARTESIAN_POINT ( 'NONE',  ( -14.16423886937410082, -3.196251165086032131, 4.336808689942017736E-15 ) ) ;
#24466=LINE ( 'NONE', #79427, #62989 ) ;
#24467=CARTESIAN_POINT ( 'NONE',  ( -7.313705784284733724, 14.49999999999999112, 13.09617149020743199 ) ) ;
#24468=CARTESIAN_POINT ( 'NONE',  ( 0.8060400322139245066, 0.000000000000000000, -5.393339789881740565 ) ) ;
#24478=DIRECTION ( 'NONE',  ( 0.000000000000000000, 0.000000000000000000, 1.000000000000000000 ) ) ;
#24487=ORIENTED_EDGE ( 'NONE', *, *, #95058, .T. ) ;
#24496=CARTESIAN_POINT ( 'NONE',  ( 13.34343830728404079, 0.5000000000000004441, -6.852200678592596184 ) ) ;
#24500=CARTESIAN_POINT ( 'NONE',  ( 3.836325488036083087, 0.3640475087720985159, 14.50112432709425470 ) ) ;
#24511=EDGE_CURVE ( 'NONE', #31058, #45767, #19243, .T. ) ;
#24516=DIRECTION ( 'NONE',  ( -0.000000000000000000, -1.000000000000000000, -0.000000000000000000 ) ) ;
#24517=ORIENTED_EDGE ( 'NONE', *, *, #42116, .F. ) ;
#24518=ORIENTED_EDGE ( 'NONE', *, *, #35087, .T. ) ;
#24519=TOROIDAL_SURFACE ( 'NONE', #42066, 14.49999999999999822, 0.5000000000000000000 ) ;
#24524=CARTESIAN_POINT ( 'NONE',  ( -13.21382278599144300, 3.049318610115481221E-16, 6.271621331965429924 ) ) ;
#24534=CARTESIAN_POINT ( 'NONE',  ( -3.469446951953614189E-15, 24.75893115100079456, -9.846743663894594434 ) ) ;
#24535=VERTEX_POINT ( 'NONE', #58715 ) ;
#24544=ADVANCED_FACE ( 'NONE', ( #20229 ), #50733, .F. ) ;
#24545=VECTOR ( 'NONE', #77821, 1000.000000000000000 ) ;
#24547=ORIENTED_EDGE ( 'NONE', *, *, #31638, .T. ) ;
#24559=DIRECTION ( 'NONE',  ( -0.5519369853120501546, 0.000000000000000000, -0.8338858220671735433 ) ) ;
#24566=CYLINDRICAL_SURFACE ( 'NONE', #31436, 15.00000000000000000 ) ;
#24573=DIRECTION ( 'NONE',  ( -0.000000000000000000, 1.000000000000000000, 0.000000000000000000 ) ) ;
#24583=CARTESIAN_POINT ( 'NONE',  ( -9.898881779040587858, 15.00000000000000000, -10.25059215482589714 ) ) ;
#24596=CARTESIAN_POINT ( 'NONE',  ( -9.422509992056145478, -2.352981322511826789, -5.440088680355541939 ) ) ;
#24601=CARTESIAN_POINT ( 'NONE',  ( -13.21272562211566104, -3.175103002782743638E-15, -6.271554226548334832 ) ) ;
#24602=CARTESIAN_POINT ( 'NONE',  ( -12.34086200392831678, -0.03417435944610275333, 7.124999999999885425 ) ) ;
#24625=FACE_OUTER_BOUND ( 'NONE', #75895, .T. ) ;
#24637=CARTESIAN_POINT ( 'NONE',  ( -9.065164099344672266, 14.49999999999999112, 11.95084933600764820 ) ) ;
#24639=CARTESIAN_POINT ( 'NONE',  ( -3.469446951953614189E-15, -10.24106884899921077, -9.846743663894594434 ) ) ;
#24640=ORIENTED_EDGE ( 'NONE', *, *, #77270, .F. ) ;
#24643=VERTEX_POINT ( 'NONE', #6218 ) ;
#24651=ADVANCED_FACE ( 'NONE', ( #22711 ), #37709, .T. ) ;
#24656=EDGE_CURVE ( 'NONE', #92022, #54254, #73906, .T. ) ;
#24667=ORIENTED_EDGE ( 'NONE', *, *, #51950, .F. ) ;
#24671=ORIENTED_EDGE ( 'NONE', *, *, #5865, .F. ) ;
#24675=LINE ( 'NONE', #9168, #42727 ) ;
#24676=VERTEX_POINT ( 'NONE', #83201 ) ;
#24683=ORIENTED_EDGE ( 'NONE', *, *, #29211, .F. ) ;
#24689=ADVANCED_FACE ( 'NONE', ( #51723 ), #46784, .T. ) ;
#24691=ORIENTED_EDGE ( 'NONE', *, *, #64564, .T. ) ;
#24693=DIRECTION ( 'NONE',  ( 0.000000000000000000, 0.000000000000000000, 1.000000000000000000 ) ) ;
#24700=DIRECTION ( 'NONE',  ( 0.000000000000000000, 0.000000000000000000, 1.000000000000000000 ) ) ;
#24702=FACE_OUTER_BOUND ( 'NONE', #18733, .T. ) ;
#24705=CARTESIAN_POINT ( 'NONE',  ( 3.469446951953614189E-15, 28.05374883491396076, 14.16423886937410259 ) ) ;
#24709=AXIS2_PLACEMENT_3D ( 'NONE', #55632, #8168, #2165 ) ;
#24726=ORIENTED_EDGE ( 'NONE', *, *, #71380, .T. ) ;
#24732=CARTESIAN_POINT ( 'NONE',  ( -7.618303901328417282, 15.00000000000000711, -12.48478900416272275 ) ) ;
#24739=CARTESIAN_POINT ( 'NONE',  ( -14.47650479471817242, 15.00000000000000000, -3.928206833722204028 ) ) ;
#24745=CARTESIAN_POINT ( 'NONE',  ( -0.7375392941519102186, 14.49999999999999112, 14.98185688723476616 ) ) ;
#24748=PLANE ( 'NONE',  #34234 ) ;
#24758=ORIENTED_EDGE ( 'NONE', *, *, #67641, .F. ) ;
#24761=VERTEX_POINT ( 'NONE', #98733 ) ;
#24767=DIRECTION ( 'NONE',  ( 0.000000000000000000, 0.000000000000000000, 1.000000000000000000 ) ) ;
#24770=CYLINDRICAL_SURFACE ( 'NONE', #544, 15.00000000000000000 ) ;
#24772=EDGE_CURVE ( 'NONE', #6306, #20656, #36217, .T. ) ;
#24773=CARTESIAN_POINT ( 'NONE',  ( 9.382169495545419124, 0.9986346699304144980, 9.382169495545417348 ) ) ;
#24782=CARTESIAN_POINT ( 'NONE',  ( 14.64921366071500053, 0.04962891916449693047, -1.748670679918162163 ) ) ;
#24788=VERTEX_POINT ( 'NONE', #13715 ) ;
#24810=EDGE_CURVE ( 'NONE', #59012, #26974, #67213, .T. ) ;
#24815=VERTEX_POINT ( 'NONE', #76192 ) ;
#24820=DIRECTION ( 'NONE',  ( 0.000000000000000000, 1.000000000000000000, -0.000000000000000000 ) ) ;
#24832=VECTOR ( 'NONE', #71204, 1000.000000000000000 ) ;
#24845=LINE ( 'NONE', #18813, #60389 ) ;
#24855=CARTESIAN_POINT ( 'NONE',  ( -1.983216688680738082, 15.00000000000000000, -14.11131997956740491 ) ) ;
#24881=ORIENTED_EDGE ( 'NONE', *, *, #7250, .F. ) ;
#24883=LINE ( 'NONE', #55368, #68063 ) ;
#24884=AXIS2_PLACEMENT_3D ( 'NONE', #41108, #18590, #79586 ) ;
#24889=B_SPLINE_CURVE_WITH_KNOTS ( 'NONE', 3,
 ( #27605, #13099, #36093, #67093, #20107, #66599, #43595, #82087, #35605, #50610, #52092, #74587, #82586, #67597, #483, #81588, #36606, #30931, #21606, #81102 ),
 .UNSPECIFIED., .F., .F.,
 ( 4, 2, 2, 2, 2, 2, 2, 2, 2, 4 ),
 ( 0.000000000000000000, 0.003408369840167499009, 0.004260462300209373436, 0.005112554760251249164, 0.006816739680334997151, 0.008520924600418745137, 0.01022510952050249486, 0.01107720198054436972, 0.01192929444058624285, 0.01363347936066999083 ),
 .UNSPECIFIED. ) ;
#24891=DIRECTION ( 'NONE',  ( 0.000000000000000000, 0.000000000000000000, 1.000000000000000000 ) ) ;
#24908=CIRCLE ( 'NONE', #71147, 14.49999999999999822 ) ;
#24915=VERTEX_POINT ( 'NONE', #60196 ) ;
#24921=FACE_OUTER_BOUND ( 'NONE', #26449, .T. ) ;
#24946=ORIENTED_EDGE ( 'NONE', *, *, #23888, .T. ) ;
#24950=FACE_OUTER_BOUND ( 'NONE', #31019, .T. ) ;
#24953=CARTESIAN_POINT ( 'NONE',  ( 14.16423886937410437, -5.904584498419365168, 3.795296366450304770 ) ) ;
#24955=DIRECTION ( 'NONE',  ( 0.9366721892483971246, 0.000000000000000000, 0.3502073812594687086 ) ) ;
#24957=AXIS2_PLACEMENT_3D ( 'NONE', #90656, #14690, #30637 ) ;
#24970=CARTESIAN_POINT ( 'NONE',  ( 14.47650479471820262, 0.3640475087720640990, 3.928206833722112989 ) ) ;
#24972=DIRECTION ( 'NONE',  ( -0.000000000000000000, -1.000000000000000000, -0.000000000000000000 ) ) ;
#24995=ORIENTED_EDGE ( 'NONE', *, *, #93455, .F. ) ;
#25005=CIRCLE ( 'NONE', #48954, 14.49999999999999822 ) ;
#25013=FACE_OUTER_BOUND ( 'NONE', #1515, .T. ) ;
#25024=CARTESIAN_POINT ( 'NONE',  ( 9.846743663894590881, 23.71726448433412671, -2.638427012816833894 ) ) ;
#25025=ORIENTED_EDGE ( 'NONE', *, *, #83219, .T. ) ;
#25043=( BOUNDED_CURVE ( )  B_SPLINE_CURVE ( 2, ( #12540, #96553, #28028, #43041, #97054, #14035, #29007, #36535, #66026, #89032, #82018, #44012, #75012 ),
 .UNSPECIFIED., .F., .T. ) 
 B_SPLINE_CURVE_WITH_KNOTS ( ( 3, 2, 2, 2, 2, 2, 3 ),
 ( 0.6333333333333334147, 0.6388888888888889506, 0.6444444444444445974, 0.6500000000000001332, 0.6555555555555556690, 0.6611111111111112049, 0.6666666666666667407 ),
 .UNSPECIFIED. ) 
 CURVE ( )  GEOMETRIC_REPRESENTATION_ITEM ( )  RATIONAL_B_SPLINE_CURVE ( ( 0.9999999999999993339, 0.9659258262890688673, 1.000000000000000000, 0.9659258262890682012, 1.000000000000000000, 0.9659258262890682012, 1.000000000000000000, 0.9659258262890682012, 1.000000000000000000, 0.9659258262890682012, 1.000000000000000000, 0.9659258262890675351, 1.000000000000000666 ) ) 
 REPRESENTATION_ITEM ( '' )  );
#25046=CARTESIAN_POINT ( 'NONE',  ( -4.431036607602665711, 0.3640475087720917435, 14.33059365769909377 ) ) ;
#25053=AXIS2_PLACEMENT_3D ( 'NONE', #94382, #41419, #86406 ) ;
#25054=CARTESIAN_POINT ( 'NONE',  ( -2.962741594153171842, -0.03417435944610275333, 13.93860331045670975 ) ) ;
#25062=CARTESIAN_POINT ( 'NONE',  ( 11.81378540890936080, 0.000000000000000000, -7.968498874458115999 ) ) ;
#25066=ORIENTED_EDGE ( 'NONE', *, *, #43468, .F. ) ;
#25068=CLOSED_SHELL ( 'NONE', ( #71821, #44002, #44199, #13454, #87358, #62476, #63363, #37181, #30849, #32161, #95451, #32404, #30912, #54514, #16187, #56006, #24446, #59833, #24129, #19860, #57112, #81298, #87175, #31400, #21479, #51599, #6555, #12089, #14348, #12440, #67016, #71449, #21820, #46855, #81837, #22973, #98926, #81005, #11312, #50103, #63857, #21236, #10413, #66732, #65900, #83333, #45072, #47461, #38892, #3516, #57554, #18394, #70036, #18426, #83188, #81719, #19188, #58623, #73020, #32741, #5454, #82177, #10021, #26756, #80402, #69771, #63722, #21333, #62080, #56133, #18872, #95034, #98285, #9769, #68774, #82192, #46934, #39414, #27026, #34203, #55892, #13283, #65593, #89479, #29123, #28652, #12648, #28611, #89635, #53915, #98911, #24651, #32508, #78700, #54574, #87387, #5731, #85268, #85033, #79632, #58306, #35795, #66053, #82308, #83992, #46388, #39488, #77522, #85821, #53419, #61245, #32283, #23744, #5089, #40668, #88789, #1847, #41361, #35817, #26009, #41668, #63044, #80248, #93784, #96508, #79584, #16908, #72694, #57789, #80731, #25380, #59147, #97385, #53662, #12798, #15059, #96180, #79495, #44635, #30364, #24689, #67991, #67186, #47932, #9503, #97344, #54771, #79464, #7083, #38064, #85146, #3799, #64130, #62395, #46170, #75889, #27225, #31317, #76349, #7464, #43580, #37610, #40448, #41439, #32070, #53192, #64944, #48098, #2296, #8454, #19203, #72579, #49944, #93265, #76044, #44922, #25261, #41471, #51823, #46411, #56873, #82239, #82174, #82784, #75106, #93495, #36623, #8137, #172, #50824, #74434, #84356, #81877, #8924, #56694, #17649, #34563, #64105, #48649, #72582, #33724, #38141, #71611, #91686, #62806, #50236, #74140, #68998, #69282, #38382, #37750, #71797, #56399, #16436, #34440, #56602, #53086, #50708, #25193, #11795, #65225, #64661, #81319, #26105, #91479, #88616, #960, #31038, #49130, #86609, #6974, #87232, #41614, #48218, #14875, #72698, #74628, #46744, #84880, #44936, #44182, #94436, #83595, #88832, #74747, #61525, #39540, #28477, #20571, #97958, #83997, #14958, #38537, #59594, #51858, #11975, #10942, #92040, #60169, #68315, #17375, #5797, #25533, #38529, #31952, #62890, #7343, #38499, #42805, #27438, #96289, #62770, #54870, #47412, #26201, #53541, #91268, #88868, #87499, #8873, #73, #85759, #55096, #10857, #15727, #36593, #14723, #44691, #83433, #59522, #594, #92168, #42244, #25333, #95153, #40088, #20268, #67214, #23271, #65235, #9166, #31922, #46023, #90218, #52307, #11886, #65805, #50705, #65825, #18192, #27755, #6387, #76668, #12635, #72843, #33635, #2741, #48122, #51043, #47291, #76537, #75882, #65143, #5713, #78133, #74178, #19221, #23976, #86027, #3404, #87915, #63993, #62658, #52384, #62005, #49667, #94512, #89785, #47237, #63558, #76880, #34892, #50283, #26968, #34652, #41360, #25805, #22481, #61636, #61996, #75396, #39321, #45291, #52946, #29469, #87650, #3930, #63357, #39207, #33489, #91235, #84666, #94729, #22845, #1178, #78012, #22131, #30281, #10744, #57347, #24200, #43007, #5154, #98008, #35370, #20964, #43376, #20221, #33290, #86545, #25625, #12130, #2947, #64711, #12295, #59142, #55962, #49166, #44575, #17556, #93143, #63999, #51802, #14832, #61527, #7816, #72550, #81600, #85259, #29917, #87026, #85510, #15519, #12698, #11359, #73303, #45524, #80887, #68718, #19973, #15369, #69438, #89218, #78923, #80706, #23148, #71155, #84806, #45746, #20383, #76103, #2870, #36479, #24544, #76650, #37945, #80198, #22356, #43356, #73135, #12924, #23862, #33993, #66721, #3407, #70015, #20002, #70240, #90705, #76662, #46132, #75757, #27447, #9697, #34668, #47051, #62061, #62635, #43591, #79395, #96666, #84282, #77555, #36738, #63331, #50410, #71077, #8404, #6209, #68104, #5242, #47447, #65453, #50827, #41501, #41468, #72254, #59949, #85028, #62183 ) ) ;
#25080=VERTEX_POINT ( 'NONE', #10029 ) ;
#25087=DIRECTION ( 'NONE',  ( -0.000000000000000000, -1.000000000000000000, -0.000000000000000000 ) ) ;
#25093=CARTESIAN_POINT ( 'NONE',  ( 2.915334737309921209, 1.605352010821511133, -10.88017736071110164 ) ) ;
#25104=DIRECTION ( 'NONE',  ( 0.000000000000000000, 0.000000000000000000, -1.000000000000000000 ) ) ;
#25105=VECTOR ( 'NONE', #60575, 1000.000000000000000 ) ;
#25113=ORIENTED_EDGE ( 'NONE', *, *, #79929, .F. ) ;
#25121=VECTOR ( 'NONE', #32728, 1000.000000000000227 ) ;
#25124=CARTESIAN_POINT ( 'NONE',  ( 0.000000000000000000, 0.000000000000000000, 0.000000000000000000 ) ) ;
#25131=VERTEX_POINT ( 'NONE', #40530 ) ;
#25146=CARTESIAN_POINT ( 'NONE',  ( 4.923371831947301658, -7.324402182332545586, 8.527530157486175710 ) ) ;
#25150=EDGE_LOOP ( 'NONE', ( #95111, #1013, #4103, #19703 ) ) ;
#25156=CARTESIAN_POINT ( 'NONE',  ( -12.60874940350935169, 15.00000000000000000, -7.160268045227203615 ) ) ;
#25157=B_SPLINE_CURVE_WITH_KNOTS ( 'NONE', 3,
 ( #71877, #48875, #79385, #33855, #65347, #78394 ),
 .UNSPECIFIED., .F., .F.,
 ( 4, 2, 4 ),
 ( 3.409110551494648722E-05, 0.0004400426677367935105, 0.0008459942299586405406 ),
 .UNSPECIFIED. ) ;
#25160=ORIENTED_EDGE ( 'NONE', *, *, #32527, .F. ) ;
#25171=VECTOR ( 'NONE', #26635, 1000.000000000000000 ) ;
#25172=CARTESIAN_POINT ( 'NONE',  ( 0.2078280073304309694, 0.04958531807300550764, -14.75174119393810557 ) ) ;
#25177=DIRECTION ( 'NONE',  ( 0.008726535498381206638, 0.000000000000000000, -0.9999619230641713097 ) ) ;
#25186=ORIENTED_EDGE ( 'NONE', *, *, #20646, .F. ) ;
#25193=ADVANCED_FACE ( 'NONE', ( #33008 ), #38887, .T. ) ;
#25196=VECTOR ( 'NONE', #86843, 1000.000000000000000 ) ;
#25198=ORIENTED_EDGE ( 'NONE', *, *, #16836, .F. ) ;
#25205=CARTESIAN_POINT ( 'NONE',  ( 13.55255535720591986, 15.00000000000000000, 4.403492169843056914 ) ) ;
#25206=DIRECTION ( 'NONE',  ( 0.8038568606172245001, 0.000000000000000000, -0.5948227867513318223 ) ) ;
#25210=CARTESIAN_POINT ( 'NONE',  ( 10.88017736071110519, -34.43631465584515894, -2.602085213965210642E-15 ) ) ;
#25213=DIRECTION ( 'NONE',  ( 0.9483236552061956592, 0.000000000000000000, 0.3173046564051031915 ) ) ;
#25220=EDGE_LOOP ( 'NONE', ( #63963, #16012, #70181, #22220 ) ) ;
#25222=EDGE_CURVE ( 'NONE', #79627, #46342, #33484, .T. ) ;
#25226=CARTESIAN_POINT ( 'NONE',  ( -2.258648100792082225, 14.95077488074853456, -14.57890972981275723 ) ) ;
#25240=DIRECTION ( 'NONE',  ( 0.000000000000000000, 1.000000000000000000, 0.000000000000000000 ) ) ;
#25244=ORIENTED_EDGE ( 'NONE', *, *, #91444, .T. ) ;
#25245=VERTEX_POINT ( 'NONE', #55015 ) ;
#25246=DIRECTION ( 'NONE',  ( -0.000000000000000000, -1.000000000000000000, -0.000000000000000000 ) ) ;
#25254=CARTESIAN_POINT ( 'NONE',  ( 14.17193700899790265, 15.00000000000000000, -1.489530601564018175 ) ) ;
#25257=CARTESIAN_POINT ( 'NONE',  ( 13.34343830728408697, 14.49999999999999112, -6.852200678592647698 ) ) ;
#25261=ADVANCED_FACE ( 'NONE', ( #78026 ), #8546, .T. ) ;
#25263=EDGE_CURVE ( 'NONE', #52889, #64121, #78515, .T. ) ;
#25264=ORIENTED_EDGE ( 'NONE', *, *, #6237, .F. ) ;
#25272=EDGE_CURVE ( 'NONE', #74162, #45188, #90722, .T. ) ;
#25275=VERTEX_POINT ( 'NONE', #11489 ) ;
#25276=AXIS2_PLACEMENT_3D ( 'NONE', #12684, #5200, #18727 ) ;
#25278=CARTESIAN_POINT ( 'NONE',  ( -11.09922568453594316, -10.45969866340290544, 6.408140936763246920 ) ) ;
#25279=VERTEX_POINT ( 'NONE', #87489 ) ;
#25285=LINE ( 'NONE', #62756, #67148 ) ;
#25288=DIRECTION ( 'NONE',  ( 0.000000000000000000, 1.000000000000000000, 0.000000000000000000 ) ) ;
#25290=CARTESIAN_POINT ( 'NONE',  ( 2.120353041430538266, 15.00000000000000000, 14.34413130794944635 ) ) ;
#25292=DIRECTION ( 'NONE',  ( -0.6755902076156641289, 0.000000000000000000, 0.7372773368101205316 ) ) ;
#25294=CARTESIAN_POINT ( 'NONE',  ( 14.94699059465100888, 15.00000000000000000, 1.259949270174915981 ) ) ;
#25299=CARTESIAN_POINT ( 'NONE',  ( 7.618485323809187193, 2.541098841762901017E-16, 12.48587314215767741 ) ) ;
#25308=VECTOR ( 'NONE', #34442, 1000.000000000000000 ) ;
#25310=SHAPE_REPRESENTATION_RELATIONSHIP ( 'NONE' , 'NONE' ,  #81163, #72777 ) ;
#25325=CARTESIAN_POINT ( 'NONE',  ( -9.876730923139204421, 14.49999999999999112, -11.28938378619079863 ) ) ;
#25331=CARTESIAN_POINT ( 'NONE',  ( 0.000000000000000000, 14.49999999999999822, 0.000000000000000000 ) ) ;
#25332=ORIENTED_EDGE ( 'NONE', *, *, #934, .F. ) ;
#25333=ADVANCED_FACE ( 'NONE', ( #86394 ), #40410, .F. ) ;
#25339=CARTESIAN_POINT ( 'NONE',  ( 3.270119481323575439, 14.95077488074853456, 14.38584091150422850 ) ) ;
#25344=EDGE_CURVE ( 'NONE', #72583, #45054, #15716, .T. ) ;
#25347=LINE ( 'NONE', #47323, #49249 ) ;
#25366=B_SPLINE_CURVE_WITH_KNOTS ( 'NONE', 3,
 ( #29191, #61172, #91678, #75186, #60185, #23197 ),
 .UNSPECIFIED., .F., .F.,
 ( 4, 2, 4 ),
 ( 3.409110551496220137E-05, 0.0004400426677368005578, 0.0008459942299586389143 ),
 .UNSPECIFIED. ) ;
#25376=ORIENTED_EDGE ( 'NONE', *, *, #70131, .T. ) ;
#25378=ORIENTED_EDGE ( 'NONE', *, *, #38637, .T. ) ;
#25380=ADVANCED_FACE ( 'NONE', ( #92893 ), #91550, .T. ) ;
#25382=ORIENTED_EDGE ( 'NONE', *, *, #95950, .F. ) ;
#25386=CARTESIAN_POINT ( 'NONE',  ( 4.873787042390699931, 15.00000000000000000, 13.39061984619922718 ) ) ;
#25394=ORIENTED_EDGE ( 'NONE', *, *, #79255, .F. ) ;
#25395=CARTESIAN_POINT ( 'NONE',  ( -10.64017930668194367, 0.3639309529147286004, -10.57291749337231757 ) ) ;
#25403=VECTOR ( 'NONE', #90401, 1000.000000000000000 ) ;
#25405=FACE_OUTER_BOUND ( 'NONE', #93237, .T. ) ;
#25406=ORIENTED_EDGE ( 'NONE', *, *, #12093, .T. ) ;
#25409=EDGE_CURVE ( 'NONE', #56402, #88170, #53210, .T. ) ;
#25411=ORIENTED_EDGE ( 'NONE', *, *, #33098, .T. ) ;
#25412=CARTESIAN_POINT ( 'NONE',  ( 3.420591144908446957, 0.5000000000000004441, 14.60477854057958425 ) ) ;
#25418=CARTESIAN_POINT ( 'NONE',  ( -1.796787675079396296, 0.2301501525784628854, 14.83218748772990025 ) ) ;
#25419=CARTESIAN_POINT ( 'NONE',  ( 0.000000000000000000, 0.000000000000000000, 0.000000000000000000 ) ) ;
#25420=CARTESIAN_POINT ( 'NONE',  ( -14.24131928502210975, -0.03417435944610275333, -0.4973178280107823923 ) ) ;
#25421=AXIS2_PLACEMENT_3D ( 'NONE', #56375, #56851, #78869 ) ;
#25425=EDGE_CURVE ( 'NONE', #46976, #2401, #87366, .T. ) ;
#25432=EDGE_CURVE ( 'NONE', #3732, #39776, #48427, .T. ) ;
#25445=VERTEX_POINT ( 'NONE', #16678 ) ;
#25448=DIRECTION ( 'NONE',  ( -0.000000000000000000, -1.000000000000000000, -0.000000000000000000 ) ) ;
#25450=CARTESIAN_POINT ( 'NONE',  ( -8.564643372776702179, 15.00000000000000000, 12.31449893000734797 ) ) ;
#25451=CARTESIAN_POINT ( 'NONE',  ( 7.082119434687047743, 5.137082168247313341, -12.26659068614894821 ) ) ;
#25459=CARTESIAN_POINT ( 'NONE',  ( -10.93781366033335622, 14.49999999999999112, -10.26470809774086490 ) ) ;
#25465=CARTESIAN_POINT ( 'NONE',  ( 0.000000000000000000, 0.5000000000000004441, 0.000000000000000000 ) ) ;
#25468=CARTESIAN_POINT ( 'NONE',  ( 14.15369600240090797, 1.135024149320762060E-15, 3.689340892730358146 ) ) ;
#25470=LINE ( 'NONE', #16972, #36815 ) ;
#25486=CARTESIAN_POINT ( 'NONE',  ( 5.803070148808322948, 15.00000000000000000, -13.28812917035385510 ) ) ;
#25488=VERTEX_POINT ( 'NONE', #31661 ) ;
#25499=CARTESIAN_POINT ( 'NONE',  ( 0.000000000000000000, 0.000000000000000000, 0.000000000000000000 ) ) ;
#25500=ORIENTED_EDGE ( 'NONE', *, *, #70529, .F. ) ;
#25505=CARTESIAN_POINT ( 'NONE',  ( 13.74385066382880183, 0.2306972965111846186, 5.860428621090457035 ) ) ;
#25506=DIRECTION ( 'NONE',  ( -0.000000000000000000, -1.000000000000000000, -0.000000000000000000 ) ) ;
#25513=CARTESIAN_POINT ( 'NONE',  ( -8.564643372776448160, 0.5000000000000004441, -12.31449893000752205 ) ) ;
#25515=CARTESIAN_POINT ( 'NONE',  ( -12.81628187352647608, -25.87636533006957507, 3.903127820947815962E-15 ) ) ;
#25526=VERTEX_POINT ( 'NONE', #45691 ) ;
#25531=DIRECTION ( 'NONE',  ( -0.7716245833877234395, 0.000000000000000000, 0.6360782202777597316 ) ) ;
#25533=ADVANCED_FACE ( 'NONE', ( #98224 ), #10121, .T. ) ;
#25542=DIRECTION ( 'NONE',  ( -0.1822355254921381451, 0.000000000000000000, -0.9832549075639562819 ) ) ;
#25544=ORIENTED_EDGE ( 'NONE', *, *, #75537, .F. ) ;
#25545=CARTESIAN_POINT ( 'NONE',  ( 12.34086200392821908, 15.00000000000000000, 7.125000000000058620 ) ) ;
#25555=VERTEX_POINT ( 'NONE', #91183 ) ;
#25561=CARTESIAN_POINT ( 'NONE',  ( -13.75801628063882909, 15.00000000000000000, 4.578972376164350599 ) ) ;
#25564=CARTESIAN_POINT ( 'NONE',  ( 0.1556627343491842341, 15.00000000000000711, 14.62580308442188404 ) ) ;
#25567=ORIENTED_EDGE ( 'NONE', *, *, #46090, .T. ) ;
#25575=EDGE_CURVE ( 'NONE', #69540, #97076, #88472, .T. ) ;
#25579=CARTESIAN_POINT ( 'NONE',  ( -9.422509992056145478, 7.647018677488174987, -5.440088680355541939 ) ) ;
#25580=CARTESIAN_POINT ( 'NONE',  ( 14.43100913236849614, 4.781026887021415124E-16, 1.412789942453260839 ) ) ;
#25584=CARTESIAN_POINT ( 'NONE',  ( -14.17193700899788134, -0.03417435944610275333, -1.489530601564206247 ) ) ;
#25588=CARTESIAN_POINT ( 'NONE',  ( 7.993487411949370625, 14.95037111676401587, -12.40005926694708549 ) ) ;
#25589=CARTESIAN_POINT ( 'NONE',  ( -13.82671409943291785, -0.03417435944610275333, -3.447387012295409114 ) ) ;
#25596=ORIENTED_EDGE ( 'NONE', *, *, #90075, .F. ) ;
#25609=LINE ( 'NONE', #87079, #18452 ) ;
#25611=ORIENTED_EDGE ( 'NONE', *, *, #91572, .T. ) ;
#25624=CARTESIAN_POINT ( 'NONE',  ( 8.527530157486175710, -6.074402182332544697, -4.923371831947298993 ) ) ;
#25625=ADVANCED_FACE ( 'NONE', ( #54164 ), #38690, .F. ) ;
#25629=( BOUNDED_CURVE ( )  B_SPLINE_CURVE ( 2, ( #92294, #46787, #23817, #54279, #84796, #16305, #62269 ),
 .UNSPECIFIED., .F., .F. ) 
 B_SPLINE_CURVE_WITH_KNOTS ( ( 3, 2, 2, 3 ),
 ( 0.6999999999999999556, 0.7055555555555556024, 0.7111111111111111382, 0.7150761194637891283 ),
 .UNSPECIFIED. ) 
 CURVE ( )  GEOMETRIC_REPRESENTATION_ITEM ( )  RATIONAL_B_SPLINE_CURVE ( ( 1.000000000000000000, 0.9659258262890684232, 1.000000000000000000, 0.9659258262890684232, 1.000000000000000000, 0.9756812109925998566, 0.9860751345400877721 ) ) 
 REPRESENTATION_ITEM ( '' )  );
#25631=VECTOR ( 'NONE', #46774, 1000.000000000000000 ) ;
#25632=ORIENTED_EDGE ( 'NONE', *, *, #84233, .F. ) ;
#25638=EDGE_CURVE ( 'NONE', #96742, #8774, #38205, .T. ) ;
#25639=CARTESIAN_POINT ( 'NONE',  ( 0.000000000000000000, 15.00000000000000000, 0.000000000000000000 ) ) ;
#25645=ORIENTED_EDGE ( 'NONE', *, *, #54907, .F. ) ;
#25651=CARTESIAN_POINT ( 'NONE',  ( 0.1034006766821536916, 0.000000000000000000, -14.49963131600461352 ) ) ;
#25663=ORIENTED_EDGE ( 'NONE', *, *, #47511, .F. ) ;
#25678=AXIS2_PLACEMENT_3D ( 'NONE', #58516, #20027, #66018 ) ;
#25679=EDGE_LOOP ( 'NONE', ( #35196, #75417, #35611, #1525 ) ) ;
#25684=CARTESIAN_POINT ( 'NONE',  ( 4.473274078425821365, 13.14893278465882887, -11.04690489162689104 ) ) ;
#25687=CARTESIAN_POINT ( 'NONE',  ( -5.419894505350392855, 14.49999999999999822, -13.98659156302466045 ) ) ;
#25692=CARTESIAN_POINT ( 'NONE',  ( -5.204170427930421283E-15, -33.18631465584515894, -10.88017736071110342 ) ) ;
#25694=CIRCLE ( 'NONE', #57576, 14.49999999999999822 ) ;
#25696=DIRECTION ( 'NONE',  ( -0.000000000000000000, 1.000000000000000000, 0.000000000000000000 ) ) ;
#25721=LINE ( 'NONE', #86709, #97487 ) ;
#25723=VECTOR ( 'NONE', #51376, 1000.000000000000114 ) ;
#25725=DIRECTION ( 'NONE',  ( -0.000000000000000000, -1.000000000000000000, -0.000000000000000000 ) ) ;
#25727=EDGE_LOOP ( 'NONE', ( #63394, #90124, #58062, #52173 ) ) ;
#25730=B_SPLINE_CURVE_WITH_KNOTS ( 'NONE', 3,
 ( #98890, #1366, #98395, #83853, #62314, #23859 ),
 .UNSPECIFIED., .F., .F.,
 ( 4, 2, 4 ),
 ( 3.409110551474236583E-05, 0.0004400426677365819827, 0.0008459942299584215317 ),
 .UNSPECIFIED. ) ;
#25742=( BOUNDED_CURVE ( )  B_SPLINE_CURVE ( 2, ( #38380, #91869, #59879, #6891, #37404, #30863, #83873, #61360, #51899, #45883, #7399, #7888, #90368 ),
 .UNSPECIFIED., .F., .F. ) 
 B_SPLINE_CURVE_WITH_KNOTS ( ( 3, 2, 2, 2, 2, 2, 3 ),
 ( 0.5388110034902238166, 0.5388888888888888618, 0.5444444444444443976, 0.5500000000000000444, 0.5555555555555556912, 0.5611111111111112271, 0.5666666666666667629 ),
 .UNSPECIFIED. ) 
 CURVE ( )  GEOMETRIC_REPRESENTATION_ITEM ( )  RATIONAL_B_SPLINE_CURVE ( ( 0.9990579970486470618, 0.9995223014913415804, 1.000000000000000000, 0.9659258262890682012, 1.000000000000000000, 0.9659258262890682012, 1.000000000000000000, 0.9659258262890682012, 1.000000000000000000, 0.9659258262890682012, 1.000000000000000000, 0.9659258262890675351, 1.000000000000000666 ) ) 
 REPRESENTATION_ITEM ( '' )  );
#25748=FACE_OUTER_BOUND ( 'NONE', #25890, .T. ) ;
#25749=ORIENTED_EDGE ( 'NONE', *, *, #31079, .T. ) ;
#25756=CIRCLE ( 'NONE', #94385, 14.49999999999999822 ) ;
#25759=CARTESIAN_POINT ( 'NONE',  ( -6.408140936763232709, -0.04303199673624108490, 11.09922568453595026 ) ) ;
#25771=EDGE_CURVE ( 'NONE', #18519, #34814, #33616, .T. ) ;
#25773=CARTESIAN_POINT ( 'NONE',  ( 2.361410439757232194, 14.76930270348881002, 14.75336556272938360 ) ) ;
#25776=EDGE_CURVE ( 'NONE', #70273, #93127, #92024, .T. ) ;
#25780=DIRECTION ( 'NONE',  ( -0.2503800040544323924, 0.000000000000000000, -0.9681476403781101858 ) ) ;
#25787=CARTESIAN_POINT ( 'NONE',  ( 4.841308736149603220, 14.76984994420195996, 14.13449535775536958 ) ) ;
#25793=ORIENTED_EDGE ( 'NONE', *, *, #11863, .F. ) ;
#25800=LINE ( 'NONE', #56301, #77066 ) ;
#25803=DIRECTION ( 'NONE',  ( 0.1650476058606741014, -0.000000000000000000, 0.9862856015372319929 ) ) ;
#25805=ADVANCED_FACE ( 'NONE', ( #34107 ), #10644, .F. ) ;
#25809=TOROIDAL_SURFACE ( 'NONE', #64104, 14.49999999999999822, 0.5000000000000000000 ) ;
#25812=ORIENTED_EDGE ( 'NONE', *, *, #2016, .T. ) ;
#25822=VERTEX_POINT ( 'NONE', #40159 ) ;
#25829=DIRECTION ( 'NONE',  ( 0.000000000000000000, 0.000000000000000000, -1.000000000000000000 ) ) ;
#25834=CARTESIAN_POINT ( 'NONE',  ( 1.114591949025028450, 15.00000000000000000, -14.45709807627964416 ) ) ;
#25835=CIRCLE ( 'NONE', #53010, 15.00000000000000000 ) ;
#25836=LINE ( 'NONE', #95298, #86263 ) ;
#25845=DIRECTION ( 'NONE',  ( 0.000000000000000000, 0.000000000000000000, 1.000000000000000000 ) ) ;
#25863=CARTESIAN_POINT ( 'NONE',  ( -11.35178980618980304, 0.5000000000000004441, 9.804941009311846756 ) ) ;
#25864=CIRCLE ( 'NONE', #33818, 15.00000000000000000 ) ;
#25874=ORIENTED_EDGE ( 'NONE', *, *, #15606, .F. ) ;
#25875=DIRECTION ( 'NONE',  ( -0.000000000000000000, -1.000000000000000000, -0.000000000000000000 ) ) ;
#25883=EDGE_CURVE ( 'NONE', #74605, #49327, #26616, .T. ) ;
#25890=EDGE_LOOP ( 'NONE', ( #32970, #59718, #37799, #34480, #8535, #23803 ) ) ;
#25891=AXIS2_PLACEMENT_3D ( 'NONE', #82540, #30514, #91529 ) ;
#25898=DIRECTION ( 'NONE',  ( 0.2503800040544389427, -0.000000000000000000, 0.9681476403781082984 ) ) ;
#25905=CARTESIAN_POINT ( 'NONE',  ( -14.02068044289386783, 14.63606918466436113, 5.331089937175564231 ) ) ;
#25908=ORIENTED_EDGE ( 'NONE', *, *, #12642, .T. ) ;
#25909=CARTESIAN_POINT ( 'NONE',  ( 8.564643372776616914, 14.49999999999999822, -12.31449893000740836 ) ) ;
#25924=CARTESIAN_POINT ( 'NONE',  ( -3.243710765982357636, 0.000000000000000000, 4.383623511354867830 ) ) ;
#25925=CARTESIAN_POINT ( 'NONE',  ( 7.082119434687054849, 8.470415501580639273, 12.26659068614894288 ) ) ;
#25929=ORIENTED_EDGE ( 'NONE', *, *, #63531, .T. ) ;
#25935=CARTESIAN_POINT ( 'NONE',  ( -3.195792623639597707, 8.646642702460848540, -11.92686044187652961 ) ) ;
#25937=CARTESIAN_POINT ( 'NONE',  ( 10.14667048435145169, 4.379817243679289018E-16, -10.35833375027041292 ) ) ;
#25939=CARTESIAN_POINT ( 'NONE',  ( 0.000000000000000000, 0.000000000000000000, 0.000000000000000000 ) ) ;
#25941=FACE_OUTER_BOUND ( 'NONE', #64131, .T. ) ;
#25951=VECTOR ( 'NONE', #6110, 999.9999999999998863 ) ;
#25957=CARTESIAN_POINT ( 'NONE',  ( -5.817157072110620497, 14.49999999999999112, -13.82608706751101302 ) ) ;
#25959=ORIENTED_EDGE ( 'NONE', *, *, #78614, .F. ) ;
#25969=ORIENTED_EDGE ( 'NONE', *, *, #20438, .F. ) ;
#25976=ORIENTED_EDGE ( 'NONE', *, *, #9159, .T. ) ;
#25993=CARTESIAN_POINT ( 'NONE',  ( 12.81628187352647608, -33.58469866340291077, 3.434112377981052511 ) ) ;
#25994=ORIENTED_EDGE ( 'NONE', *, *, #53507, .F. ) ;
#26002=B_SPLINE_CURVE_WITH_KNOTS ( 'NONE', 3,
 ( #10725, #26218, #9246, #86728, #24266, #17257 ),
 .UNSPECIFIED., .F., .F.,
 ( 4, 2, 4 ),
 ( 0.0002800630492131283558, 0.0006862688956284094047, 0.001092474742043690345 ),
 .UNSPECIFIED. ) ;
#26004=AXIS2_PLACEMENT_3D ( 'NONE', #53187, #37703, #83194 ) ;
#26006=ORIENTED_EDGE ( 'NONE', *, *, #40925, .F. ) ;
#26009=ADVANCED_FACE ( 'NONE', ( #93644 ), #97926, .T. ) ;
#26010=B_SPLINE_CURVE_WITH_KNOTS ( 'NONE', 3,
 ( #17919, #86418, #39445, #1456, #92915, #77917 ),
 .UNSPECIFIED., .F., .F.,
 ( 4, 2, 4 ),
 ( 0.0002800715030460633101, 0.0006862774322447769745, 0.001092483361443490585 ),
 .UNSPECIFIED. ) ;
#26011=EDGE_LOOP ( 'NONE', ( #63931, #72837 ) ) ;
#26018=CARTESIAN_POINT ( 'NONE',  ( -4.862001128006864903, 4.306586084822671512E-16, 13.66056166602457012 ) ) ;
#26023=CARTESIAN_POINT ( 'NONE',  ( -15.99538290524656503, 15.00000000000000000, -0.1584996864330918964 ) ) ;
#26034=CARTESIAN_POINT ( 'NONE',  ( 0.000000000000000000, 14.49999999999999822, 0.000000000000000000 ) ) ;
#26039=AXIS2_PLACEMENT_3D ( 'NONE', #90310, #23824, #75817 ) ;
#26045=EDGE_CURVE ( 'NONE', #67764, #5928, #30872, .T. ) ;
#26048=CARTESIAN_POINT ( 'NONE',  ( -10.36894250292378317, -37.57125116508602503, 10.36894250292379560 ) ) ;
#26051=VERTEX_POINT ( 'NONE', #18154 ) ;
#26057=DIRECTION ( 'NONE',  ( 0.9890158633619168249, 0.000000000000000000, 0.1478094111296113511 ) ) ;
#26062=CARTESIAN_POINT ( 'NONE',  ( -7.964842623401179544, 12.43868534415484639, -7.964842623401174215 ) ) ;
#26065=DIRECTION ( 'NONE',  ( -0.000000000000000000, -1.000000000000000000, -0.000000000000000000 ) ) ;
#26068=DIRECTION ( 'NONE',  ( 0.6087614290087297597, 0.000000000000000000, -0.7933533402912281707 ) ) ;
#26105=ADVANCED_FACE ( 'NONE', ( #32143 ), #85187, .T. ) ;
#26106=AXIS2_PLACEMENT_3D ( 'NONE', #80362, #91685, #23204 ) ;
#26109=CARTESIAN_POINT ( 'NONE',  ( -8.527530157486173934, 6.425597817667459744, 4.923371831947302546 ) ) ;
#26110=VERTEX_POINT ( 'NONE', #55144 ) ;
#26120=EDGE_CURVE ( 'NONE', #3454, #74236, #95567, .T. ) ;
#26122=DIRECTION ( 'NONE',  ( 0.000000000000000000, 0.000000000000000000, 1.000000000000000000 ) ) ;
#26134=CYLINDRICAL_SURFACE ( 'NONE', #28074, 11.92686044187656513 ) ;
#26136=EDGE_LOOP ( 'NONE', ( #58298, #22586, #11331, #55112 ) ) ;
#26142=ORIENTED_EDGE ( 'NONE', *, *, #205, .F. ) ;
#26148=VERTEX_POINT ( 'NONE', #73588 ) ;
#26149=CARTESIAN_POINT ( 'NONE',  ( -13.14228782657329653, 15.00000000000000000, -7.230509711182418364 ) ) ;
#26156=CARTESIAN_POINT ( 'NONE',  ( 7.684764310694878198, 0.5000000000000004441, -12.88194075009934991 ) ) ;
#26164=AXIS2_PLACEMENT_3D ( 'NONE', #71182, #24211, #93174 ) ;
#26165=CARTESIAN_POINT ( 'NONE',  ( 13.61464873478163007, 14.63595249122790598, 6.296136897217930795 ) ) ;
#26166=CARTESIAN_POINT ( 'NONE',  ( 0.000000000000000000, 15.00000000000000000, 0.000000000000000000 ) ) ;
#26169=CARTESIAN_POINT ( 'NONE',  ( -10.88017736071110164, -32.14464798917849464, -2.915334737309917212 ) ) ;
#26173=CARTESIAN_POINT ( 'NONE',  ( 8.564643372776533425, 0.3640475087720987379, 12.31449893000747053 ) ) ;
#26174=EDGE_CURVE ( 'NONE', #74650, #63206, #67575, .T. ) ;
#26186=DIRECTION ( 'NONE',  ( 0.000000000000000000, 0.000000000000000000, 1.000000000000000000 ) ) ;
#26191=ORIENTED_EDGE ( 'NONE', *, *, #21699, .F. ) ;
#26201=ADVANCED_FACE ( 'NONE', ( #73092 ), #80337, .T. ) ;
#26204=EDGE_CURVE ( 'NONE', #55265, #24815, #6900, .T. ) ;
#26207=CARTESIAN_POINT ( 'NONE',  ( 5.625000000000005329, 9.588468844518212464, 9.742785792574933268 ) ) ;
#26216=EDGE_CURVE ( 'NONE', #14939, #50302, #68123, .T. ) ;
#26218=CARTESIAN_POINT ( 'NONE',  ( -4.180366052176671232, -3.678240573451797645E-15, -14.01545757926333557 ) ) ;
#26219=CARTESIAN_POINT ( 'NONE',  ( 0.000000000000000000, 0.5000000000000004441, 0.000000000000000000 ) ) ;
#26225=ORIENTED_EDGE ( 'NONE', *, *, #50585, .T. ) ;
#26231=DIRECTION ( 'NONE',  ( -3.375077994860475883E-14, 0.000000000000000000, 1.000000000000000000 ) ) ;
#26234=CARTESIAN_POINT ( 'NONE',  ( -11.09922568453595382, -6.293031996736239364, -6.408140936763226492 ) ) ;
#26235=ORIENTED_EDGE ( 'NONE', *, *, #58802, .F. ) ;
#26238=VECTOR ( 'NONE', #20, 1000.000000000000000 ) ;
#26240=ORIENTED_EDGE ( 'NONE', *, *, #42464, .T. ) ;
#26249=DIRECTION ( 'NONE',  ( -0.000000000000000000, -1.000000000000000000, -0.000000000000000000 ) ) ;
#26257=CARTESIAN_POINT ( 'NONE',  ( 14.82269085861167035, 0.5000000000000004441, 2.299529454047060550 ) ) ;
#26265=CARTESIAN_POINT ( 'NONE',  ( 15.86177583122252344, -0.03417435944610275333, -2.069169861586653170 ) ) ;
#26273=CARTESIAN_POINT ( 'NONE',  ( -10.58981376305295008, -0.03417435944610275333, 9.535111140613638625 ) ) ;
#26277=CARTESIAN_POINT ( 'NONE',  ( -11.48952521350030587, 4.186587853438871531E-16, 8.845383562533662314 ) ) ;
#26296=EDGE_LOOP ( 'NONE', ( #92985, #30633, #50320, #23802 ) ) ;
#26298=CARTESIAN_POINT ( 'NONE',  ( 2.888614318722440899, 15.00000000000000888, -14.33855829812821980 ) ) ;
#26315=CIRCLE ( 'NONE', #77409, 14.49999999999999822 ) ;
#26323=EDGE_CURVE ( 'NONE', #65699, #18711, #51600, .T. ) ;
#26326=CARTESIAN_POINT ( 'NONE',  ( 0.000000000000000000, 12.49999999999999112, 0.000000000000000000 ) ) ;
#26334=AXIS2_PLACEMENT_3D ( 'NONE', #78129, #16652, #71131 ) ;
#26337=VERTEX_POINT ( 'NONE', #88104 ) ;
#26339=DIRECTION ( 'NONE',  ( 0.000000000000000000, 1.000000000000000000, 0.000000000000000000 ) ) ;
#26340=CARTESIAN_POINT ( 'NONE',  ( 0.000000000000000000, 0.5000000000000004441, 0.000000000000000000 ) ) ;
#26360=FACE_OUTER_BOUND ( 'NONE', #53578, .T. ) ;
#26361=VERTEX_POINT ( 'NONE', #50108 ) ;
#26362=TOROIDAL_SURFACE ( 'NONE', #80694, 14.49999999999999822, 0.5000000000000000000 ) ;
#26373=LINE ( 'NONE', #64362, #71433 ) ;
#26382=CARTESIAN_POINT ( 'NONE',  ( 3.014428414850136129, 6.576366962315981723, 11.25000000000000000 ) ) ;
#26391=CARTESIAN_POINT ( 'NONE',  ( 12.54342190210046759, 14.76984988503095764, -8.116945096741293497 ) ) ;
#26392=CARTESIAN_POINT ( 'NONE',  ( -7.993487411949188548, 0.04962888323599694979, -12.40005926694717786 ) ) ;
#26399=CARTESIAN_POINT ( 'NONE',  ( -3.795296366450300773, 2.845415501580633499, 14.16423886937410437 ) ) ;
#26402=ORIENTED_EDGE ( 'NONE', *, *, #93509, .T. ) ;
#26403=AXIS2_PLACEMENT_3D ( 'NONE', #36138, #66645, #34153 ) ;
#26417=CARTESIAN_POINT ( 'NONE',  ( 12.79413655343697265, 0.2301508429231309272, -7.715718893782876897 ) ) ;
#26426=AXIS2_PLACEMENT_3D ( 'NONE', #35650, #42665, #81146 ) ;
#26437=CARTESIAN_POINT ( 'NONE',  ( -5.810213597521615370, 14.95037102642602278, -13.56092647078879310 ) ) ;
#26438=EDGE_LOOP ( 'NONE', ( #35652, #40177, #2564, #2271, #1245, #98170 ) ) ;
#26441=CARTESIAN_POINT ( 'NONE',  ( -3.541595367958713769, 0.000000000000000000, 4.146675399920569660 ) ) ;
#26445=ORIENTED_EDGE ( 'NONE', *, *, #30927, .F. ) ;
#26449=EDGE_LOOP ( 'NONE', ( #46027, #98859, #74050, #30760, #9487, #98155 ) ) ;
#26453=VECTOR ( 'NONE', #92449, 999.9999999999998863 ) ;
#26465=CARTESIAN_POINT ( 'NONE',  ( -6.408140936763246032, -26.70969866340291077, -11.09922568453594316 ) ) ;
#26480=ORIENTED_EDGE ( 'NONE', *, *, #27801, .F. ) ;
#26497=ORIENTED_EDGE ( 'NONE', *, *, #94550, .T. ) ;
#26499=CARTESIAN_POINT ( 'NONE',  ( 5.817157072110707539, 14.63606918420059877, 13.82608706751094907 ) ) ;
#26503=CARTESIAN_POINT ( 'NONE',  ( -12.03829478939432462, 15.00000000000000888, 8.307695547791295709 ) ) ;
#26519=CARTESIAN_POINT ( 'NONE',  ( 11.94720539484412569, 0.2306972965111893092, -8.972309510150163092 ) ) ;
#26522=CARTESIAN_POINT ( 'NONE',  ( -7.082119434687044190, -32.36291783175269643, 12.26659068614894998 ) ) ;
#26532=B_SPLINE_CURVE_WITH_KNOTS ( 'NONE', 3,
 ( #79, #82053, #74553, #31992, #85514, #55512 ),
 .UNSPECIFIED., .F., .F.,
 ( 4, 2, 4 ),
 ( 0.0002800011564896231716, 0.0006862063972211615310, 0.001092411637952699728 ),
 .UNSPECIFIED. ) ;
#26534=DIRECTION ( 'NONE',  ( 0.000000000000000000, 1.000000000000000000, 0.000000000000000000 ) ) ;
#26539=CARTESIAN_POINT ( 'NONE',  ( -5.440088680355558814, 17.23035201082151602, -9.422509992056136596 ) ) ;
#26542=AXIS2_PLACEMENT_3D ( 'NONE', #34036, #43034, #65019 ) ;
#26547=DIRECTION ( 'NONE',  ( 0.000000000000000000, 1.000000000000000000, 0.000000000000000000 ) ) ;
#26548=EDGE_CURVE ( 'NONE', #79151, #22706, #63723, .T. ) ;
#26555=VERTEX_POINT ( 'NONE', #54535 ) ;
#26557=EDGE_CURVE ( 'NONE', #77887, #27971, #44580, .T. ) ;
#26559=DIRECTION ( 'NONE',  ( -0.09584575252022722869, 0.000000000000000000, 0.9953961983671785196 ) ) ;
#26575=LINE ( 'NONE', #11094, #3566 ) ;
#26579=VECTOR ( 'NONE', #86149, 1000.000000000000000 ) ;
#26580=B_SPLINE_CURVE_WITH_KNOTS ( 'NONE', 3,
 ( #59194, #11732, #26731, #3758, #66710, #34216 ),
 .UNSPECIFIED., .F., .F.,
 ( 4, 2, 4 ),
 ( 3.409110551495777647E-05, 0.0004400426677367824516, 0.0008459942299586071471 ),
 .UNSPECIFIED. ) ;
#26583=CARTESIAN_POINT ( 'NONE',  ( 2.638427012816835227, 7.467264484334121377, 9.846743663894590881 ) ) ;
#26584=VERTEX_POINT ( 'NONE', #60572 ) ;
#26586=DIRECTION ( 'NONE',  ( 0.000000000000000000, 0.000000000000000000, 1.000000000000000000 ) ) ;
#26592=CARTESIAN_POINT ( 'NONE',  ( 0.3329122712636403691, 0.000000000000000000, -5.443067521379384210 ) ) ;
#26597=VECTOR ( 'NONE', #23101, 1000.000000000000000 ) ;
#26599=ORIENTED_EDGE ( 'NONE', *, *, #64961, .F. ) ;
#26601=EDGE_LOOP ( 'NONE', ( #28898, #36538, #38070, #24179 ) ) ;
#26603=ORIENTED_EDGE ( 'NONE', *, *, #80162, .F. ) ;
#26611=CIRCLE ( 'NONE', #55392, 14.49999999999999822 ) ;
#26615=B_SPLINE_CURVE_WITH_KNOTS ( 'NONE', 3,
 ( #35771, #57287, #51270, #12282, #42789, #81272 ),
 .UNSPECIFIED., .F., .F.,
 ( 4, 2, 4 ),
 ( 0.0002800138956522149549, 0.0006862192609926520345, 0.001092424626333089168 ),
 .UNSPECIFIED. ) ;
#26616=LINE ( 'NONE', #87610, #59625 ) ;
#26631=CARTESIAN_POINT ( 'NONE',  ( -10.64017930668197209, 14.49999999999999112, -10.57291749337233000 ) ) ;
#26632=EDGE_CURVE ( 'NONE', #71139, #20387, #7856, .T. ) ;
#26635=DIRECTION ( 'NONE',  ( 0.3826834323650877834, -0.000000000000000000, -0.9238795325112876267 ) ) ;
#26636=EDGE_CURVE ( 'NONE', #8161, #75142, #85885, .T. ) ;
#26637=AXIS2_PLACEMENT_3D ( 'NONE', #8200, #230, #6711 ) ;
#26645=CARTESIAN_POINT ( 'NONE',  ( 11.32252723389645510, 12.55781760004707692, 0.3396460154096309636 ) ) ;
#26650=CARTESIAN_POINT ( 'NONE',  ( 2.915334737309928315, -30.47798132251182324, 10.88017736071109987 ) ) ;
#26652=CARTESIAN_POINT ( 'NONE',  ( 14.99847009497944583, 0.5000000000000004441, -0.2142307401080305596 ) ) ;
#26654=CARTESIAN_POINT ( 'NONE',  ( 12.60874940350947959, 15.00000000000000000, -7.160268045227033973 ) ) ;
#26655=CARTESIAN_POINT ( 'NONE',  ( -10.19513985507819598, 14.63606907090794351, -11.00268709613235174 ) ) ;
#26660=VECTOR ( 'NONE', #41102, 1000.000000000000000 ) ;
#26667=FACE_OUTER_BOUND ( 'NONE', #26682, .T. ) ;
#26670=ORIENTED_EDGE ( 'NONE', *, *, #1740, .T. ) ;
#26672=CARTESIAN_POINT ( 'NONE',  ( 0.000000000000000000, 14.49999999999999822, 0.000000000000000000 ) ) ;
#26682=EDGE_LOOP ( 'NONE', ( #127, #95373, #39065, #55893, #54635, #37545 ) ) ;
#26686=CARTESIAN_POINT ( 'NONE',  ( 5.991992585808537441, 4.355491999677157623E-16, 13.20401548210299048 ) ) ;
#26698=CARTESIAN_POINT ( 'NONE',  ( -2.863845842055730895, 0.04922511925147109862, -14.47219703936417545 ) ) ;
#26701=DIRECTION ( 'NONE',  ( 0.000000000000000000, 0.000000000000000000, 1.000000000000000000 ) ) ;
#26702=VERTEX_POINT ( 'NONE', #11350 ) ;
#26710=EDGE_CURVE ( 'NONE', #33681, #11587, #14749, .T. ) ;
#26715=CARTESIAN_POINT ( 'NONE',  ( -9.382169495545422677, 13.49863466993042316, -9.382169495545417348 ) ) ;
#26719=EDGE_LOOP ( 'NONE', ( #17160, #50676, #79502, #40738, #52927, #37379 ) ) ;
#26731=CARTESIAN_POINT ( 'NONE',  ( 10.17198128013136227, 0.2306972965111899476, 10.94389562857672438 ) ) ;
#26738=DIRECTION ( 'NONE',  ( -0.000000000000000000, -1.000000000000000000, -0.000000000000000000 ) ) ;
#26740=CARTESIAN_POINT ( 'NONE',  ( -1.983216688681034068, 15.00000000000000000, 14.11131997956736406 ) ) ;
#26745=CARTESIAN_POINT ( 'NONE',  ( 14.48718990079892066, 4.852832169489322230E-16, 0.6093675230841453239 ) ) ;
#26754=SHAPE_DEFINITION_REPRESENTATION ( #6738, #81163 ) ;
#26755=CARTESIAN_POINT ( 'NONE',  ( -12.87930560075679942, 14.95037102969557452, 7.195887444332292660 ) ) ;
#26756=ADVANCED_FACE ( 'NONE', ( #95342 ), #42350, .T. ) ;
#26759=VERTEX_POINT ( 'NONE', #40394 ) ;
#26768=DIRECTION ( 'NONE',  ( 0.000000000000000000, 0.000000000000000000, 1.000000000000000000 ) ) ;
#26773=AXIS2_PLACEMENT_3D ( 'NONE', #42093, #11579, #57077 ) ;
#26776=VERTEX_POINT ( 'NONE', #17399 ) ;
#26779=DIRECTION ( 'NONE',  ( 0.7933533402912409382, 0.000000000000000000, -0.6087614290087131064 ) ) ;
#26794=AXIS2_PLACEMENT_3D ( 'NONE', #7677, #44665, #83659 ) ;
#26796=DIRECTION ( 'NONE',  ( 0.9681476403781101858, 0.000000000000000000, -0.2503800040544323924 ) ) ;
#26797=CARTESIAN_POINT ( 'NONE',  ( 14.97687855664608314, 0.5000000000000004441, -0.8325315005900512100 ) ) ;
#26801=DIRECTION ( 'NONE',  ( 0.5519369853120676961, 0.000000000000000000, -0.8338858220671618859 ) ) ;
#26804=AXIS2_PLACEMENT_3D ( 'NONE', #42892, #89371, #66363 ) ;
#26808=CARTESIAN_POINT ( 'NONE',  ( -2.174473938468956646, 0.000000000000000000, 5.000947681547202706 ) ) ;
#26814=DIRECTION ( 'NONE',  ( -0.000000000000000000, -1.000000000000000000, -0.000000000000000000 ) ) ;
#26825=EDGE_LOOP ( 'NONE', ( #38930, #17272, #55163, #12598, #39967, #91011 ) ) ;
#26832=DIRECTION ( 'NONE',  ( 0.000000000000000000, 1.000000000000000000, 0.000000000000000000 ) ) ;
#26840=ORIENTED_EDGE ( 'NONE', *, *, #40456, .F. ) ;
#26846=CARTESIAN_POINT ( 'NONE',  ( -13.95749458852073133, 14.76930270348882068, -5.331641351773216186 ) ) ;
#26853=DIRECTION ( 'NONE',  ( 0.000000000000000000, 0.000000000000000000, 1.000000000000000000 ) ) ;
#26854=ORIENTED_EDGE ( 'NONE', *, *, #37493, .F. ) ;
#26858=EDGE_LOOP ( 'NONE', ( #37639, #94198, #38779, #73064 ) ) ;
#26865=CARTESIAN_POINT ( 'NONE',  ( -14.49154782522698071, 14.95037109980891543, -2.766288502467150412 ) ) ;
#26868=VECTOR ( 'NONE', #33546, 1000.000000000000000 ) ;
#26873=CIRCLE ( 'NONE', #93977, 14.49999999999999822 ) ;
#26879=CARTESIAN_POINT ( 'NONE',  ( 9.742785792574936821, 7.201366962315986164, 5.624999999999996447 ) ) ;
#26883=FACE_OUTER_BOUND ( 'NONE', #76035, .T. ) ;
#26889=LINE ( 'NONE', #50371, #6298 ) ;
#26906=LINE ( 'NONE', #95915, #51257 ) ;
#26915=CARTESIAN_POINT ( 'NONE',  ( 14.24131928502211331, -0.03417435944610275333, 0.4973178280106892446 ) ) ;
#26920=CARTESIAN_POINT ( 'NONE',  ( 0.000000000000000000, 14.49999999999999822, 0.000000000000000000 ) ) ;
#26923=CARTESIAN_POINT ( 'NONE',  ( -10.84451454130513426, 4.265732461173792237E-16, 9.625305416630759225 ) ) ;
#26931=FACE_OUTER_BOUND ( 'NONE', #10132, .T. ) ;
#26942=AXIS2_PLACEMENT_3D ( 'NONE', #78620, #31626, #69642 ) ;
#26944=CARTESIAN_POINT ( 'NONE',  ( -14.24131928502210975, 0.000000000000000000, -0.4973178280107823923 ) ) ;
#26946=VERTEX_POINT ( 'NONE', #59521 ) ;
#26957=CARTESIAN_POINT ( 'NONE',  ( -5.991992585808451288, 3.888230080364882544E-16, -13.20401548210303311 ) ) ;
#26961=CARTESIAN_POINT ( 'NONE',  ( 3.434112377981054287, -27.33469866340291077, -12.81628187352647608 ) ) ;
#26968=ADVANCED_FACE ( 'NONE', ( #82521 ), #90502, .F. ) ;
#26971=DIRECTION ( 'NONE',  ( 0.000000000000000000, 1.000000000000000000, 0.000000000000000000 ) ) ;
#26972=EDGE_CURVE ( 'NONE', #35670, #8560, #55813, .T. ) ;
#26974=VERTEX_POINT ( 'NONE', #22527 ) ;
#26981=CARTESIAN_POINT ( 'NONE',  ( -14.04391541078760675, 15.00000000000000000, -3.608107528143027043 ) ) ;
#26987=LINE ( 'NONE', #4991, #54735 ) ;
#26990=ORIENTED_EDGE ( 'NONE', *, *, #89741, .F. ) ;
#26991=CARTESIAN_POINT ( 'NONE',  ( -8.606322355891443010, 3.794835101497137347E-16, 11.66967075398801335 ) ) ;
#26994=ORIENTED_EDGE ( 'NONE', *, *, #28772, .F. ) ;
#26998=DIRECTION ( 'NONE',  ( 0.000000000000000000, 1.000000000000000000, 0.000000000000000000 ) ) ;
#27014=CARTESIAN_POINT ( 'NONE',  ( 3.795296366450306547, -29.65458449841936428, -14.16423886937410259 ) ) ;
#27023=CARTESIAN_POINT ( 'NONE',  ( -14.82629065241402699, 14.76984952912780003, -1.844815641836186293 ) ) ;
#27026=ADVANCED_FACE ( 'NONE', ( #30987 ), #46489, .T. ) ;
#27029=CARTESIAN_POINT ( 'NONE',  ( 10.88017736071110164, 15.35535201082150891, 2.915334737309921209 ) ) ;
#27031=CARTESIAN_POINT ( 'NONE',  ( -11.94665733272764463, 0.2301501672491015338, -8.972157519073791221 ) ) ;
#27042=LINE ( 'NONE', #5050, #9832 ) ;
#27044=ORIENTED_EDGE ( 'NONE', *, *, #80497, .T. ) ;
#27057=DIRECTION ( 'NONE',  ( 0.000000000000000000, 0.000000000000000000, 1.000000000000000000 ) ) ;
#27071=CARTESIAN_POINT ( 'NONE',  ( -7.208316651077756099, 6.633931151000788340, 7.208316651077766757 ) ) ;
#27076=ORIENTED_EDGE ( 'NONE', *, *, #17316, .T. ) ;
#27081=DIRECTION ( 'NONE',  ( 0.000000000000000000, 0.000000000000000000, 1.000000000000000000 ) ) ;
#27082=EDGE_CURVE ( 'NONE', #41530, #30913, #39004, .T. ) ;
#27098=ORIENTED_EDGE ( 'NONE', *, *, #82331, .F. ) ;
#27107=CARTESIAN_POINT ( 'NONE',  ( 7.313705784284593392, 15.00000000000000000, -13.09617149020743732 ) ) ;
#27108=ORIENTED_EDGE ( 'NONE', *, *, #46885, .F. ) ;
#27110=CARTESIAN_POINT ( 'NONE',  ( -1.326515405095929800, 14.76930270348882068, -14.88215077106016970 ) ) ;
#27116=CARTESIAN_POINT ( 'NONE',  ( -12.00809552683946357, 0.5000000000000004441, -8.989195838243713155 ) ) ;
#27124=EDGE_LOOP ( 'NONE', ( #88297, #3629, #96856, #19610, #13285, #4731 ) ) ;
#27133=CARTESIAN_POINT ( 'NONE',  ( 0.000000000000000000, 0.000000000000000000, 0.000000000000000000 ) ) ;
#27136=CARTESIAN_POINT ( 'NONE',  ( -10.88017736071110164, -22.14464798917849109, -2.915334737309917212 ) ) ;
#27141=CARTESIAN_POINT ( 'NONE',  ( -10.19513985507820486, 14.49999999999999112, -11.00268709613237306 ) ) ;
#27152=CARTESIAN_POINT ( 'NONE',  ( -14.69227023463708726, 14.95077488074851502, -1.335400878252729573 ) ) ;
#27162=DIRECTION ( 'NONE',  ( 0.000000000000000000, 1.000000000000000000, 0.000000000000000000 ) ) ;
#27172=ORIENTED_EDGE ( 'NONE', *, *, #94988, .T. ) ;
#27188=CARTESIAN_POINT ( 'NONE',  ( 2.638427012816829897, -35.44940218233254114, -9.846743663894592657 ) ) ;
#27197=CARTESIAN_POINT ( 'NONE',  ( 0.000000000000000000, 15.00000000000000000, 0.000000000000000000 ) ) ;
#27200=B_SPLINE_CURVE_WITH_KNOTS ( 'NONE', 3,
 ( #73316, #20330, #18854, #66807, #19823, #35315 ),
 .UNSPECIFIED., .F., .F.,
 ( 4, 2, 4 ),
 ( 0.0002800808511812542118, 0.0006862868719359076263, 0.001092492892690561041 ),
 .UNSPECIFIED. ) ;
#27203=CARTESIAN_POINT ( 'NONE',  ( 3.434112377981054287, 2.665301336597088788, -12.81628187352647608 ) ) ;
#27217=EDGE_CURVE ( 'NONE', #8762, #9509, #63775, .T. ) ;
#27218=CARTESIAN_POINT ( 'NONE',  ( 14.37657372141816126, 15.00000000000000888, -2.693041920167344117 ) ) ;
#27220=CARTESIAN_POINT ( 'NONE',  ( 0.7166339456633684657, 0.000000000000000000, -15.98010739087745868 ) ) ;
#27224=VECTOR ( 'NONE', #54943, 1000.000000000000000 ) ;
#27225=ADVANCED_FACE ( 'NONE', ( #41478 ), #31882, .T. ) ;
#27226=DIRECTION ( 'NONE',  ( 0.4305110968082926370, 0.000000000000000000, 0.9025852843498617384 ) ) ;
#27229=CARTESIAN_POINT ( 'NONE',  ( -9.641087339108999288, 0.04922511925147086270, 11.16671550067042418 ) ) ;
#27233=CARTESIAN_POINT ( 'NONE',  ( -4.023424921641842289, 15.00000000000000000, 15.48190712851503648 ) ) ;
#27234=CARTESIAN_POINT ( 'NONE',  ( 7.684764310694791156, 0.3640475087720984049, 12.88194075009940853 ) ) ;
#27246=CARTESIAN_POINT ( 'NONE',  ( -5.624999999999997335, 3.755135511184878538, 9.742785792574938597 ) ) ;
#27257=CARTESIAN_POINT ( 'NONE',  ( 12.00809552683965364, 14.49999999999999112, -8.989195838243565717 ) ) ;
#27259=EDGE_CURVE ( 'NONE', #14459, #80097, #32957, .T. ) ;
#27267=DIRECTION ( 'NONE',  ( 0.9304175679820282374, 0.000000000000000000, -0.3665012267242880872 ) ) ;
#27268=CARTESIAN_POINT ( 'NONE',  ( 9.898881779040660689, 0.000000000000000000, 10.25059215482582786 ) ) ;
#27298=CARTESIAN_POINT ( 'NONE',  ( 8.439016546559823695, 15.00000000000000000, 11.79122553964979048 ) ) ;
#27302=VECTOR ( 'NONE', #84377, 1000.000000000000000 ) ;
#27307=ORIENTED_EDGE ( 'NONE', *, *, #57997, .F. ) ;
#27310=ORIENTED_EDGE ( 'NONE', *, *, #70682, .F. ) ;
#27314=DIRECTION ( 'NONE',  ( 0.000000000000000000, 1.000000000000000000, 0.000000000000000000 ) ) ;
#27316=CARTESIAN_POINT ( 'NONE',  ( -12.98685442714190508, 4.246409518909109890E-16, -6.449155920601135072 ) ) ;
#27319=CARTESIAN_POINT ( 'NONE',  ( -3.195792623639597263, 11.62045670184115664, -11.92686044187653494 ) ) ;
#27324=EDGE_CURVE ( 'NONE', #15285, #26110, #16994, .T. ) ;
#27330=ORIENTED_EDGE ( 'NONE', *, *, #19518, .F. ) ;
#27341=AXIS2_PLACEMENT_3D ( 'NONE', #89993, #89506, #60967 ) ;
#27349=VERTEX_POINT ( 'NONE', #82395 ) ;
#27350=CARTESIAN_POINT ( 'NONE',  ( -7.595945211628411187, 15.00000000000000000, 12.35117874301633734 ) ) ;
#27373=CARTESIAN_POINT ( 'NONE',  ( 12.83294900548064099, 14.63595249122789177, -7.766300266068371982 ) ) ;
#27378=CARTESIAN_POINT ( 'NONE',  ( 7.684764310694801814, 14.49999999999999112, 12.88194075009947248 ) ) ;
#27379=VECTOR ( 'NONE', #52637, 1000.000000000000000 ) ;
#27381=CARTESIAN_POINT ( 'NONE',  ( -7.771322705631335204, 4.741813304736951008E-16, -12.24159072199927678 ) ) ;
#27383=ORIENTED_EDGE ( 'NONE', *, *, #26174, .F. ) ;
#27386=CARTESIAN_POINT ( 'NONE',  ( 14.26139399674457309, 4.693468746458063789E-16, -2.619664342929806988 ) ) ;
#27390=CARTESIAN_POINT ( 'NONE',  ( -14.62617646268084926, 14.63595249122789177, -3.327906561567075983 ) ) ;
#27392=CARTESIAN_POINT ( 'NONE',  ( -11.24999999999999822, 8.130135511184871433, 3.014428414850141458 ) ) ;
#27395=CARTESIAN_POINT ( 'NONE',  ( -14.09356342482591451, 14.95077488074853456, -4.360913911515565289 ) ) ;
#27397=DIRECTION ( 'NONE',  ( 0.000000000000000000, 0.000000000000000000, 1.000000000000000000 ) ) ;
#27398=VERTEX_POINT ( 'NONE', #12914 ) ;
#27430=ORIENTED_EDGE ( 'NONE', *, *, #90385, .T. ) ;
#27433=CARTESIAN_POINT ( 'NONE',  ( 0.000000000000000000, 35.00000000000000000, 0.000000000000000000 ) ) ;
#27438=ADVANCED_FACE ( 'NONE', ( #36413 ), #70166, .T. ) ;
#27442=CARTESIAN_POINT ( 'NONE',  ( -1.354709868695722852, 0.5000000000000004441, 14.93870011653150698 ) ) ;
#27447=ADVANCED_FACE ( 'NONE', ( #57432 ), #27911, .F. ) ;
#27448=DIRECTION ( 'NONE',  ( 0.000000000000000000, 1.000000000000000000, 0.000000000000000000 ) ) ;
#27450=CIRCLE ( 'NONE', #30650, 15.00000000000000000 ) ;
#27453=CARTESIAN_POINT ( 'NONE',  ( -6.408140936763232709, -35.04303199673624647, 11.09922568453595026 ) ) ;
#27454=VECTOR ( 'NONE', #11025, 1000.000000000000000 ) ;
#27463=CARTESIAN_POINT ( 'NONE',  ( -14.26139399674456776, 15.00000000000000000, 2.619664342929695966 ) ) ;
#27481=VERTEX_POINT ( 'NONE', #57917 ) ;
#27488=CARTESIAN_POINT ( 'NONE',  ( 4.023424921641736596, -0.03417435944610275333, -15.48190712851506667 ) ) ;
#27503=CARTESIAN_POINT ( 'NONE',  ( -3.795296366450300773, -32.15458449841936073, 14.16423886937410437 ) ) ;
#27515=CARTESIAN_POINT ( 'NONE',  ( 14.22901244993681757, 15.00000000000000888, 3.387263120971414576 ) ) ;
#27518=CARTESIAN_POINT ( 'NONE',  ( -6.742022620658322474, 0.04962897188439633483, 13.12259272460500092 ) ) ;
#27520=CARTESIAN_POINT ( 'NONE',  ( 10.88017736071109987, 10.77201867748817321, -2.915334737309928315 ) ) ;
#27523=VERTEX_POINT ( 'NONE', #87925 ) ;
#27530=CARTESIAN_POINT ( 'NONE',  ( 0.000000000000000000, 0.5000000000000004441, 0.000000000000000000 ) ) ;
#27536=CARTESIAN_POINT ( 'NONE',  ( 0.000000000000000000, 14.49999999999999822, 0.000000000000000000 ) ) ;
#27547=CARTESIAN_POINT ( 'NONE',  ( 13.61464873478166737, 0.5000000000000004441, -6.296136897217838424 ) ) ;
#27551=ORIENTED_EDGE ( 'NONE', *, *, #64906, .T. ) ;
#27552=VERTEX_POINT ( 'NONE', #89899 ) ;
#27553=AXIS2_PLACEMENT_3D ( 'NONE', #79372, #56860, #49846 ) ;
#27559=CARTESIAN_POINT ( 'NONE',  ( 0.000000000000000000, 14.49999999999999822, 0.000000000000000000 ) ) ;
#27566=CARTESIAN_POINT ( 'NONE',  ( -7.208316651077756099, 1.633931151000786341, 7.208316651077766757 ) ) ;
#27567=ORIENTED_EDGE ( 'NONE', *, *, #55005, .T. ) ;
#27568=CARTESIAN_POINT ( 'NONE',  ( -7.771322705631335204, 4.741813304736951008E-16, -12.24159072199927678 ) ) ;
#27570=CARTESIAN_POINT ( 'NONE',  ( 13.61464873478173843, 14.49999999999999112, -6.296136897217843753 ) ) ;
#27576=CARTESIAN_POINT ( 'NONE',  ( 12.07856007377822394, 4.551077920620485022E-16, 8.022367888854921247 ) ) ;
#27578=AXIS2_PLACEMENT_3D ( 'NONE', #41949, #49419, #65897 ) ;
#27592=AXIS2_PLACEMENT_3D ( 'NONE', #52250, #28754, #66251 ) ;
#27596=EDGE_CURVE ( 'NONE', #65885, #42615, #72924, .T. ) ;
#27598=ORIENTED_EDGE ( 'NONE', *, *, #19770, .F. ) ;
#27605=CARTESIAN_POINT ( 'NONE',  ( -9.509319644403765537, 13.17686044187662020, 7.198808227794258663 ) ) ;
#27609=DIRECTION ( 'NONE',  ( -0.1993679344172108459, -0.000000000000000000, 0.9799247046208268141 ) ) ;
#27610=VERTEX_POINT ( 'NONE', #98919 ) ;
#27622=VERTEX_POINT ( 'NONE', #9732 ) ;
#27628=DIRECTION ( 'NONE',  ( -0.000000000000000000, -1.000000000000000000, -0.000000000000000000 ) ) ;
#27629=CARTESIAN_POINT ( 'NONE',  ( -3.897244926436316703, 15.00000000000000000, 13.96644127841325300 ) ) ;
#27635=CARTESIAN_POINT ( 'NONE',  ( -7.964842623401172439, -26.31131465584515539, 7.964842623401183097 ) ) ;
#27647=CARTESIAN_POINT ( 'NONE',  ( 2.962741594153077251, 0.000000000000000000, -13.93860331045673107 ) ) ;
#27648=AXIS2_PLACEMENT_3D ( 'NONE', #76674, #15705, #83694 ) ;
#27663=CARTESIAN_POINT ( 'NONE',  ( -12.80781515976305762, 15.00000000000000000, -6.246788841744501219 ) ) ;
#27666=CARTESIAN_POINT ( 'NONE',  ( -14.16722289976688565, 15.00000000000000000, 4.928467845925418089 ) ) ;
#27668=EDGE_LOOP ( 'NONE', ( #79985, #77231, #79900, #83761, #97327, #30320 ) ) ;
#27670=CARTESIAN_POINT ( 'NONE',  ( -14.24131928502211863, 15.00000000000000000, 0.4973178280104966764 ) ) ;
#27686=EDGE_CURVE ( 'NONE', #56421, #4086, #75386, .T. ) ;
#27687=CARTESIAN_POINT ( 'NONE',  ( 9.846743663894590881, -36.69940218233254114, 2.638427012816828565 ) ) ;
#27688=ORIENTED_EDGE ( 'NONE', *, *, #70921, .T. ) ;
#27690=EDGE_LOOP ( 'NONE', ( #66517, #96293, #87567, #37873 ) ) ;
#27696=CARTESIAN_POINT ( 'NONE',  ( 13.78891971893208357, 0.5000000000000004441, -5.904717858191528279 ) ) ;
#27699=CARTESIAN_POINT ( 'NONE',  ( -12.81628187352647252, 4.331968003263747313, 3.434112377981066722 ) ) ;
#27705=EDGE_CURVE ( 'NONE', #78351, #21503, #48968, .T. ) ;
#27713=B_SPLINE_CURVE_WITH_KNOTS ( 'NONE', 3,
 ( #94656, #26165, #56658, #72144, #92685, #54677 ),
 .UNSPECIFIED., .F., .F.,
 ( 4, 2, 4 ),
 ( 3.409110551496208618E-05, 0.0004400426677367994194, 0.0008459942299586367459 ),
 .UNSPECIFIED. ) ;
#27714=CARTESIAN_POINT ( 'NONE',  ( 12.34086200392821908, 0.000000000000000000, 7.125000000000058620 ) ) ;
#27716=CARTESIAN_POINT ( 'NONE',  ( 0.000000000000000000, 14.49999999999999822, 0.000000000000000000 ) ) ;
#27717=LINE ( 'NONE', #21215, #54748 ) ;
#27718=CARTESIAN_POINT ( 'NONE',  ( -12.83294900548068895, 0.5000000000000004441, 7.766300266068274283 ) ) ;
#27728=DIRECTION ( 'NONE',  ( -0.8433914458128884961, 0.000000000000000000, 0.5372996083468194461 ) ) ;
#27731=DIRECTION ( 'NONE',  ( 0.000000000000000000, 1.000000000000000000, 0.000000000000000000 ) ) ;
#27739=CARTESIAN_POINT ( 'NONE',  ( -3.014428414850141458, 4.076366962315985276, -11.25000000000000000 ) ) ;
#27755=ADVANCED_FACE ( 'NONE', ( #45897 ), #93712, .F. ) ;
#27759=VERTEX_POINT ( 'NONE', #93216 ) ;
#27770=ORIENTED_EDGE ( 'NONE', *, *, #34348, .F. ) ;
#27778=CARTESIAN_POINT ( 'NONE',  ( -0.8653096853310142667, 14.99999999999806377, -14.59999144043309016 ) ) ;
#27779=CARTESIAN_POINT ( 'NONE',  ( -6.382347221874512755, 15.00000000000000000, 13.57444820018223375 ) ) ;
#27786=VERTEX_POINT ( 'NONE', #83886 ) ;
#27795=CARTESIAN_POINT ( 'NONE',  ( -7.684764310694707667, 0.5000000000000004441, -12.88194075009945472 ) ) ;
#27796=CARTESIAN_POINT ( 'NONE',  ( -12.60589901313227124, 15.00000000000000000, 8.129656208641961257 ) ) ;
#27801=EDGE_CURVE ( 'NONE', #89795, #87207, #55218, .T. ) ;
#27807=ORIENTED_EDGE ( 'NONE', *, *, #40035, .F. ) ;
#27811=LINE ( 'NONE', #78852, #64900 ) ;
#27812=DIRECTION ( 'NONE',  ( -0.000000000000000000, -1.000000000000000000, -0.000000000000000000 ) ) ;
#27813=ORIENTED_EDGE ( 'NONE', *, *, #33783, .T. ) ;
#27824=DIRECTION ( 'NONE',  ( 0.7604059656000297096, -0.000000000000000000, 0.6494480483301851015 ) ) ;
#27830=VECTOR ( 'NONE', #4820, 1000.000000000000114 ) ;
#27831=EDGE_CURVE ( 'NONE', #27552, #94563, #54293, .T. ) ;
#27851=CARTESIAN_POINT ( 'NONE',  ( 0.000000000000000000, 15.00000000000000000, 0.000000000000000000 ) ) ;
#27854=AXIS2_PLACEMENT_3D ( 'NONE', #82959, #14474, #88481 ) ;
#27858=B_SPLINE_CURVE_WITH_KNOTS ( 'NONE', 3,
 ( #35776, #13273, #30109, #60615, #42796, #96800 ),
 .UNSPECIFIED., .F., .F.,
 ( 4, 2, 4 ),
 ( 0.0002800065468393074129, 0.0006862118402932828112, 0.001092417133747258318 ),
 .UNSPECIFIED. ) ;
#27863=CARTESIAN_POINT ( 'NONE',  ( 7.684764310694887079, 0.3639308364404311713, -12.88194075009938899 ) ) ;
#27867=DIRECTION ( 'NONE',  ( -0.000000000000000000, -1.000000000000000000, -0.000000000000000000 ) ) ;
#27878=CARTESIAN_POINT ( 'NONE',  ( 14.99847009497950800, 14.49999999999999112, -0.2142307401080081053 ) ) ;
#27880=EDGE_CURVE ( 'NONE', #76346, #51781, #17247, .T. ) ;
#27881=EDGE_CURVE ( 'NONE', #86629, #5244, #58860, .T. ) ;
#27882=CARTESIAN_POINT ( 'NONE',  ( 0.000000000000000000, 0.5000000000000004441, 0.000000000000000000 ) ) ;
#27889=ORIENTED_EDGE ( 'NONE', *, *, #87102, .T. ) ;
#27895=CARTESIAN_POINT ( 'NONE',  ( 0.000000000000000000, 14.49999999999999822, 0.000000000000000000 ) ) ;
#27896=DIRECTION ( 'NONE',  ( -0.000000000000000000, -1.000000000000000000, -0.000000000000000000 ) ) ;
#27901=PLANE ( 'NONE',  #27578 ) ;
#27903=CIRCLE ( 'NONE', #61445, 14.49999999999999822 ) ;
#27910=DIRECTION ( 'NONE',  ( 0.000000000000000000, 1.000000000000000000, 0.000000000000000000 ) ) ;
#27911=PLANE ( 'NONE',  #67015 ) ;
#27919=ORIENTED_EDGE ( 'NONE', *, *, #95494, .T. ) ;
#27920=VECTOR ( 'NONE', #9456, 1000.000000000000000 ) ;
#27923=CARTESIAN_POINT ( 'NONE',  ( -12.22474924877131031, 14.76984934309701636, -8.589397507025012146 ) ) ;
#27928=CARTESIAN_POINT ( 'NONE',  ( 0.000000000000000000, 0.000000000000000000, 0.000000000000000000 ) ) ;
#27931=AXIS2_PLACEMENT_3D ( 'NONE', #67341, #59335, #50356 ) ;
#27937=DIRECTION ( 'NONE',  ( 0.7604059656000297096, 0.000000000000000000, 0.6494480483301851015 ) ) ;
#27942=CARTESIAN_POINT ( 'NONE',  ( 11.09922568453595026, -13.79303199673624647, 6.408140936763232709 ) ) ;
#27952=DIRECTION ( 'NONE',  ( -0.000000000000000000, -1.000000000000000000, -0.000000000000000000 ) ) ;
#27971=VERTEX_POINT ( 'NONE', #71501 ) ;
#27978=DIRECTION ( 'NONE',  ( 0.000000000000000000, 0.000000000000000000, 1.000000000000000000 ) ) ;
#27984=CARTESIAN_POINT ( 'NONE',  ( -11.42945456197624665, 15.00000000000000888, 9.127207413380620693 ) ) ;
#27996=CARTESIAN_POINT ( 'NONE',  ( -7.082119434687058401, -14.02958449841935895, -12.26659068614894110 ) ) ;
#28000=VERTEX_POINT ( 'NONE', #25513 ) ;
#28002=VECTOR ( 'NONE', #4456, 1000.000000000000114 ) ;
#28003=EDGE_CURVE ( 'NONE', #46643, #23582, #12755, .T. ) ;
#28010=CARTESIAN_POINT ( 'NONE',  ( -6.715867195167534831, 4.123781235506717606E-16, 12.85095824508322693 ) ) ;
#28013=CARTESIAN_POINT ( 'NONE',  ( -5.440088680355547268, 18.89701867748817676, 9.422509992056143702 ) ) ;
#28015=ORIENTED_EDGE ( 'NONE', *, *, #87250, .T. ) ;
#28021=CARTESIAN_POINT ( 'NONE',  ( -14.17193700899791153, -0.03417435944610275333, 1.489530601563921808 ) ) ;
#28022=VECTOR ( 'NONE', #82610, 1000.000000000000114 ) ;
#28024=EDGE_CURVE ( 'NONE', #28504, #60588, #31988, .T. ) ;
#28028=CARTESIAN_POINT ( 'NONE',  ( 5.963430220938287007, 9.328790035174485240, 10.32896413005679825 ) ) ;
#28037=FACE_OUTER_BOUND ( 'NONE', #12335, .T. ) ;
#28042=FACE_OUTER_BOUND ( 'NONE', #42138, .T. ) ;
#28051=VECTOR ( 'NONE', #33319, 1000.000000000000000 ) ;
#28057=DIRECTION ( 'NONE',  ( 0.000000000000000000, 0.000000000000000000, 1.000000000000000000 ) ) ;
#28060=CARTESIAN_POINT ( 'NONE',  ( 9.846743663894590881, 3.717264484334123598, -2.638427012816833894 ) ) ;
#28061=ORIENTED_EDGE ( 'NONE', *, *, #18993, .F. ) ;
#28062=ORIENTED_EDGE ( 'NONE', *, *, #27082, .F. ) ;
#28071=CIRCLE ( 'NONE', #26426, 11.25000000000000178 ) ;
#28072=VECTOR ( 'NONE', #32855, 1000.000000000000000 ) ;
#28073=AXIS2_PLACEMENT_3D ( 'NONE', #43843, #74338, #91323 ) ;
#28074=AXIS2_PLACEMENT_3D ( 'NONE', #41150, #8664, #17660 ) ;
#28079=ORIENTED_EDGE ( 'NONE', *, *, #30121, .F. ) ;
#28085=DIRECTION ( 'NONE',  ( -3.996802888650564177E-14, 0.000000000000000000, 1.000000000000000000 ) ) ;
#28087=CARTESIAN_POINT ( 'NONE',  ( 1.175037534397131322, -2.824431362619463692E-15, 14.57833316477037400 ) ) ;
#28090=AXIS2_PLACEMENT_3D ( 'NONE', #14127, #6127, #85450 ) ;
#28098=DIRECTION ( 'NONE',  ( 0.000000000000000000, 1.000000000000000000, 0.000000000000000000 ) ) ;
#28101=ORIENTED_EDGE ( 'NONE', *, *, #54099, .F. ) ;
#28105=AXIS2_PLACEMENT_3D ( 'NONE', #32068, #71082, #17102 ) ;
#28106=VECTOR ( 'NONE', #20122, 1000.000000000000000 ) ;
#28123=B_SPLINE_CURVE_WITH_KNOTS ( 'NONE', 3,
 ( #48283, #86791, #39329, #77796, #78795, #62296 ),
 .UNSPECIFIED., .F., .F.,
 ( 4, 2, 4 ),
 ( 3.409110551494651432E-05, 0.0004400426677367913963, 0.0008459942299586362038 ),
 .UNSPECIFIED. ) ;
#28125=DIRECTION ( 'NONE',  ( -0.000000000000000000, -1.000000000000000000, -0.000000000000000000 ) ) ;
#28130=CARTESIAN_POINT ( 'NONE',  ( 7.964842623401181321, -30.06131465584516249, 7.964842623401174215 ) ) ;
#28135=CARTESIAN_POINT ( 'NONE',  ( 2.261421327065750830, 0.000000000000000000, -4.962236210031242045 ) ) ;
#28159=DIRECTION ( 'NONE',  ( -0.8241261886220241362, -0.000000000000000000, 0.5664062369248205053 ) ) ;
#28160=DIRECTION ( 'NONE',  ( 0.9981347984218662539, 0.000000000000000000, 0.06104853953487057033 ) ) ;
#28162=ORIENTED_EDGE ( 'NONE', *, *, #11560, .F. ) ;
#28163=CARTESIAN_POINT ( 'NONE',  ( 2.913501739333663743, 15.00000000000000000, 14.20427779279537184 ) ) ;
#28165=CIRCLE ( 'NONE', #25053, 15.00000000000000000 ) ;
#28181=LINE ( 'NONE', #65678, #35476 ) ;
#28184=CARTESIAN_POINT ( 'NONE',  ( -3.469446951953614189E-15, -35.24106884899921255, -9.846743663894594434 ) ) ;
#28188=ORIENTED_EDGE ( 'NONE', *, *, #42477, .F. ) ;
#28195=CARTESIAN_POINT ( 'NONE',  ( 3.469446951953614189E-15, 10.37363466993042316, 12.81628187352647608 ) ) ;
#28196=ORIENTED_EDGE ( 'NONE', *, *, #96714, .F. ) ;
#28208=CARTESIAN_POINT ( 'NONE',  ( 0.000000000000000000, 14.49999999999999822, 0.000000000000000000 ) ) ;
#28210=DIRECTION ( 'NONE',  ( -0.000000000000000000, -1.000000000000000000, -0.000000000000000000 ) ) ;
#28212=TOROIDAL_SURFACE ( 'NONE', #23465, 14.49999999999999822, 0.5000000000000000000 ) ;
#28213=DIRECTION ( 'NONE',  ( 0.000000000000000000, -1.000000000000000000, 0.000000000000000000 ) ) ;
#28216=CARTESIAN_POINT ( 'NONE',  ( 3.115783986955559470, 4.823715477197806954E-16, -14.16128137375397777 ) ) ;
#28223=CARTESIAN_POINT ( 'NONE',  ( 13.34343830728404079, 15.00000000000000000, -6.852200678592596184 ) ) ;
#28229=TOROIDAL_SURFACE ( 'NONE', #84139, 14.49999999999999822, 0.5000000000000000000 ) ;
#28237=ORIENTED_EDGE ( 'NONE', *, *, #34348, .T. ) ;
#28245=DIRECTION ( 'NONE',  ( -0.5664062369248369366, 0.000000000000000000, 0.8241261886220129229 ) ) ;
#28249=CARTESIAN_POINT ( 'NONE',  ( -7.082119434687058401, 10.97041550158064283, -12.26659068614894110 ) ) ;
#28257=ORIENTED_EDGE ( 'NONE', *, *, #8210, .F. ) ;
#28261=CARTESIAN_POINT ( 'NONE',  ( -13.75801628063875803, 15.00000000000000000, -4.578972376164643698 ) ) ;
#28263=CIRCLE ( 'NONE', #85743, 15.00000000000000000 ) ;
#28264=LINE ( 'NONE', #66760, #13191 ) ;
#28267=VERTEX_POINT ( 'NONE', #50945 ) ;
#28275=DIRECTION ( 'NONE',  ( 0.06104853953485662316, 0.000000000000000000, 0.9981347984218670311 ) ) ;
#28276=EDGE_CURVE ( 'NONE', #36269, #49707, #81439, .T. ) ;
#28286=ORIENTED_EDGE ( 'NONE', *, *, #68762, .T. ) ;
#28288=DIRECTION ( 'NONE',  ( -0.9170600743851211600, 0.000000000000000000, -0.3987490689252528031 ) ) ;
#28294=AXIS2_PLACEMENT_3D ( 'NONE', #24071, #40048, #1085 ) ;
#28298=CARTESIAN_POINT ( 'NONE',  ( -14.69227023463711568, 0.04922511925147164680, 1.335400878252435808 ) ) ;
#28303=ORIENTED_EDGE ( 'NONE', *, *, #11000, .F. ) ;
#28311=FACE_OUTER_BOUND ( 'NONE', #11482, .T. ) ;
#28331=ORIENTED_EDGE ( 'NONE', *, *, #40561, .F. ) ;
#28337=AXIS2_PLACEMENT_3D ( 'NONE', #78887, #76917, #77898 ) ;
#28340=CARTESIAN_POINT ( 'NONE',  ( -7.640917710489092407, 14.95077488074853811, 12.61992379908748418 ) ) ;
#28344=CARTESIAN_POINT ( 'NONE',  ( -7.313705784284714184, 14.63606873438734546, 13.09617149020741778 ) ) ;
#28347=CARTESIAN_POINT ( 'NONE',  ( 10.84451454130500636, 4.196149184706192213E-16, 9.625305416630906663 ) ) ;
#28353=EDGE_LOOP ( 'NONE', ( #11722, #4832, #52423, #55489, #31991, #71519 ) ) ;
#28357=EDGE_CURVE ( 'NONE', #91269, #49746, #35445, .T. ) ;
#28359=DIRECTION ( 'NONE',  ( 0.000000000000000000, 0.000000000000000000, -1.000000000000000000 ) ) ;
#28363=EDGE_CURVE ( 'NONE', #75159, #90793, #28747, .T. ) ;
#28370=CARTESIAN_POINT ( 'NONE',  ( -10.76445796112991360, -3.815459910906994300E-15, 9.901260316209766543 ) ) ;
#28373=VECTOR ( 'NONE', #12872, 1000.000000000000114 ) ;
#28384=DIRECTION ( 'NONE',  ( 0.000000000000000000, 1.000000000000000000, 0.000000000000000000 ) ) ;
#28391=ORIENTED_EDGE ( 'NONE', *, *, #41225, .F. ) ;
#28399=CARTESIAN_POINT ( 'NONE',  ( 0.000000000000000000, 0.000000000000000000, 0.000000000000000000 ) ) ;
#28403=LINE ( 'NONE', #98413, #55472 ) ;
#28404=LINE ( 'NONE', #95425, #19591 ) ;
#28407=EDGE_CURVE ( 'NONE', #8981, #50127, #10981, .T. ) ;
#28413=ORIENTED_EDGE ( 'NONE', *, *, #97438, .T. ) ;
#28421=VERTEX_POINT ( 'NONE', #36585 ) ;
#28426=ORIENTED_EDGE ( 'NONE', *, *, #47526, .T. ) ;
#28436=DIRECTION ( 'NONE',  ( 0.2164396139380906914, 0.000000000000000000, 0.9762960071199361378 ) ) ;
#28441=VERTEX_POINT ( 'NONE', #65709 ) ;
#28443=CARTESIAN_POINT ( 'NONE',  ( -6.408140936763232709, -25.04303199673624292, 11.09922568453595026 ) ) ;
#28453=EDGE_CURVE ( 'NONE', #51651, #89050, #64714, .T. ) ;
#28455=B_SPLINE_CURVE_WITH_KNOTS ( 'NONE', 3,
 ( #10271, #28087, #51088, #93759, #88094, #65085 ),
 .UNSPECIFIED., .F., .F.,
 ( 4, 2, 4 ),
 ( 0.0002800267093036927718, 0.0006862322000113845692, 0.001092437690719076258 ),
 .UNSPECIFIED. ) ;
#28456=CARTESIAN_POINT ( 'NONE',  ( -10.64017930668218881, 14.49999999999999112, 10.57291749337211151 ) ) ;
#28457=EDGE_CURVE ( 'NONE', #18519, #74674, #60035, .T. ) ;
#28458=ORIENTED_EDGE ( 'NONE', *, *, #66199, .T. ) ;
#28463=ORIENTED_EDGE ( 'NONE', *, *, #92676, .T. ) ;
#28477=ADVANCED_FACE ( 'NONE', ( #73209 ), #41554, .T. ) ;
#28481=CARTESIAN_POINT ( 'NONE',  ( 11.62719953690058361, 0.5000000000000004441, 9.476720473301874392 ) ) ;
#28497=CARTESIAN_POINT ( 'NONE',  ( 0.000000000000000000, 14.49999999999999822, 0.000000000000000000 ) ) ;
#28500=CARTESIAN_POINT ( 'NONE',  ( -7.082119434687058401, -19.02958449841936428, -12.26659068614894110 ) ) ;
#28504=VERTEX_POINT ( 'NONE', #6212 ) ;
#28510=FACE_OUTER_BOUND ( 'NONE', #93710, .T. ) ;
#28515=CARTESIAN_POINT ( 'NONE',  ( -5.204170427930421283E-15, 26.81368534415484817, -10.88017736071110342 ) ) ;
#28528=DIRECTION ( 'NONE',  ( -0.6225146366376237417, 0.000000000000000000, 0.7826081568524104748 ) ) ;
#28536=CARTESIAN_POINT ( 'NONE',  ( 13.34343830728399283, 15.00000000000000000, 6.852200678592689442 ) ) ;
#28540=CIRCLE ( 'NONE', #79634, 15.00000000000000000 ) ;
#28542=DIRECTION ( 'NONE',  ( -0.6087614290087131064, 0.000000000000000000, -0.7933533402912409382 ) ) ;
#28548=ORIENTED_EDGE ( 'NONE', *, *, #83671, .T. ) ;
#28552=CARTESIAN_POINT ( 'NONE',  ( 4.180366052176858638, 15.00000000000000711, -14.01545757926328584 ) ) ;
#28560=CARTESIAN_POINT ( 'NONE',  ( 2.638427012816835227, 22.46726448433412315, 9.846743663894590881 ) ) ;
#28563=EDGE_CURVE ( 'NONE', #92892, #52439, #77915, .T. ) ;
#28564=ORIENTED_EDGE ( 'NONE', *, *, #93242, .T. ) ;
#28572=EDGE_CURVE ( 'NONE', #44777, #1179, #28540, .T. ) ;
#28575=EDGE_LOOP ( 'NONE', ( #28614, #87497, #68562, #81339 ) ) ;
#28578=ORIENTED_EDGE ( 'NONE', *, *, #9865, .T. ) ;
#28583=CIRCLE ( 'NONE', #55779, 14.49999999999999822 ) ;
#28588=CIRCLE ( 'NONE', #84492, 14.49999999999999822 ) ;
#28591=EDGE_LOOP ( 'NONE', ( #14742, #97207, #21806, #48206 ) ) ;
#28594=EDGE_CURVE ( 'NONE', #21190, #15328, #97732, .T. ) ;
#28596=VERTEX_POINT ( 'NONE', #74191 ) ;
#28601=PLANE ( 'NONE',  #40304 ) ;
#28603=CARTESIAN_POINT ( 'NONE',  ( -8.731067818237029599, 5.313309369127510173, 8.731067818237042033 ) ) ;
#28605=LINE ( 'NONE', #90088, #25951 ) ;
#28611=ADVANCED_FACE ( 'NONE', ( #5724 ), #13709, .T. ) ;
#28612=CARTESIAN_POINT ( 'NONE',  ( -6.382347221874519860, 0.3640475087720974057, 13.57444820018223908 ) ) ;
#28613=B_SPLINE_CURVE_WITH_KNOTS ( 'NONE', 3,
 ( #62460, #84497, #1010, #536, #38507, #24496 ),
 .UNSPECIFIED., .F., .F.,
 ( 4, 2, 4 ),
 ( 0.0002800760588349493702, 0.0006862820326512249040, 0.001092488006467500329 ),
 .UNSPECIFIED. ) ;
#28614=ORIENTED_EDGE ( 'NONE', *, *, #30245, .T. ) ;
#28622=DIRECTION ( 'NONE',  ( 0.6755902076156493630, 0.000000000000000000, 0.7372773368101340763 ) ) ;
#28623=DIRECTION ( 'NONE',  ( 0.9890158633619168249, -0.000000000000000000, 0.1478094111296113511 ) ) ;
#28626=CARTESIAN_POINT ( 'NONE',  ( -10.88017736071110342, -26.93631465584515894, 3.903127820947815962E-15 ) ) ;
#28630=LINE ( 'NONE', #97651, #6499 ) ;
#28631=CARTESIAN_POINT ( 'NONE',  ( 14.35840480524206697, 14.49999999999999112, -4.340070442838847242 ) ) ;
#28650=CARTESIAN_POINT ( 'NONE',  ( 8.606322355898619492, 15.00000000000000000, -11.66967075399251996 ) ) ;
#28652=ADVANCED_FACE ( 'NONE', ( #74702 ), #21718, .T. ) ;
#28653=ORIENTED_EDGE ( 'NONE', *, *, #91547, .T. ) ;
#28654=CARTESIAN_POINT ( 'NONE',  ( -6.689969769698787871, -0.03417435944610275333, -12.58200319823979285 ) ) ;
#28656=ORIENTED_EDGE ( 'NONE', *, *, #43887, .T. ) ;
#28658=CARTESIAN_POINT ( 'NONE',  ( -14.88232117145528655, 0.5000000000000004441, -1.875237731503337946 ) ) ;
#28674=CARTESIAN_POINT ( 'NONE',  ( -4.923371831947292776, -18.15773551566587685, 8.527530157486181039 ) ) ;
#28675=ORIENTED_EDGE ( 'NONE', *, *, #17613, .T. ) ;
#28676=DIRECTION ( 'NONE',  ( -0.000000000000000000, -1.000000000000000000, -0.000000000000000000 ) ) ;
#28681=DIRECTION ( 'NONE',  ( 0.000000000000000000, 0.000000000000000000, 1.000000000000000000 ) ) ;
#28682=CARTESIAN_POINT ( 'NONE',  ( 6.767445849361153343, 0.5000000000000004441, 13.38662304974501360 ) ) ;
#28687=CARTESIAN_POINT ( 'NONE',  ( 3.434112377981054287, 7.665301336597081239, -12.81628187352647608 ) ) ;
#28689=ORIENTED_EDGE ( 'NONE', *, *, #61551, .F. ) ;
#28698=DIRECTION ( 'NONE',  ( 0.1132032137679171296, 0.000000000000000000, -0.9935718556765862353 ) ) ;
#28704=CARTESIAN_POINT ( 'NONE',  ( -12.60874940350938189, 3.923185800807110140E-16, -7.160268045227207168 ) ) ;
#28706=EDGE_CURVE ( 'NONE', #83059, #75159, #32579, .T. ) ;
#28707=CARTESIAN_POINT ( 'NONE',  ( -12.80781515976305762, 15.00000000000000000, -6.246788841744501219 ) ) ;
#28733=DIRECTION ( 'NONE',  ( 0.000000000000000000, 1.000000000000000000, 0.000000000000000000 ) ) ;
#28737=DIRECTION ( 'NONE',  ( 0.000000000000000000, 0.000000000000000000, 1.000000000000000000 ) ) ;
#28741=CARTESIAN_POINT ( 'NONE',  ( -14.16423886937410082, 6.803748834913976751, 4.336808689942017736E-15 ) ) ;
#28746=DIRECTION ( 'NONE',  ( -4.085620730620576069E-14, 0.000000000000000000, 1.000000000000000000 ) ) ;
#28747=CIRCLE ( 'NONE', #23992, 15.00000000000000000 ) ;
#28751=VERTEX_POINT ( 'NONE', #706 ) ;
#28754=DIRECTION ( 'NONE',  ( -0.4146932426562403573, 0.000000000000000000, 0.9099612708765426605 ) ) ;
#28763=CARTESIAN_POINT ( 'NONE',  ( -14.82269085861174140, 14.63606914776923418, 2.299529454046852273 ) ) ;
#28767=DIRECTION ( 'NONE',  ( 0.1305261922200514901, 0.000000000000000000, 0.9914448613738104932 ) ) ;
#28772=EDGE_CURVE ( 'NONE', #1179, #21240, #53673, .T. ) ;
#28790=ORIENTED_EDGE ( 'NONE', *, *, #21764, .T. ) ;
#28793=ORIENTED_EDGE ( 'NONE', *, *, #64138, .T. ) ;
#28796=ORIENTED_EDGE ( 'NONE', *, *, #25263, .T. ) ;
#28797=VECTOR ( 'NONE', #11189, 1000.000000000000000 ) ;
#28799=EDGE_CURVE ( 'NONE', #60724, #55655, #43383, .T. ) ;
#28800=EDGE_CURVE ( 'NONE', #87709, #14505, #12274, .T. ) ;
#28801=ORIENTED_EDGE ( 'NONE', *, *, #26710, .F. ) ;
#28805=ORIENTED_EDGE ( 'NONE', *, *, #60675, .F. ) ;
#28806=AXIS2_PLACEMENT_3D ( 'NONE', #93466, #32953, #79933 ) ;
#28808=VERTEX_POINT ( 'NONE', #1195 ) ;
#28812=CARTESIAN_POINT ( 'NONE',  ( -12.98685442714202232, 15.00000000000000000, 6.449155920600843750 ) ) ;
#28824=LINE ( 'NONE', #66331, #37257 ) ;
#28830=CARTESIAN_POINT ( 'NONE',  ( -11.39601241150444189, -0.03417435944610275333, -11.22534175661882294 ) ) ;
#28832=VERTEX_POINT ( 'NONE', #15699 ) ;
#28836=CARTESIAN_POINT ( 'NONE',  ( 11.25000000000000000, 7.409700295649311208, 3.014428414850128135 ) ) ;
#28846=CARTESIAN_POINT ( 'NONE',  ( 0.000000000000000000, 0.5000000000000004441, 0.000000000000000000 ) ) ;
#28852=CARTESIAN_POINT ( 'NONE',  ( 10.69820648722788015, 1.823139558123380688, 5.272416709312279792 ) ) ;
#28855=CIRCLE ( 'NONE', #86339, 15.00000000000000000 ) ;
#28857=FACE_OUTER_BOUND ( 'NONE', #78849, .T. ) ;
#28858=ORIENTED_EDGE ( 'NONE', *, *, #51717, .T. ) ;
#28861=CARTESIAN_POINT ( 'NONE',  ( -3.927832320392065313, -0.03417435944610275333, -13.69797916712109398 ) ) ;
#28880=DIRECTION ( 'NONE',  ( 0.9862856015372331031, 0.000000000000000000, -0.1650476058606676344 ) ) ;
#28883=EDGE_CURVE ( 'NONE', #9875, #31048, #28263, .T. ) ;
#28898=ORIENTED_EDGE ( 'NONE', *, *, #51816, .T. ) ;
#28910=EDGE_CURVE ( 'NONE', #54024, #27786, #41060, .T. ) ;
#28914=DIRECTION ( 'NONE',  ( 0.000000000000000000, 0.000000000000000000, 1.000000000000000000 ) ) ;
#28916=CARTESIAN_POINT ( 'NONE',  ( 8.564643372776545860, 14.63606914147656646, 12.31449893000750428 ) ) ;
#28922=CARTESIAN_POINT ( 'NONE',  ( 6.408140936763236262, -12.54303199673624469, -11.09922568453595026 ) ) ;
#28930=AXIS2_PLACEMENT_3D ( 'NONE', #92955, #16983, #62954 ) ;
#28931=FACE_OUTER_BOUND ( 'NONE', #42415, .T. ) ;
#28932=VERTEX_POINT ( 'NONE', #39179 ) ;
#28936=AXIS2_PLACEMENT_3D ( 'NONE', #62461, #46975, #92964 ) ;
#28937=DIRECTION ( 'NONE',  ( 0.000000000000000000, 1.000000000000000000, 0.000000000000000000 ) ) ;
#28940=CARTESIAN_POINT ( 'NONE',  ( -12.60589901313227124, 0.5000000000000004441, 8.129656208641961257 ) ) ;
#28942=AXIS2_PLACEMENT_3D ( 'NONE', #39626, #8622, #39132 ) ;
#28950=DIRECTION ( 'NONE',  ( -0.000000000000000000, -1.000000000000000000, -0.000000000000000000 ) ) ;
#28955=CARTESIAN_POINT ( 'NONE',  ( 0.1552420861328543400, -3.159856409732166232E-15, 14.62478754979302842 ) ) ;
#28968=ORIENTED_EDGE ( 'NONE', *, *, #24656, .T. ) ;
#28978=CARTESIAN_POINT ( 'NONE',  ( -14.16423886937409726, -17.98791783175269643, 3.795296366450320757 ) ) ;
#28982=ORIENTED_EDGE ( 'NONE', *, *, #39699, .F. ) ;
#28984=CARTESIAN_POINT ( 'NONE',  ( 10.82361996478181432, 14.95037106895532020, 10.02529603627583121 ) ) ;
#28987=DIRECTION ( 'NONE',  ( 0.9588197348681928300, 0.000000000000000000, 0.2840153447039234780 ) ) ;
#28989=CARTESIAN_POINT ( 'NONE',  ( -2.915334737309934532, 32.02201867748817676, -10.88017736071109987 ) ) ;
#28995=EDGE_LOOP ( 'NONE', ( #84560, #23188, #90586, #30784 ) ) ;
#28997=EDGE_CURVE ( 'NONE', #60588, #7347, #98054, .T. ) ;
#29007=CARTESIAN_POINT ( 'NONE',  ( 11.92686044187656691, 10.16212336850781028, -2.602085213965210642E-15 ) ) ;
#29011=ORIENTED_EDGE ( 'NONE', *, *, #98083, .T. ) ;
#29016=DIRECTION ( 'NONE',  ( 0.000000000000000000, 1.000000000000000000, 0.000000000000000000 ) ) ;
#29023=EDGE_CURVE ( 'NONE', #11086, #44839, #51590, .T. ) ;
#29024=DIRECTION ( 'NONE',  ( 0.000000000000000000, 0.000000000000000000, -1.000000000000000000 ) ) ;
#29027=VERTEX_POINT ( 'NONE', #57 ) ;
#29041=DIRECTION ( 'NONE',  ( -0.000000000000000000, -1.000000000000000000, -0.000000000000000000 ) ) ;
#29042=CARTESIAN_POINT ( 'NONE',  ( -7.208316651077764980, 10.38393115100079100, -7.208316651077759651 ) ) ;
#29043=VERTEX_POINT ( 'NONE', #6051 ) ;
#29045=EDGE_LOOP ( 'NONE', ( #49812, #56430, #39875, #31536, #64427, #10433 ) ) ;
#29053=B_SPLINE_CURVE_WITH_KNOTS ( 'NONE', 3,
 ( #95459, #3485, #88443, #50437, #71961, #87943 ),
 .UNSPECIFIED., .F., .F.,
 ( 4, 2, 4 ),
 ( 3.409110551494651432E-05, 0.0004400426677367951910, 0.0008459942299586437932 ),
 .UNSPECIFIED. ) ;
#29055=CIRCLE ( 'NONE', #1965, 14.49999999999999822 ) ;
#29058=ORIENTED_EDGE ( 'NONE', *, *, #85472, .T. ) ;
#29061=ORIENTED_EDGE ( 'NONE', *, *, #64702, .F. ) ;
#29067=DIRECTION ( 'NONE',  ( 0.6494480483301745544, 0.000000000000000000, 0.7604059656000387024 ) ) ;
#29072=VECTOR ( 'NONE', #441, 1000.000000000000114 ) ;
#29077=CARTESIAN_POINT ( 'NONE',  ( 4.850115630859590965, 0.04922511925147064066, 13.93278430610810936 ) ) ;
#29080=AXIS2_PLACEMENT_3D ( 'NONE', #42095, #59046, #13053 ) ;
#29082=DIRECTION ( 'NONE',  ( 0.000000000000000000, 0.000000000000000000, 1.000000000000000000 ) ) ;
#29087=EDGE_LOOP ( 'NONE', ( #13161, #37588, #2003, #54058 ) ) ;
#29088=CARTESIAN_POINT ( 'NONE',  ( -11.92686044187656691, 4.479976035794177136, -3.195792623639521324 ) ) ;
#29090=DIRECTION ( 'NONE',  ( 0.000000000000000000, 1.000000000000000000, 0.000000000000000000 ) ) ;
#29098=ORIENTED_EDGE ( 'NONE', *, *, #62557, .F. ) ;
#29107=DIRECTION ( 'NONE',  ( 0.7253743710122867450, 0.000000000000000000, -0.6883545756937550220 ) ) ;
#29110=CARTESIAN_POINT ( 'NONE',  ( -7.964842623401172439, -11.31131465584515361, 7.964842623401183097 ) ) ;
#29112=CARTESIAN_POINT ( 'NONE',  ( 4.431036607602467647, 14.49999999999999822, 14.33059365769914351 ) ) ;
#29114=CARTESIAN_POINT ( 'NONE',  ( -13.40508947812168827, 15.00000000000000000, 5.527528931045992522 ) ) ;
#29118=TOROIDAL_SURFACE ( 'NONE', #88217, 14.49999999999999822, 0.5000000000000000000 ) ;
#29120=LINE ( 'NONE', #53602, #4225 ) ;
#29122=EDGE_CURVE ( 'NONE', #10914, #59056, #5115, .T. ) ;
#29123=ADVANCED_FACE ( 'NONE', ( #7037 ), #67039, .T. ) ;
#29136=CARTESIAN_POINT ( 'NONE',  ( 0.000000000000000000, 15.00000000000000000, 0.000000000000000000 ) ) ;
#29139=CARTESIAN_POINT ( 'NONE',  ( -14.76100041229768856, 14.76930270348881002, -2.313205896731025391 ) ) ;
#29142=ORIENTED_EDGE ( 'NONE', *, *, #82411, .T. ) ;
#29158=EDGE_CURVE ( 'NONE', #10376, #14429, #90026, .T. ) ;
#29159=CIRCLE ( 'NONE', #81821, 14.49999999999999822 ) ;
#29160=CARTESIAN_POINT ( 'NONE',  ( 2.638427012816835227, -27.53273551566587329, 9.846743663894590881 ) ) ;
#29161=ORIENTED_EDGE ( 'NONE', *, *, #95830, .T. ) ;
#29172=CARTESIAN_POINT ( 'NONE',  ( 3.836325488036083087, 0.5000000000000004441, 14.50112432709425114 ) ) ;
#29173=DIRECTION ( 'NONE',  ( -0.000000000000000000, -1.000000000000000000, -0.000000000000000000 ) ) ;
#29175=TOROIDAL_SURFACE ( 'NONE', #52929, 14.49999999999999822, 0.5000000000000000000 ) ;
#29177=CARTESIAN_POINT ( 'NONE',  ( -9.382169495545422677, 23.49863466993043204, -9.382169495545417348 ) ) ;
#29178=VERTEX_POINT ( 'NONE', #22048 ) ;
#29188=DIRECTION ( 'NONE',  ( 0.000000000000000000, 1.000000000000000000, 0.000000000000000000 ) ) ;
#29191=CARTESIAN_POINT ( 'NONE',  ( -3.836325488036279818, 14.49999999999999822, 14.50112432709419963 ) ) ;
#29193=CARTESIAN_POINT ( 'NONE',  ( -3.753761956877497585, 0.000000000000000000, 3.955639745193215706 ) ) ;
#29199=DIRECTION ( 'NONE',  ( 0.000000000000000000, 1.000000000000000000, 0.000000000000000000 ) ) ;
#29200=ORIENTED_EDGE ( 'NONE', *, *, #24417, .T. ) ;
#29207=CARTESIAN_POINT ( 'NONE',  ( -4.096035146099030300, 15.00000000000000000, 13.90943910019935714 ) ) ;
#29210=CARTESIAN_POINT ( 'NONE',  ( -10.93781366033333313, 0.3640475087720989600, -10.26470809774081339 ) ) ;
#29211=EDGE_CURVE ( 'NONE', #60175, #25131, #96965, .T. ) ;
#29215=DIRECTION ( 'NONE',  ( -0.5075383629607084224, 0.000000000000000000, 0.8616291604415232674 ) ) ;
#29217=VECTOR ( 'NONE', #53194, 1000.000000000000114 ) ;
#29220=CARTESIAN_POINT ( 'NONE',  ( -8.235571585149871865, 4.493033628982647798, -8.235571585149866536 ) ) ;
#29230=CARTESIAN_POINT ( 'NONE',  ( -1.847340224724952629, 14.95077488074853456, 14.63671528203489558 ) ) ;
#29232=CARTESIAN_POINT ( 'NONE',  ( -7.082119434687044190, 17.63708216824730357, 12.26659068614894998 ) ) ;
#29234=EDGE_CURVE ( 'NONE', #50106, #57707, #5564, .T. ) ;
#29247=CARTESIAN_POINT ( 'NONE',  ( 0.000000000000000000, 0.5000000000000004441, 0.000000000000000000 ) ) ;
#29260=CARTESIAN_POINT ( 'NONE',  ( -12.25993886608611660, 0.5000000000000004441, 8.642563219313529999 ) ) ;
#29266=AXIS2_PLACEMENT_3D ( 'NONE', #19162, #58124, #72153 ) ;
#29277=CARTESIAN_POINT ( 'NONE',  ( -14.35840480524209894, 14.49999999999999112, 4.340070442838745102 ) ) ;
#29282=EDGE_CURVE ( 'NONE', #48771, #17080, #31398, .T. ) ;
#29291=ORIENTED_EDGE ( 'NONE', *, *, #91840, .F. ) ;
#29293=VECTOR ( 'NONE', #89877, 1000.000000000000000 ) ;
#29294=AXIS2_PLACEMENT_3D ( 'NONE', #41158, #71154, #86647 ) ;
#29303=CARTESIAN_POINT ( 'NONE',  ( 2.393480905993186969, 14.49999999999999112, -14.80781041047757185 ) ) ;
#29305=FACE_OUTER_BOUND ( 'NONE', #3751, .T. ) ;
#29308=VERTEX_POINT ( 'NONE', #31972 ) ;
#29315=CARTESIAN_POINT ( 'NONE',  ( 15.96747533562963639, -0.03417435944610275333, -0.9576679184940652956 ) ) ;
#29323=EDGE_CURVE ( 'NONE', #97221, #27349, #23531, .T. ) ;
#29326=VERTEX_POINT ( 'NONE', #2015 ) ;
#29328=CARTESIAN_POINT ( 'NONE',  ( -5.204170427930421283E-15, 6.412123368507812948, -11.92686044187656513 ) ) ;
#29337=CARTESIAN_POINT ( 'NONE',  ( 0.000000000000000000, 14.49999999999999822, 0.000000000000000000 ) ) ;
#29345=ORIENTED_EDGE ( 'NONE', *, *, #87540, .F. ) ;
#29346=DIRECTION ( 'NONE',  ( -0.8870108331782183830, 0.000000000000000000, -0.4617486132350405170 ) ) ;
#29353=CARTESIAN_POINT ( 'NONE',  ( 14.35840480524206697, 14.49999999999999112, -4.340070442838847242 ) ) ;
#29358=CARTESIAN_POINT ( 'NONE',  ( -2.361121941888906672, 0.2301505397289878574, -14.75287579053852660 ) ) ;
#29378=CARTESIAN_POINT ( 'NONE',  ( -3.420591144908359027, 14.63595249122788999, -14.60477854057961800 ) ) ;
#29382=DIRECTION ( 'NONE',  ( 0.000000000000000000, 1.000000000000000000, 0.000000000000000000 ) ) ;
#29401=ORIENTED_EDGE ( 'NONE', *, *, #9740, .T. ) ;
#29413=CARTESIAN_POINT ( 'NONE',  ( 12.81628187352647608, -18.37636533006957507, -2.602085213965210642E-15 ) ) ;
#29424=PLANE ( 'NONE',  #72231 ) ;
#29429=DIRECTION ( 'NONE',  ( 0.9969173337331278528, -0.000000000000000000, 0.07845909572784538766 ) ) ;
#29442=ORIENTED_EDGE ( 'NONE', *, *, #84593, .F. ) ;
#29461=VECTOR ( 'NONE', #45666, 1000.000000000000114 ) ;
#29465=CARTESIAN_POINT ( 'NONE',  ( -5.204170427930421283E-15, -19.44625116508602503, -14.16423886937410082 ) ) ;
#29469=ADVANCED_FACE ( 'NONE', ( #70966 ), #95424, .F. ) ;
#29470=ORIENTED_EDGE ( 'NONE', *, *, #46893, .T. ) ;
#29472=CARTESIAN_POINT ( 'NONE',  ( 10.93781366033342017, 14.63606902047321334, 10.26470809774076187 ) ) ;
#29478=CARTESIAN_POINT ( 'NONE',  ( 2.915334737309928315, 24.52201867748817676, 10.88017736071109987 ) ) ;
#29485=EDGE_LOOP ( 'NONE', ( #89752, #16624, #86138, #91933 ) ) ;
#29492=VECTOR ( 'NONE', #50386, 1000.000000000000000 ) ;
#29504=DIRECTION ( 'NONE',  ( 0.1478094111296180124, 0.000000000000000000, -0.9890158633619157147 ) ) ;
#29505=CARTESIAN_POINT ( 'NONE',  ( 0.000000000000000000, 0.000000000000000000, 0.000000000000000000 ) ) ;
#29507=EDGE_CURVE ( 'NONE', #58863, #27610, #48441, .T. ) ;
#29511=EDGE_CURVE ( 'NONE', #17634, #54629, #21864, .T. ) ;
#29514=ORIENTED_EDGE ( 'NONE', *, *, #73348, .F. ) ;
#29520=CARTESIAN_POINT ( 'NONE',  ( -4.431036607602414357, 14.49999999999999112, -14.33059365769922167 ) ) ;
#29521=CARTESIAN_POINT ( 'NONE',  ( 2.120353041430647512, 4.078855811979330250E-16, -14.34413130794945523 ) ) ;
#29526=CARTESIAN_POINT ( 'NONE',  ( 0.000000000000000000, 0.000000000000000000, 0.000000000000000000 ) ) ;
#29530=CARTESIAN_POINT ( 'NONE',  ( -1.180296924652843193, 0.000000000000000000, -5.323975374878068934 ) ) ;
#29531=CARTESIAN_POINT ( 'NONE',  ( -7.208316651077764980, 20.38393115100079100, -7.208316651077759651 ) ) ;
#29533=ORIENTED_EDGE ( 'NONE', *, *, #31434, .T. ) ;
#29535=ORIENTED_EDGE ( 'NONE', *, *, #87540, .T. ) ;
#29544=VERTEX_POINT ( 'NONE', #80427 ) ;
#29550=ORIENTED_EDGE ( 'NONE', *, *, #8025, .F. ) ;
#29561=ORIENTED_EDGE ( 'NONE', *, *, #37719, .F. ) ;
#29563=EDGE_CURVE ( 'NONE', #90631, #79877, #90367, .T. ) ;
#29567=DIRECTION ( 'NONE',  ( 0.000000000000000000, 1.000000000000000000, 0.000000000000000000 ) ) ;
#29571=ORIENTED_EDGE ( 'NONE', *, *, #29507, .F. ) ;
#29572=FACE_OUTER_BOUND ( 'NONE', #47853, .T. ) ;
#29580=AXIS2_PLACEMENT_3D ( 'NONE', #69724, #61708, #1250 ) ;
#29582=VERTEX_POINT ( 'NONE', #59382 ) ;
#29589=DIRECTION ( 'NONE',  ( 0.6626200482157461602, 0.000000000000000000, -0.7489557207889945278 ) ) ;
#29591=EDGE_CURVE ( 'NONE', #78512, #59678, #10784, .T. ) ;
#29592=DIRECTION ( 'NONE',  ( -0.000000000000000000, -1.000000000000000000, -0.000000000000000000 ) ) ;
#29593=CARTESIAN_POINT ( 'NONE',  ( 13.07661834287964986, 14.99999999999796252, 6.550615570657222442 ) ) ;
#29597=CARTESIAN_POINT ( 'NONE',  ( 10.88017736071110519, -14.43631465584515539, -2.602085213965210642E-15 ) ) ;
#29602=CARTESIAN_POINT ( 'NONE',  ( 0.000000000000000000, 0.000000000000000000, 0.000000000000000000 ) ) ;
#29608=CARTESIAN_POINT ( 'NONE',  ( -6.898461952320262824, 4.061641280801676772E-16, -12.75387089053318590 ) ) ;
#29613=EDGE_LOOP ( 'NONE', ( #59506, #55610, #30032, #77907, #53625, #16773 ) ) ;
#29623=EDGE_CURVE ( 'NONE', #5095, #42806, #68350, .T. ) ;
#29624=ORIENTED_EDGE ( 'NONE', *, *, #60493, .T. ) ;
#29625=LINE ( 'NONE', #90135, #27379 ) ;
#29645=CARTESIAN_POINT ( 'NONE',  ( 9.846743663894590881, -26.28273551566587685, -2.638427012816833894 ) ) ;
#29647=CARTESIAN_POINT ( 'NONE',  ( 0.000000000000000000, 15.00000000000000000, 0.000000000000000000 ) ) ;
#29650=ORIENTED_EDGE ( 'NONE', *, *, #79964, .F. ) ;
#29660=B_SPLINE_CURVE_WITH_KNOTS ( 'NONE', 3,
 ( #19786, #27778, #58263, #89274, #88778, #57780 ),
 .UNSPECIFIED., .F., .F.,
 ( 4, 2, 4 ),
 ( 0.0002800124554209686796, 0.0006862178066679820113, 0.001092423157914995235 ),
 .UNSPECIFIED. ) ;
#29661=CARTESIAN_POINT ( 'NONE',  ( 6.408140936763243367, 15.79030133659708923, 11.09922568453594494 ) ) ;
#29663=EDGE_CURVE ( 'NONE', #38633, #74198, #28403, .T. ) ;
#29672=FACE_OUTER_BOUND ( 'NONE', #68405, .T. ) ;
#29680=LINE ( 'NONE', #90685, #56216 ) ;
#29685=EDGE_CURVE ( 'NONE', #97713, #67262, #43883, .T. ) ;
#29686=CARTESIAN_POINT ( 'NONE',  ( 6.767445849361157784, 14.63606917768312954, 13.38662304974505624 ) ) ;
#29688=ORIENTED_EDGE ( 'NONE', *, *, #66504, .F. ) ;
#29703=DIRECTION ( 'NONE',  ( 0.000000000000000000, 0.000000000000000000, 1.000000000000000000 ) ) ;
#29705=EDGE_CURVE ( 'NONE', #50542, #16647, #74229, .T. ) ;
#29707=CIRCLE ( 'NONE', #80830, 14.49999999999999822 ) ;
#29716=CARTESIAN_POINT ( 'NONE',  ( 13.50171220565083807, 15.00000000000000711, 5.622479820943917517 ) ) ;
#29722=CARTESIAN_POINT ( 'NONE',  ( -3.795296366450322534, 25.76208216824730357, -14.16423886937409904 ) ) ;
#29729=ORIENTED_EDGE ( 'NONE', *, *, #24423, .T. ) ;
#29738=ORIENTED_EDGE ( 'NONE', *, *, #40260, .F. ) ;
#29741=FACE_OUTER_BOUND ( 'NONE', #68298, .T. ) ;
#29752=AXIS2_PLACEMENT_3D ( 'NONE', #11062, #72050, #3579 ) ;
#29754=ORIENTED_EDGE ( 'NONE', *, *, #55694, .T. ) ;
#29771=ORIENTED_EDGE ( 'NONE', *, *, #543, .T. ) ;
#29785=VERTEX_POINT ( 'NONE', #82380 ) ;
#29787=DIRECTION ( 'NONE',  ( 0.000000000000000000, 1.000000000000000000, 0.000000000000000000 ) ) ;
#29791=CARTESIAN_POINT ( 'NONE',  ( 0.000000000000000000, 15.00000000000000000, 0.000000000000000000 ) ) ;
#29792=EDGE_CURVE ( 'NONE', #16296, #13218, #49036, .T. ) ;
#29798=EDGE_CURVE ( 'NONE', #38777, #5117, #82716, .T. ) ;
#29802=CARTESIAN_POINT ( 'NONE',  ( -15.33206046421386759, 15.00000000000000000, -4.561284726668966449 ) ) ;
#29807=FACE_OUTER_BOUND ( 'NONE', #90283, .T. ) ;
#29813=FACE_OUTER_BOUND ( 'NONE', #39291, .T. ) ;
#29834=CARTESIAN_POINT ( 'NONE',  ( 12.07856007377828078, 4.686601975994315497E-16, -8.022367888854837759 ) ) ;
#29841=DIRECTION ( 'NONE',  ( -0.000000000000000000, -1.000000000000000000, -0.000000000000000000 ) ) ;
#29842=EDGE_CURVE ( 'NONE', #62099, #50486, #14739, .T. ) ;
#29852=FACE_OUTER_BOUND ( 'NONE', #60650, .T. ) ;
#29869=CARTESIAN_POINT ( 'NONE',  ( -5.810213597521888040, 0.04962897357397404868, 13.56092647078866875 ) ) ;
#29870=LINE ( 'NONE', #52875, #70704 ) ;
#29881=CARTESIAN_POINT ( 'NONE',  ( -5.418184704451235234, 0.000000000000000000, -0.6173241701923803948 ) ) ;
#29887=EDGE_CURVE ( 'NONE', #3919, #5292, #77938, .T. ) ;
#29898=DIRECTION ( 'NONE',  ( 0.2840153447039300283, 0.000000000000000000, -0.9588197348681908316 ) ) ;
#29899=DIRECTION ( 'NONE',  ( 0.000000000000000000, 0.000000000000000000, 1.000000000000000000 ) ) ;
#29907=ORIENTED_EDGE ( 'NONE', *, *, #49448, .F. ) ;
#29909=CARTESIAN_POINT ( 'NONE',  ( -12.81628187352647608, -20.87636533006957507, 3.903127820947815962E-15 ) ) ;
#29917=ADVANCED_FACE ( 'NONE', ( #16365 ), #46846, .F. ) ;
#29919=ORIENTED_EDGE ( 'NONE', *, *, #22377, .T. ) ;
#29925=ORIENTED_EDGE ( 'NONE', *, *, #50734, .F. ) ;
#29931=CARTESIAN_POINT ( 'NONE',  ( 13.78891971893209245, 14.49999999999999112, 5.904717858191670388 ) ) ;
#29935=VECTOR ( 'NONE', #80368, 1000.000000000000114 ) ;
#29939=EDGE_LOOP ( 'NONE', ( #20352, #75176, #64369, #39920 ) ) ;
#29941=CARTESIAN_POINT ( 'NONE',  ( 2.815433093577117685, 0.3639308411966863388, -14.73340885523753307 ) ) ;
#29954=CARTESIAN_POINT ( 'NONE',  ( -11.25000000000000000, 10.32636696231598172, 3.014428414850140570 ) ) ;
#29961=CARTESIAN_POINT ( 'NONE',  ( -9.399392868737642459, 15.00000000000000000, -11.04089732309485861 ) ) ;
#29964=CARTESIAN_POINT ( 'NONE',  ( 7.082119434687047743, -19.86291783175269643, -12.26659068614894821 ) ) ;
#29970=B_SPLINE_CURVE_WITH_KNOTS ( 'NONE', 3,
 ( #49278, #87761, #11277, #50765, #12753, #26277 ),
 .UNSPECIFIED., .F., .F.,
 ( 4, 2, 4 ),
 ( 3.409110551326300585E-05, 0.0004400426677350938610, 0.0008459942299569247906 ),
 .UNSPECIFIED. ) ;
#29975=DIRECTION ( 'NONE',  ( 0.000000000000000000, 0.000000000000000000, 1.000000000000000000 ) ) ;
#29981=CARTESIAN_POINT ( 'NONE',  ( -5.204170427930421283E-15, 31.81368534415485172, -10.88017736071110342 ) ) ;
#29987=ORIENTED_EDGE ( 'NONE', *, *, #46442, .T. ) ;
#29996=CYLINDRICAL_SURFACE ( 'NONE', #92686, 15.00000000000000000 ) ;
#29997=CARTESIAN_POINT ( 'NONE',  ( 0.000000000000000000, 15.00000000000000000, 0.000000000000000000 ) ) ;
#30003=CARTESIAN_POINT ( 'NONE',  ( 0.000000000000000000, 14.49999999999999822, 0.000000000000000000 ) ) ;
#30010=CARTESIAN_POINT ( 'NONE',  ( 12.25993886608605443, 0.5000000000000004441, -8.642563219313617040 ) ) ;
#30016=ORIENTED_EDGE ( 'NONE', *, *, #88507, .T. ) ;
#30021=DIRECTION ( 'NONE',  ( -1.776356839400250780E-14, 0.000000000000000000, 1.000000000000000000 ) ) ;
#30026=DIRECTION ( 'NONE',  ( -0.6626200482157408311, 0.000000000000000000, 0.7489557207889990798 ) ) ;
#30028=CARTESIAN_POINT ( 'NONE',  ( -7.208316651077756099, 11.63393115100078212, 7.208316651077766757 ) ) ;
#30029=ORIENTED_EDGE ( 'NONE', *, *, #45642, .F. ) ;
#30031=CARTESIAN_POINT ( 'NONE',  ( 1.354709868695638697, 14.63606900606171557, -14.93870011653155316 ) ) ;
#30032=ORIENTED_EDGE ( 'NONE', *, *, #56947, .T. ) ;
#30043=ORIENTED_EDGE ( 'NONE', *, *, #19506, .F. ) ;
#30052=VECTOR ( 'NONE', #78818, 1000.000000000000000 ) ;
#30059=DIRECTION ( 'NONE',  ( -0.9832549075639539504, 0.000000000000000000, -0.1822355254921514123 ) ) ;
#30061=B_SPLINE_CURVE_WITH_KNOTS ( 'NONE', 3,
 ( #30594, #14645, #38610, #24105, #61099, #60608 ),
 .UNSPECIFIED., .F., .F.,
 ( 4, 2, 4 ),
 ( 0.0002800187770386834392, 0.0006862241901302594451, 0.001092429603221835559 ),
 .UNSPECIFIED. ) ;
#30077=VECTOR ( 'NONE', #52761, 1000.000000000000000 ) ;
#30081=VERTEX_POINT ( 'NONE', #25834 ) ;
#30088=CARTESIAN_POINT ( 'NONE',  ( 14.22901244993685843, 2.270048298641524909E-16, -3.387263120971315988 ) ) ;
#30094=CARTESIAN_POINT ( 'NONE',  ( 10.88017736071109987, -9.227981322511825013, -2.915334737309928315 ) ) ;
#30098=CARTESIAN_POINT ( 'NONE',  ( 13.07751017357376888, 15.00000000000000000, 6.263284095430594611 ) ) ;
#30109=CARTESIAN_POINT ( 'NONE',  ( 8.502721643904074256, 0.04962896249296737394, -12.05657636697101331 ) ) ;
#30113=CARTESIAN_POINT ( 'NONE',  ( -13.75801628063885040, 4.154966894009843400E-16, 4.578972376164368363 ) ) ;
#30120=DIRECTION ( 'NONE',  ( 0.000000000000000000, 1.000000000000000000, 0.000000000000000000 ) ) ;
#30121=EDGE_CURVE ( 'NONE', #83033, #26759, #23516, .T. ) ;
#30122=CARTESIAN_POINT ( 'NONE',  ( -14.56332774647470174, 14.95077488074853456, -2.357028871694378580 ) ) ;
#30139=CARTESIAN_POINT ( 'NONE',  ( -8.527530157486173934, -18.57440218233254470, 4.923371831947302546 ) ) ;
#30140=EDGE_LOOP ( 'NONE', ( #54614, #27567, #73065, #21767 ) ) ;
#30141=PLANE ( 'NONE',  #26794 ) ;
#30144=ORIENTED_EDGE ( 'NONE', *, *, #73617, .F. ) ;
#30154=EDGE_CURVE ( 'NONE', #86853, #40259, #37409, .T. ) ;
#30155=B_SPLINE_CURVE_WITH_KNOTS ( 'NONE', 3,
 ( #38870, #69361, #60366, #76848, #90361, #21899 ),
 .UNSPECIFIED., .F., .F.,
 ( 4, 2, 4 ),
 ( 3.409110551494643978E-05, 0.0004400426677367921553, 0.0008459942299586379385 ),
 .UNSPECIFIED. ) ;
#30156=CARTESIAN_POINT ( 'NONE',  ( -9.382169495545413795, 24.74863466993042493, 9.382169495545428006 ) ) ;
#30157=VERTEX_POINT ( 'NONE', #17838 ) ;
#30167=CARTESIAN_POINT ( 'NONE',  ( 13.34343830728399816, 0.3640475087720989045, 6.852200678592694771 ) ) ;
#30175=DIRECTION ( 'NONE',  ( 0.000000000000000000, 0.000000000000000000, 1.000000000000000000 ) ) ;
#30182=DIRECTION ( 'NONE',  ( -0.000000000000000000, -1.000000000000000000, -0.000000000000000000 ) ) ;
#30183=DIRECTION ( 'NONE',  ( 0.000000000000000000, 0.000000000000000000, -1.000000000000000000 ) ) ;
#30191=CARTESIAN_POINT ( 'NONE',  ( -9.383795276901851778, 14.76930270348881002, 11.62679839395687864 ) ) ;
#30200=ORIENTED_EDGE ( 'NONE', *, *, #11057, .T. ) ;
#30201=CARTESIAN_POINT ( 'NONE',  ( 6.741983435833431848, 0.04922511925147219497, 13.12218577464092917 ) ) ;
#30206=DIRECTION ( 'NONE',  ( 0.000000000000000000, 0.000000000000000000, 1.000000000000000000 ) ) ;
#30212=DIRECTION ( 'NONE',  ( -0.1132032137678971873, 0.000000000000000000, -0.9935718556765885667 ) ) ;
#30213=CARTESIAN_POINT ( 'NONE',  ( -10.36894250292379205, 26.17874883491397497, -10.36894250292378672 ) ) ;
#30219=FACE_OUTER_BOUND ( 'NONE', #91059, .T. ) ;
#30220=ORIENTED_EDGE ( 'NONE', *, *, #96632, .F. ) ;
#30225=CARTESIAN_POINT ( 'NONE',  ( 14.29730467489529389, 15.00000000000000000, 2.416004766803322656 ) ) ;
#30230=VERTEX_POINT ( 'NONE', #16428 ) ;
#30233=CARTESIAN_POINT ( 'NONE',  ( -14.29730467490344736, 15.00000000000000000, 2.416004766801328696 ) ) ;
#30245=EDGE_CURVE ( 'NONE', #84144, #39231, #76242, .T. ) ;
#30255=EDGE_CURVE ( 'NONE', #42986, #98896, #1650, .T. ) ;
#30256=EDGE_CURVE ( 'NONE', #83033, #96742, #33369, .T. ) ;
#30264=CARTESIAN_POINT ( 'NONE',  ( -6.715867195167534831, 4.123781235506717606E-16, 12.85095824508322693 ) ) ;
#30281=ADVANCED_FACE ( 'NONE', ( #24921 ), #91924, .F. ) ;
#30286=FACE_OUTER_BOUND ( 'NONE', #89798, .T. ) ;
#30290=ORIENTED_EDGE ( 'NONE', *, *, #36622, .F. ) ;
#30291=B_SPLINE_CURVE_WITH_KNOTS ( 'NONE', 3,
 ( #77418, #14984, #60943, #69942, #84937, #45455 ),
 .UNSPECIFIED., .F., .F.,
 ( 4, 2, 4 ),
 ( 0.0002800039672440423157, 0.0006862092354666148638, 0.001092414503689187249 ),
 .UNSPECIFIED. ) ;
#30292=FACE_OUTER_BOUND ( 'NONE', #39680, .T. ) ;
#30301=DIRECTION ( 'NONE',  ( -4.884981308350689409E-14, 0.000000000000000000, 1.000000000000000000 ) ) ;
#30304=DIRECTION ( 'NONE',  ( 0.9099612708765483227, 0.000000000000000000, -0.4146932426562279228 ) ) ;
#30312=EDGE_CURVE ( 'NONE', #76776, #33114, #33823, .T. ) ;
#30316=CARTESIAN_POINT ( 'NONE',  ( -4.873787042390880231, -0.03417435944610275333, 13.39061984619915791 ) ) ;
#30320=ORIENTED_EDGE ( 'NONE', *, *, #79405, .F. ) ;
#30329=AXIS2_PLACEMENT_3D ( 'NONE', #35246, #72747, #28245 ) ;
#30348=ORIENTED_EDGE ( 'NONE', *, *, #25272, .F. ) ;
#30355=DIRECTION ( 'NONE',  ( -0.000000000000000000, -1.000000000000000000, -0.000000000000000000 ) ) ;
#30362=EDGE_CURVE ( 'NONE', #23295, #20205, #36264, .T. ) ;
#30364=ADVANCED_FACE ( 'NONE', ( #86399 ), #13942, .T. ) ;
#30374=AXIS2_PLACEMENT_3D ( 'NONE', #12405, #27896, #64412 ) ;
#30382=VERTEX_POINT ( 'NONE', #9913 ) ;
#30387=FACE_OUTER_BOUND ( 'NONE', #32213, .T. ) ;
#30395=LINE ( 'NONE', #45402, #29072 ) ;
#30396=CARTESIAN_POINT ( 'NONE',  ( 9.997910040112534702, 15.00000000000000000, 10.50199004140724490 ) ) ;
#30403=CARTESIAN_POINT ( 'NONE',  ( -6.408140936763232709, -10.04303199673624292, 11.09922568453595026 ) ) ;
#30404=VECTOR ( 'NONE', #44620, 1000.000000000000227 ) ;
#30408=DIRECTION ( 'NONE',  ( 0.000000000000000000, 1.000000000000000000, 0.000000000000000000 ) ) ;
#30415=DIRECTION ( 'NONE',  ( -0.000000000000000000, -1.000000000000000000, -0.000000000000000000 ) ) ;
#30426=CARTESIAN_POINT ( 'NONE',  ( -9.159723438033276821, -0.03417435944610275333, 10.91613331444536250 ) ) ;
#30429=FACE_OUTER_BOUND ( 'NONE', #90501, .T. ) ;
#30430=DIRECTION ( 'NONE',  ( -0.9969173337331285190, 0.000000000000000000, 0.07845909572783862918 ) ) ;
#30432=AXIS2_PLACEMENT_3D ( 'NONE', #4553, #96042, #57532 ) ;
#30445=CARTESIAN_POINT ( 'NONE',  ( -8.235571585149871865, 9.493033628982651351, -8.235571585149866536 ) ) ;
#30456=CARTESIAN_POINT ( 'NONE',  ( 10.36894250292379027, -1.321251165086033907, 10.36894250292378672 ) ) ;
#30466=PLANE ( 'NONE',  #27341 ) ;
#30471=CARTESIAN_POINT ( 'NONE',  ( -7.964842623401179544, 32.43868534415485527, -7.964842623401174215 ) ) ;
#30482=DIRECTION ( 'NONE',  ( 0.000000000000000000, 0.000000000000000000, 1.000000000000000000 ) ) ;
#30483=EDGE_CURVE ( 'NONE', #65662, #48512, #36333, .T. ) ;
#30493=ORIENTED_EDGE ( 'NONE', *, *, #26174, .T. ) ;
#30502=CARTESIAN_POINT ( 'NONE',  ( -13.82671409943298357, 15.00000000000000000, 3.447387012295131115 ) ) ;
#30504=DIRECTION ( 'NONE',  ( -0.000000000000000000, -1.000000000000000000, -0.000000000000000000 ) ) ;
#30506=CARTESIAN_POINT ( 'NONE',  ( 0.000000000000000000, 0.5000000000000004441, 0.000000000000000000 ) ) ;
#30507=AXIS2_PLACEMENT_3D ( 'NONE', #84603, #14136, #77088 ) ;
#30509=ORIENTED_EDGE ( 'NONE', *, *, #80043, .T. ) ;
#30514=DIRECTION ( 'NONE',  ( 0.000000000000000000, 1.000000000000000000, 0.000000000000000000 ) ) ;
#30521=TOROIDAL_SURFACE ( 'NONE', #6549, 14.49999999999999822, 0.5000000000000000000 ) ;
#30524=CARTESIAN_POINT ( 'NONE',  ( 7.208316651077762316, 19.13393115100078745, -7.208316651077764980 ) ) ;
#30526=CARTESIAN_POINT ( 'NONE',  ( -5.171435456984247558, 0.000000000000000000, 1.730338099013940978 ) ) ;
#30540=ORIENTED_EDGE ( 'NONE', *, *, #74328, .F. ) ;
#30542=ORIENTED_EDGE ( 'NONE', *, *, #67677, .F. ) ;
#30551=VERTEX_POINT ( 'NONE', #5456 ) ;
#30563=ORIENTED_EDGE ( 'NONE', *, *, #79610, .T. ) ;
#30564=CARTESIAN_POINT ( 'NONE',  ( -11.92686044187656513, 4.688309369127514614, 3.903127820947815962E-15 ) ) ;
#30570=CARTESIAN_POINT ( 'NONE',  ( 7.684764310694881750, 14.63595249122788999, -12.88194075009936057 ) ) ;
#30573=TOROIDAL_SURFACE ( 'NONE', #43348, 14.49999999999999822, 0.5000000000000000000 ) ;
#30575=ORIENTED_EDGE ( 'NONE', *, *, #67635, .T. ) ;
#30583=DIRECTION ( 'NONE',  ( 0.9636304532086229502, 0.000000000000000000, -0.2672383760782571227 ) ) ;
#30588=CARTESIAN_POINT ( 'NONE',  ( 10.88017736071109987, -14.22798132251182679, -2.915334737309928315 ) ) ;
#30590=DIRECTION ( 'NONE',  ( -0.000000000000000000, 1.000000000000000000, -0.000000000000000000 ) ) ;
#30592=CARTESIAN_POINT ( 'NONE',  ( 0.000000000000000000, 13.17686044187655270, 0.000000000000000000 ) ) ;
#30593=PLANE ( 'NONE',  #37019 ) ;
#30594=CARTESIAN_POINT ( 'NONE',  ( -0.1034006766853582671, 15.00000000000000000, 14.49963131601234956 ) ) ;
#30600=EDGE_CURVE ( 'NONE', #7752, #74794, #29053, .T. ) ;
#30608=DIRECTION ( 'NONE',  ( 0.9890158633619187123, 0.000000000000000000, -0.1478094111295981949 ) ) ;
#30616=ORIENTED_EDGE ( 'NONE', *, *, #94013, .T. ) ;
#30632=CARTESIAN_POINT ( 'NONE',  ( -2.638427012816824124, -22.94940218233254470, 9.846743663894596210 ) ) ;
#30633=ORIENTED_EDGE ( 'NONE', *, *, #47623, .T. ) ;
#30635=VERTEX_POINT ( 'NONE', #12933 ) ;
#30636=ORIENTED_EDGE ( 'NONE', *, *, #57231, .T. ) ;
#30637=DIRECTION ( 'NONE',  ( 0.000000000000000000, 0.000000000000000000, 1.000000000000000000 ) ) ;
#30646=VECTOR ( 'NONE', #96336, 1000.000000000000000 ) ;
#30648=CARTESIAN_POINT ( 'NONE',  ( -6.408140936763246032, 23.29030133659709634, -11.09922568453594316 ) ) ;
#30649=VERTEX_POINT ( 'NONE', #57934 ) ;
#30650=AXIS2_PLACEMENT_3D ( 'NONE', #68909, #60894, #23416 ) ;
#30654=VERTEX_POINT ( 'NONE', #42458 ) ;
#30660=DIRECTION ( 'NONE',  ( 0.000000000000000000, 1.000000000000000000, 0.000000000000000000 ) ) ;
#30664=CARTESIAN_POINT ( 'NONE',  ( -13.75801628063875803, 4.618045246005505222E-16, -4.578972376164643698 ) ) ;
#30666=CARTESIAN_POINT ( 'NONE',  ( -14.29730467489530632, 4.415605380435452030E-16, -2.416004766803409254 ) ) ;
#30675=CARTESIAN_POINT ( 'NONE',  ( -10.58171042697183850, 14.76984967302771601, 10.54749450092394625 ) ) ;
#30676=ORIENTED_EDGE ( 'NONE', *, *, #96432, .F. ) ;
#30678=CARTESIAN_POINT ( 'NONE',  ( -13.82192141328815715, 4.664367351173465489E-16, 4.382292601468585680 ) ) ;
#30688=CARTESIAN_POINT ( 'NONE',  ( 0.7577696756376512965, 0.2301502180066073988, -14.92139465029747747 ) ) ;
#30689=TOROIDAL_SURFACE ( 'NONE', #414, 14.49999999999999822, 0.5000000000000000000 ) ;
#30692=DIRECTION ( 'NONE',  ( -4.618527782440651208E-14, 0.000000000000000000, 1.000000000000000000 ) ) ;
#30704=CARTESIAN_POINT ( 'NONE',  ( -10.36894250292378317, 22.42874883491397853, 10.36894250292379560 ) ) ;
#30710=AXIS2_PLACEMENT_3D ( 'NONE', #66100, #29090, #37602 ) ;
#30721=VECTOR ( 'NONE', #7825, 1000.000000000000000 ) ;
#30726=ORIENTED_EDGE ( 'NONE', *, *, #66459, .F. ) ;
#30729=CARTESIAN_POINT ( 'NONE',  ( -12.25993886608593364, 0.5000000000000004441, -8.642563219313787570 ) ) ;
#30736=CARTESIAN_POINT ( 'NONE',  ( 5.428133280998942212, 0.000000000000000000, 0.5226697871167882425 ) ) ;
#30739=AXIS2_PLACEMENT_3D ( 'NONE', #71785, #60950, #40806 ) ;
#30740=ORIENTED_EDGE ( 'NONE', *, *, #56486, .F. ) ;
#30741=ORIENTED_EDGE ( 'NONE', *, *, #70598, .F. ) ;
#30743=PLANE ( 'NONE',  #81195 ) ;
#30748=DIRECTION ( 'NONE',  ( 0.3665012267242945265, 0.000000000000000000, 0.9304175679820255729 ) ) ;
#30760=ORIENTED_EDGE ( 'NONE', *, *, #28453, .F. ) ;
#30766=ORIENTED_EDGE ( 'NONE', *, *, #86264, .F. ) ;
#30779=CARTESIAN_POINT ( 'NONE',  ( 13.34343830728399283, 0.5000000000000004441, 6.852200678592689442 ) ) ;
#30784=ORIENTED_EDGE ( 'NONE', *, *, #39699, .T. ) ;
#30789=AXIS2_PLACEMENT_3D ( 'NONE', #67713, #82701, #52207 ) ;
#30794=B_SPLINE_CURVE_WITH_KNOTS ( 'NONE', 3,
 ( #32804, #18312, #41811, #63299, #10319, #87774 ),
 .UNSPECIFIED., .F., .F.,
 ( 4, 2, 4 ),
 ( 3.409110551419719510E-05, 0.0004400426677360445436, 0.0008459942299578918990 ),
 .UNSPECIFIED. ) ;
#30795=B_SPLINE_CURVE_WITH_KNOTS ( 'NONE', 3,
 ( #15, #512, #54932, #84473, #93437, #1970 ),
 .UNSPECIFIED., .F., .F.,
 ( 4, 2, 4 ),
 ( 0.0002800075630655414352, 0.0006862128664597091660, 0.001092418169853877005 ),
 .UNSPECIFIED. ) ;
#30810=EDGE_CURVE ( 'NONE', #53420, #52573, #18570, .T. ) ;
#30817=EDGE_LOOP ( 'NONE', ( #46295, #32752, #5052, #318, #52787, #83077 ) ) ;
#30820=LINE ( 'NONE', #91325, #83875 ) ;
#30831=CARTESIAN_POINT ( 'NONE',  ( 9.519554572442881835, -3.083623444479279201E-15, 11.10344954678186369 ) ) ;
#30837=VERTEX_POINT ( 'NONE', #81429 ) ;
#30838=EDGE_CURVE ( 'NONE', #71952, #5095, #63413, .T. ) ;
#30841=DIRECTION ( 'NONE',  ( -0.9426414910921805390, 0.000000000000000000, 0.3338068592337649076 ) ) ;
#30842=FACE_OUTER_BOUND ( 'NONE', #67074, .T. ) ;
#30849=ADVANCED_FACE ( 'NONE', ( #18971 ), #48962, .F. ) ;
#30850=EDGE_LOOP ( 'NONE', ( #70940, #74394, #81581, #59648 ) ) ;
#30852=CARTESIAN_POINT ( 'NONE',  ( -10.97324858046188467, 15.00000000000000711, -9.670892530813352650 ) ) ;
#30858=PLANE ( 'NONE',  #43214 ) ;
#30862=CARTESIAN_POINT ( 'NONE',  ( 5.419894505350511871, 0.3639313574487206271, 13.98659156302465156 ) ) ;
#30863=CARTESIAN_POINT ( 'NONE',  ( -11.92686044187656869, 2.453790035174480355, -3.195792623639521768 ) ) ;
#30867=AXIS2_PLACEMENT_3D ( 'NONE', #43387, #12399, #95919 ) ;
#30872=CIRCLE ( 'NONE', #29294, 15.00000000000000000 ) ;
#30877=CIRCLE ( 'NONE', #81969, 14.49999999999999822 ) ;
#30883=EDGE_CURVE ( 'NONE', #13031, #70888, #57065, .T. ) ;
#30895=CARTESIAN_POINT ( 'NONE',  ( -13.96521320569119595, 0.04922511925147229905, -4.755935267939353395 ) ) ;
#30897=ORIENTED_EDGE ( 'NONE', *, *, #84820, .F. ) ;
#30901=DIRECTION ( 'NONE',  ( 0.000000000000000000, 1.000000000000000000, 0.000000000000000000 ) ) ;
#30912=ADVANCED_FACE ( 'NONE', ( #33962 ), #48985, .T. ) ;
#30913=VERTEX_POINT ( 'NONE', #71980 ) ;
#30918=DIRECTION ( 'NONE',  ( 0.3007057995042831666, 0.000000000000000000, -0.9537169507482237130 ) ) ;
#30927=EDGE_CURVE ( 'NONE', #11366, #339, #5152, .T. ) ;
#30931=CARTESIAN_POINT ( 'NONE',  ( -10.29676451088645095, 12.55750643096800445, -4.707860652926549427 ) ) ;
#30943=ORIENTED_EDGE ( 'NONE', *, *, #45390, .F. ) ;
#30947=CARTESIAN_POINT ( 'NONE',  ( -0.9940297508538862292, 0.000000000000000000, 14.21528771620248932 ) ) ;
#30950=CARTESIAN_POINT ( 'NONE',  ( -3.795296366450300773, -7.154584498419361616, 14.16423886937410437 ) ) ;
#30964=CARTESIAN_POINT ( 'NONE',  ( -0.8218345515130114354, 14.95077488074853456, 14.72992491912909152 ) ) ;
#30975=ORIENTED_EDGE ( 'NONE', *, *, #4099, .F. ) ;
#30978=DIRECTION ( 'NONE',  ( -0.000000000000000000, -1.000000000000000000, -0.000000000000000000 ) ) ;
#30983=CYLINDRICAL_SURFACE ( 'NONE', #40029, 15.00000000000000000 ) ;
#30985=ORIENTED_EDGE ( 'NONE', *, *, #87380, .T. ) ;
#30987=FACE_OUTER_BOUND ( 'NONE', #93511, .T. ) ;
#31000=CARTESIAN_POINT ( 'NONE',  ( 4.020549461440701577, 0.000000000000000000, 3.684154808197116271 ) ) ;
#31002=EDGE_LOOP ( 'NONE', ( #90982, #80496, #13679, #67311 ) ) ;
#31017=CARTESIAN_POINT ( 'NONE',  ( 6.408140936763243367, -39.20969866340291077, 11.09922568453594494 ) ) ;
#31019=EDGE_LOOP ( 'NONE', ( #96242, #15216, #23201, #50305 ) ) ;
#31031=VERTEX_POINT ( 'NONE', #79975 ) ;
#31038=ADVANCED_FACE ( 'NONE', ( #72462 ), #90538, .T. ) ;
#31040=CARTESIAN_POINT ( 'NONE',  ( 4.838527690343618737, 14.49999999999999822, -14.19819177887726624 ) ) ;
#31041=AXIS2_PLACEMENT_3D ( 'NONE', #62343, #77350, #47837 ) ;
#31044=ORIENTED_EDGE ( 'NONE', *, *, #57243, .T. ) ;
#31048=VERTEX_POINT ( 'NONE', #93430 ) ;
#31049=LINE ( 'NONE', #606, #98592 ) ;
#31053=CARTESIAN_POINT ( 'NONE',  ( 5.056330833731640162, 15.00000000000000000, 13.58983143750701394 ) ) ;
#31058=VERTEX_POINT ( 'NONE', #40936 ) ;
#31061=B_SPLINE_CURVE_WITH_KNOTS ( 'NONE', 3,
 ( #5250, #36224, #5738, #97249, #49256, #50225 ),
 .UNSPECIFIED., .F., .F.,
 ( 4, 2, 4 ),
 ( 3.409110551496096809E-05, 0.0004400426677367859211, 0.0008459942299586109419 ),
 .UNSPECIFIED. ) ;
#31076=DIRECTION ( 'NONE',  ( 0.000000000000000000, 1.000000000000000000, 0.000000000000000000 ) ) ;
#31079=EDGE_CURVE ( 'NONE', #75433, #1023, #87403, .T. ) ;
#31084=CARTESIAN_POINT ( 'NONE',  ( -10.88017736071109987, 8.272018677488171434, 2.915334737309934532 ) ) ;
#31088=CARTESIAN_POINT ( 'NONE',  ( -3.420591144908390113, 14.49999999999999112, -14.60477854057966063 ) ) ;
#31098=DIRECTION ( 'NONE',  ( 0.000000000000000000, 0.000000000000000000, 1.000000000000000000 ) ) ;
#31103=DIRECTION ( 'NONE',  ( 0.9366721892483971246, -0.000000000000000000, 0.3502073812594687086 ) ) ;
#31127=CARTESIAN_POINT ( 'NONE',  ( 2.638427012816835227, -7.532735515665882176, 9.846743663894590881 ) ) ;
#31129=ORIENTED_EDGE ( 'NONE', *, *, #3195, .F. ) ;
#31130=CARTESIAN_POINT ( 'NONE',  ( 14.16722289976690163, 14.49999999999999112, -4.928467845925561974 ) ) ;
#31132=ORIENTED_EDGE ( 'NONE', *, *, #74382, .T. ) ;
#31134=ORIENTED_EDGE ( 'NONE', *, *, #62317, .F. ) ;
#31140=EDGE_CURVE ( 'NONE', #189, #62655, #19401, .T. ) ;
#31141=CARTESIAN_POINT ( 'NONE',  ( -2.393480905993287777, 14.49999999999999112, 14.80781041047755409 ) ) ;
#31145=CARTESIAN_POINT ( 'NONE',  ( 6.408140936763243367, 20.79030133659709634, 11.09922568453594494 ) ) ;
#31154=CARTESIAN_POINT ( 'NONE',  ( -14.62617646268089899, 0.5000000000000004441, 3.327906561566782440 ) ) ;
#31159=TOROIDAL_SURFACE ( 'NONE', #16834, 14.49999999999999822, 0.5000000000000000000 ) ;
#31160=DIRECTION ( 'NONE',  ( 0.000000000000000000, 0.000000000000000000, 1.000000000000000000 ) ) ;
#31162=CARTESIAN_POINT ( 'NONE',  ( -8.606322355891206755, 3.940577227621431661E-16, -11.66967075398818743 ) ) ;
#31163=VERTEX_POINT ( 'NONE', #40444 ) ;
#31172=CARTESIAN_POINT ( 'NONE',  ( 11.36220558718861717, 15.00000000000000000, -9.008345252845218809 ) ) ;
#31173=CARTESIAN_POINT ( 'NONE',  ( -11.36220558719268325, 15.00000000000000000, -9.008345252852777207 ) ) ;
#31185=TOROIDAL_SURFACE ( 'NONE', #87084, 14.49999999999999822, 0.5000000000000000000 ) ;
#31187=ORIENTED_EDGE ( 'NONE', *, *, #32, .F. ) ;
#31188=CARTESIAN_POINT ( 'NONE',  ( 0.000000000000000000, 0.5000000000000004441, 0.000000000000000000 ) ) ;
#31194=CARTESIAN_POINT ( 'NONE',  ( 8.731067818237042033, 4.537123368507811172, 8.731067818237033151 ) ) ;
#31199=CARTESIAN_POINT ( 'NONE',  ( 10.36894250292378850, 14.92874883491396254, -10.36894250292379027 ) ) ;
#31214=AXIS2_PLACEMENT_3D ( 'NONE', #527, #91978, #15514 ) ;
#31218=ORIENTED_EDGE ( 'NONE', *, *, #53839, .F. ) ;
#31220=DIRECTION ( 'NONE',  ( 0.000000000000000000, 0.000000000000000000, 1.000000000000000000 ) ) ;
#31240=CARTESIAN_POINT ( 'NONE',  ( 6.138934250732054565, 15.00000000000000000, -14.77128574976607389 ) ) ;
#31248=EDGE_LOOP ( 'NONE', ( #81452, #89092, #97120, #22777 ) ) ;
#31249=CARTESIAN_POINT ( 'NONE',  ( 5.451370222425311773, 0.000000000000000000, 0.1427491530890473426 ) ) ;
#31252=ORIENTED_EDGE ( 'NONE', *, *, #91835, .T. ) ;
#31253=VECTOR ( 'NONE', #11270, 1000.000000000000000 ) ;
#31261=CARTESIAN_POINT ( 'NONE',  ( 12.21238578216004633, 15.00000000000000711, 8.049595036947206239 ) ) ;
#31265=EDGE_LOOP ( 'NONE', ( #51065, #50815, #41804, #69719 ) ) ;
#31269=LINE ( 'NONE', #54268, #60652 ) ;
#31273=CIRCLE ( 'NONE', #55264, 15.00000000000000000 ) ;
#31276=EDGE_CURVE ( 'NONE', #7752, #82423, #93924, .T. ) ;
#31279=DIRECTION ( 'NONE',  ( 0.000000000000000000, 1.000000000000000000, 0.000000000000000000 ) ) ;
#31280=VECTOR ( 'NONE', #96443, 1000.000000000000000 ) ;
#31286=FACE_OUTER_BOUND ( 'NONE', #11265, .T. ) ;
#31291=CARTESIAN_POINT ( 'NONE',  ( 14.43100913236850502, 4.664102659404345836E-16, -1.412789942453164693 ) ) ;
#31295=CARTESIAN_POINT ( 'NONE',  ( 12.60589901313219663, 0.3639308464568737356, 8.129656208642145998 ) ) ;
#31307=CARTESIAN_POINT ( 'NONE',  ( -7.771322705631588335, 4.175205849424987664E-16, 12.24159072199911868 ) ) ;
#31317=ADVANCED_FACE ( 'NONE', ( #33885 ), #21908, .T. ) ;
#31319=FACE_OUTER_BOUND ( 'NONE', #4600, .T. ) ;
#31335=ORIENTED_EDGE ( 'NONE', *, *, #29323, .T. ) ;
#31336=CARTESIAN_POINT ( 'NONE',  ( 10.82078848414219330, -0.03417435944610275333, -11.78082904627298433 ) ) ;
#31342=DIRECTION ( 'NONE',  ( 0.000000000000000000, 1.000000000000000000, 0.000000000000000000 ) ) ;
#31354=B_SPLINE_CURVE_WITH_KNOTS ( 'NONE', 3,
 ( #8334, #22363, #23843, #84823, #16330, #46813 ),
 .UNSPECIFIED., .F., .F.,
 ( 4, 2, 4 ),
 ( 3.409110551494637202E-05, 0.0004400426677367937816, 0.0008459942299586411911 ),
 .UNSPECIFIED. ) ;
#31370=FACE_OUTER_BOUND ( 'NONE', #67060, .T. ) ;
#31376=FACE_OUTER_BOUND ( 'NONE', #40674, .T. ) ;
#31380=DIRECTION ( 'NONE',  ( -0.9969173337331274087, 0.000000000000000000, -0.07845909572785238206 ) ) ;
#31383=ORIENTED_EDGE ( 'NONE', *, *, #7055, .F. ) ;
#31398=CIRCLE ( 'NONE', #61737, 14.49999999999999822 ) ;
#31400=ADVANCED_FACE ( 'NONE', ( #90340 ), #21374, .T. ) ;
#31401=ORIENTED_EDGE ( 'NONE', *, *, #37851, .F. ) ;
#31408=LINE ( 'NONE', #76433, #6945 ) ;
#31410=LINE ( 'NONE', #46910, #3645 ) ;
#31411=DIRECTION ( 'NONE',  ( 0.7253743710122867450, 0.000000000000000000, -0.6883545756937550220 ) ) ;
#31413=ORIENTED_EDGE ( 'NONE', *, *, #6577, .T. ) ;
#31414=CARTESIAN_POINT ( 'NONE',  ( 11.49638213510182005, 14.95077488074853811, -9.245501498401928586 ) ) ;
#31425=LINE ( 'NONE', #38465, #86099 ) ;
#31432=DIRECTION ( 'NONE',  ( 0.000000000000000000, 1.000000000000000000, -0.000000000000000000 ) ) ;
#31434=EDGE_CURVE ( 'NONE', #93127, #29027, #34715, .T. ) ;
#31436=AXIS2_PLACEMENT_3D ( 'NONE', #87011, #48020, #10042 ) ;
#31438=CARTESIAN_POINT ( 'NONE',  ( 3.469446951953614189E-15, -11.94625116508602680, 14.16423886937410259 ) ) ;
#31439=VECTOR ( 'NONE', #74137, 1000.000000000000000 ) ;
#31444=ORIENTED_EDGE ( 'NONE', *, *, #70473, .T. ) ;
#31449=CARTESIAN_POINT ( 'NONE',  ( -13.40508947812159235, 3.877950237245923868E-16, -5.527528931046294502 ) ) ;
#31451=FACE_OUTER_BOUND ( 'NONE', #15574, .T. ) ;
#31452=DIRECTION ( 'NONE',  ( 0.000000000000000000, 0.000000000000000000, 1.000000000000000000 ) ) ;
#31462=CARTESIAN_POINT ( 'NONE',  ( -5.419894505350674407, 15.00000000000000000, 13.98659156302455031 ) ) ;
#31483=VERTEX_POINT ( 'NONE', #73373 ) ;
#31485=EDGE_CURVE ( 'NONE', #20205, #79142, #52356, .T. ) ;
#31489=ORIENTED_EDGE ( 'NONE', *, *, #92124, .F. ) ;
#31499=CIRCLE ( 'NONE', #53849, 15.00000000000000000 ) ;
#31505=CARTESIAN_POINT ( 'NONE',  ( -3.434112377981047626, -39.83469866340291787, 12.81628187352647963 ) ) ;
#31506=TOROIDAL_SURFACE ( 'NONE', #50637, 14.49999999999999822, 0.5000000000000000000 ) ;
#31507=ORIENTED_EDGE ( 'NONE', *, *, #61311, .T. ) ;
#31510=EDGE_CURVE ( 'NONE', #25131, #28832, #70300, .T. ) ;
#31526=EDGE_CURVE ( 'NONE', #65924, #65919, #57877, .T. ) ;
#31536=ORIENTED_EDGE ( 'NONE', *, *, #79405, .T. ) ;
#31538=ORIENTED_EDGE ( 'NONE', *, *, #12207, .F. ) ;
#31539=VERTEX_POINT ( 'NONE', #27386 ) ;
#31546=VECTOR ( 'NONE', #89234, 1000.000000000000000 ) ;
#31551=ORIENTED_EDGE ( 'NONE', *, *, #64028, .F. ) ;
#31555=DIRECTION ( 'NONE',  ( -0.4461978131098006117, 0.000000000000000000, -0.8949343616020291048 ) ) ;
#31558=PLANE ( 'NONE',  #68137 ) ;
#31559=AXIS2_PLACEMENT_3D ( 'NONE', #95070, #81059, #65051 ) ;
#31561=ORIENTED_EDGE ( 'NONE', *, *, #56250, .T. ) ;
#31573=B_SPLINE_CURVE_WITH_KNOTS ( 'NONE', 3,
 ( #73131, #58126, #13631, #58637, #89137, #95659 ),
 .UNSPECIFIED., .F., .F.,
 ( 4, 2, 4 ),
 ( 0.0002800075630785946873, 0.0006862128664728985939, 0.001092418169867202500 ),
 .UNSPECIFIED. ) ;
#31574=CARTESIAN_POINT ( 'NONE',  ( 5.440088680355549045, 1.397018677488176541, -9.422509992056141925 ) ) ;
#31579=VECTOR ( 'NONE', #47683, 1000.000000000000000 ) ;
#31584=CARTESIAN_POINT ( 'NONE',  ( -6.898461952320240620, 15.00000000000000000, -12.75387089053316636 ) ) ;
#31591=ORIENTED_EDGE ( 'NONE', *, *, #86174, .F. ) ;
#31602=EDGE_CURVE ( 'NONE', #59678, #62057, #80888, .T. ) ;
#31618=EDGE_CURVE ( 'NONE', #44682, #1372, #81375, .T. ) ;
#31622=CARTESIAN_POINT ( 'NONE',  ( 9.846743663894594434, -6.491068848999207219, -2.168404344971008868E-15 ) ) ;
#31624=LINE ( 'NONE', #93114, #69917 ) ;
#31626=DIRECTION ( 'NONE',  ( -0.000000000000000000, -1.000000000000000000, -0.000000000000000000 ) ) ;
#31633=EDGE_CURVE ( 'NONE', #90793, #83574, #43370, .T. ) ;
#31638=EDGE_CURVE ( 'NONE', #15080, #14929, #73046, .T. ) ;
#31640=ORIENTED_EDGE ( 'NONE', *, *, #8766, .F. ) ;
#31653=CIRCLE ( 'NONE', #44435, 14.49999999999999822 ) ;
#31655=ORIENTED_EDGE ( 'NONE', *, *, #73462, .T. ) ;
#31658=ORIENTED_EDGE ( 'NONE', *, *, #37056, .F. ) ;
#31661=CARTESIAN_POINT ( 'NONE',  ( 0.9940297508537879745, 15.00000000000000000, -14.21528771620249820 ) ) ;
#31663=ORIENTED_EDGE ( 'NONE', *, *, #91354, .T. ) ;
#31665=DIRECTION ( 'NONE',  ( 0.000000000000000000, 0.000000000000000000, 1.000000000000000000 ) ) ;
#31687=EDGE_CURVE ( 'NONE', #36285, #20560, #93571, .T. ) ;
#31691=CARTESIAN_POINT ( 'NONE',  ( -2.915334737309934532, -32.97798132251182324, -10.88017736071109987 ) ) ;
#31701=VERTEX_POINT ( 'NONE', #75849 ) ;
#31707=CARTESIAN_POINT ( 'NONE',  ( 6.689969769698871360, 0.000000000000000000, 12.58200319823975022 ) ) ;
#31724=DIRECTION ( 'NONE',  ( 0.000000000000000000, -0.000000000000000000, 1.000000000000000000 ) ) ;
#31725=TOROIDAL_SURFACE ( 'NONE', #49281, 14.49999999999999822, 0.5000000000000000000 ) ;
#31726=EDGE_CURVE ( 'NONE', #56575, #13765, #9178, .T. ) ;
#31727=ORIENTED_EDGE ( 'NONE', *, *, #78519, .T. ) ;
#31728=EDGE_LOOP ( 'NONE', ( #19214, #11349, #3511, #74790, #60299, #65876 ) ) ;
#31736=DIRECTION ( 'NONE',  ( -0.9996573249755573709, 0.000000000000000000, 0.02617694830786938473 ) ) ;
#31738=EDGE_CURVE ( 'NONE', #41155, #91322, #85848, .T. ) ;
#31741=DIRECTION ( 'NONE',  ( -0.000000000000000000, -1.000000000000000000, -0.000000000000000000 ) ) ;
#31746=CARTESIAN_POINT ( 'NONE',  ( -1.354709868695410657, 0.5000000000000004441, -14.93870011653153362 ) ) ;
#31748=ORIENTED_EDGE ( 'NONE', *, *, #61362, .T. ) ;
#31755=ORIENTED_EDGE ( 'NONE', *, *, #91797, .T. ) ;
#31761=EDGE_CURVE ( 'NONE', #31031, #65562, #90605, .T. ) ;
#31766=CARTESIAN_POINT ( 'NONE',  ( 2.815433093577122126, 0.5000000000000004441, -14.73340885523749932 ) ) ;
#31769=ORIENTED_EDGE ( 'NONE', *, *, #15084, .F. ) ;
#31776=DIRECTION ( 'NONE',  ( -0.9762960071199316969, 0.000000000000000000, -0.2164396139381103423 ) ) ;
#31783=DIRECTION ( 'NONE',  ( 0.000000000000000000, 0.000000000000000000, -1.000000000000000000 ) ) ;
#31786=DIRECTION ( 'NONE',  ( -0.8141155183563145714, 0.000000000000000000, -0.5807029557109463225 ) ) ;
#31800=EDGE_CURVE ( 'NONE', #64703, #81191, #54229, .T. ) ;
#31808=CARTESIAN_POINT ( 'NONE',  ( 0.000000000000000000, 14.49999999999999822, 0.000000000000000000 ) ) ;
#31812=CARTESIAN_POINT ( 'NONE',  ( 11.36220558718863138, 4.417444789370043464E-16, -9.008345252845243678 ) ) ;
#31817=CARTESIAN_POINT ( 'NONE',  ( 12.74414838903271452, 15.00000000000000888, 7.178093659842060603 ) ) ;
#31826=CARTESIAN_POINT ( 'NONE',  ( 3.715841784917714108, 15.00000000000000000, 15.55859621770270529 ) ) ;
#31834=FACE_OUTER_BOUND ( 'NONE', #35443, .T. ) ;
#31838=DIRECTION ( 'NONE',  ( 0.000000000000000000, 1.000000000000000000, 0.000000000000000000 ) ) ;
#31841=VECTOR ( 'NONE', #26065, 1000.000000000000000 ) ;
#31843=EDGE_CURVE ( 'NONE', #41037, #81080, #17190, .T. ) ;
#31846=CARTESIAN_POINT ( 'NONE',  ( 5.200846386093635587, 0.000000000000000000, -1.639820566680944225 ) ) ;
#31877=DIRECTION ( 'NONE',  ( 0.000000000000000000, 0.000000000000000000, -1.000000000000000000 ) ) ;
#31882=TOROIDAL_SURFACE ( 'NONE', #46253, 14.49999999999999822, 0.5000000000000000000 ) ;
#31888=ORIENTED_EDGE ( 'NONE', *, *, #97816, .T. ) ;
#31893=DIRECTION ( 'NONE',  ( 0.000000000000000000, 0.000000000000000000, 1.000000000000000000 ) ) ;
#31897=DIRECTION ( 'NONE',  ( 0.000000000000000000, 0.000000000000000000, 1.000000000000000000 ) ) ;
#31900=CARTESIAN_POINT ( 'NONE',  ( 0.000000000000000000, 0.5000000000000004441, 0.000000000000000000 ) ) ;
#31908=CARTESIAN_POINT ( 'NONE',  ( 14.62617646268087768, 0.5000000000000004441, -3.327906561566883692 ) ) ;
#31913=DIRECTION ( 'NONE',  ( -0.1132032137679106348, 0.000000000000000000, 0.9935718556765871234 ) ) ;
#31922=ADVANCED_FACE ( 'NONE', ( #31319 ), #61819, .F. ) ;
#31925=CARTESIAN_POINT ( 'NONE',  ( 3.795296366450306547, -9.654584498419360727, -14.16423886937410259 ) ) ;
#31932=CARTESIAN_POINT ( 'NONE',  ( 0.000000000000000000, 14.49999999999999822, 0.000000000000000000 ) ) ;
#31935=CARTESIAN_POINT ( 'NONE',  ( -14.26139399674459263, 4.837279266207889341E-16, 2.619664342929711509 ) ) ;
#31948=ORIENTED_EDGE ( 'NONE', *, *, #92212, .F. ) ;
#31952=ADVANCED_FACE ( 'NONE', ( #22368 ), #52353, .T. ) ;
#31958=LINE ( 'NONE', #16989, #59133 ) ;
#31959=CARTESIAN_POINT ( 'NONE',  ( 10.91061041304821977, 0.2306972965111880602, 10.20767530377056431 ) ) ;
#31961=CARTESIAN_POINT ( 'NONE',  ( 11.96291822454875842, 15.00000000000000000, 8.193813980849165901 ) ) ;
#31967=AXIS2_PLACEMENT_3D ( 'NONE', #58740, #4280, #50245 ) ;
#31971=VERTEX_POINT ( 'NONE', #85816 ) ;
#31972=CARTESIAN_POINT ( 'NONE',  ( -6.898461952320262824, 4.061641280801676772E-16, -12.75387089053318590 ) ) ;
#31986=LINE ( 'NONE', #93496, #68436 ) ;
#31988=LINE ( 'NONE', #38171, #43094 ) ;
#31990=CARTESIAN_POINT ( 'NONE',  ( 9.846743663894590881, 23.30059781766746596, 2.638427012816828565 ) ) ;
#31991=ORIENTED_EDGE ( 'NONE', *, *, #41900, .T. ) ;
#31992=CARTESIAN_POINT ( 'NONE',  ( -6.761335002692915985, 14.76984993307862837, -13.32315948060046829 ) ) ;
#32006=ORIENTED_EDGE ( 'NONE', *, *, #42012, .T. ) ;
#32007=TOROIDAL_SURFACE ( 'NONE', #91114, 14.49999999999999822, 0.5000000000000000000 ) ;
#32010=ORIENTED_EDGE ( 'NONE', *, *, #1305, .T. ) ;
#32016=CARTESIAN_POINT ( 'NONE',  ( -5.302565485995502037, 0.000000000000000000, 1.273033341818796460 ) ) ;
#32019=ORIENTED_EDGE ( 'NONE', *, *, #64952, .T. ) ;
#32023=CARTESIAN_POINT ( 'NONE',  ( 12.60589901313216110, 0.5000000000000004441, 8.129656208642140669 ) ) ;
#32033=ORIENTED_EDGE ( 'NONE', *, *, #97652, .T. ) ;
#32036=VECTOR ( 'NONE', #30583, 1000.000000000000000 ) ;
#32039=EDGE_CURVE ( 'NONE', #54527, #30230, #95582, .T. ) ;
#32046=VERTEX_POINT ( 'NONE', #79780 ) ;
#32054=DIRECTION ( 'NONE',  ( 0.000000000000000000, 0.000000000000000000, -1.000000000000000000 ) ) ;
#32058=CARTESIAN_POINT ( 'NONE',  ( -7.964842623401179544, 2.438685344154844170, -7.964842623401174215 ) ) ;
#32060=CARTESIAN_POINT ( 'NONE',  ( 14.56089864659469946, -2.824431362619463692E-15, 1.374314915485391753 ) ) ;
#32064=CARTESIAN_POINT ( 'NONE',  ( 0.000000000000000000, 15.00000000000000000, 0.000000000000000000 ) ) ;
#32068=CARTESIAN_POINT ( 'NONE',  ( 0.000000000000000000, 15.00000000000000000, 0.000000000000000000 ) ) ;
#32069=CARTESIAN_POINT ( 'NONE',  ( 3.469446951953614189E-15, 10.93830936912750573, 11.92686044187656513 ) ) ;
#32070=ADVANCED_FACE ( 'NONE', ( #70824 ), #56986, .T. ) ;
#32077=ORIENTED_EDGE ( 'NONE', *, *, #54836, .F. ) ;
#32105=CARTESIAN_POINT ( 'NONE',  ( 2.638427012816829897, -15.44940218233254470, -9.846743663894592657 ) ) ;
#32107=LINE ( 'NONE', #16644, #97065 ) ;
#32108=ORIENTED_EDGE ( 'NONE', *, *, #97600, .F. ) ;
#32111=AXIS2_PLACEMENT_3D ( 'NONE', #59361, #91341, #22869 ) ;
#32117=DIRECTION ( 'NONE',  ( 0.000000000000000000, 1.000000000000000000, 0.000000000000000000 ) ) ;
#32119=CARTESIAN_POINT ( 'NONE',  ( -13.96552416078061043, 14.95037115134968708, -4.756200848675268489 ) ) ;
#32120=EDGE_CURVE ( 'NONE', #64665, #33002, #45755, .T. ) ;
#32121=TOROIDAL_SURFACE ( 'NONE', #14599, 14.49999999999999822, 0.5000000000000000000 ) ;
#32123=ORIENTED_EDGE ( 'NONE', *, *, #55919, .T. ) ;
#32125=ORIENTED_EDGE ( 'NONE', *, *, #64785, .T. ) ;
#32127=VERTEX_POINT ( 'NONE', #15275 ) ;
#32135=CARTESIAN_POINT ( 'NONE',  ( 0.000000000000000000, 14.49999999999999822, 0.000000000000000000 ) ) ;
#32143=FACE_OUTER_BOUND ( 'NONE', #53859, .T. ) ;
#32146=CARTESIAN_POINT ( 'NONE',  ( 14.17193700899789022, 0.000000000000000000, 1.489530601564113654 ) ) ;
#32147=ORIENTED_EDGE ( 'NONE', *, *, #11098, .T. ) ;
#32155=VECTOR ( 'NONE', #21164, 1000.000000000000000 ) ;
#32161=ADVANCED_FACE ( 'NONE', ( #85232 ), #92718, .F. ) ;
#32163=EDGE_CURVE ( 'NONE', #85662, #48243, #54223, .T. ) ;
#32171=LINE ( 'NONE', #93672, #18254 ) ;
#32176=CARTESIAN_POINT ( 'NONE',  ( 5.440088680355556150, -35.26964798917848753, 9.422509992056138373 ) ) ;
#32180=VECTOR ( 'NONE', #85316, 1000.000000000000114 ) ;
#32192=DIRECTION ( 'NONE',  ( 0.6360782202777701677, 0.000000000000000000, -0.7716245833877148907 ) ) ;
#32193=CARTESIAN_POINT ( 'NONE',  ( -2.393480905992977803, 14.49999999999999112, -14.80781041047760382 ) ) ;
#32212=EDGE_LOOP ( 'NONE', ( #68303, #71729, #32245, #33229 ) ) ;
#32213=EDGE_LOOP ( 'NONE', ( #86633, #58288, #93434, #78428, #69643, #17490 ) ) ;
#32214=CARTESIAN_POINT ( 'NONE',  ( 14.09394518620612224, 15.00000000000000000, -3.407449058785360752 ) ) ;
#32215=DIRECTION ( 'NONE',  ( -0.9914448613738113814, 0.000000000000000000, 0.1305261922200445512 ) ) ;
#32223=CARTESIAN_POINT ( 'NONE',  ( 0.000000000000000000, 14.49999999999999822, 0.000000000000000000 ) ) ;
#32227=VECTOR ( 'NONE', #6812, 1000.000000000000000 ) ;
#32236=ORIENTED_EDGE ( 'NONE', *, *, #39579, .T. ) ;
#32238=ORIENTED_EDGE ( 'NONE', *, *, #39625, .F. ) ;
#32242=VERTEX_POINT ( 'NONE', #51904 ) ;
#32244=CARTESIAN_POINT ( 'NONE',  ( -12.81628187352647608, -5.876365330069576842, 3.903127820947815962E-15 ) ) ;
#32245=ORIENTED_EDGE ( 'NONE', *, *, #57243, .F. ) ;
#32249=ORIENTED_EDGE ( 'NONE', *, *, #98486, .F. ) ;
#32257=EDGE_CURVE ( 'NONE', #1146, #13064, #60377, .T. ) ;
#32258=ORIENTED_EDGE ( 'NONE', *, *, #27217, .T. ) ;
#32262=CARTESIAN_POINT ( 'NONE',  ( 2.189666204609191702, 15.00000000000000888, 14.46180170876167992 ) ) ;
#32265=CARTESIAN_POINT ( 'NONE',  ( 12.00809552683952752, 0.5000000000000004441, 8.989195838243626113 ) ) ;
#32272=DIRECTION ( 'NONE',  ( -0.000000000000000000, -1.000000000000000000, -0.000000000000000000 ) ) ;
#32276=CARTESIAN_POINT ( 'NONE',  ( 1.354709868695515684, 0.5000000000000004441, 14.93870011653152652 ) ) ;
#32280=VECTOR ( 'NONE', #94741, 1000.000000000000114 ) ;
#32283=ADVANCED_FACE ( 'NONE', ( #73902 ), #13830, .T. ) ;
#32287=VECTOR ( 'NONE', #47759, 1000.000000000000000 ) ;
#32288=FACE_OUTER_BOUND ( 'NONE', #46282, .T. ) ;
#32299=DIRECTION ( 'NONE',  ( 0.000000000000000000, 0.000000000000000000, 1.000000000000000000 ) ) ;
#32303=CIRCLE ( 'NONE', #48295, 14.49999999999999822 ) ;
#32305=DIRECTION ( 'NONE',  ( -0.9969173337331274087, 0.000000000000000000, -0.07845909572785238206 ) ) ;
#32319=CARTESIAN_POINT ( 'NONE',  ( 1.780824192092501423, 15.00000000000000000, -14.89391369643513485 ) ) ;
#32320=EDGE_CURVE ( 'NONE', #80097, #78251, #35905, .T. ) ;
#32342=CARTESIAN_POINT ( 'NONE',  ( 0.000000000000000000, 15.00000000000000000, 0.000000000000000000 ) ) ;
#32357=ORIENTED_EDGE ( 'NONE', *, *, #68238, .T. ) ;
#32363=VERTEX_POINT ( 'NONE', #66900 ) ;
#32381=CARTESIAN_POINT ( 'NONE',  ( 0.000000000000000000, 0.000000000000000000, 0.000000000000000000 ) ) ;
#32385=EDGE_LOOP ( 'NONE', ( #79342, #58498, #36456, #48535 ) ) ;
#32386=TOROIDAL_SURFACE ( 'NONE', #88283, 14.49999999999999822, 0.5000000000000000000 ) ;
#32391=LINE ( 'NONE', #10887, #8993 ) ;
#32394=CARTESIAN_POINT ( 'NONE',  ( -14.71525861348291819, 14.49999999999999112, -2.908807992686814003 ) ) ;
#32404=ADVANCED_FACE ( 'NONE', ( #31370 ), #92375, .F. ) ;
#32407=CARTESIAN_POINT ( 'NONE',  ( -13.07751017357388257, 4.569076162262063760E-16, 6.263284095430414311 ) ) ;
#32428=CARTESIAN_POINT ( 'NONE',  ( -3.795296366450300773, -2.154584498419360283, 14.16423886937410437 ) ) ;
#32431=ORIENTED_EDGE ( 'NONE', *, *, #89671, .F. ) ;
#32436=DIRECTION ( 'NONE',  ( -0.000000000000000000, -1.000000000000000000, -0.000000000000000000 ) ) ;
#32438=VECTOR ( 'NONE', #69548, 999.9999999999998863 ) ;
#32466=CARTESIAN_POINT ( 'NONE',  ( 10.93781366033340063, 0.5000000000000004441, 10.26470809774072634 ) ) ;
#32468=ORIENTED_EDGE ( 'NONE', *, *, #97807, .T. ) ;
#32478=ORIENTED_EDGE ( 'NONE', *, *, #9656, .F. ) ;
#32482=ORIENTED_EDGE ( 'NONE', *, *, #40571, .F. ) ;
#32483=ORIENTED_EDGE ( 'NONE', *, *, #79645, .F. ) ;
#32484=VECTOR ( 'NONE', #40417, 1000.000000000000000 ) ;
#32497=CARTESIAN_POINT ( 'NONE',  ( 8.527530157486179263, 28.09226448433413381, 4.923371831947292776 ) ) ;
#32499=LINE ( 'NONE', #93994, #62125 ) ;
#32507=EDGE_CURVE ( 'NONE', #59552, #52000, #27811, .T. ) ;
#32508=ADVANCED_FACE ( 'NONE', ( #11826 ), #64806, .T. ) ;
#32515=VERTEX_POINT ( 'NONE', #49328 ) ;
#32520=LINE ( 'NONE', #63018, #61841 ) ;
#32522=CARTESIAN_POINT ( 'NONE',  ( -5.056330833731569108, 4.047076681631624764E-16, -13.58983143750706724 ) ) ;
#32527=EDGE_CURVE ( 'NONE', #94433, #88013, #79344, .T. ) ;
#32536=DIRECTION ( 'NONE',  ( 0.4146932426562279228, 0.000000000000000000, 0.9099612708765483227 ) ) ;
#32537=CARTESIAN_POINT ( 'NONE',  ( -14.47650479471824880, 0.5000000000000004441, 3.928206833721914482 ) ) ;
#32546=FACE_OUTER_BOUND ( 'NONE', #49125, .T. ) ;
#32558=DIRECTION ( 'NONE',  ( 0.000000000000000000, 0.000000000000000000, 1.000000000000000000 ) ) ;
#32563=CARTESIAN_POINT ( 'NONE',  ( -9.422509992056145478, 2.647018677488177651, -5.440088680355541939 ) ) ;
#32567=EDGE_CURVE ( 'NONE', #27610, #96556, #17888, .T. ) ;
#32568=CARTESIAN_POINT ( 'NONE',  ( 0.000000000000000000, 0.5000000000000004441, 0.000000000000000000 ) ) ;
#32572=DIRECTION ( 'NONE',  ( 0.8433914458128849434, 0.000000000000000000, 0.5372996083468249973 ) ) ;
#32579=B_SPLINE_CURVE_WITH_KNOTS ( 'NONE', 3,
 ( #14715, #43208, #22211, #45190, #22704, #73702 ),
 .UNSPECIFIED., .F., .F.,
 ( 4, 2, 4 ),
 ( 0.0002800484630363999391, 0.0006862541666483241206, 0.001092459870260248465 ),
 .UNSPECIFIED. ) ;
#32600=B_SPLINE_CURVE_WITH_KNOTS ( 'NONE', 3,
 ( #35866, #28370, #51365, #58857, #81852, #5872 ),
 .UNSPECIFIED., .F., .F.,
 ( 4, 2, 4 ),
 ( 0.0002800245631444383903, 0.0006862300328522850414, 0.001092435502560131855 ),
 .UNSPECIFIED. ) ;
#32610=CARTESIAN_POINT ( 'NONE',  ( 3.469446951953614189E-15, -7.741068848999208107, 9.846743663894594434 ) ) ;
#32611=EDGE_LOOP ( 'NONE', ( #93359, #61012, #56981, #6879, #96001, #22156 ) ) ;
#32612=DIRECTION ( 'NONE',  ( 0.3987490689252528031, 0.000000000000000000, -0.9170600743851211600 ) ) ;
#32615=VERTEX_POINT ( 'NONE', #86361 ) ;
#32621=CYLINDRICAL_SURFACE ( 'NONE', #73414, 15.00000000000000000 ) ;
#32622=EDGE_CURVE ( 'NONE', #17080, #60216, #819, .T. ) ;
#32623=EDGE_CURVE ( 'NONE', #35666, #29544, #65305, .T. ) ;
#32627=ORIENTED_EDGE ( 'NONE', *, *, #31485, .T. ) ;
#32632=B_SPLINE_CURVE_WITH_KNOTS ( 'NONE', 3,
 ( #71432, #2946, #9436, #85938, #78421, #17930 ),
 .UNSPECIFIED., .F., .F.,
 ( 4, 2, 4 ),
 ( 0.0002800015744458416345, 0.0006862068192651665267, 0.001092412064084491473 ),
 .UNSPECIFIED. ) ;
#32641=DIRECTION ( 'NONE',  ( 0.000000000000000000, 1.000000000000000000, 0.000000000000000000 ) ) ;
#32642=ORIENTED_EDGE ( 'NONE', *, *, #60181, .T. ) ;
#32656=EDGE_LOOP ( 'NONE', ( #23084, #62526, #57974, #9335, #79236, #41869 ) ) ;
#32663=VECTOR ( 'NONE', #54814, 1000.000000000000000 ) ;
#32674=CARTESIAN_POINT ( 'NONE',  ( -12.26659068614894110, 32.22041550158063927, 7.082119434687058401 ) ) ;
#32690=DIRECTION ( 'NONE',  ( 0.000000000000000000, 0.000000000000000000, 1.000000000000000000 ) ) ;
#32691=DIRECTION ( 'NONE',  ( 0.000000000000000000, 1.000000000000000000, 0.000000000000000000 ) ) ;
#32696=CARTESIAN_POINT ( 'NONE',  ( 0.000000000000000000, -0.03417435944610275333, 14.25000000000000000 ) ) ;
#32718=CARTESIAN_POINT ( 'NONE',  ( 0.000000000000000000, 0.5000000000000004441, 0.000000000000000000 ) ) ;
#32723=CARTESIAN_POINT ( 'NONE',  ( -11.35178980618984568, 14.63606909211651264, 9.804941009311860967 ) ) ;
#32728=DIRECTION ( 'NONE',  ( 0.9914448613738084948, 0.000000000000000000, 0.1305261922200653124 ) ) ;
#32735=CARTESIAN_POINT ( 'NONE',  ( 14.71525861348288799, 0.3640475087720990710, 2.908807992686685218 ) ) ;
#32736=EDGE_CURVE ( 'NONE', #63206, #75691, #18687, .T. ) ;
#32739=FACE_OUTER_BOUND ( 'NONE', #21977, .T. ) ;
#32741=ADVANCED_FACE ( 'NONE', ( #54780 ), #61301, .T. ) ;
#32743=CARTESIAN_POINT ( 'NONE',  ( 9.382169495545419124, -9.001365330069580395, 9.382169495545417348 ) ) ;
#32752=ORIENTED_EDGE ( 'NONE', *, *, #65812, .T. ) ;
#32754=CARTESIAN_POINT ( 'NONE',  ( -6.189940676892205396, 14.95037117674007376, 13.39186120658999357 ) ) ;
#32755=VECTOR ( 'NONE', #94677, 1000.000000000000000 ) ;
#32757=DIRECTION ( 'NONE',  ( 0.000000000000000000, 1.000000000000000000, 0.000000000000000000 ) ) ;
#32761=FACE_OUTER_BOUND ( 'NONE', #74939, .T. ) ;
#32762=TOROIDAL_SURFACE ( 'NONE', #69549, 14.49999999999999822, 0.5000000000000000000 ) ;
#32764=LINE ( 'NONE', #41285, #18601 ) ;
#32778=CARTESIAN_POINT ( 'NONE',  ( -0.9082943533635161604, 4.683954948888111413E-16, -14.47152380945586359 ) ) ;
#32786=FACE_OUTER_BOUND ( 'NONE', #11138, .T. ) ;
#32797=ORIENTED_EDGE ( 'NONE', *, *, #50672, .T. ) ;
#32798=VECTOR ( 'NONE', #9448, 1000.000000000000000 ) ;
#32801=CARTESIAN_POINT ( 'NONE',  ( 0.000000000000000000, 0.000000000000000000, 0.000000000000000000 ) ) ;
#32804=CARTESIAN_POINT ( 'NONE',  ( 5.419894505350532299, 14.49999999999999112, 13.98659156302467466 ) ) ;
#32816=PLANE ( 'NONE',  #36884 ) ;
#32823=AXIS2_PLACEMENT_3D ( 'NONE', #80261, #28733, #89728 ) ;
#32852=DIRECTION ( 'NONE',  ( -0.000000000000000000, 1.000000000000000000, -0.000000000000000000 ) ) ;
#32853=VECTOR ( 'NONE', #45334, 1000.000000000000114 ) ;
#32854=CARTESIAN_POINT ( 'NONE',  ( 14.56332774647473904, 0.04922511925146993983, -2.357028871694184513 ) ) ;
#32855=DIRECTION ( 'NONE',  ( -0.000000000000000000, -1.000000000000000000, -0.000000000000000000 ) ) ;
#32864=VERTEX_POINT ( 'NONE', #24315 ) ;
#32869=CARTESIAN_POINT ( 'NONE',  ( -13.75503023589414830, 0.04922511925147124434, 5.333408231410639466 ) ) ;
#32876=ORIENTED_EDGE ( 'NONE', *, *, #76553, .T. ) ;
#32880=ORIENTED_EDGE ( 'NONE', *, *, #2629, .F. ) ;
#32886=DIRECTION ( 'NONE',  ( 0.000000000000000000, 0.000000000000000000, 1.000000000000000000 ) ) ;
#32890=AXIS2_PLACEMENT_3D ( 'NONE', #59621, #61588, #22136 ) ;
#32891=PLANE ( 'NONE',  #43611 ) ;
#32893=CARTESIAN_POINT ( 'NONE',  ( 0.7375392941517191492, 0.3640475087720981828, 14.98185688723472353 ) ) ;
#32894=DIRECTION ( 'NONE',  ( 0.000000000000000000, 0.000000000000000000, 1.000000000000000000 ) ) ;
#32898=CARTESIAN_POINT ( 'NONE',  ( 13.78891971893208357, 14.49999999999999822, -5.904717858191528279 ) ) ;
#32902=VERTEX_POINT ( 'NONE', #22835 ) ;
#32914=ORIENTED_EDGE ( 'NONE', *, *, #95950, .T. ) ;
#32916=CARTESIAN_POINT ( 'NONE',  ( 0.000000000000000000, 0.000000000000000000, 0.000000000000000000 ) ) ;
#32920=CARTESIAN_POINT ( 'NONE',  ( 3.795296366450306547, 5.345415501580633943, -14.16423886937410259 ) ) ;
#32928=CARTESIAN_POINT ( 'NONE',  ( -6.189940676891933613, 0.04962882325992939991, -13.39186120659011614 ) ) ;
#32931=DIRECTION ( 'NONE',  ( -0.000000000000000000, -1.000000000000000000, -0.000000000000000000 ) ) ;
#32935=CARTESIAN_POINT ( 'NONE',  ( -14.99847009497944583, 15.00000000000000000, 0.2142307401079343032 ) ) ;
#32943=EDGE_CURVE ( 'NONE', #73495, #18004, #37020, .T. ) ;
#32953=DIRECTION ( 'NONE',  ( -0.000000000000000000, -1.000000000000000000, -0.000000000000000000 ) ) ;
#32957=LINE ( 'NONE', #56937, #14287 ) ;
#32969=ORIENTED_EDGE ( 'NONE', *, *, #91547, .F. ) ;
#32970=ORIENTED_EDGE ( 'NONE', *, *, #58486, .T. ) ;
#32975=CARTESIAN_POINT ( 'NONE',  ( 10.58981376305288613, 15.00000000000000000, -9.535111140613709679 ) ) ;
#32986=CARTESIAN_POINT ( 'NONE',  ( 9.846743663894594434, 23.50893115100079100, -2.168404344971008868E-15 ) ) ;
#32987=ORIENTED_EDGE ( 'NONE', *, *, #34089, .T. ) ;
#32988=CARTESIAN_POINT ( 'NONE',  ( 5.795997163830165277, 15.00000000000000000, -13.01802277140705932 ) ) ;
#32995=VECTOR ( 'NONE', #40808, 1000.000000000000000 ) ;
#32998=CIRCLE ( 'NONE', #63323, 14.49999999999999822 ) ;
#33002=VERTEX_POINT ( 'NONE', #87738 ) ;
#33006=EDGE_LOOP ( 'NONE', ( #53552, #9714, #68153, #34092 ) ) ;
#33008=FACE_OUTER_BOUND ( 'NONE', #13806, .T. ) ;
#33017=CARTESIAN_POINT ( 'NONE',  ( 14.36383853300405988, 0.04962896932678220047, 3.367113227849034551 ) ) ;
#33018=AXIS2_PLACEMENT_3D ( 'NONE', #36497, #5515, #35992 ) ;
#33021=ORIENTED_EDGE ( 'NONE', *, *, #26972, .F. ) ;
#33022=DIRECTION ( 'NONE',  ( -0.000000000000000000, 1.000000000000000000, -0.000000000000000000 ) ) ;
#33027=CARTESIAN_POINT ( 'NONE',  ( 1.087200977610002450, 0.000000000000000000, -5.343763529286909453 ) ) ;
#33040=ORIENTED_EDGE ( 'NONE', *, *, #98157, .F. ) ;
#33047=DIRECTION ( 'NONE',  ( -0.000000000000000000, 1.000000000000000000, 0.000000000000000000 ) ) ;
#33049=CARTESIAN_POINT ( 'NONE',  ( 0.000000000000000000, 15.00000000000000000, 0.000000000000000000 ) ) ;
#33052=CARTESIAN_POINT ( 'NONE',  ( 9.422509992056141925, 5.147018677488180316, 5.440088680355547268 ) ) ;
#33056=EDGE_CURVE ( 'NONE', #40528, #95502, #59217, .T. ) ;
#33058=CARTESIAN_POINT ( 'NONE',  ( -13.61464873478178284, 14.49999999999999112, 6.296136897217746942 ) ) ;
#33069=CARTESIAN_POINT ( 'NONE',  ( 0.000000000000000000, 0.5000000000000004441, 0.000000000000000000 ) ) ;
#33071=VERTEX_POINT ( 'NONE', #71764 ) ;
#33082=AXIS2_PLACEMENT_3D ( 'NONE', #95480, #26971, #57469 ) ;
#33086=VECTOR ( 'NONE', #96326, 1000.000000000000000 ) ;
#33087=ORIENTED_EDGE ( 'NONE', *, *, #55445, .F. ) ;
#33090=EDGE_CURVE ( 'NONE', #72566, #59600, #17790, .T. ) ;
#33098=EDGE_CURVE ( 'NONE', #18747, #69558, #3389, .T. ) ;
#33099=CARTESIAN_POINT ( 'NONE',  ( 10.17177286909470624, 0.2301502795151879610, -10.94336654633681327 ) ) ;
#33101=CARTESIAN_POINT ( 'NONE',  ( 9.846743663894590881, -6.282735515665877735, -2.638427012816833894 ) ) ;
#33104=VERTEX_POINT ( 'NONE', #26745 ) ;
#33111=CARTESIAN_POINT ( 'NONE',  ( -13.86102707272217494, 15.00000000000000711, -4.666951904077385471 ) ) ;
#33113=CARTESIAN_POINT ( 'NONE',  ( -11.09922568453595382, 28.70696800326377840, -6.408140936763226492 ) ) ;
#33114=VERTEX_POINT ( 'NONE', #57729 ) ;
#33124=EDGE_CURVE ( 'NONE', #12575, #30635, #11254, .T. ) ;
#33125=TOROIDAL_SURFACE ( 'NONE', #41149, 14.49999999999999822, 0.5000000000000000000 ) ;
#33131=CARTESIAN_POINT ( 'NONE',  ( -14.66196617519555545, 0.2306972965111886154, -2.874856965128016473 ) ) ;
#33138=CARTESIAN_POINT ( 'NONE',  ( 11.96291822454875842, 15.00000000000000000, 8.193813980849165901 ) ) ;
#33140=CARTESIAN_POINT ( 'NONE',  ( 14.15281240980445077, 15.00000000000000178, 3.688687068602797492 ) ) ;
#33146=VECTOR ( 'NONE', #47588, 1000.000000000000000 ) ;
#33149=VECTOR ( 'NONE', #82661, 999.9999999999998863 ) ;
#33153=DIRECTION ( 'NONE',  ( -0.000000000000000000, -1.000000000000000000, -0.000000000000000000 ) ) ;
#33157=CARTESIAN_POINT ( 'NONE',  ( -13.61464873478158211, 0.5000000000000004441, -6.296136897218027606 ) ) ;
#33158=CARTESIAN_POINT ( 'NONE',  ( 0.000000000000000000, 14.49999999999999822, 0.000000000000000000 ) ) ;
#33162=B_SPLINE_CURVE_WITH_KNOTS ( 'NONE', 3,
 ( #8785, #1322, #82812, #53299, #98344, #38803 ),
 .UNSPECIFIED., .F., .F.,
 ( 4, 2, 4 ),
 ( 3.409110551482055714E-05, 0.0004400426677366462216, 0.0008459942299584719471 ),
 .UNSPECIFIED. ) ;
#33163=CARTESIAN_POINT ( 'NONE',  ( -7.964842623401179544, -37.56131465584516604, -7.964842623401174215 ) ) ;
#33167=PLANE ( 'NONE',  #58015 ) ;
#33175=B_SPLINE_CURVE_WITH_KNOTS ( 'NONE', 3,
 ( #40619, #8636, #85129, #16640, #78613, #63104 ),
 .UNSPECIFIED., .F., .F.,
 ( 4, 2, 4 ),
 ( 3.409110551496089355E-05, 0.0004400426677367838069, 0.0008459942299586067135 ),
 .UNSPECIFIED. ) ;
#33182=CARTESIAN_POINT ( 'NONE',  ( -2.120353041430432128, 15.00000000000000000, -14.34413130794946234 ) ) ;
#33188=PLANE ( 'NONE',  #98830 ) ;
#33195=FACE_OUTER_BOUND ( 'NONE', #83792, .T. ) ;
#33198=CARTESIAN_POINT ( 'NONE',  ( 7.882504294823842628, 15.00000000000000711, 12.32089577884796050 ) ) ;
#33201=LINE ( 'NONE', #35165, #80476 ) ;
#33211=CARTESIAN_POINT ( 'NONE',  ( 11.10136736363534560, 0.04922511925147036310, -9.716261771424912652 ) ) ;
#33213=DIRECTION ( 'NONE',  ( -0.9025852843498618494, 0.000000000000000000, 0.4305110968082926926 ) ) ;
#33220=ORIENTED_EDGE ( 'NONE', *, *, #17437, .F. ) ;
#33221=VERTEX_POINT ( 'NONE', #19741 ) ;
#33223=ORIENTED_EDGE ( 'NONE', *, *, #16283, .T. ) ;
#33229=ORIENTED_EDGE ( 'NONE', *, *, #52279, .F. ) ;
#33232=DIRECTION ( 'NONE',  ( 0.8788171126619646056, -0.000000000000000000, 0.4771587602596096267 ) ) ;
#33233=CARTESIAN_POINT ( 'NONE',  ( -12.81628187352647963, -1.084698663402915653, -3.434112377981046293 ) ) ;
#33248=DIRECTION ( 'NONE',  ( 0.5664062369248205053, 0.000000000000000000, 0.8241261886220241362 ) ) ;
#33254=EDGE_CURVE ( 'NONE', #11366, #95706, #46554, .T. ) ;
#33273=CARTESIAN_POINT ( 'NONE',  ( -7.551349515323269479, -0.03417435944610275333, 12.08468537022900868 ) ) ;
#33283=CARTESIAN_POINT ( 'NONE',  ( -12.34557190004669458, 14.95077488074853456, -8.076692058882660064 ) ) ;
#33284=EDGE_CURVE ( 'NONE', #24535, #23105, #80659, .T. ) ;
#33288=ORIENTED_EDGE ( 'NONE', *, *, #7658, .T. ) ;
#33290=ADVANCED_FACE ( 'NONE', ( #82710 ), #54052, .F. ) ;
#33292=DIRECTION ( 'NONE',  ( 0.000000000000000000, 0.000000000000000000, 1.000000000000000000 ) ) ;
#33296=DIRECTION ( 'NONE',  ( 0.000000000000000000, 1.000000000000000000, 0.000000000000000000 ) ) ;
#33301=CARTESIAN_POINT ( 'NONE',  ( 2.863845842055925406, 14.95077488074853456, -14.47219703936412927 ) ) ;
#33307=CARTESIAN_POINT ( 'NONE',  ( -7.684764310694706779, 0.3640475087720986269, -12.88194075009946182 ) ) ;
#33319=DIRECTION ( 'NONE',  ( -0.8433914458128813907, 0.000000000000000000, -0.5372996083468306594 ) ) ;
#33326=EDGE_CURVE ( 'NONE', #69120, #80329, #50741, .T. ) ;
#33332=ORIENTED_EDGE ( 'NONE', *, *, #66504, .T. ) ;
#33358=DIRECTION ( 'NONE',  ( -0.000000000000000000, -1.000000000000000000, -0.000000000000000000 ) ) ;
#33359=ORIENTED_EDGE ( 'NONE', *, *, #96875, .T. ) ;
#33368=CARTESIAN_POINT ( 'NONE',  ( 10.39692778084940272, 14.95037106203290911, -10.46714871971199301 ) ) ;
#33369=LINE ( 'NONE', #62392, #39493 ) ;
#33371=FACE_OUTER_BOUND ( 'NONE', #55861, .T. ) ;
#33376=ORIENTED_EDGE ( 'NONE', *, *, #48758, .F. ) ;
#33380=CARTESIAN_POINT ( 'NONE',  ( -4.267749253172059554, 0.000000000000000000, -3.394721039305347077 ) ) ;
#33384=CARTESIAN_POINT ( 'NONE',  ( -1.514341385896341929, -0.03417435944610275333, -15.92432625271835533 ) ) ;
#33391=DIRECTION ( 'NONE',  ( 0.000000000000000000, 0.000000000000000000, 1.000000000000000000 ) ) ;
#33398=CARTESIAN_POINT ( 'NONE',  ( -5.204170427930421283E-15, 0.5537488349139709776, -14.16423886937410082 ) ) ;
#33412=CARTESIAN_POINT ( 'NONE',  ( 10.39655283154085197, 0.04922511925147234763, -10.46698568711264699 ) ) ;
#33414=FACE_OUTER_BOUND ( 'NONE', #70119, .T. ) ;
#33433=CARTESIAN_POINT ( 'NONE',  ( -5.803070148808146200, 15.00000000000000000, -13.28812917035395813 ) ) ;
#33440=EDGE_CURVE ( 'NONE', #3959, #36305, #49647, .T. ) ;
#33450=CARTESIAN_POINT ( 'NONE',  ( 9.399392868737743711, 4.718572659598065102E-16, 11.04089732309480532 ) ) ;
#33455=CARTESIAN_POINT ( 'NONE',  ( 0.000000000000000000, 0.000000000000000000, 0.000000000000000000 ) ) ;
#33465=CARTESIAN_POINT ( 'NONE',  ( -9.382169495545413795, -30.25136533006957507, 9.382169495545428006 ) ) ;
#33467=CIRCLE ( 'NONE', #43054, 15.00000000000000000 ) ;
#33475=DIRECTION ( 'NONE',  ( 0.000000000000000000, 0.000000000000000000, -1.000000000000000000 ) ) ;
#33478=ORIENTED_EDGE ( 'NONE', *, *, #59394, .F. ) ;
#33483=CARTESIAN_POINT ( 'NONE',  ( 14.61146088927471176, 15.00000000000000888, -0.6660010753334455469 ) ) ;
#33484=LINE ( 'NONE', #62515, #32438 ) ;
#33489=ADVANCED_FACE ( 'NONE', ( #72142 ), #80641, .F. ) ;
#33491=CARTESIAN_POINT ( 'NONE',  ( -5.204170427930421283E-15, 11.67180217785154817, -11.25000000000000178 ) ) ;
#33494=EDGE_LOOP ( 'NONE', ( #29688, #29561, #84037, #8737 ) ) ;
#33497=EDGE_LOOP ( 'NONE', ( #44578, #83017, #64063, #61964, #94948, #56162 ) ) ;
#33498=EDGE_LOOP ( 'NONE', ( #64956, #21456, #3099, #54519 ) ) ;
#33505=DIRECTION ( 'NONE',  ( 0.000000000000000000, 0.000000000000000000, 1.000000000000000000 ) ) ;
#33516=VECTOR ( 'NONE', #5466, 1000.000000000000000 ) ;
#33520=CARTESIAN_POINT ( 'NONE',  ( -7.082119434687058401, -39.02958449841936073, -12.26659068614894110 ) ) ;
#33525=EDGE_CURVE ( 'NONE', #42002, #7455, #64136, .T. ) ;
#33531=LINE ( 'NONE', #79042, #25723 ) ;
#33537=CARTESIAN_POINT ( 'NONE',  ( -5.204170427930421283E-15, 11.81368534415484817, -10.88017736071110342 ) ) ;
#33540=DIRECTION ( 'NONE',  ( 0.000000000000000000, 1.000000000000000000, 0.000000000000000000 ) ) ;
#33541=LINE ( 'NONE', #64035, #84903 ) ;
#33542=DIRECTION ( 'NONE',  ( 0.2840153447039108769, 0.000000000000000000, 0.9588197348681966048 ) ) ;
#33545=CARTESIAN_POINT ( 'NONE',  ( -12.60589901313216998, 14.49999999999999112, -8.129656208642240145 ) ) ;
#33546=DIRECTION ( 'NONE',  ( -0.000000000000000000, 1.000000000000000000, 0.000000000000000000 ) ) ;
#33564=DIRECTION ( 'NONE',  ( 0.000000000000000000, 0.000000000000000000, 1.000000000000000000 ) ) ;
#33570=VERTEX_POINT ( 'NONE', #75602 ) ;
#33575=DIRECTION ( 'NONE',  ( -0.000000000000000000, -1.000000000000000000, -0.000000000000000000 ) ) ;
#33582=CARTESIAN_POINT ( 'NONE',  ( 4.923371831947295441, 9.342264484334124930, -8.527530157486179263 ) ) ;
#33588=ORIENTED_EDGE ( 'NONE', *, *, #57686, .F. ) ;
#33598=B_SPLINE_CURVE_WITH_KNOTS ( 'NONE', 3,
 ( #38710, #15729, #75216, #30201, #61682, #22729 ),
 .UNSPECIFIED., .F., .F.,
 ( 4, 2, 4 ),
 ( 3.409110551496108329E-05, 0.0004400426677367840237, 0.0008459942299586070387 ),
 .UNSPECIFIED. ) ;
#33601=EDGE_LOOP ( 'NONE', ( #3125, #23701, #8992, #75660 ) ) ;
#33603=AXIS2_PLACEMENT_3D ( 'NONE', #5150, #88632, #48664 ) ;
#33609=B_SPLINE_CURVE_WITH_KNOTS ( 'NONE', 3,
 ( #438, #61385, #76399, #9377, #23906, #84406 ),
 .UNSPECIFIED., .F., .F.,
 ( 4, 2, 4 ),
 ( 0.0002800630492131323673, 0.0006862688956284098384, 0.001092474742043687309 ),
 .UNSPECIFIED. ) ;
#33610=FACE_OUTER_BOUND ( 'NONE', #16561, .T. ) ;
#33613=ORIENTED_EDGE ( 'NONE', *, *, #83129, .T. ) ;
#33616=LINE ( 'NONE', #87120, #70787 ) ;
#33622=ORIENTED_EDGE ( 'NONE', *, *, #90191, .F. ) ;
#33628=CARTESIAN_POINT ( 'NONE',  ( -10.64017930668192058, 14.63595249122789177, -10.57291749337230868 ) ) ;
#33630=CARTESIAN_POINT ( 'NONE',  ( 14.29730467489533652, 15.00000000000000000, -2.416004766803220072 ) ) ;
#33632=EDGE_CURVE ( 'NONE', #48866, #32363, #19276, .T. ) ;
#33634=ORIENTED_EDGE ( 'NONE', *, *, #18349, .T. ) ;
#33635=ADVANCED_FACE ( 'NONE', ( #58113 ), #66622, .F. ) ;
#33638=VECTOR ( 'NONE', #39363, 1000.000000000000114 ) ;
#33640=CARTESIAN_POINT ( 'NONE',  ( 3.840373378095567336, 13.17686044187654559, -11.29165764256138260 ) ) ;
#33647=CARTESIAN_POINT ( 'NONE',  ( -14.16423886937410082, 26.80374883491398919, 4.336808689942017736E-15 ) ) ;
#33668=EDGE_LOOP ( 'NONE', ( #47264, #76003, #31252, #75178, #72537, #45835 ) ) ;
#33676=CARTESIAN_POINT ( 'NONE',  ( 14.03351048042395632, 15.00000000000000000, 2.474486531753810059 ) ) ;
#33680=CARTESIAN_POINT ( 'NONE',  ( 1.457314710996591600, 0.000000000000000000, -5.254907083456943795 ) ) ;
#33681=VERTEX_POINT ( 'NONE', #97639 ) ;
#33682=ORIENTED_EDGE ( 'NONE', *, *, #90448, .F. ) ;
#33683=VECTOR ( 'NONE', #21509, 1000.000000000000000 ) ;
#33695=DIRECTION ( 'NONE',  ( -0.000000000000000000, -1.000000000000000000, -0.000000000000000000 ) ) ;
#33696=CARTESIAN_POINT ( 'NONE',  ( 0.7375392941518260637, 14.63595249122790065, -14.98185688723471287 ) ) ;
#33700=ORIENTED_EDGE ( 'NONE', *, *, #48004, .F. ) ;
#33705=VERTEX_POINT ( 'NONE', #97149 ) ;
#33709=DIRECTION ( 'NONE',  ( -0.000000000000000000, -1.000000000000000000, -0.000000000000000000 ) ) ;
#33713=CARTESIAN_POINT ( 'NONE',  ( 11.09922568453595026, -3.793031996736244249, 6.408140936763232709 ) ) ;
#33714=ORIENTED_EDGE ( 'NONE', *, *, #28997, .F. ) ;
#33722=DIRECTION ( 'NONE',  ( -0.000000000000000000, -1.000000000000000000, -0.000000000000000000 ) ) ;
#33724=ADVANCED_FACE ( 'NONE', ( #52115 ), #79946, .T. ) ;
#33726=CARTESIAN_POINT ( 'NONE',  ( 14.71525861348291286, 14.63595249122789177, -2.908807992686589294 ) ) ;
#33729=DIRECTION ( 'NONE',  ( -0.000000000000000000, -1.000000000000000000, -0.000000000000000000 ) ) ;
#33733=CARTESIAN_POINT ( 'NONE',  ( -6.767445849361073407, 14.49999999999999112, -13.38662304974512729 ) ) ;
#33741=CARTESIAN_POINT ( 'NONE',  ( 9.399392868737814766, 4.153235915537064750E-16, -11.04089732309474314 ) ) ;
#33750=ORIENTED_EDGE ( 'NONE', *, *, #30483, .T. ) ;
#33761=CARTESIAN_POINT ( 'NONE',  ( -0.2850016562179802371, 14.76967010231060762, -14.93805486374025193 ) ) ;
#33764=ORIENTED_EDGE ( 'NONE', *, *, #78386, .T. ) ;
#33767=CARTESIAN_POINT ( 'NONE',  ( -13.48086198287156101, -0.03417435944610275333, -8.610676897597642210 ) ) ;
#33772=CARTESIAN_POINT ( 'NONE',  ( 11.22915323889574601, -0.03417435944610275333, 8.773176023390684364 ) ) ;
#33777=CARTESIAN_POINT ( 'NONE',  ( 10.58981376305282041, 15.00000000000000000, 9.535111140613782510 ) ) ;
#33783=EDGE_CURVE ( 'NONE', #325, #98695, #57597, .T. ) ;
#33786=CARTESIAN_POINT ( 'NONE',  ( -14.22901244993688152, 6.166399856011304496E-16, 3.387263120971218289 ) ) ;
#33789=CIRCLE ( 'NONE', #59349, 14.49999999999999822 ) ;
#33793=EDGE_CURVE ( 'NONE', #44015, #43096, #47568, .T. ) ;
#33813=CARTESIAN_POINT ( 'NONE',  ( 13.61464873478173843, 14.49999999999999112, -6.296136897217843753 ) ) ;
#33818=AXIS2_PLACEMENT_3D ( 'NONE', #36178, #50185, #57193 ) ;
#33823=B_SPLINE_CURVE_WITH_KNOTS ( 'NONE', 3,
 ( #70910, #54405, #63386, #1935, #85410, #15933 ),
 .UNSPECIFIED., .F., .F.,
 ( 4, 2, 4 ),
 ( 0.0002800001171688671947, 0.0006862053477355151403, 0.001092410578302163140 ),
 .UNSPECIFIED. ) ;
#33834=CARTESIAN_POINT ( 'NONE',  ( -2.393480905992944496, 15.00000000000000000, -14.80781041047754520 ) ) ;
#33840=CARTESIAN_POINT ( 'NONE',  ( 0.000000000000000000, 15.00000000000000000, 0.000000000000000000 ) ) ;
#33841=EDGE_CURVE ( 'NONE', #59170, #71199, #17729, .T. ) ;
#33855=CARTESIAN_POINT ( 'NONE',  ( -12.87890026492928541, 14.95077488074853456, -7.195834080858529269 ) ) ;
#33857=CARTESIAN_POINT ( 'NONE',  ( -10.84451454130491399, 15.00000000000000000, -9.625305416630974165 ) ) ;
#33858=CARTESIAN_POINT ( 'NONE',  ( 0.000000000000000000, 0.5000000000000004441, 0.000000000000000000 ) ) ;
#33861=AXIS2_PLACEMENT_3D ( 'NONE', #78813, #33296, #94296 ) ;
#33862=B_SPLINE_CURVE_WITH_KNOTS ( 'NONE', 3,
 ( #10902, #79880, #79396, #41907, #25905, #86893 ),
 .UNSPECIFIED., .F., .F.,
 ( 4, 2, 4 ),
 ( 0.0002800001171688651347, 0.0006862053477355225129, 0.001092410578302179837 ),
 .UNSPECIFIED. ) ;
#33865=EDGE_CURVE ( 'NONE', #43087, #68316, #24093, .T. ) ;
#33867=CARTESIAN_POINT ( 'NONE',  ( -1.780824192092276048, 14.49999999999999112, -14.89391369643522545 ) ) ;
#33878=DIRECTION ( 'NONE',  ( 0.8241261886220204724, 0.000000000000000000, -0.5664062369248259454 ) ) ;
#33879=CARTESIAN_POINT ( 'NONE',  ( 0.000000000000000000, 15.00000000000000000, 0.000000000000000000 ) ) ;
#33885=FACE_OUTER_BOUND ( 'NONE', #78584, .T. ) ;
#33886=CARTESIAN_POINT ( 'NONE',  ( 10.36894250292378850, 4.928748834913970533, -10.36894250292379027 ) ) ;
#33894=CARTESIAN_POINT ( 'NONE',  ( -10.70613742633244669, 15.00000000000000000, -9.778988772285387654 ) ) ;
#33897=CARTESIAN_POINT ( 'NONE',  ( 3.836325488036183451, 0.5000000000000004441, -14.50112432709422627 ) ) ;
#33911=ORIENTED_EDGE ( 'NONE', *, *, #51830, .F. ) ;
#33922=CIRCLE ( 'NONE', #59494, 15.00000000000000000 ) ;
#33923=VERTEX_POINT ( 'NONE', #84591 ) ;
#33931=EDGE_LOOP ( 'NONE', ( #52152, #34193, #76285, #39256, #50267, #71037 ) ) ;
#33932=VECTOR ( 'NONE', #3305, 1000.000000000000000 ) ;
#33935=DIRECTION ( 'NONE',  ( 0.000000000000000000, 1.000000000000000000, -0.000000000000000000 ) ) ;
#33943=CARTESIAN_POINT ( 'NONE',  ( -7.551349515323020789, 15.00000000000000000, -12.08468537022916323 ) ) ;
#33953=CARTESIAN_POINT ( 'NONE',  ( -12.81628187352647252, -30.66803199673624292, 3.434112377981066722 ) ) ;
#33962=FACE_OUTER_BOUND ( 'NONE', #89585, .T. ) ;
#33966=EDGE_CURVE ( 'NONE', #42118, #97832, #75881, .T. ) ;
#33972=CARTESIAN_POINT ( 'NONE',  ( -5.795997163830251431, 0.000000000000000000, 13.01802277140702024 ) ) ;
#33978=CARTESIAN_POINT ( 'NONE',  ( -5.147851794455697849, -3.098870037529856607E-15, -13.68970903997134236 ) ) ;
#33983=CARTESIAN_POINT ( 'NONE',  ( 14.09394518620612224, 3.883508853191620072E-16, -3.407449058785360752 ) ) ;
#33991=CIRCLE ( 'NONE', #49998, 15.00000000000000000 ) ;
#33993=ADVANCED_FACE ( 'NONE', ( #70572 ), #94539, .F. ) ;
#33998=CARTESIAN_POINT ( 'NONE',  ( -12.80781515976318907, -0.03417435944610275333, 6.246788841744232990 ) ) ;
#34012=CARTESIAN_POINT ( 'NONE',  ( -3.927832320392339316, 0.000000000000000000, 13.69797916712101404 ) ) ;
#34015=ORIENTED_EDGE ( 'NONE', *, *, #38300, .T. ) ;
#34021=CARTESIAN_POINT ( 'NONE',  ( 14.62617646268092209, 14.49999999999999112, 3.327906561566971622 ) ) ;
#34024=DIRECTION ( 'NONE',  ( -1.048050535246147774E-13, 0.000000000000000000, 1.000000000000000000 ) ) ;
#34028=CARTESIAN_POINT ( 'NONE',  ( -2.915334737309917656, 14.10535201082150714, 10.88017736071110164 ) ) ;
#34031=DIRECTION ( 'NONE',  ( 0.000000000000000000, 0.000000000000000000, -1.000000000000000000 ) ) ;
#34032=FACE_OUTER_BOUND ( 'NONE', #40127, .T. ) ;
#34036=CARTESIAN_POINT ( 'NONE',  ( 0.000000000000000000, 15.00000000000000000, 0.000000000000000000 ) ) ;
#34055=EDGE_CURVE ( 'NONE', #64180, #57542, #2592, .T. ) ;
#34058=VERTEX_POINT ( 'NONE', #63542 ) ;
#34059=ORIENTED_EDGE ( 'NONE', *, *, #44238, .F. ) ;
#34064=DIRECTION ( 'NONE',  ( -0.7933533402912367194, 0.000000000000000000, 0.6087614290087187685 ) ) ;
#34073=VECTOR ( 'NONE', #18954, 1000.000000000000114 ) ;
#34074=CARTESIAN_POINT ( 'NONE',  ( -7.208316651077764980, 5.383931151000783899, -7.208316651077759651 ) ) ;
#34075=ORIENTED_EDGE ( 'NONE', *, *, #97402, .T. ) ;
#34078=VECTOR ( 'NONE', #27728, 1000.000000000000000 ) ;
#34089=EDGE_CURVE ( 'NONE', #13116, #44015, #33531, .T. ) ;
#34092=ORIENTED_EDGE ( 'NONE', *, *, #59394, .T. ) ;
#34104=ORIENTED_EDGE ( 'NONE', *, *, #47623, .F. ) ;
#34107=FACE_OUTER_BOUND ( 'NONE', #95811, .T. ) ;
#34109=EDGE_CURVE ( 'NONE', #49327, #2489, #92725, .T. ) ;
#34110=DIRECTION ( 'NONE',  ( 0.000000000000000000, 1.000000000000000000, 0.000000000000000000 ) ) ;
#34116=LINE ( 'NONE', #57121, #61059 ) ;
#34117=ORIENTED_EDGE ( 'NONE', *, *, #59868, .T. ) ;
#34118=DIRECTION ( 'NONE',  ( -0.000000000000000000, -1.000000000000000000, -0.000000000000000000 ) ) ;
#34125=LINE ( 'NONE', #95127, #25171 ) ;
#34129=DIRECTION ( 'NONE',  ( -0.9953961983671791858, 0.000000000000000000, 0.09584575252022038694 ) ) ;
#34138=CARTESIAN_POINT ( 'NONE',  ( 5.440088680355549045, -18.60298132251182324, -9.422509992056141925 ) ) ;
#34143=CARTESIAN_POINT ( 'NONE',  ( 0.000000000000000000, 0.5000000000000004441, 0.000000000000000000 ) ) ;
#34153=DIRECTION ( 'NONE',  ( 0.000000000000000000, 0.000000000000000000, 1.000000000000000000 ) ) ;
#34159=ORIENTED_EDGE ( 'NONE', *, *, #51023, .T. ) ;
#34160=DIRECTION ( 'NONE',  ( 0.000000000000000000, 1.000000000000000000, 0.000000000000000000 ) ) ;
#34165=EDGE_CURVE ( 'NONE', #935, #67657, #20889, .T. ) ;
#34169=CARTESIAN_POINT ( 'NONE',  ( 0.000000000000000000, 0.000000000000000000, 0.000000000000000000 ) ) ;
#34172=ORIENTED_EDGE ( 'NONE', *, *, #85151, .F. ) ;
#34173=CARTESIAN_POINT ( 'NONE',  ( -4.838527690343430443, 0.5000000000000004441, -14.19819177887733375 ) ) ;
#34174=ORIENTED_EDGE ( 'NONE', *, *, #98116, .F. ) ;
#34176=DIRECTION ( 'NONE',  ( 0.2334453638559155775, 0.000000000000000000, -0.9723699203976741146 ) ) ;
#34192=CARTESIAN_POINT ( 'NONE',  ( 3.469446951953614189E-15, -37.74106884899921255, 9.846743663894594434 ) ) ;
#34193=ORIENTED_EDGE ( 'NONE', *, *, #48499, .T. ) ;
#34197=EDGE_LOOP ( 'NONE', ( #68514, #63608, #23184, #82740, #37807, #4793 ) ) ;
#34203=ADVANCED_FACE ( 'NONE', ( #18551 ), #11047, .T. ) ;
#34205=VECTOR ( 'NONE', #95999, 1000.000000000000000 ) ;
#34207=CARTESIAN_POINT ( 'NONE',  ( -3.434112377981047626, 5.165301336597089232, 12.81628187352647963 ) ) ;
#34216=CARTESIAN_POINT ( 'NONE',  ( 9.997910040112534702, 4.470079180682592273E-16, 10.50199004140724490 ) ) ;
#34223=CARTESIAN_POINT ( 'NONE',  ( 3.193136578977092466, 6.674619624363884700E-16, -14.27383009353652277 ) ) ;
#34229=LINE ( 'NONE', #27233, #46868 ) ;
#34233=PLANE ( 'NONE',  #90241 ) ;
#34234=AXIS2_PLACEMENT_3D ( 'NONE', #39754, #31736, #93224 ) ;
#34246=DIRECTION ( 'NONE',  ( 0.000000000000000000, 0.000000000000000000, 1.000000000000000000 ) ) ;
#34254=CARTESIAN_POINT ( 'NONE',  ( 14.17193700899790265, 15.00000000000000000, -1.489530601564018175 ) ) ;
#34276=PLANE ( 'NONE',  #55948 ) ;
#34280=CARTESIAN_POINT ( 'NONE',  ( 0.000000000000000000, 15.00000000000000000, 0.000000000000000000 ) ) ;
#34288=AXIS2_PLACEMENT_3D ( 'NONE', #29247, #59247, #82245 ) ;
#34289=DIRECTION ( 'NONE',  ( 0.000000000000000000, 1.000000000000000000, 0.000000000000000000 ) ) ;
#34295=DIRECTION ( 'NONE',  ( -0.000000000000000000, -1.000000000000000000, -0.000000000000000000 ) ) ;
#34303=DIRECTION ( 'NONE',  ( 0.000000000000000000, 1.000000000000000000, 0.000000000000000000 ) ) ;
#34308=CIRCLE ( 'NONE', #42261, 14.49999999999999822 ) ;
#34311=ORIENTED_EDGE ( 'NONE', *, *, #30810, .F. ) ;
#34313=CARTESIAN_POINT ( 'NONE',  ( 13.82671409943296226, -0.03417435944610275333, -3.447387012295225261 ) ) ;
#34325=B_SPLINE_CURVE_WITH_KNOTS ( 'NONE', 3,
 ( #90474, #52971, #28984, #73997, #29472, #51502 ),
 .UNSPECIFIED., .F., .F.,
 ( 4, 2, 4 ),
 ( 0.0002800245631527670145, 0.0006862300328564149843, 0.001092435502560062900 ),
 .UNSPECIFIED. ) ;
#34327=VERTEX_POINT ( 'NONE', #29353 ) ;
#34341=ORIENTED_EDGE ( 'NONE', *, *, #16959, .F. ) ;
#34345=ORIENTED_EDGE ( 'NONE', *, *, #76004, .F. ) ;
#34346=DIRECTION ( 'NONE',  ( 0.000000000000000000, 0.000000000000000000, 1.000000000000000000 ) ) ;
#34347=DIRECTION ( 'NONE',  ( -0.000000000000000000, 1.000000000000000000, -0.000000000000000000 ) ) ;
#34348=EDGE_CURVE ( 'NONE', #23697, #73387, #22373, .T. ) ;
#34361=CARTESIAN_POINT ( 'NONE',  ( 5.361923921558569894, 0.000000000000000000, 0.9937738586172348842 ) ) ;
#34363=ORIENTED_EDGE ( 'NONE', *, *, #69233, .T. ) ;
#34387=CARTESIAN_POINT ( 'NONE',  ( -0.1556627343491930049, 2.117582368135750848E-16, 14.62580308442190713 ) ) ;
#34391=CARTESIAN_POINT ( 'NONE',  ( -14.22901244993679448, 15.00000000000000888, -3.387263120971507835 ) ) ;
#34393=CARTESIAN_POINT ( 'NONE',  ( -6.382347221874291598, 14.49999999999999112, -13.57444820018240783 ) ) ;
#34398=ORIENTED_EDGE ( 'NONE', *, *, #17197, .T. ) ;
#34403=LINE ( 'NONE', #50401, #44790 ) ;
#34410=ORIENTED_EDGE ( 'NONE', *, *, #76121, .T. ) ;
#34414=VECTOR ( 'NONE', #11085, 1000.000000000000114 ) ;
#34423=VERTEX_POINT ( 'NONE', #75353 ) ;
#34432=DIRECTION ( 'NONE',  ( -0.000000000000000000, -1.000000000000000000, -0.000000000000000000 ) ) ;
#34440=ADVANCED_FACE ( 'NONE', ( #28857 ), #62449, .T. ) ;
#34442=DIRECTION ( 'NONE',  ( 0.000000000000000000, 1.000000000000000000, -0.000000000000000000 ) ) ;
#34451=CARTESIAN_POINT ( 'NONE',  ( 12.81628187352647608, -28.58469866340290721, 3.434112377981052511 ) ) ;
#34452=ORIENTED_EDGE ( 'NONE', *, *, #74844, .T. ) ;
#34469=VERTEX_POINT ( 'NONE', #89864 ) ;
#34476=CARTESIAN_POINT ( 'NONE',  ( -4.838527690343711107, 0.3639308167276193995, 14.19819177887727157 ) ) ;
#34480=ORIENTED_EDGE ( 'NONE', *, *, #62201, .T. ) ;
#34481=CARTESIAN_POINT ( 'NONE',  ( -9.011287250621867528, 0.2306972965111889207, 11.91783356064781607 ) ) ;
#34484=AXIS2_PLACEMENT_3D ( 'NONE', #84187, #21716, #38682 ) ;
#34488=CARTESIAN_POINT ( 'NONE',  ( 4.922013193295439848, 0.000000000000000000, -2.347679864819448348 ) ) ;
#34501=CARTESIAN_POINT ( 'NONE',  ( -1.114591949025129258, 15.00000000000000000, 14.45709807627963706 ) ) ;
#34503=CARTESIAN_POINT ( 'NONE',  ( -7.082119434687058401, -34.02958449841936073, -12.26659068614894110 ) ) ;
#34518=CARTESIAN_POINT ( 'NONE',  ( -9.422509992056136596, 18.48035201082151602, 5.440088680355559703 ) ) ;
#34522=EDGE_CURVE ( 'NONE', #63596, #18620, #51875, .T. ) ;
#34526=EDGE_CURVE ( 'NONE', #89588, #60892, #70468, .T. ) ;
#34532=DIRECTION ( 'NONE',  ( 0.000000000000000000, 0.000000000000000000, 1.000000000000000000 ) ) ;
#34544=CARTESIAN_POINT ( 'NONE',  ( -9.402796353260987061, 14.49999999999999112, -11.68706210897776465 ) ) ;
#34548=CARTESIAN_POINT ( 'NONE',  ( 0.000000000000000000, 14.49999999999999822, 0.000000000000000000 ) ) ;
#34551=ORIENTED_EDGE ( 'NONE', *, *, #8255, .F. ) ;
#34561=DIRECTION ( 'NONE',  ( -0.000000000000000000, -1.000000000000000000, -0.000000000000000000 ) ) ;
#34563=ADVANCED_FACE ( 'NONE', ( #46824 ), #36917, .T. ) ;
#34564=CARTESIAN_POINT ( 'NONE',  ( -8.527530157486173934, 1.425597817667455303, 4.923371831947302546 ) ) ;
#34566=DIRECTION ( 'NONE',  ( -0.8788171126619679363, 0.000000000000000000, 0.4771587602596037980 ) ) ;
#34576=AXIS2_PLACEMENT_3D ( 'NONE', #63869, #2436, #32894 ) ;
#34579=ORIENTED_EDGE ( 'NONE', *, *, #10994, .T. ) ;
#34582=EDGE_LOOP ( 'NONE', ( #37499, #15103, #10632, #27076, #25332, #65317 ) ) ;
#34591=DIRECTION ( 'NONE',  ( 0.000000000000000000, 0.000000000000000000, 1.000000000000000000 ) ) ;
#34596=ORIENTED_EDGE ( 'NONE', *, *, #2317, .F. ) ;
#34609=ORIENTED_EDGE ( 'NONE', *, *, #91797, .F. ) ;
#34610=CARTESIAN_POINT ( 'NONE',  ( 0.000000000000000000, 15.00000000000000000, 0.000000000000000000 ) ) ;
#34615=CARTESIAN_POINT ( 'NONE',  ( 5.419894505350582925, 0.5000000000000004441, -13.98659156302458761 ) ) ;
#34621=ORIENTED_EDGE ( 'NONE', *, *, #86987, .T. ) ;
#34626=CARTESIAN_POINT ( 'NONE',  ( 10.16173502257720607, 12.81517340034854868, -5.532277395377471763 ) ) ;
#34632=CARTESIAN_POINT ( 'NONE',  ( 10.88017736071110164, -29.64464798917849109, 2.915334737309921209 ) ) ;
#34637=FACE_OUTER_BOUND ( 'NONE', #77820, .T. ) ;
#34646=EDGE_CURVE ( 'NONE', #95455, #19933, #17815, .T. ) ;
#34652=ADVANCED_FACE ( 'NONE', ( #39826 ), #78803, .F. ) ;
#34657=ORIENTED_EDGE ( 'NONE', *, *, #98641, .T. ) ;
#34667=AXIS2_PLACEMENT_3D ( 'NONE', #2742, #78715, #31724 ) ;
#34668=ADVANCED_FACE ( 'NONE', ( #63292 ), #23854, .F. ) ;
#34670=CARTESIAN_POINT ( 'NONE',  ( 7.771322705631394712, 15.00000000000000000, 12.24159072199921283 ) ) ;
#34672=VERTEX_POINT ( 'NONE', #31812 ) ;
#34673=CARTESIAN_POINT ( 'NONE',  ( 9.742785792574936821, 10.00513551118487499, 5.624999999999997335 ) ) ;
#34680=CARTESIAN_POINT ( 'NONE',  ( -0.7375392941519317569, 0.5000000000000004441, 14.98185688723470044 ) ) ;
#34690=CARTESIAN_POINT ( 'NONE',  ( -9.846743663894596210, -39.19940218233254825, -2.638427012816824124 ) ) ;
#34691=ORIENTED_EDGE ( 'NONE', *, *, #69650, .F. ) ;
#34695=ORIENTED_EDGE ( 'NONE', *, *, #8089, .F. ) ;
#34701=B_SPLINE_CURVE_WITH_KNOTS ( 'NONE', 3,
 ( #65100, #95621, #27110, #80621, #12115, #7092 ),
 .UNSPECIFIED., .F., .F.,
 ( 4, 2, 4 ),
 ( 3.409110551495867094E-05, 0.0004400426677367964921, 0.0008459942299586342522 ),
 .UNSPECIFIED. ) ;
#34702=CARTESIAN_POINT ( 'NONE',  ( 11.09922568453595026, 6.206968003263757083, 6.408140936763232709 ) ) ;
#34703=EDGE_LOOP ( 'NONE', ( #50499, #57589, #2160, #9434 ) ) ;
#34705=ORIENTED_EDGE ( 'NONE', *, *, #1141, .F. ) ;
#34707=AXIS2_PLACEMENT_3D ( 'NONE', #53549, #44070, #90070 ) ;
#34715=CIRCLE ( 'NONE', #60282, 14.49999999999999822 ) ;
#34717=AXIS2_PLACEMENT_3D ( 'NONE', #5562, #59035, #1021 ) ;
#34725=EDGE_CURVE ( 'NONE', #38271, #68316, #15856, .T. ) ;
#34727=DIRECTION ( 'NONE',  ( 0.000000000000000000, 1.000000000000000000, 0.000000000000000000 ) ) ;
#34735=CARTESIAN_POINT ( 'NONE',  ( -14.99847009497944583, 0.5000000000000004441, 0.2142307401079343032 ) ) ;
#34745=B_SPLINE_CURVE_WITH_KNOTS ( 'NONE', 3,
 ( #70503, #55500, #86001, #69518, #24524, #17512 ),
 .UNSPECIFIED., .F., .F.,
 ( 4, 2, 4 ),
 ( 3.409110551496079191E-05, 0.0004400426677367849453, 0.0008459942299586090987 ),
 .UNSPECIFIED. ) ;
#34747=CARTESIAN_POINT ( 'NONE',  ( -11.24999999999999822, 3.130135511184870545, 3.014428414850141458 ) ) ;
#34751=DIRECTION ( 'NONE',  ( 0.000000000000000000, 1.000000000000000000, 0.000000000000000000 ) ) ;
#34760=CARTESIAN_POINT ( 'NONE',  ( 12.83294900548058415, 0.5000000000000004441, 7.766300266068450142 ) ) ;
#34763=CIRCLE ( 'NONE', #14028, 15.00000000000000000 ) ;
#34770=DIRECTION ( 'NONE',  ( -0.3665012267242880317, 0.000000000000000000, -0.9304175679820281264 ) ) ;
#34771=FACE_OUTER_BOUND ( 'NONE', #4878, .T. ) ;
#34785=FACE_OUTER_BOUND ( 'NONE', #10549, .T. ) ;
#34788=DIRECTION ( 'NONE',  ( 0.000000000000000000, 1.000000000000000000, 0.000000000000000000 ) ) ;
#34791=AXIS2_PLACEMENT_3D ( 'NONE', #1356, #75349, #90841 ) ;
#34814=VERTEX_POINT ( 'NONE', #54319 ) ;
#34820=CARTESIAN_POINT ( 'NONE',  ( 2.913501739333662854, 4.325554204331052541E-16, 14.20427779279537184 ) ) ;
#34821=CARTESIAN_POINT ( 'NONE',  ( 0.000000000000000000, 0.000000000000000000, 0.000000000000000000 ) ) ;
#34827=ORIENTED_EDGE ( 'NONE', *, *, #36258, .T. ) ;
#34834=CARTESIAN_POINT ( 'NONE',  ( -6.305254017448156389, 1.877203152459836266, -10.07310051930115513 ) ) ;
#34846=CARTESIAN_POINT ( 'NONE',  ( -13.82671409943291785, 15.00000000000000000, -3.447387012295409114 ) ) ;
#34851=CARTESIAN_POINT ( 'NONE',  ( -10.14667048435152097, 15.00000000000000000, 10.35833375027034542 ) ) ;
#34852=CARTESIAN_POINT ( 'NONE',  ( -10.70613742633264565, 4.864377723017530212E-16, 9.778988772285165609 ) ) ;
#34858=ORIENTED_EDGE ( 'NONE', *, *, #89671, .T. ) ;
#34859=B_SPLINE_CURVE_WITH_KNOTS ( 'NONE', 3,
 ( #63479, #93983, #25505, #55992, #86493, #17993 ),
 .UNSPECIFIED., .F., .F.,
 ( 4, 2, 4 ),
 ( 3.409110551475769374E-05, 0.0004400426677365839884, 0.0008459942299584103645 ),
 .UNSPECIFIED. ) ;
#34862=CARTESIAN_POINT ( 'NONE',  ( 7.108715748589077066, 14.95077488074853456, 12.92719074505371246 ) ) ;
#34865=LINE ( 'NONE', #73851, #69618 ) ;
#34892=ADVANCED_FACE ( 'NONE', ( #72273 ), #50255, .F. ) ;
#34893=CARTESIAN_POINT ( 'NONE',  ( 11.35178980618978173, 14.63606909211789464, -9.804941009311937350 ) ) ;
#34895=CARTESIAN_POINT ( 'NONE',  ( 0.000000000000000000, 0.000000000000000000, 0.000000000000000000 ) ) ;
#34907=DIRECTION ( 'NONE',  ( -0.9636304532086248376, 0.000000000000000000, 0.2672383760782501838 ) ) ;
#34931=CARTESIAN_POINT ( 'NONE',  ( 6.382347221874423937, 0.5000000000000004441, -13.57444820018227638 ) ) ;
#34934=EDGE_LOOP ( 'NONE', ( #15302, #30043, #82146, #66062, #70525, #4719 ) ) ;
#34938=FACE_OUTER_BOUND ( 'NONE', #31248, .T. ) ;
#34942=FACE_OUTER_BOUND ( 'NONE', #41421, .T. ) ;
#34946=CARTESIAN_POINT ( 'NONE',  ( 9.382169495545419124, -29.00136533006957862, 9.382169495545417348 ) ) ;
#34981=PLANE ( 'NONE',  #2480 ) ;
#34986=DIRECTION ( 'NONE',  ( 0.000000000000000000, 1.000000000000000000, 0.000000000000000000 ) ) ;
#34997=CARTESIAN_POINT ( 'NONE',  ( -14.16423886937410082, -28.19625116508602503, 4.336808689942017736E-15 ) ) ;
#35000=EDGE_CURVE ( 'NONE', #7097, #37440, #36376, .T. ) ;
#35006=LINE ( 'NONE', #4544, #67252 ) ;
#35008=EDGE_CURVE ( 'NONE', #81310, #7169, #10592, .T. ) ;
#35010=AXIS2_PLACEMENT_3D ( 'NONE', #66689, #97707, #51193 ) ;
#35013=CARTESIAN_POINT ( 'NONE',  ( 5.440088680355549045, 21.39701867748818032, -9.422509992056141925 ) ) ;
#35027=CARTESIAN_POINT ( 'NONE',  ( -8.722765153436172980, 15.00000000000000888, -11.74102699209696432 ) ) ;
#35046=ORIENTED_EDGE ( 'NONE', *, *, #54951, .T. ) ;
#35055=CARTESIAN_POINT ( 'NONE',  ( 10.19513985507833276, 0.5000000000000004441, -11.00268709613217055 ) ) ;
#35057=EDGE_CURVE ( 'NONE', #50602, #81607, #13248, .T. ) ;
#35058=CARTESIAN_POINT ( 'NONE',  ( -13.14228782657329653, 0.5000000000000004441, -7.230509711182418364 ) ) ;
#35059=CARTESIAN_POINT ( 'NONE',  ( 9.846743663894590881, 3.300597817667453526, 2.638427012816828565 ) ) ;
#35063=DIRECTION ( 'NONE',  ( 0.000000000000000000, 1.000000000000000000, 0.000000000000000000 ) ) ;
#35075=ORIENTED_EDGE ( 'NONE', *, *, #63155, .F. ) ;
#35077=ORIENTED_EDGE ( 'NONE', *, *, #19140, .T. ) ;
#35079=VECTOR ( 'NONE', #80422, 1000.000000000000000 ) ;
#35087=EDGE_CURVE ( 'NONE', #89457, #8159, #32998, .T. ) ;
#35089=ORIENTED_EDGE ( 'NONE', *, *, #1974, .F. ) ;
#35093=EDGE_CURVE ( 'NONE', #43087, #55079, #80889, .T. ) ;
#35094=CARTESIAN_POINT ( 'NONE',  ( 4.838527690343521925, 0.3640475087720984604, 14.19819177887730888 ) ) ;
#35097=VECTOR ( 'NONE', #43850, 1000.000000000000000 ) ;
#35099=FACE_OUTER_BOUND ( 'NONE', #89104, .T. ) ;
#35104=CARTESIAN_POINT ( 'NONE',  ( 0.000000000000000000, 15.00000000000000000, 0.000000000000000000 ) ) ;
#35124=DIRECTION ( 'NONE',  ( -0.000000000000000000, -1.000000000000000000, -0.000000000000000000 ) ) ;
#35128=CARTESIAN_POINT ( 'NONE',  ( -10.88017736071110164, -27.14464798917849109, -2.915334737309917212 ) ) ;
#35130=CARTESIAN_POINT ( 'NONE',  ( 14.74963345907815437, 0.04922511925147114720, -0.3072669459660632985 ) ) ;
#35141=DIRECTION ( 'NONE',  ( -0.000000000000000000, -1.000000000000000000, -0.000000000000000000 ) ) ;
#35150=VECTOR ( 'NONE', #75623, 1000.000000000000000 ) ;
#35157=LINE ( 'NONE', #96179, #84017 ) ;
#35164=VERTEX_POINT ( 'NONE', #81250 ) ;
#35165=CARTESIAN_POINT ( 'NONE',  ( 1.983216688680843109, 15.00000000000000000, 14.11131997956739070 ) ) ;
#35179=CARTESIAN_POINT ( 'NONE',  ( 4.923371831947301658, -32.32440218233254825, 8.527530157486175710 ) ) ;
#35182=ORIENTED_EDGE ( 'NONE', *, *, #91387, .F. ) ;
#35191=CARTESIAN_POINT ( 'NONE',  ( 12.81628187352647252, 6.831968003263756195, -3.434112377981059172 ) ) ;
#35196=ORIENTED_EDGE ( 'NONE', *, *, #5571, .T. ) ;
#35203=DIRECTION ( 'NONE',  ( -0.000000000000000000, -1.000000000000000000, -0.000000000000000000 ) ) ;
#35205=ORIENTED_EDGE ( 'NONE', *, *, #21764, .F. ) ;
#35209=CARTESIAN_POINT ( 'NONE',  ( 13.61802159414299140, -2.298423902374543181E-15, 5.334603887713582182 ) ) ;
#35216=ORIENTED_EDGE ( 'NONE', *, *, #51977, .F. ) ;
#35228=CARTESIAN_POINT ( 'NONE',  ( 0.000000000000000000, 0.5000000000000004441, 0.000000000000000000 ) ) ;
#35234=CARTESIAN_POINT ( 'NONE',  ( -2.120353041430744323, 4.696395766537044518E-16, 14.34413130794943925 ) ) ;
#35237=ORIENTED_EDGE ( 'NONE', *, *, #39252, .T. ) ;
#35239=CARTESIAN_POINT ( 'NONE',  ( -13.14228782657336581, 14.49999999999999112, -7.230509711182429022 ) ) ;
#35242=LINE ( 'NONE', #96269, #40840 ) ;
#35246=CARTESIAN_POINT ( 'NONE',  ( -4.023424921641842289, -0.03417435944610275333, 15.48190712851503648 ) ) ;
#35258=CARTESIAN_POINT ( 'NONE',  ( 11.36220558718857276, 15.00000000000000000, 9.008345252845320061 ) ) ;
#35272=CARTESIAN_POINT ( 'NONE',  ( -3.468686501387172161, 0.000000000000000000, 4.207853202970306405 ) ) ;
#35278=CARTESIAN_POINT ( 'NONE',  ( 14.67697702673042848, -0.03417435944610275333, -6.361111679013412790 ) ) ;
#35287=ORIENTED_EDGE ( 'NONE', *, *, #17045, .T. ) ;
#35304=ORIENTED_EDGE ( 'NONE', *, *, #66128, .T. ) ;
#35310=DIRECTION ( 'NONE',  ( 0.000000000000000000, 1.000000000000000000, 0.000000000000000000 ) ) ;
#35311=CARTESIAN_POINT ( 'NONE',  ( -11.35178980618986877, 14.49999999999999112, 9.804941009311868072 ) ) ;
#35312=ORIENTED_EDGE ( 'NONE', *, *, #53164, .T. ) ;
#35315=CARTESIAN_POINT ( 'NONE',  ( -5.419894505350723257, 14.49999999999999112, 13.98659156302460183 ) ) ;
#35324=CARTESIAN_POINT ( 'NONE',  ( 2.189108318723745672, 15.00000000000000178, -14.46085460646898646 ) ) ;
#35325=EDGE_CURVE ( 'NONE', #20839, #40449, #81695, .T. ) ;
#35328=CARTESIAN_POINT ( 'NONE',  ( -9.997910040112461871, 4.266261872180168263E-16, -10.50199004140731773 ) ) ;
#35331=AXIS2_PLACEMENT_3D ( 'NONE', #18795, #63773, #32299 ) ;
#35334=ORIENTED_EDGE ( 'NONE', *, *, #66707, .F. ) ;
#35343=EDGE_LOOP ( 'NONE', ( #9704, #47737, #5414, #61744, #51063, #32483 ) ) ;
#35346=CARTESIAN_POINT ( 'NONE',  ( -3.836325488035988052, 0.5000000000000004441, -14.50112432709427424 ) ) ;
#35352=FACE_OUTER_BOUND ( 'NONE', #58046, .T. ) ;
#35362=CARTESIAN_POINT ( 'NONE',  ( 0.000000000000000000, 15.00000000000000000, 0.000000000000000000 ) ) ;
#35369=CARTESIAN_POINT ( 'NONE',  ( 9.972640495195376431, 15.00000000000000000, -12.50695158660345818 ) ) ;
#35370=ADVANCED_FACE ( 'NONE', ( #15738 ), #37256, .F. ) ;
#35374=CARTESIAN_POINT ( 'NONE',  ( 7.595945211629608451, 15.00000000000000000, 12.35117874302463292 ) ) ;
#35381=CARTESIAN_POINT ( 'NONE',  ( -5.204170427930421283E-15, 3.438309369127513726, -11.92686044187656513 ) ) ;
#35384=DIRECTION ( 'NONE',  ( 0.000000000000000000, 1.000000000000000000, 0.000000000000000000 ) ) ;
#35391=CARTESIAN_POINT ( 'NONE',  ( -10.32896413005680536, 9.271642702460850316, -5.963430220938272797 ) ) ;
#35395=CARTESIAN_POINT ( 'NONE',  ( -7.551349515323020789, 15.00000000000000000, -12.08468537022916323 ) ) ;
#35398=FACE_OUTER_BOUND ( 'NONE', #60793, .T. ) ;
#35399=CYLINDRICAL_SURFACE ( 'NONE', #73552, 15.00000000000000000 ) ;
#35416=FACE_OUTER_BOUND ( 'NONE', #14037, .T. ) ;
#35428=CARTESIAN_POINT ( 'NONE',  ( -12.60589901313233874, 14.49999999999999112, 8.129656208641975468 ) ) ;
#35429=AXIS2_PLACEMENT_3D ( 'NONE', #88942, #74922, #51933 ) ;
#35430=ORIENTED_EDGE ( 'NONE', *, *, #84910, .F. ) ;
#35441=DIRECTION ( 'NONE',  ( 0.000000000000000000, 0.000000000000000000, 1.000000000000000000 ) ) ;
#35443=EDGE_LOOP ( 'NONE', ( #98599, #63349, #31727, #22005, #10647, #48850 ) ) ;
#35444=TOROIDAL_SURFACE ( 'NONE', #5114, 14.49999999999999822, 0.5000000000000000000 ) ;
#35445=LINE ( 'NONE', #63960, #33516 ) ;
#35447=CARTESIAN_POINT ( 'NONE',  ( -11.09922568453595382, -26.29303199673624292, -6.408140936763226492 ) ) ;
#35456=CARTESIAN_POINT ( 'NONE',  ( 0.000000000000000000, 15.00000000000000000, 0.000000000000000000 ) ) ;
#35457=ORIENTED_EDGE ( 'NONE', *, *, #62201, .F. ) ;
#35460=EDGE_CURVE ( 'NONE', #59552, #1757, #10176, .T. ) ;
#35475=ORIENTED_EDGE ( 'NONE', *, *, #4531, .T. ) ;
#35476=VECTOR ( 'NONE', #89176, 1000.000000000000000 ) ;
#35477=CARTESIAN_POINT ( 'NONE',  ( 0.3093388210927633941, 0.5000000000000004441, 14.99680997725065978 ) ) ;
#35479=ORIENTED_EDGE ( 'NONE', *, *, #67432, .T. ) ;
#35484=DIRECTION ( 'NONE',  ( 0.000000000000000000, 1.000000000000000000, 0.000000000000000000 ) ) ;
#35491=DIRECTION ( 'NONE',  ( 0.000000000000000000, 0.000000000000000000, 1.000000000000000000 ) ) ;
#35499=FACE_OUTER_BOUND ( 'NONE', #39167, .T. ) ;
#35501=CARTESIAN_POINT ( 'NONE',  ( -12.26659068614894110, -32.77958449841936073, 7.082119434687058401 ) ) ;
#35505=ORIENTED_EDGE ( 'NONE', *, *, #43351, .T. ) ;
#35512=VECTOR ( 'NONE', #94140, 1000.000000000000000 ) ;
#35519=CARTESIAN_POINT ( 'NONE',  ( -5.204170427930421283E-15, 16.81368534415483751, -10.88017736071110342 ) ) ;
#35525=B_SPLINE_CURVE_WITH_KNOTS ( 'NONE', 3,
 ( #47749, #78246, #2282, #86250, #31261, #8770 ),
 .UNSPECIFIED., .F., .F.,
 ( 4, 2, 4 ),
 ( 3.409110551494648044E-05, 0.0004400426677367906374, 0.0008459942299586347943 ),
 .UNSPECIFIED. ) ;
#35532=CARTESIAN_POINT ( 'NONE',  ( 14.16722289976685190, 14.63606870530283999, 4.928467845925642798 ) ) ;
#35535=ORIENTED_EDGE ( 'NONE', *, *, #9396, .T. ) ;
#35547=DIRECTION ( 'NONE',  ( 0.000000000000000000, 1.000000000000000000, 0.000000000000000000 ) ) ;
#35554=ORIENTED_EDGE ( 'NONE', *, *, #52290, .F. ) ;
#35559=FACE_OUTER_BOUND ( 'NONE', #67990, .T. ) ;
#35562=EDGE_CURVE ( 'NONE', #4144, #63596, #28071, .T. ) ;
#35563=CARTESIAN_POINT ( 'NONE',  ( -14.71525861348285957, 0.5000000000000004441, -2.908807992686776700 ) ) ;
#35566=CARTESIAN_POINT ( 'NONE',  ( 8.527530157486179263, 8.092264484334123154, 4.923371831947292776 ) ) ;
#35577=CIRCLE ( 'NONE', #49920, 14.49999999999999822 ) ;
#35586=AXIS2_PLACEMENT_3D ( 'NONE', #49817, #25506, #54495 ) ;
#35588=ORIENTED_EDGE ( 'NONE', *, *, #54641, .T. ) ;
#35598=EDGE_LOOP ( 'NONE', ( #12706, #49972, #81813, #48245 ) ) ;
#35601=AXIS2_PLACEMENT_3D ( 'NONE', #89314, #3855, #5336 ) ;
#35605=CARTESIAN_POINT ( 'NONE',  ( -11.55579792925658111, 12.87141902714432362, 1.357825507271567922 ) ) ;
#35606=DIRECTION ( 'NONE',  ( 0.7132504491541801217, 0.000000000000000000, 0.7009092642998523415 ) ) ;
#35611=ORIENTED_EDGE ( 'NONE', *, *, #19983, .T. ) ;
#35612=CARTESIAN_POINT ( 'NONE',  ( -3.195792623639539975, 3.646642702460842766, -11.92686044187656158 ) ) ;
#35616=VECTOR ( 'NONE', #42652, 999.9999999999998863 ) ;
#35622=CARTESIAN_POINT ( 'NONE',  ( -12.07856007377816887, 4.482427100288500905E-16, -8.022367888855006512 ) ) ;
#35632=CARTESIAN_POINT ( 'NONE',  ( -10.93781366033335622, 14.49999999999999112, -10.26470809774086490 ) ) ;
#35636=CARTESIAN_POINT ( 'NONE',  ( 9.422509992056141925, -24.85298132251182679, 5.440088680355547268 ) ) ;
#35640=DIRECTION ( 'NONE',  ( 0.000000000000000000, 1.000000000000000000, 0.000000000000000000 ) ) ;
#35642=LINE ( 'NONE', #81138, #3399 ) ;
#35648=AXIS2_PLACEMENT_3D ( 'NONE', #94372, #93883, #46900 ) ;
#35650=CARTESIAN_POINT ( 'NONE',  ( 0.000000000000000000, 12.49999999999999112, 0.000000000000000000 ) ) ;
#35652=ORIENTED_EDGE ( 'NONE', *, *, #14633, .T. ) ;
#35655=LINE ( 'NONE', #94685, #49322 ) ;
#35662=AXIS2_PLACEMENT_3D ( 'NONE', #9789, #41289, #9292 ) ;
#35663=DIRECTION ( 'NONE',  ( 0.000000000000000000, 1.000000000000000000, 0.000000000000000000 ) ) ;
#35665=EDGE_CURVE ( 'NONE', #94935, #97969, #25609, .T. ) ;
#35666=VERTEX_POINT ( 'NONE', #77598 ) ;
#35670=VERTEX_POINT ( 'NONE', #3597 ) ;
#35685=CARTESIAN_POINT ( 'NONE',  ( -2.913501739333569152, 4.140530414402051497E-16, -14.20427779279538960 ) ) ;
#35688=CARTESIAN_POINT ( 'NONE',  ( -7.208316651077756099, -38.36606884899921255, 7.208316651077766757 ) ) ;
#35689=EDGE_LOOP ( 'NONE', ( #31413, #78671, #50659, #62019 ) ) ;
#35690=PLANE ( 'NONE',  #76274 ) ;
#35691=ORIENTED_EDGE ( 'NONE', *, *, #51256, .T. ) ;
#35692=ORIENTED_EDGE ( 'NONE', *, *, #28706, .T. ) ;
#35696=CYLINDRICAL_SURFACE ( 'NONE', #17700, 15.00000000000000000 ) ;
#35699=CARTESIAN_POINT ( 'NONE',  ( -11.09922568453594316, 4.540301336597093673, 6.408140936763246920 ) ) ;
#35704=EDGE_LOOP ( 'NONE', ( #41128, #44411, #86293, #44295 ) ) ;
#35709=CARTESIAN_POINT ( 'NONE',  ( 11.35178980618967337, 15.00000000000000000, 9.804941009311999522 ) ) ;
#35712=VERTEX_POINT ( 'NONE', #64552 ) ;
#35715=DIRECTION ( 'NONE',  ( 0.000000000000000000, 1.000000000000000000, 0.000000000000000000 ) ) ;
#35716=DIRECTION ( 'NONE',  ( -0.9981347984218674751, 0.000000000000000000, 0.06104853953484969814 ) ) ;
#35717=LINE ( 'NONE', #96738, #68506 ) ;
#35721=CARTESIAN_POINT ( 'NONE',  ( 15.61289147378509057, -0.03417435944610275333, 3.480663193108788800 ) ) ;
#35722=EDGE_LOOP ( 'NONE', ( #93882, #96847, #13802, #13520, #40608, #3711 ) ) ;
#35724=CARTESIAN_POINT ( 'NONE',  ( -10.97324858046209961, 7.322546142722302618E-32, 9.670892530813134158 ) ) ;
#35729=CARTESIAN_POINT ( 'NONE',  ( 8.606322355891288467, 3.856550154308941175E-16, 11.66967075398812703 ) ) ;
#35737=LINE ( 'NONE', #66225, #31546 ) ;
#35751=CARTESIAN_POINT ( 'NONE',  ( -14.16423886937409726, 2.012082168247306679, 3.795296366450320757 ) ) ;
#35766=LINE ( 'NONE', #90242, #73847 ) ;
#35769=ORIENTED_EDGE ( 'NONE', *, *, #52501, .F. ) ;
#35771=CARTESIAN_POINT ( 'NONE',  ( -10.84451454130493708, 4.806230040756559413E-16, -9.625305416630981270 ) ) ;
#35776=CARTESIAN_POINT ( 'NONE',  ( 8.439016546559898302, 4.734672723634894724E-16, -11.79122553964973541 ) ) ;
#35781=CARTESIAN_POINT ( 'NONE',  ( -11.94665733272784003, 14.76984983275088936, 8.972157519073542531 ) ) ;
#35795=ADVANCED_FACE ( 'NONE', ( #40607 ), #77524, .T. ) ;
#35800=CARTESIAN_POINT ( 'NONE',  ( -14.94699059465103375, 0.3640475087720990710, 1.259949270174711700 ) ) ;
#35802=AXIS2_PLACEMENT_3D ( 'NONE', #33158, #3177, #24700 ) ;
#35805=ORIENTED_EDGE ( 'NONE', *, *, #98641, .F. ) ;
#35807=ORIENTED_EDGE ( 'NONE', *, *, #15810, .T. ) ;
#35813=ORIENTED_EDGE ( 'NONE', *, *, #6089, .F. ) ;
#35817=ADVANCED_FACE ( 'NONE', ( #63580 ), #45632, .T. ) ;
#35822=EDGE_CURVE ( 'NONE', #84126, #47538, #70117, .T. ) ;
#35824=ORIENTED_EDGE ( 'NONE', *, *, #11758, .F. ) ;
#35832=AXIS2_PLACEMENT_3D ( 'NONE', #96320, #88305, #12791 ) ;
#35833=VERTEX_POINT ( 'NONE', #85114 ) ;
#35840=ORIENTED_EDGE ( 'NONE', *, *, #42103, .F. ) ;
#35844=CARTESIAN_POINT ( 'NONE',  ( 10.64017930668198453, 0.5000000000000004441, 10.57291749337222875 ) ) ;
#35855=CARTESIAN_POINT ( 'NONE',  ( 11.25000000000000000, 7.826366962315981723, -3.014428414850133908 ) ) ;
#35860=VECTOR ( 'NONE', #21511, 1000.000000000000000 ) ;
#35866=CARTESIAN_POINT ( 'NONE',  ( -10.70613742633264565, 4.864377723017530212E-16, 9.778988772285165609 ) ) ;
#35867=CARTESIAN_POINT ( 'NONE',  ( 0.000000000000000000, 0.5000000000000004441, 0.000000000000000000 ) ) ;
#35873=CARTESIAN_POINT ( 'NONE',  ( 10.32896413005679825, 2.604976035794182021, -5.963430220938286119 ) ) ;
#35876=VECTOR ( 'NONE', #89261, 1000.000000000000000 ) ;
#35879=CARTESIAN_POINT ( 'NONE',  ( 2.962741594152983993, 15.00000000000000000, 13.93860331045674883 ) ) ;
#35887=CARTESIAN_POINT ( 'NONE',  ( 1.915564264621337554, 4.132324795315745510E-16, 14.37291249357991774 ) ) ;
#35905=LINE ( 'NONE', #82388, #96928 ) ;
#35914=CARTESIAN_POINT ( 'NONE',  ( -0.9940297508538862292, -0.03417435944610275333, 14.21528771620248932 ) ) ;
#35922=CARTESIAN_POINT ( 'NONE',  ( 0.000000000000000000, 14.49999999999999822, 0.000000000000000000 ) ) ;
#35924=ORIENTED_EDGE ( 'NONE', *, *, #25883, .T. ) ;
#35927=PLANE ( 'NONE',  #16266 ) ;
#35937=ORIENTED_EDGE ( 'NONE', *, *, #51230, .F. ) ;
#35938=EDGE_CURVE ( 'NONE', #48953, #57022, #6627, .T. ) ;
#35940=CARTESIAN_POINT ( 'NONE',  ( -6.408140936763232709, -20.04303199673624292, 11.09922568453595026 ) ) ;
#35958=B_SPLINE_CURVE_WITH_KNOTS ( 'NONE', 3,
 ( #86036, #4019, #34481, #64975, #95500, #26991 ),
 .UNSPECIFIED., .F., .F.,
 ( 4, 2, 4 ),
 ( 3.409110551490396616E-05, 0.0004400426677367293800, 0.0008459942299585547802 ),
 .UNSPECIFIED. ) ;
#35968=ORIENTED_EDGE ( 'NONE', *, *, #53164, .F. ) ;
#35974=DIRECTION ( 'NONE',  ( 0.000000000000000000, 0.000000000000000000, 1.000000000000000000 ) ) ;
#35977=EDGE_CURVE ( 'NONE', #28751, #325, #68530, .T. ) ;
#35981=CARTESIAN_POINT ( 'NONE',  ( -11.62719953690074881, 14.49999999999999112, 9.476720473301769587 ) ) ;
#35991=EDGE_CURVE ( 'NONE', #82266, #17685, #95087, .T. ) ;
#35992=DIRECTION ( 'NONE',  ( 0.000000000000000000, 0.000000000000000000, 1.000000000000000000 ) ) ;
#35994=CARTESIAN_POINT ( 'NONE',  ( 7.082119434687047743, -24.86291783175269288, -12.26659068614894821 ) ) ;
#35995=CIRCLE ( 'NONE', #91891, 14.49999999999999822 ) ;
#35999=ORIENTED_EDGE ( 'NONE', *, *, #76445, .T. ) ;
#36001=AXIS2_PLACEMENT_3D ( 'NONE', #97043, #59505, #7009 ) ;
#36008=CARTESIAN_POINT ( 'NONE',  ( 0.000000000000000000, 14.49999999999999822, 0.000000000000000000 ) ) ;
#36011=CARTESIAN_POINT ( 'NONE',  ( -2.915334737309934532, 27.02201867748817321, -10.88017736071109987 ) ) ;
#36014=FACE_OUTER_BOUND ( 'NONE', #71366, .T. ) ;
#36018=EDGE_CURVE ( 'NONE', #35833, #47206, #84020, .T. ) ;
#36022=EDGE_CURVE ( 'NONE', #37077, #29308, #83897, .T. ) ;
#36025=CARTESIAN_POINT ( 'NONE',  ( 0.000000000000000000, 15.00000000000000000, 0.000000000000000000 ) ) ;
#36028=EDGE_LOOP ( 'NONE', ( #22415, #81915, #44588, #90617, #8198, #13532 ) ) ;
#36040=CARTESIAN_POINT ( 'NONE',  ( 0.000000000000000000, 35.00000000000000000, -11.92686044187656513 ) ) ;
#36042=CARTESIAN_POINT ( 'NONE',  ( 13.61912076658548365, 6.962610826430346815E-16, -5.334594295380906459 ) ) ;
#36043=ORIENTED_EDGE ( 'NONE', *, *, #85196, .F. ) ;
#36048=AXIS2_PLACEMENT_3D ( 'NONE', #1884, #85355, #70366 ) ;
#36054=EDGE_CURVE ( 'NONE', #46734, #11368, #8512, .T. ) ;
#36059=DIRECTION ( 'NONE',  ( 0.4305110968083047940, 0.000000000000000000, -0.9025852843498560762 ) ) ;
#36060=CARTESIAN_POINT ( 'NONE',  ( -4.923371831947302546, 10.17559781766745530, -8.527530157486173934 ) ) ;
#36062=EDGE_LOOP ( 'NONE', ( #93131, #11710, #89600, #18995 ) ) ;
#36063=DIRECTION ( 'NONE',  ( 0.000000000000000000, 0.000000000000000000, 1.000000000000000000 ) ) ;
#36071=AXIS2_PLACEMENT_3D ( 'NONE', #51805, #27812, #20818 ) ;
#36077=ORIENTED_EDGE ( 'NONE', *, *, #3280, .F. ) ;
#36079=ORIENTED_EDGE ( 'NONE', *, *, #35325, .F. ) ;
#36086=CARTESIAN_POINT ( 'NONE',  ( 10.09792486685183199, 14.95037105583725534, 10.75589247084419675 ) ) ;
#36092=EDGE_LOOP ( 'NONE', ( #16423, #66763, #15571, #26990 ) ) ;
#36093=CARTESIAN_POINT ( 'NONE',  ( -10.65882794182087778, 13.06867033551286639, 5.232423767642232271 ) ) ;
#36096=FACE_OUTER_BOUND ( 'NONE', #54961, .T. ) ;
#36098=CARTESIAN_POINT ( 'NONE',  ( 9.402796353261129170, 14.63595249122791664, -11.68706210897758169 ) ) ;
#36100=CARTESIAN_POINT ( 'NONE',  ( -12.98685442714202232, 15.00000000000000000, 6.449155920600843750 ) ) ;
#36101=AXIS2_PLACEMENT_3D ( 'NONE', #57624, #88122, #12618 ) ;
#36109=VERTEX_POINT ( 'NONE', #9995 ) ;
#36116=DIRECTION ( 'NONE',  ( -3.375077994860475883E-14, 0.000000000000000000, 1.000000000000000000 ) ) ;
#36118=CARTESIAN_POINT ( 'NONE',  ( 0.000000000000000000, 14.49999999999999822, 0.000000000000000000 ) ) ;
#36121=CARTESIAN_POINT ( 'NONE',  ( 3.469446951953614189E-15, -30.68631465584515894, 10.88017736071110342 ) ) ;
#36125=PLANE ( 'NONE',  #89509 ) ;
#36138=CARTESIAN_POINT ( 'NONE',  ( 0.000000000000000000, 0.5000000000000004441, 0.000000000000000000 ) ) ;
#36139=VECTOR ( 'NONE', #24175, 1000.000000000000000 ) ;
#36141=EDGE_CURVE ( 'NONE', #24045, #70993, #35995, .T. ) ;
#36154=DIRECTION ( 'NONE',  ( 0.5664062369248205053, 0.000000000000000000, 0.8241261886220241362 ) ) ;
#36156=B_SPLINE_CURVE_WITH_KNOTS ( 'NONE', 3,
 ( #52009, #7990, #6498, #68000, #518, #7510 ),
 .UNSPECIFIED., .F., .F.,
 ( 4, 2, 4 ),
 ( 3.409110551496140855E-05, 0.0004400426677367876016, 0.0008459942299586138692 ),
 .UNSPECIFIED. ) ;
#36157=AXIS2_PLACEMENT_3D ( 'NONE', #15234, #37735, #30692 ) ;
#36158=ORIENTED_EDGE ( 'NONE', *, *, #12093, .F. ) ;
#36161=TOROIDAL_SURFACE ( 'NONE', #39394, 14.49999999999999822, 0.5000000000000000000 ) ;
#36164=CARTESIAN_POINT ( 'NONE',  ( 0.3998276802503074046, 15.00000000000000000, 15.99117050944548879 ) ) ;
#36167=AXIS2_PLACEMENT_3D ( 'NONE', #51112, #97629, #81599 ) ;
#36178=CARTESIAN_POINT ( 'NONE',  ( 0.000000000000000000, 0.5000000000000004441, 0.000000000000000000 ) ) ;
#36182=CARTESIAN_POINT ( 'NONE',  ( 13.21272562211570012, -2.664342135588400928E-15, 6.271554226548244237 ) ) ;
#36193=B_SPLINE_CURVE_WITH_KNOTS ( 'NONE', 3,
 ( #68183, #83171, #38180, #84174, #46639, #31141 ),
 .UNSPECIFIED., .F., .F.,
 ( 4, 2, 4 ),
 ( 0.0002800364959417991299, 0.0006862420824208958397, 0.001092447668899992549 ),
 .UNSPECIFIED. ) ;
#36195=CARTESIAN_POINT ( 'NONE',  ( -3.434112377981067610, 13.08196800326375175, -12.81628187352647252 ) ) ;
#36196=VECTOR ( 'NONE', #68526, 1000.000000000000114 ) ;
#36207=VECTOR ( 'NONE', #25803, 1000.000000000000114 ) ;
#36212=DIRECTION ( 'NONE',  ( 0.000000000000000000, 0.000000000000000000, 1.000000000000000000 ) ) ;
#36213=VECTOR ( 'NONE', #10533, 1000.000000000000114 ) ;
#36217=LINE ( 'NONE', #66717, #29217 ) ;
#36218=ORIENTED_EDGE ( 'NONE', *, *, #61852, .F. ) ;
#36220=CARTESIAN_POINT ( 'NONE',  ( -11.35178980618981370, 0.3640475087720883018, 9.804941009311852085 ) ) ;
#36224=CARTESIAN_POINT ( 'NONE',  ( -14.47650479471817597, 0.3640475087720992375, -3.928206833722206692 ) ) ;
#36225=DIRECTION ( 'NONE',  ( -0.8949343616020228875, 0.000000000000000000, -0.4461978131098131573 ) ) ;
#36233=CIRCLE ( 'NONE', #1145, 14.49999999999999822 ) ;
#36235=PLANE ( 'NONE',  #74668 ) ;
#36236=TOROIDAL_SURFACE ( 'NONE', #69792, 14.49999999999999822, 0.5000000000000000000 ) ;
#36243=DIRECTION ( 'NONE',  ( 0.000000000000000000, 1.000000000000000000, 0.000000000000000000 ) ) ;
#36249=CARTESIAN_POINT ( 'NONE',  ( -14.16423886937410082, 11.80374883491398030, 4.336808689942017736E-15 ) ) ;
#36258=EDGE_CURVE ( 'NONE', #42615, #42002, #8875, .T. ) ;
#36262=FACE_OUTER_BOUND ( 'NONE', #59571, .T. ) ;
#36264=CIRCLE ( 'NONE', #5946, 15.00000000000000000 ) ;
#36269=VERTEX_POINT ( 'NONE', #55492 ) ;
#36284=AXIS2_PLACEMENT_3D ( 'NONE', #1746, #46722, #31220 ) ;
#36285=VERTEX_POINT ( 'NONE', #33450 ) ;
#36303=ORIENTED_EDGE ( 'NONE', *, *, #1167, .T. ) ;
#36305=VERTEX_POINT ( 'NONE', #40497 ) ;
#36309=CARTESIAN_POINT ( 'NONE',  ( 10.84451454130507209, 15.00000000000000000, -9.625305416630832056 ) ) ;
#36311=VECTOR ( 'NONE', #71833, 1000.000000000000000 ) ;
#36313=CARTESIAN_POINT ( 'NONE',  ( -9.957606878385396598, 13.12720750352077381, 6.606639848592291919 ) ) ;
#36317=ORIENTED_EDGE ( 'NONE', *, *, #27217, .F. ) ;
#36320=ORIENTED_EDGE ( 'NONE', *, *, #74212, .F. ) ;
#36327=ORIENTED_EDGE ( 'NONE', *, *, #33793, .F. ) ;
#36330=CARTESIAN_POINT ( 'NONE',  ( -8.209432707284955555, 0.3640475087720992375, 12.55409154915480308 ) ) ;
#36333=CIRCLE ( 'NONE', #87434, 14.49999999999999822 ) ;
#36336=AXIS2_PLACEMENT_3D ( 'NONE', #14235, #98244, #29703 ) ;
#36345=EDGE_CURVE ( 'NONE', #29582, #47699, #1027, .T. ) ;
#36350=CARTESIAN_POINT ( 'NONE',  ( -14.16722289976678617, 0.5000000000000004441, -4.928467845925704083 ) ) ;
#36353=CARTESIAN_POINT ( 'NONE',  ( -4.289191146912808207E-15, 8.868033628982656680, -11.25000000000000178 ) ) ;
#36359=LINE ( 'NONE', #35369, #72709 ) ;
#36364=DIRECTION ( 'NONE',  ( 0.000000000000000000, 0.000000000000000000, 1.000000000000000000 ) ) ;
#36365=B_SPLINE_CURVE_WITH_KNOTS ( 'NONE', 3,
 ( #11058, #24601, #18073, #70583, #55067, #87052 ),
 .UNSPECIFIED., .F., .F.,
 ( 4, 2, 4 ),
 ( 0.0002800005319459032628, 0.0006862057665691756025, 0.001092411001192447996 ),
 .UNSPECIFIED. ) ;
#36367=EDGE_CURVE ( 'NONE', #9889, #12702, #11454, .T. ) ;
#36376=B_SPLINE_CURVE_WITH_KNOTS ( 'NONE', 3,
 ( #35258, #18799, #80276, #96281, #18305, #10805 ),
 .UNSPECIFIED., .F., .F.,
 ( 4, 2, 4 ),
 ( 0.0002800338592528457487, 0.0006862394199277645993, 0.001092444980602683613 ),
 .UNSPECIFIED. ) ;
#36382=CARTESIAN_POINT ( 'NONE',  ( 0.000000000000000000, 0.5000000000000004441, 0.000000000000000000 ) ) ;
#36389=EDGE_CURVE ( 'NONE', #27786, #79719, #73192, .T. ) ;
#36390=LINE ( 'NONE', #5416, #62840 ) ;
#36397=FACE_OUTER_BOUND ( 'NONE', #65577, .T. ) ;
#36401=CARTESIAN_POINT ( 'NONE',  ( -5.817157072110894056, 0.3639308157993875747, 13.82608706751086913 ) ) ;
#36413=FACE_OUTER_BOUND ( 'NONE', #80341, .T. ) ;
#36420=EDGE_LOOP ( 'NONE', ( #43954, #77723, #47168, #50962 ) ) ;
#36427=TOROIDAL_SURFACE ( 'NONE', #74743, 14.49999999999999822, 0.5000000000000000000 ) ;
#36428=ORIENTED_EDGE ( 'NONE', *, *, #79964, .T. ) ;
#36436=DIRECTION ( 'NONE',  ( 0.000000000000000000, 1.000000000000000000, 0.000000000000000000 ) ) ;
#36443=CARTESIAN_POINT ( 'NONE',  ( -9.382169495545422677, -16.50136533006957862, -9.382169495545417348 ) ) ;
#36444=VECTOR ( 'NONE', #61185, 1000.000000000000000 ) ;
#36453=CIRCLE ( 'NONE', #9316, 14.49999999999999822 ) ;
#36454=VECTOR ( 'NONE', #76030, 999.9999999999998863 ) ;
#36455=DIRECTION ( 'NONE',  ( -0.8526401643540884034, 0.000000000000000000, -0.5224985647159551272 ) ) ;
#36456=ORIENTED_EDGE ( 'NONE', *, *, #35991, .T. ) ;
#36470=FACE_OUTER_BOUND ( 'NONE', #53381, .T. ) ;
#36473=ORIENTED_EDGE ( 'NONE', *, *, #93228, .F. ) ;
#36474=EDGE_CURVE ( 'NONE', #81080, #23413, #66107, .T. ) ;
#36479=ADVANCED_FACE ( 'NONE', ( #50928 ), #89422, .F. ) ;
#36481=EDGE_CURVE ( 'NONE', #56358, #60281, #50478, .T. ) ;
#36490=CARTESIAN_POINT ( 'NONE',  ( 10.70613742633251420, 4.218616272510096815E-16, 9.778988772285311271 ) ) ;
#36497=CARTESIAN_POINT ( 'NONE',  ( 0.000000000000000000, 14.49999999999999822, 0.000000000000000000 ) ) ;
#36500=CARTESIAN_POINT ( 'NONE',  ( -10.36894250292379205, -18.82125116508602858, -10.36894250292378672 ) ) ;
#36510=CARTESIAN_POINT ( 'NONE',  ( 0.000000000000000000, 0.000000000000000000, -14.25000000000000000 ) ) ;
#36517=CARTESIAN_POINT ( 'NONE',  ( -5.440088680355558814, 22.23035201082151957, -9.422509992056136596 ) ) ;
#36528=TOROIDAL_SURFACE ( 'NONE', #92399, 14.49999999999999822, 0.5000000000000000000 ) ;
#36530=B_SPLINE_CURVE_WITH_KNOTS ( 'NONE', 3,
 ( #58370, #59861, #44369, #29358, #90348, #88398 ),
 .UNSPECIFIED., .F., .F.,
 ( 4, 2, 4 ),
 ( 0.0002800364959418003225, 0.0006862420824208872745, 0.001092447668899974335 ),
 .UNSPECIFIED. ) ;
#36535=CARTESIAN_POINT ( 'NONE',  ( 11.92686044187656869, 10.37045670184114599, -3.195792623639533758 ) ) ;
#36538=ORIENTED_EDGE ( 'NONE', *, *, #61077, .T. ) ;
#36549=CARTESIAN_POINT ( 'NONE',  ( 6.090257717040610252, 15.00000000000000533, -13.29726560978568806 ) ) ;
#36552=EDGE_LOOP ( 'NONE', ( #62152, #63128, #28101, #65531 ) ) ;
#36564=CARTESIAN_POINT ( 'NONE',  ( 12.80781515976314822, -0.03417435944610275333, -6.246788841744324472 ) ) ;
#36567=CARTESIAN_POINT ( 'NONE',  ( 2.638427012816829897, 19.55059781766745175, -9.846743663894592657 ) ) ;
#36569=ORIENTED_EDGE ( 'NONE', *, *, #2134, .T. ) ;
#36570=CARTESIAN_POINT ( 'NONE',  ( 1.354709868695649577, 14.49999999999999112, -14.93870011653157448 ) ) ;
#36581=ORIENTED_EDGE ( 'NONE', *, *, #57670, .T. ) ;
#36585=CARTESIAN_POINT ( 'NONE',  ( 7.771322705631503069, 4.156677014937179135E-16, -12.24159072199917375 ) ) ;
#36587=VERTEX_POINT ( 'NONE', #26944 ) ;
#36593=ADVANCED_FACE ( 'NONE', ( #71956 ), #57445, .F. ) ;
#36596=AXIS2_PLACEMENT_3D ( 'NONE', #23055, #59058, #97584 ) ;
#36598=EDGE_CURVE ( 'NONE', #94453, #36109, #1683, .T. ) ;
#36602=CARTESIAN_POINT ( 'NONE',  ( 0.000000000000000000, 14.49999999999999822, 0.000000000000000000 ) ) ;
#36603=EDGE_CURVE ( 'NONE', #26702, #91250, #18303, .T. ) ;
#36606=CARTESIAN_POINT ( 'NONE',  ( -10.65450226470440676, 12.60126542628704627, -3.926157240590227193 ) ) ;
#36607=CARTESIAN_POINT ( 'NONE',  ( 14.43100913236850502, 4.664102659404345836E-16, -1.412789942453164693 ) ) ;
#36611=DIRECTION ( 'NONE',  ( 0.000000000000000000, 1.000000000000000000, 0.000000000000000000 ) ) ;
#36615=FACE_OUTER_BOUND ( 'NONE', #460, .T. ) ;
#36622=EDGE_CURVE ( 'NONE', #18004, #91280, #82768, .T. ) ;
#36623=ADVANCED_FACE ( 'NONE', ( #21929 ), #5742, .T. ) ;
#36624=ORIENTED_EDGE ( 'NONE', *, *, #3671, .F. ) ;
#36632=CARTESIAN_POINT ( 'NONE',  ( -9.065164099344372062, 14.49999999999999822, -11.95084933600779742 ) ) ;
#36633=LINE ( 'NONE', #47443, #95103 ) ;
#36638=CARTESIAN_POINT ( 'NONE',  ( 7.964842623401181321, -5.061314655845157162, 7.964842623401174215 ) ) ;
#36641=CARTESIAN_POINT ( 'NONE',  ( 14.91937968691864747, 0.2306972965111891982, 0.8063277559919165283 ) ) ;
#36649=ORIENTED_EDGE ( 'NONE', *, *, #77270, .T. ) ;
#36651=B_SPLINE_CURVE_WITH_KNOTS ( 'NONE', 3,
 ( #14267, #38737, #275, #54211, #83246, #52251 ),
 .UNSPECIFIED., .F., .F.,
 ( 4, 2, 4 ),
 ( 0.0002800338592536502809, 0.0006862394199285692942, 0.001092444980603488307 ),
 .UNSPECIFIED. ) ;
#36660=LINE ( 'NONE', #89155, #54351 ) ;
#36663=DIRECTION ( 'NONE',  ( 0.000000000000000000, 1.000000000000000000, 0.000000000000000000 ) ) ;
#36667=CARTESIAN_POINT ( 'NONE',  ( -14.64885433385998326, 0.04922511925147129291, -1.748475581354406616 ) ) ;
#36682=VECTOR ( 'NONE', #44382, 1000.000000000000000 ) ;
#36683=CARTESIAN_POINT ( 'NONE',  ( -2.638427012816840111, -30.03273551566588040, -9.846743663894590881 ) ) ;
#36685=CARTESIAN_POINT ( 'NONE',  ( 0.3093388210927642268, 14.49999999999999822, -14.99680997725065978 ) ) ;
#36686=ORIENTED_EDGE ( 'NONE', *, *, #70683, .T. ) ;
#36688=AXIS2_PLACEMENT_3D ( 'NONE', #96851, #79366, #10873 ) ;
#36690=DIRECTION ( 'NONE',  ( 0.000000000000000000, 0.7071067811865465735, 0.7071067811865485719 ) ) ;
#36695=DIRECTION ( 'NONE',  ( 0.000000000000000000, 1.000000000000000000, 0.000000000000000000 ) ) ;
#36697=AXIS2_PLACEMENT_3D ( 'NONE', #68516, #46978, #91505 ) ;
#36700=CARTESIAN_POINT ( 'NONE',  ( -5.204170427930421283E-15, 27.87363466993042493, -12.81628187352647608 ) ) ;
#36704=ORIENTED_EDGE ( 'NONE', *, *, #8830, .T. ) ;
#36708=CARTESIAN_POINT ( 'NONE',  ( 14.48718990079892066, 15.00000000000000000, 0.6093675230841449908 ) ) ;
#36711=CARTESIAN_POINT ( 'NONE',  ( 6.898461952320432466, 4.226027835726576547E-16, -12.75387089053309175 ) ) ;
#36716=CARTESIAN_POINT ( 'NONE',  ( -0.3093388210927753845, 0.3625444014373740975, -14.99680997725068821 ) ) ;
#36726=CARTESIAN_POINT ( 'NONE',  ( -14.49440716394874151, 3.911302179139366829E-16, 0.4026921475165256004 ) ) ;
#36738=ADVANCED_FACE ( 'NONE', ( #30387 ), #15427, .F. ) ;
#36739=ORIENTED_EDGE ( 'NONE', *, *, #55802, .F. ) ;
#36740=CARTESIAN_POINT ( 'NONE',  ( -5.625000000000007994, 4.284700295649321866, -9.742785792574931492 ) ) ;
#36747=AXIS2_PLACEMENT_3D ( 'NONE', #87299, #86329, #25829 ) ;
#36752=CARTESIAN_POINT ( 'NONE',  ( 1.847340224724751456, 0.04922511925147066841, 14.63671528203493288 ) ) ;
#36753=CARTESIAN_POINT ( 'NONE',  ( -7.082119434687058401, 15.97041550158064638, -12.26659068614894110 ) ) ;
#36756=CARTESIAN_POINT ( 'NONE',  ( -10.19513985507841980, 0.3639309290920410001, 11.00268709613213503 ) ) ;
#36760=ORIENTED_EDGE ( 'NONE', *, *, #33525, .T. ) ;
#36764=CARTESIAN_POINT ( 'NONE',  ( 2.120353041430538266, 15.00000000000000000, 14.34413130794944635 ) ) ;
#36765=DIRECTION ( 'NONE',  ( 0.000000000000000000, 0.000000000000000000, 1.000000000000000000 ) ) ;
#36773=CARTESIAN_POINT ( 'NONE',  ( -14.56372689393802311, 14.95037103587093874, 2.356940382831874015 ) ) ;
#36786=ORIENTED_EDGE ( 'NONE', *, *, #66771, .T. ) ;
#36788=DIRECTION ( 'NONE',  ( 0.3826834323650877279, 0.000000000000000000, 0.9238795325112876267 ) ) ;
#36793=DIRECTION ( 'NONE',  ( -0.000000000000000000, -1.000000000000000000, -0.000000000000000000 ) ) ;
#36813=ORIENTED_EDGE ( 'NONE', *, *, #58991, .F. ) ;
#36815=VECTOR ( 'NONE', #69969, 1000.000000000000000 ) ;
#36823=DIRECTION ( 'NONE',  ( -0.9099612708765455471, 0.000000000000000000, 0.4146932426562339180 ) ) ;
#36827=ORIENTED_EDGE ( 'NONE', *, *, #57066, .T. ) ;
#36831=CARTESIAN_POINT ( 'NONE',  ( 14.71525861348291464, 14.63606890215477918, 2.908807992686703425 ) ) ;
#36832=B_SPLINE_CURVE_WITH_KNOTS ( 'NONE', 3,
 ( #22550, #6542, #76518, #53020, #83535, #15054 ),
 .UNSPECIFIED., .F., .F.,
 ( 4, 2, 4 ),
 ( 0.0002800015744541034719, 0.0006862068192693090464, 0.001092412064084514675 ),
 .UNSPECIFIED. ) ;
#36838=CIRCLE ( 'NONE', #71950, 15.00000000000000000 ) ;
#36841=DIRECTION ( 'NONE',  ( 0.000000000000000000, 1.000000000000000000, -0.000000000000000000 ) ) ;
#36849=CARTESIAN_POINT ( 'NONE',  ( -10.93781366033354274, 14.49999999999999822, 10.26470809774057891 ) ) ;
#36850=CARTESIAN_POINT ( 'NONE',  ( 7.313705784284555200, 14.49999999999999112, 13.09617149020753146 ) ) ;
#36864=CARTESIAN_POINT ( 'NONE',  ( -9.898881779040801021, 15.00000000000000000, 10.25059215482569641 ) ) ;
#36871=CARTESIAN_POINT ( 'NONE',  ( 11.92686044187656513, 2.007122731651787007, 2.779367613825428407 ) ) ;
#36877=ORIENTED_EDGE ( 'NONE', *, *, #20069, .F. ) ;
#36884=AXIS2_PLACEMENT_3D ( 'NONE', #65274, #64778, #56328 ) ;
#36888=DIRECTION ( 'NONE',  ( -0.8870108331782244893, 0.000000000000000000, 0.4617486132350284156 ) ) ;
#36889=EDGE_CURVE ( 'NONE', #1776, #45067, #33862, .T. ) ;
#36895=CYLINDRICAL_SURFACE ( 'NONE', #49437, 15.00000000000000000 ) ;
#36896=DIRECTION ( 'NONE',  ( -0.9426414910921759871, 0.000000000000000000, -0.3338068592337775642 ) ) ;
#36904=DIRECTION ( 'NONE',  ( 0.04361938736533305799, -0.000000000000000000, 0.9990482215818579093 ) ) ;
#36917=TOROIDAL_SURFACE ( 'NONE', #75232, 14.49999999999999822, 0.5000000000000000000 ) ;
#36919=CIRCLE ( 'NONE', #68903, 14.49999999999999822 ) ;
#36930=DIRECTION ( 'NONE',  ( 3.552713678800500929E-14, 0.000000000000000000, 1.000000000000000000 ) ) ;
#36935=CARTESIAN_POINT ( 'NONE',  ( -3.927832320392339316, 15.00000000000000000, 13.69797916712101404 ) ) ;
#36938=VERTEX_POINT ( 'NONE', #78901 ) ;
#36940=CARTESIAN_POINT ( 'NONE',  ( -11.09922568453594316, -20.45969866340291077, 6.408140936763246920 ) ) ;
#36951=ORIENTED_EDGE ( 'NONE', *, *, #93389, .F. ) ;
#36957=ORIENTED_EDGE ( 'NONE', *, *, #98268, .T. ) ;
#36965=CARTESIAN_POINT ( 'NONE',  ( -6.382347221874564269, 14.49999999999999112, 13.57444820018227993 ) ) ;
#36968=ORIENTED_EDGE ( 'NONE', *, *, #20881, .F. ) ;
#36973=CARTESIAN_POINT ( 'NONE',  ( -14.88232117145532385, 0.5000000000000004441, 1.875237731503040628 ) ) ;
#36980=CARTESIAN_POINT ( 'NONE',  ( 0.000000000000000000, 0.5000000000000004441, 0.000000000000000000 ) ) ;
#36984=VECTOR ( 'NONE', #57757, 1000.000000000000000 ) ;
#36985=ORIENTED_EDGE ( 'NONE', *, *, #77348, .T. ) ;
#36993=CARTESIAN_POINT ( 'NONE',  ( 7.082119434687047743, -14.86291783175269465, -12.26659068614894821 ) ) ;
#37006=CARTESIAN_POINT ( 'NONE',  ( 1.175527996597014457, 15.00000000000000888, 14.57931687975696811 ) ) ;
#37008=CARTESIAN_POINT ( 'NONE',  ( 2.915334737309921209, 26.60535201082150891, -10.88017736071110164 ) ) ;
#37019=AXIS2_PLACEMENT_3D ( 'NONE', #91608, #53597, #46111 ) ;
#37020=CIRCLE ( 'NONE', #19308, 14.49999999999999822 ) ;
#37023=B_SPLINE_CURVE_WITH_KNOTS ( 'NONE', 3,
 ( #70951, #2470, #32928, #54444, #16464, #93933 ),
 .UNSPECIFIED., .F., .F.,
 ( 4, 2, 4 ),
 ( 0.0002800858945027832718, 0.0006862919646584851509, 0.001092498034814187030 ),
 .UNSPECIFIED. ) ;
#37027=EDGE_CURVE ( 'NONE', #77111, #70022, #85922, .T. ) ;
#37030=VERTEX_POINT ( 'NONE', #32407 ) ;
#37031=DIRECTION ( 'NONE',  ( -0.9762960071199316969, 0.000000000000000000, -0.2164396139381103701 ) ) ;
#37036=CARTESIAN_POINT ( 'NONE',  ( 0.000000000000000000, 15.00000000000000000, 0.000000000000000000 ) ) ;
#37040=AXIS2_PLACEMENT_3D ( 'NONE', #82089, #75084, #52094 ) ;
#37041=CARTESIAN_POINT ( 'NONE',  ( 5.991992585808628036, 15.00000000000000000, -13.20401548210295140 ) ) ;
#37042=EDGE_CURVE ( 'NONE', #97109, #93052, #91081, .T. ) ;
#37051=CARTESIAN_POINT ( 'NONE',  ( 4.265913727722193904, 14.95037113646324478, -14.12300574719579416 ) ) ;
#37056=EDGE_CURVE ( 'NONE', #16083, #32902, #64374, .T. ) ;
#37057=EDGE_CURVE ( 'NONE', #3541, #2122, #60779, .T. ) ;
#37059=CARTESIAN_POINT ( 'NONE',  ( 0.000000000000000000, 15.00000000000000000, 0.000000000000000000 ) ) ;
#37061=DIRECTION ( 'NONE',  ( 0.000000000000000000, 0.000000000000000000, 1.000000000000000000 ) ) ;
#37062=CARTESIAN_POINT ( 'NONE',  ( 9.846743663894590881, 13.30059781766745708, 2.638427012816828565 ) ) ;
#37065=CARTESIAN_POINT ( 'NONE',  ( -14.19749592853509768, 15.00000000000000000, 7.369430493279844008 ) ) ;
#37077=VERTEX_POINT ( 'NONE', #42874 ) ;
#37081=EDGE_CURVE ( 'NONE', #71137, #11622, #34865, .T. ) ;
#37083=EDGE_LOOP ( 'NONE', ( #16176, #73656, #16405, #89677, #25382, #85373 ) ) ;
#37087=FACE_OUTER_BOUND ( 'NONE', #52149, .T. ) ;
#37097=AXIS2_PLACEMENT_3D ( 'NONE', #85010, #19333, #55993 ) ;
#37098=VERTEX_POINT ( 'NONE', #50865 ) ;
#37109=CARTESIAN_POINT ( 'NONE',  ( 0.000000000000000000, 0.000000000000000000, 0.000000000000000000 ) ) ;
#37116=B_SPLINE_CURVE_WITH_KNOTS ( 'NONE', 3,
 ( #47140, #86998, #76663, #77637, #33483, #63980 ),
 .UNSPECIFIED., .F., .F.,
 ( 4, 2, 4 ),
 ( 3.409110551494641268E-05, 0.0004400426677367931852, 0.0008459942299586398901 ),
 .UNSPECIFIED. ) ;
#37118=ORIENTED_EDGE ( 'NONE', *, *, #67558, .F. ) ;
#37127=CARTESIAN_POINT ( 'NONE',  ( -4.267749253172081758, 0.000000000000000000, 3.394721039305316879 ) ) ;
#37128=AXIS2_PLACEMENT_3D ( 'NONE', #87980, #66463, #73464 ) ;
#37132=CARTESIAN_POINT ( 'NONE',  ( -10.88017736071110342, -16.93631465584515539, 3.903127820947815962E-15 ) ) ;
#37136=CARTESIAN_POINT ( 'NONE',  ( 14.94699059465101598, 14.63595249122788999, 1.259949270174913316 ) ) ;
#37137=EDGE_CURVE ( 'NONE', #74265, #59795, #51849, .T. ) ;
#37141=CIRCLE ( 'NONE', #94579, 15.00000000000000000 ) ;
#37144=DIRECTION ( 'NONE',  ( -0.9426414910921805390, 0.000000000000000000, 0.3338068592337649076 ) ) ;
#37160=EDGE_CURVE ( 'NONE', #89788, #44051, #12368, .T. ) ;
#37161=VERTEX_POINT ( 'NONE', #73357 ) ;
#37181=ADVANCED_FACE ( 'NONE', ( #57860 ), #4884, .F. ) ;
#37183=VECTOR ( 'NONE', #40550, 1000.000000000000000 ) ;
#37186=CIRCLE ( 'NONE', #59497, 14.49999999999999822 ) ;
#37188=CARTESIAN_POINT ( 'NONE',  ( -8.527530157486182816, -24.40773551566587685, -4.923371831947288335 ) ) ;
#37190=FACE_OUTER_BOUND ( 'NONE', #93026, .T. ) ;
#37192=VERTEX_POINT ( 'NONE', #89354 ) ;
#37201=CARTESIAN_POINT ( 'NONE',  ( 6.408140936763236262, 22.45696800326375708, -11.09922568453595026 ) ) ;
#37204=B_SPLINE_CURVE_WITH_KNOTS ( 'NONE', 3,
 ( #61388, #7917, #38413, #15908, #67925, #84891 ),
 .UNSPECIFIED., .F., .F.,
 ( 4, 2, 4 ),
 ( 0.0002800008091676931660, 0.0006862060465022924369, 0.001092411283836891654 ),
 .UNSPECIFIED. ) ;
#37207=ORIENTED_EDGE ( 'NONE', *, *, #45495, .T. ) ;
#37208=CIRCLE ( 'NONE', #49959, 14.49999999999999822 ) ;
#37214=FACE_OUTER_BOUND ( 'NONE', #21881, .T. ) ;
#37219=ORIENTED_EDGE ( 'NONE', *, *, #44824, .F. ) ;
#37221=DIRECTION ( 'NONE',  ( -0.000000000000000000, -1.000000000000000000, -0.000000000000000000 ) ) ;
#37222=LINE ( 'NONE', #67707, #61053 ) ;
#37224=CARTESIAN_POINT ( 'NONE',  ( 0.000000000000000000, 15.00000000000000000, 0.000000000000000000 ) ) ;
#37227=EDGE_LOOP ( 'NONE', ( #14372, #91786, #13160, #9643 ) ) ;
#37242=AXIS2_PLACEMENT_3D ( 'NONE', #36602, #4630, #20103 ) ;
#37243=VERTEX_POINT ( 'NONE', #80870 ) ;
#37244=DIRECTION ( 'NONE',  ( 0.000000000000000000, 1.000000000000000000, 0.000000000000000000 ) ) ;
#37249=LINE ( 'NONE', #77190, #66708 ) ;
#37252=DIRECTION ( 'NONE',  ( 0.000000000000000000, 0.000000000000000000, -1.000000000000000000 ) ) ;
#37256=PLANE ( 'NONE',  #72881 ) ;
#37257=VECTOR ( 'NONE', #58833, 1000.000000000000000 ) ;
#37258=CARTESIAN_POINT ( 'NONE',  ( 7.082119434687047743, 15.13708216824730890, -12.26659068614894821 ) ) ;
#37271=DIRECTION ( 'NONE',  ( 0.000000000000000000, 0.000000000000000000, 1.000000000000000000 ) ) ;
#37275=VERTEX_POINT ( 'NONE', #90826 ) ;
#37284=CARTESIAN_POINT ( 'NONE',  ( 4.841308736149698255, 0.2301500557980281081, -14.13449535775533050 ) ) ;
#37286=AXIS2_PLACEMENT_3D ( 'NONE', #5650, #12148, #73129 ) ;
#37290=EDGE_CURVE ( 'NONE', #71843, #80716, #79148, .T. ) ;
#37291=ORIENTED_EDGE ( 'NONE', *, *, #52783, .F. ) ;
#37293=CARTESIAN_POINT ( 'NONE',  ( 9.742785792574936821, 5.838468844518209799, -5.625000000000004441 ) ) ;
#37300=EDGE_CURVE ( 'NONE', #21605, #70392, #55309, .T. ) ;
#37309=ORIENTED_EDGE ( 'NONE', *, *, #45060, .T. ) ;
#37318=VERTEX_POINT ( 'NONE', #42628 ) ;
#37321=ORIENTED_EDGE ( 'NONE', *, *, #10567, .F. ) ;
#37322=CIRCLE ( 'NONE', #85195, 14.49999999999999822 ) ;
#37323=EDGE_CURVE ( 'NONE', #62057, #51581, #68061, .T. ) ;
#37324=ORIENTED_EDGE ( 'NONE', *, *, #27880, .F. ) ;
#37328=CARTESIAN_POINT ( 'NONE',  ( 13.86186289918442505, 1.490777987167568597E-16, 4.667665767315075875 ) ) ;
#37334=VERTEX_POINT ( 'NONE', #34615 ) ;
#37337=DIRECTION ( 'NONE',  ( 0.000000000000000000, 1.000000000000000000, 0.000000000000000000 ) ) ;
#37354=ORIENTED_EDGE ( 'NONE', *, *, #49422, .F. ) ;
#37359=ORIENTED_EDGE ( 'NONE', *, *, #6837, .T. ) ;
#37362=FACE_OUTER_BOUND ( 'NONE', #54130, .T. ) ;
#37366=DIRECTION ( 'NONE',  ( 0.000000000000000000, 1.000000000000000000, 0.000000000000000000 ) ) ;
#37370=DIRECTION ( 'NONE',  ( 0.000000000000000000, 0.000000000000000000, 1.000000000000000000 ) ) ;
#37374=DIRECTION ( 'NONE',  ( 8.881784197001252323E-16, 0.000000000000000000, 1.000000000000000000 ) ) ;
#37379=ORIENTED_EDGE ( 'NONE', *, *, #97512, .F. ) ;
#37383=DIRECTION ( 'NONE',  ( 0.000000000000000000, 1.000000000000000000, 0.000000000000000000 ) ) ;
#37390=ORIENTED_EDGE ( 'NONE', *, *, #55770, .F. ) ;
#37391=CIRCLE ( 'NONE', #8612, 14.49999999999999822 ) ;
#37393=CARTESIAN_POINT ( 'NONE',  ( 14.88232117145529720, 15.00000000000000000, 1.875237731503240024 ) ) ;
#37398=DIRECTION ( 'NONE',  ( -0.2334453638559087219, 0.000000000000000000, 0.9723699203976758909 ) ) ;
#37399=DIRECTION ( 'NONE',  ( 0.000000000000000000, 1.000000000000000000, 0.000000000000000000 ) ) ;
#37404=CARTESIAN_POINT ( 'NONE',  ( -10.32896413005680536, 2.245456701841147762, -5.963430220938272797 ) ) ;
#37409=B_SPLINE_CURVE_WITH_KNOTS ( 'NONE', 3,
 ( #56332, #18824, #3324, #11308, #64294, #95806 ),
 .UNSPECIFIED., .F., .F.,
 ( 4, 2, 4 ),
 ( 3.409110551493783393E-05, 0.0004400426677367841322, 0.0008459942299586303491 ),
 .UNSPECIFIED. ) ;
#37435=DIRECTION ( 'NONE',  ( 0.000000000000000000, 1.000000000000000000, 0.000000000000000000 ) ) ;
#37440=VERTEX_POINT ( 'NONE', #80128 ) ;
#37442=CARTESIAN_POINT ( 'NONE',  ( 6.408140936763243367, -14.20969866340290899, 11.09922568453594494 ) ) ;
#37450=EDGE_CURVE ( 'NONE', #37161, #17162, #12127, .T. ) ;
#37451=VECTOR ( 'NONE', #10038, 1000.000000000000000 ) ;
#37452=CARTESIAN_POINT ( 'NONE',  ( -9.519554572442809004, -3.087435092741923553E-15, -11.10344954678193119 ) ) ;
#37454=B_SPLINE_CURVE_WITH_KNOTS ( 'NONE', 3,
 ( #11304, #80791, #37637, #96302, #50274, #43275 ),
 .UNSPECIFIED., .F., .F.,
 ( 4, 2, 4 ),
 ( 0.0002800005319541506261, 0.0006862057665733079306, 0.001092411001192465344 ),
 .UNSPECIFIED. ) ;
#37459=AXIS2_PLACEMENT_3D ( 'NONE', #66511, #66007, #97037 ) ;
#37469=CARTESIAN_POINT ( 'NONE',  ( 0.4278561937608114096, 0.000000000000000000, 5.436428395565744864 ) ) ;
#37471=ORIENTED_EDGE ( 'NONE', *, *, #77348, .F. ) ;
#37473=LINE ( 'NONE', #67962, #72529 ) ;
#37492=CARTESIAN_POINT ( 'NONE',  ( -9.520529577030321988, 15.00000000000000888, -11.10395710204432973 ) ) ;
#37493=EDGE_CURVE ( 'NONE', #48192, #3803, #93624, .T. ) ;
#37495=CARTESIAN_POINT ( 'NONE',  ( 14.16423886937410437, -20.90458449841936428, 3.795296366450304770 ) ) ;
#37499=ORIENTED_EDGE ( 'NONE', *, *, #85946, .T. ) ;
#37509=CARTESIAN_POINT ( 'NONE',  ( -7.964842623401172439, 23.68868534415484106, 7.964842623401183097 ) ) ;
#37516=VERTEX_POINT ( 'NONE', #4646 ) ;
#37519=CARTESIAN_POINT ( 'NONE',  ( 0.000000000000000000, 12.49999999999999112, 0.000000000000000000 ) ) ;
#37521=MECHANICAL_DESIGN_GEOMETRIC_PRESENTATION_REPRESENTATION('',(#59829),#56627);
#37527=CARTESIAN_POINT ( 'NONE',  ( -5.093587308868599450, -0.03417435944610275333, 15.16353404595993837 ) ) ;
#37530=EDGE_LOOP ( 'NONE', ( #57993, #1662, #71146, #32987, #95393, #97834 ) ) ;
#37540=PLANE ( 'NONE',  #34717 ) ;
#37545=ORIENTED_EDGE ( 'NONE', *, *, #91912, .F. ) ;
#37551=CARTESIAN_POINT ( 'NONE',  ( -4.265659168453120209, 14.95077488074853456, -14.12268572233456787 ) ) ;
#37557=CARTESIAN_POINT ( 'NONE',  ( -12.34086200392816757, 0.000000000000000000, -7.125000000000143885 ) ) ;
#37560=CARTESIAN_POINT ( 'NONE',  ( -9.846743663894594434, 21.00893115100079100, 3.469446951953614189E-15 ) ) ;
#37562=ORIENTED_EDGE ( 'NONE', *, *, #71865, .F. ) ;
#37571=EDGE_CURVE ( 'NONE', #57022, #96588, #47366, .T. ) ;
#37574=ORIENTED_EDGE ( 'NONE', *, *, #54836, .T. ) ;
#37579=VERTEX_POINT ( 'NONE', #67105 ) ;
#37588=ORIENTED_EDGE ( 'NONE', *, *, #44271, .F. ) ;
#37589=LINE ( 'NONE', #61548, #39460 ) ;
#37590=AXIS2_PLACEMENT_3D ( 'NONE', #20856, #88853, #51346 ) ;
#37599=ORIENTED_EDGE ( 'NONE', *, *, #7727, .T. ) ;
#37600=CARTESIAN_POINT ( 'NONE',  ( -5.963430220938290560, 3.854976035794183353, -10.32896413005679648 ) ) ;
#37602=DIRECTION ( 'NONE',  ( 0.000000000000000000, 0.000000000000000000, 1.000000000000000000 ) ) ;
#37608=( GEOMETRIC_REPRESENTATION_CONTEXT ( 3 ) GLOBAL_UNCERTAINTY_ASSIGNED_CONTEXT ( ( #50154 ) ) GLOBAL_UNIT_ASSIGNED_CONTEXT ( ( #94015, #64481, #55020 ) ) REPRESENTATION_CONTEXT ( 'NONE', 'WORKASPACE' ) );
#37610=ADVANCED_FACE ( 'NONE', ( #43607 ), #40968, .T. ) ;
#37620=CARTESIAN_POINT ( 'NONE',  ( 5.419894505350582925, 15.00000000000000000, -13.98659156302458761 ) ) ;
#37623=CARTESIAN_POINT ( 'NONE',  ( 5.440088680355556150, -15.26964798917848931, 9.422509992056138373 ) ) ;
#37627=DIRECTION ( 'NONE',  ( -0.7716245833877234395, 0.000000000000000000, 0.6360782202777597316 ) ) ;
#37637=CARTESIAN_POINT ( 'NONE',  ( -13.34989199100162871, 14.95037102702517906, 6.279943681065644157 ) ) ;
#37639=ORIENTED_EDGE ( 'NONE', *, *, #55130, .T. ) ;
#37651=VECTOR ( 'NONE', #61496, 1000.000000000000000 ) ;
#37654=ORIENTED_EDGE ( 'NONE', *, *, #29887, .F. ) ;
#37671=CARTESIAN_POINT ( 'NONE',  ( 8.527530157486179263, -21.90773551566587685, 4.923371831947292776 ) ) ;
#37674=VERTEX_POINT ( 'NONE', #52105 ) ;
#37688=CARTESIAN_POINT ( 'NONE',  ( 6.408140936763236262, 17.45696800326376774, -11.09922568453595026 ) ) ;
#37698=DIRECTION ( 'NONE',  ( 0.000000000000000000, 1.000000000000000000, 0.000000000000000000 ) ) ;
#37701=FACE_OUTER_BOUND ( 'NONE', #76276, .T. ) ;
#37702=CARTESIAN_POINT ( 'NONE',  ( -0.1558782227856948255, 1.143494478793305150E-17, -14.62632331952783993 ) ) ;
#37703=DIRECTION ( 'NONE',  ( 0.000000000000000000, 1.000000000000000000, 0.000000000000000000 ) ) ;
#37707=CARTESIAN_POINT ( 'NONE',  ( 6.742022620658147503, 14.95037102811560281, 13.12259272460509862 ) ) ;
#37709=CYLINDRICAL_SURFACE ( 'NONE', #75486, 15.00000000000000000 ) ;
#37719=EDGE_CURVE ( 'NONE', #54738, #32902, #48936, .T. ) ;
#37726=VECTOR ( 'NONE', #63280, 1000.000000000000227 ) ;
#37727=VECTOR ( 'NONE', #15181, 999.9999999999998863 ) ;
#37735=DIRECTION ( 'NONE',  ( -0.000000000000000000, -1.000000000000000000, -0.000000000000000000 ) ) ;
#37747=CARTESIAN_POINT ( 'NONE',  ( 14.16423886937410082, 14.51208216824730179, -3.795296366450314096 ) ) ;
#37750=ADVANCED_FACE ( 'NONE', ( #75093 ), #17054, .T. ) ;
#37752=CIRCLE ( 'NONE', #71290, 15.00000000000000000 ) ;
#37755=ORIENTED_EDGE ( 'NONE', *, *, #78811, .T. ) ;
#37765=ORIENTED_EDGE ( 'NONE', *, *, #29323, .F. ) ;
#37783=CARTESIAN_POINT ( 'NONE',  ( 1.780824192092403058, 0.5000000000000004441, 14.89391369643514729 ) ) ;
#37796=ORIENTED_EDGE ( 'NONE', *, *, #79282, .T. ) ;
#37799=ORIENTED_EDGE ( 'NONE', *, *, #79922, .T. ) ;
#37801=ORIENTED_EDGE ( 'NONE', *, *, #6118, .T. ) ;
#37807=ORIENTED_EDGE ( 'NONE', *, *, #5865, .T. ) ;
#37813=ORIENTED_EDGE ( 'NONE', *, *, #50365, .F. ) ;
#37818=FACE_OUTER_BOUND ( 'NONE', #23151, .T. ) ;
#37827=DIRECTION ( 'NONE',  ( 0.000000000000000000, 0.000000000000000000, 1.000000000000000000 ) ) ;
#37833=CARTESIAN_POINT ( 'NONE',  ( -10.64017930668212664, 0.5000000000000004441, 10.57291749337208309 ) ) ;
#37839=CARTESIAN_POINT ( 'NONE',  ( 14.88640444357867665, 0.2306972965111609708, -1.277895705730255571 ) ) ;
#37843=FACE_OUTER_BOUND ( 'NONE', #27690, .T. ) ;
#37847=ORIENTED_EDGE ( 'NONE', *, *, #55919, .F. ) ;
#37851=EDGE_CURVE ( 'NONE', #82904, #81875, #61154, .T. ) ;
#37858=DIRECTION ( 'NONE',  ( 0.000000000000000000, 0.000000000000000000, 1.000000000000000000 ) ) ;
#37864=DIRECTION ( 'NONE',  ( 0.000000000000000000, 1.000000000000000000, 0.000000000000000000 ) ) ;
#37865=ORIENTED_EDGE ( 'NONE', *, *, #6805, .F. ) ;
#37866=CARTESIAN_POINT ( 'NONE',  ( 6.715867195167449566, 4.285122813354096929E-16, -12.85095824508326956 ) ) ;
#37868=DIRECTION ( 'NONE',  ( 0.000000000000000000, 0.000000000000000000, 1.000000000000000000 ) ) ;
#37873=ORIENTED_EDGE ( 'NONE', *, *, #3396, .F. ) ;
#37875=TOROIDAL_SURFACE ( 'NONE', #82544, 14.49999999999999822, 0.5000000000000000000 ) ;
#37877=DIRECTION ( 'NONE',  ( -0.8141155183563226760, 0.000000000000000000, 0.5807029557109348872 ) ) ;
#37883=ORIENTED_EDGE ( 'NONE', *, *, #82737, .T. ) ;
#37896=CARTESIAN_POINT ( 'NONE',  ( 14.82679024690671099, 14.76930270348882068, -1.845086899513286527 ) ) ;
#37897=FACE_OUTER_BOUND ( 'NONE', #33668, .T. ) ;
#37899=AXIS2_PLACEMENT_3D ( 'NONE', #27928, #58422, #88936 ) ;
#37900=AXIS2_PLACEMENT_3D ( 'NONE', #86402, #2432, #49859 ) ;
#37903=DIRECTION ( 'NONE',  ( 0.000000000000000000, 0.000000000000000000, 1.000000000000000000 ) ) ;
#37910=CARTESIAN_POINT ( 'NONE',  ( 5.817157072110801685, 14.63595249122789177, -13.82608706751087979 ) ) ;
#37914=B_SPLINE_CURVE_WITH_KNOTS ( 'NONE', 3,
 ( #35374, #20382, #65369, #12379, #89852, #27378 ),
 .UNSPECIFIED., .F., .F.,
 ( 4, 2, 4 ),
 ( 0.0002800032591535108481, 0.0006862085204461408280, 0.001092413781738770916 ),
 .UNSPECIFIED. ) ;
#37923=ORIENTED_EDGE ( 'NONE', *, *, #20324, .T. ) ;
#37926=CARTESIAN_POINT ( 'NONE',  ( -5.817157072110893168, 0.5000000000000004441, 13.82608706751082828 ) ) ;
#37929=CARTESIAN_POINT ( 'NONE',  ( 0.000000000000000000, 0.5000000000000004441, 0.000000000000000000 ) ) ;
#37934=ORIENTED_EDGE ( 'NONE', *, *, #38319, .T. ) ;
#37936=CARTESIAN_POINT ( 'NONE',  ( -9.382169495545422677, -21.50136533006957862, -9.382169495545417348 ) ) ;
#37945=ADVANCED_FACE ( 'NONE', ( #54548 ), #618, .F. ) ;
#37947=DIRECTION ( 'NONE',  ( 0.000000000000000000, 0.000000000000000000, 1.000000000000000000 ) ) ;
#37957=B_SPLINE_CURVE_WITH_KNOTS ( 'NONE', 3,
 ( #23576, #25046, #54045, #84555, #57968, #58457 ),
 .UNSPECIFIED., .F., .F.,
 ( 4, 2, 4 ),
 ( 3.409110551474090893E-05, 0.0004400426677365675086, 0.0008459942299583938846 ),
 .UNSPECIFIED. ) ;
#37960=CARTESIAN_POINT ( 'NONE',  ( 14.56089864660132349, 14.99999999999807088, -1.374314915483334731 ) ) ;
#37964=DIRECTION ( 'NONE',  ( 0.000000000000000000, 1.000000000000000000, 0.000000000000000000 ) ) ;
#37970=EDGE_CURVE ( 'NONE', #32864, #91030, #55042, .T. ) ;
#37974=EDGE_CURVE ( 'NONE', #18747, #79425, #78053, .T. ) ;
#37989=CARTESIAN_POINT ( 'NONE',  ( 14.16423886937410437, -15.90458449841935895, 3.795296366450304770 ) ) ;
#37999=CARTESIAN_POINT ( 'NONE',  ( 2.815433093577016876, 14.63606915880329851, 14.73340885523756327 ) ) ;
#38004=CARTESIAN_POINT ( 'NONE',  ( -5.440088680355558814, 32.23035201082149825, -9.422509992056136596 ) ) ;
#38013=CARTESIAN_POINT ( 'NONE',  ( -13.78891971893217239, 14.49999999999999112, 5.904717858191482094 ) ) ;
#38033=DIRECTION ( 'NONE',  ( 0.000000000000000000, 0.000000000000000000, 1.000000000000000000 ) ) ;
#38035=DIRECTION ( 'NONE',  ( 0.000000000000000000, 0.000000000000000000, -1.000000000000000000 ) ) ;
#38045=CARTESIAN_POINT ( 'NONE',  ( 2.189666204609302724, 2.388632911257126956E-16, -14.46180170876169058 ) ) ;
#38053=CARTESIAN_POINT ( 'NONE',  ( 2.638427012816835227, 12.46726448433412315, 9.846743663894590881 ) ) ;
#38054=ORIENTED_EDGE ( 'NONE', *, *, #8530, .T. ) ;
#38056=CARTESIAN_POINT ( 'NONE',  ( 14.62617646268085281, 15.00000000000000000, 3.327906561566980503 ) ) ;
#38064=ADVANCED_FACE ( 'NONE', ( #92554 ), #9046, .T. ) ;
#38065=B_SPLINE_CURVE_WITH_KNOTS ( 'NONE', 3,
 ( #79899, #50382, #11904, #20885, #34387, #57395 ),
 .UNSPECIFIED., .F., .F.,
 ( 4, 2, 4 ),
 ( 3.409110551496096809E-05, 0.0004400426677367864632, 0.0008459942299586120261 ),
 .UNSPECIFIED. ) ;
#38070=ORIENTED_EDGE ( 'NONE', *, *, #29511, .T. ) ;
#38077=VECTOR ( 'NONE', #58764, 1000.000000000000000 ) ;
#38087=VERTEX_POINT ( 'NONE', #34501 ) ;
#38093=ORIENTED_EDGE ( 'NONE', *, *, #28003, .T. ) ;
#38094=DIRECTION ( 'NONE',  ( -2.042810365310288034E-14, 0.000000000000000000, 1.000000000000000000 ) ) ;
#38100=CARTESIAN_POINT ( 'NONE',  ( 13.21236992757670059, -0.03417435944610275333, 5.338143956176803151 ) ) ;
#38106=VECTOR ( 'NONE', #80078, 1000.000000000000000 ) ;
#38110=ORIENTED_EDGE ( 'NONE', *, *, #90514, .T. ) ;
#38118=DIRECTION ( 'NONE',  ( 0.4461978131097943945, 0.000000000000000000, 0.8949343616020322134 ) ) ;
#38122=CARTESIAN_POINT ( 'NONE',  ( 2.915334737309928315, -15.47798132251182857, 10.88017736071109987 ) ) ;
#38126=CARTESIAN_POINT ( 'NONE',  ( 14.16722289976681814, 0.5000000000000004441, 4.928467845925615265 ) ) ;
#38128=CARTESIAN_POINT ( 'NONE',  ( 13.86102707272223356, -3.662993980401220239E-15, -4.666951904077198954 ) ) ;
#38139=VERTEX_POINT ( 'NONE', #25561 ) ;
#38141=ADVANCED_FACE ( 'NONE', ( #80016 ), #88914, .T. ) ;
#38148=VECTOR ( 'NONE', #81150, 1000.000000000000114 ) ;
#38153=ORIENTED_EDGE ( 'NONE', *, *, #39772, .T. ) ;
#38168=CARTESIAN_POINT ( 'NONE',  ( 4.923371831947295441, -25.65773551566588040, -8.527530157486179263 ) ) ;
#38169=ORIENTED_EDGE ( 'NONE', *, *, #67548, .F. ) ;
#38171=CARTESIAN_POINT ( 'NONE',  ( -13.55255535720589322, -0.03417435944610275333, -4.403492169843143067 ) ) ;
#38180=CARTESIAN_POINT ( 'NONE',  ( -2.258855624577742027, 14.95037108984192820, 14.57926203528949038 ) ) ;
#38182=AXIS2_PLACEMENT_3D ( 'NONE', #96238, #33729, #72233 ) ;
#38185=CARTESIAN_POINT ( 'NONE',  ( 3.469446951953614189E-15, 20.37363466993041783, 12.81628187352647608 ) ) ;
#38186=EDGE_LOOP ( 'NONE', ( #45442, #78881, #1733, #91031 ) ) ;
#38189=ORIENTED_EDGE ( 'NONE', *, *, #77791, .T. ) ;
#38194=CARTESIAN_POINT ( 'NONE',  ( -5.845017550302832987, -0.03417435944610275333, -14.89003580495041668 ) ) ;
#38195=CARTESIAN_POINT ( 'NONE',  ( 10.64017930668204670, 14.49999999999999112, 10.57291749337225362 ) ) ;
#38199=CARTESIAN_POINT ( 'NONE',  ( 0.000000000000000000, 14.49999999999999822, 0.000000000000000000 ) ) ;
#38201=CARTESIAN_POINT ( 'NONE',  ( -14.76044511231849299, 0.2301501264598455332, -2.313329003772577774 ) ) ;
#38202=ORIENTED_EDGE ( 'NONE', *, *, #31510, .T. ) ;
#38205=LINE ( 'NONE', #712, #5340 ) ;
#38211=VECTOR ( 'NONE', #31913, 999.9999999999998863 ) ;
#38213=CARTESIAN_POINT ( 'NONE',  ( -11.42891328973558451, 14.99999999999803002, -9.126250717934663470 ) ) ;
#38217=CARTESIAN_POINT ( 'NONE',  ( -9.282040431732752950, 15.00000000000000888, 11.30407325590330103 ) ) ;
#38223=DIRECTION ( 'NONE',  ( -0.2503800040544323924, 0.000000000000000000, -0.9681476403781101858 ) ) ;
#38225=VERTEX_POINT ( 'NONE', #73000 ) ;
#38231=CARTESIAN_POINT ( 'NONE',  ( -7.618303901328673078, -3.182726299308032341E-15, 12.48478900416256288 ) ) ;
#38237=CARTESIAN_POINT ( 'NONE',  ( 7.082119434687054849, 18.47041550158062861, 12.26659068614894288 ) ) ;
#38240=CARTESIAN_POINT ( 'NONE',  ( 0.000000000000000000, 0.5000000000000004441, 0.000000000000000000 ) ) ;
#38242=EDGE_CURVE ( 'NONE', #29326, #52526, #24158, .T. ) ;
#38255=ORIENTED_EDGE ( 'NONE', *, *, #70369, .F. ) ;
#38266=CARTESIAN_POINT ( 'NONE',  ( 5.817157072110704874, 0.5000000000000004441, 13.82608706751090821 ) ) ;
#38271=VERTEX_POINT ( 'NONE', #11033 ) ;
#38273=CARTESIAN_POINT ( 'NONE',  ( -14.48718990079892954, 4.238615592650390652E-16, 0.6093675230839495915 ) ) ;
#38274=CARTESIAN_POINT ( 'NONE',  ( 3.014428414850127691, 6.463468844518203582, -11.25000000000000000 ) ) ;
#38287=ORIENTED_EDGE ( 'NONE', *, *, #65694, .F. ) ;
#38291=VERTEX_POINT ( 'NONE', #94525 ) ;
#38295=VECTOR ( 'NONE', #46355, 1000.000000000000000 ) ;
#38296=CARTESIAN_POINT ( 'NONE',  ( 3.843478602184544624, 14.76930270348881535, -14.43834224996323101 ) ) ;
#38300=EDGE_CURVE ( 'NONE', #70551, #243, #92129, .T. ) ;
#38311=ORIENTED_EDGE ( 'NONE', *, *, #2317, .T. ) ;
#38319=EDGE_CURVE ( 'NONE', #27398, #58242, #53800, .T. ) ;
#38320=CARTESIAN_POINT ( 'NONE',  ( -6.382347221874242749, 15.00000000000000000, -13.57444820018235987 ) ) ;
#38327=LINE ( 'NONE', #97855, #83570 ) ;
#38328=DIRECTION ( 'NONE',  ( 0.000000000000000000, 0.000000000000000000, 1.000000000000000000 ) ) ;
#38332=CARTESIAN_POINT ( 'NONE',  ( -2.621477372531479055, 15.00000000000000000, -15.77990027919564575 ) ) ;
#38342=ORIENTED_EDGE ( 'NONE', *, *, #29792, .F. ) ;
#38348=DIRECTION ( 'NONE',  ( 0.7716245833877105609, 0.000000000000000000, 0.6360782202777752747 ) ) ;
#38356=DIRECTION ( 'NONE',  ( -0.000000000000000000, -1.000000000000000000, -0.000000000000000000 ) ) ;
#38362=CARTESIAN_POINT ( 'NONE',  ( -13.30119215211272810, 14.76984893004878785, -6.804450086557387145 ) ) ;
#38375=CARTESIAN_POINT ( 'NONE',  ( 14.91886229468041947, 0.2301503527634121971, -0.8060919667644429465 ) ) ;
#38380=CARTESIAN_POINT ( 'NONE',  ( -5.888281321711915872, 1.823139558123406223, -10.37198838585826266 ) ) ;
#38382=ADVANCED_FACE ( 'NONE', ( #35499 ), #36236, .T. ) ;
#38384=AXIS2_PLACEMENT_3D ( 'NONE', #10224, #73154, #40713 ) ;
#38410=CARTESIAN_POINT ( 'NONE',  ( 14.04867373755350890, 15.00000000000000000, 7.649324326489743697 ) ) ;
#38413=CARTESIAN_POINT ( 'NONE',  ( -14.09397099617995508, 14.95037102751076752, 4.360881834954074776 ) ) ;
#38417=CARTESIAN_POINT ( 'NONE',  ( -14.16722289976679505, 0.3640475087720985159, -4.928467845925709412 ) ) ;
#38421=AXIS2_PLACEMENT_3D ( 'NONE', #30592, #1116, #48055 ) ;
#38429=AXIS2_PLACEMENT_3D ( 'NONE', #19623, #50617, #81108 ) ;
#38431=FACE_OUTER_BOUND ( 'NONE', #36420, .T. ) ;
#38436=EDGE_CURVE ( 'NONE', #21745, #70649, #20249, .T. ) ;
#38437=ORIENTED_EDGE ( 'NONE', *, *, #36889, .F. ) ;
#38438=CARTESIAN_POINT ( 'NONE',  ( -12.07856007377833407, 3.961594683405543780E-16, 8.022367888854752493 ) ) ;
#38444=CARTESIAN_POINT ( 'NONE',  ( 1.915564264621439472, 15.00000000000000000, -14.37291249357988043 ) ) ;
#38447=DIRECTION ( 'NONE',  ( 0.000000000000000000, 0.000000000000000000, 1.000000000000000000 ) ) ;
#38448=CARTESIAN_POINT ( 'NONE',  ( 14.94699059465101776, 15.00000000000000000, -1.259949270174818059 ) ) ;
#38452=CARTESIAN_POINT ( 'NONE',  ( 11.62719953690064933, 14.49999999999999822, -9.476720473301794456 ) ) ;
#38457=B_SPLINE_CURVE_WITH_KNOTS ( 'NONE', 3,
 ( #4129, #43095, #36086, #58586, #43584, #50104 ),
 .UNSPECIFIED., .F., .F.,
 ( 4, 2, 4 ),
 ( 0.0002800170536516692881, 0.0006862224498868429523, 0.001092427846122016617 ),
 .UNSPECIFIED. ) ;
#38465=CARTESIAN_POINT ( 'NONE',  ( -6.767445849361066301, 15.00000000000000000, -13.38662304974505801 ) ) ;
#38468=CARTESIAN_POINT ( 'NONE',  ( -3.193136578977206597, 2.219226321806266888E-16, 14.27383009353652454 ) ) ;
#38477=CARTESIAN_POINT ( 'NONE',  ( -12.26659068614895354, -3.612917831752694653, -7.082119434687038861 ) ) ;
#38481=ORIENTED_EDGE ( 'NONE', *, *, #29842, .T. ) ;
#38487=CARTESIAN_POINT ( 'NONE',  ( 0.000000000000000000, 15.00000000000000000, 0.000000000000000000 ) ) ;
#38498=VECTOR ( 'NONE', #33047, 1000.000000000000000 ) ;
#38499=ADVANCED_FACE ( 'NONE', ( #21003 ), #56997, .T. ) ;
#38502=CARTESIAN_POINT ( 'NONE',  ( -13.59943737456463708, 14.95077488074852390, 5.718514076972763149 ) ) ;
#38507=CARTESIAN_POINT ( 'NONE',  ( 13.34343830728406743, 0.3639313252796093079, -6.852200678592626382 ) ) ;
#38511=CARTESIAN_POINT ( 'NONE',  ( 14.43100913236849614, 4.781026887021415124E-16, 1.412789942453260839 ) ) ;
#38519=CARTESIAN_POINT ( 'NONE',  ( -0.3329122712635644854, 0.000000000000000000, -5.443067521379392204 ) ) ;
#38521=VECTOR ( 'NONE', #67222, 1000.000000000000000 ) ;
#38522=DIRECTION ( 'NONE',  ( 0.000000000000000000, 1.000000000000000000, 0.000000000000000000 ) ) ;
#38526=VERTEX_POINT ( 'NONE', #50506 ) ;
#38529=ADVANCED_FACE ( 'NONE', ( #43006 ), #74564, .T. ) ;
#38537=ADVANCED_FACE ( 'NONE', ( #81986 ), #54464, .T. ) ;
#38540=TOROIDAL_SURFACE ( 'NONE', #16186, 14.49999999999999822, 0.5000000000000000000 ) ;
#38542=CARTESIAN_POINT ( 'NONE',  ( -11.09922568453595382, -41.29303199673624647, -6.408140936763226492 ) ) ;
#38543=ORIENTED_EDGE ( 'NONE', *, *, #82290, .T. ) ;
#38544=TOROIDAL_SURFACE ( 'NONE', #1874, 14.49999999999999822, 0.5000000000000000000 ) ;
#38552=B_SPLINE_CURVE_WITH_KNOTS ( 'NONE', 3,
 ( #27381, #11896, #26392, #86425, #3911, #57387 ),
 .UNSPECIFIED., .F., .F.,
 ( 4, 2, 4 ),
 ( 0.0002800518438628012163, 0.0006862575805706620877, 0.001092463317278523013 ),
 .UNSPECIFIED. ) ;
#38565=LINE ( 'NONE', #78030, #76194 ) ;
#38567=CARTESIAN_POINT ( 'NONE',  ( -9.399392868737892925, 4.026710370808002065E-16, 11.04089732309467919 ) ) ;
#38585=CARTESIAN_POINT ( 'NONE',  ( 7.595945211628325922, 15.00000000000000000, -12.35117874301639240 ) ) ;
#38591=ORIENTED_EDGE ( 'NONE', *, *, #23056, .T. ) ;
#38592=EDGE_LOOP ( 'NONE', ( #33376, #87568, #18017, #24758 ) ) ;
#38603=CARTESIAN_POINT ( 'NONE',  ( -9.422509992056145478, -17.35298132251182324, -5.440088680355541939 ) ) ;
#38608=EDGE_CURVE ( 'NONE', #43096, #39731, #95685, .T. ) ;
#38609=CARTESIAN_POINT ( 'NONE',  ( 10.19513985507833276, 15.00000000000000000, -11.00268709613217055 ) ) ;
#38610=CARTESIAN_POINT ( 'NONE',  ( -0.2078314800230414150, 14.95037105884406792, 14.75174957775970519 ) ) ;
#38617=CARTESIAN_POINT ( 'NONE',  ( 0.000000000000000000, 14.49999999999999822, 0.000000000000000000 ) ) ;
#38633=VERTEX_POINT ( 'NONE', #30947 ) ;
#38634=CIRCLE ( 'NONE', #22724, 14.49999999999999822 ) ;
#38637=EDGE_CURVE ( 'NONE', #95614, #50302, #54435, .T. ) ;
#38646=DIRECTION ( 'NONE',  ( 0.000000000000000000, 0.000000000000000000, -1.000000000000000000 ) ) ;
#38648=CARTESIAN_POINT ( 'NONE',  ( 8.527530157486175710, -11.07440218233254114, -4.923371831947298993 ) ) ;
#38649=ORIENTED_EDGE ( 'NONE', *, *, #77886, .F. ) ;
#38651=ORIENTED_EDGE ( 'NONE', *, *, #41920, .F. ) ;
#38653=ORIENTED_EDGE ( 'NONE', *, *, #97234, .T. ) ;
#38654=CARTESIAN_POINT ( 'NONE',  ( 5.200846386093622264, 0.000000000000000000, 1.639820566680979308 ) ) ;
#38660=CARTESIAN_POINT ( 'NONE',  ( 3.469446951953614189E-15, 11.36803362898265135, 11.25000000000000178 ) ) ;
#38664=CARTESIAN_POINT ( 'NONE',  ( 9.382169495545419124, 15.99863466993042493, 9.382169495545417348 ) ) ;
#38668=ORIENTED_EDGE ( 'NONE', *, *, #93804, .T. ) ;
#38673=EDGE_CURVE ( 'NONE', #18498, #69579, #91217, .T. ) ;
#38674=B_SPLINE_CURVE_WITH_KNOTS ( 'NONE', 3,
 ( #79384, #10890, #94871, #56870, #87373, #18888 ),
 .UNSPECIFIED., .F., .F.,
 ( 4, 2, 4 ),
 ( 3.409110551496121881E-05, 0.0004400426677367870595, 0.0008459942299586128934 ),
 .UNSPECIFIED. ) ;
#38677=AXIS2_PLACEMENT_3D ( 'NONE', #81996, #15004, #74491 ) ;
#38681=EDGE_CURVE ( 'NONE', #48202, #35666, #48115, .T. ) ;
#38682=DIRECTION ( 'NONE',  ( 0.000000000000000000, 0.000000000000000000, -1.000000000000000000 ) ) ;
#38683=CARTESIAN_POINT ( 'NONE',  ( -14.82269085861165792, 0.5000000000000004441, -2.299529454047158250 ) ) ;
#38690=PLANE ( 'NONE',  #94746 ) ;
#38692=DIRECTION ( 'NONE',  ( -0.8526401643540884034, 0.000000000000000000, -0.5224985647159551272 ) ) ;
#38693=ORIENTED_EDGE ( 'NONE', *, *, #67304, .F. ) ;
#38695=CARTESIAN_POINT ( 'NONE',  ( 0.000000000000000000, 14.49999999999999822, 0.000000000000000000 ) ) ;
#38699=CARTESIAN_POINT ( 'NONE',  ( -9.322910753578032228, 14.95077488074853456, 11.43369735623869765 ) ) ;
#38706=CARTESIAN_POINT ( 'NONE',  ( -5.963430220938290560, 6.828790035174475470, -10.32896413005679648 ) ) ;
#38710=CARTESIAN_POINT ( 'NONE',  ( 6.767445849361153343, 0.5000000000000004441, 13.38662304974501360 ) ) ;
#38721=CARTESIAN_POINT ( 'NONE',  ( 12.26659068614894821, 18.88708216824730357, 7.082119434687044190 ) ) ;
#38726=EDGE_CURVE ( 'NONE', #587, #28267, #50331, .T. ) ;
#38737=CARTESIAN_POINT ( 'NONE',  ( -11.42891328973231069, -3.194161244095965395E-15, 9.126250717928300560 ) ) ;
#38745=TOROIDAL_SURFACE ( 'NONE', #94612, 14.49999999999999822, 0.5000000000000000000 ) ;
#38749=CARTESIAN_POINT ( 'NONE',  ( 0.000000000000000000, 15.00000000000000000, 0.000000000000000000 ) ) ;
#38759=ORIENTED_EDGE ( 'NONE', *, *, #82536, .T. ) ;
#38762=EDGE_CURVE ( 'NONE', #31539, #34814, #14595, .T. ) ;
#38773=AXIS2_PLACEMENT_3D ( 'NONE', #38194, #68681, #82191 ) ;
#38775=DIRECTION ( 'NONE',  ( 0.7716245833877106719, 0.000000000000000000, 0.6360782202777751637 ) ) ;
#38777=VERTEX_POINT ( 'NONE', #55433 ) ;
#38779=ORIENTED_EDGE ( 'NONE', *, *, #43120, .T. ) ;
#38783=ORIENTED_EDGE ( 'NONE', *, *, #62519, .F. ) ;
#38794=CARTESIAN_POINT ( 'NONE',  ( -12.34086200392831678, 15.00000000000000000, 7.124999999999885425 ) ) ;
#38803=CARTESIAN_POINT ( 'NONE',  ( -1.114591949025130369, 3.902037737440774503E-16, 14.45709807627963706 ) ) ;
#38810=VECTOR ( 'NONE', #61581, 1000.000000000000000 ) ;
#38816=VECTOR ( 'NONE', #91306, 1000.000000000000000 ) ;
#38822=CARTESIAN_POINT ( 'NONE',  ( 12.54342190210040187, 0.2301501149690343417, 8.116945096741376986 ) ) ;
#38832=CARTESIAN_POINT ( 'NONE',  ( -2.815433093577223378, 0.5000000000000004441, 14.73340885523747978 ) ) ;
#38834=DIRECTION ( 'NONE',  ( 0.000000000000000000, 1.000000000000000000, 0.000000000000000000 ) ) ;
#38842=DIRECTION ( 'NONE',  ( 0.9025852843498560762, 0.000000000000000000, 0.4305110968083047940 ) ) ;
#38845=EDGE_CURVE ( 'NONE', #76622, #73812, #36919, .T. ) ;
#38850=CARTESIAN_POINT ( 'NONE',  ( -13.82671409943298357, -0.03417435944610275333, 3.447387012295131115 ) ) ;
#38851=VERTEX_POINT ( 'NONE', #2461 ) ;
#38855=CARTESIAN_POINT ( 'NONE',  ( 15.81765804549837107, -0.03417435944610275333, 2.383084218346927408 ) ) ;
#38865=CARTESIAN_POINT ( 'NONE',  ( 12.00809552683959325, 14.49999999999999112, 8.989195838243645653 ) ) ;
#38870=CARTESIAN_POINT ( 'NONE',  ( 10.19513985507835763, 14.49999999999999112, -11.00268709613223450 ) ) ;
#38871=CARTESIAN_POINT ( 'NONE',  ( -0.04758788293976230072, 0.000000000000000000, 5.453031268574419776 ) ) ;
#38875=CARTESIAN_POINT ( 'NONE',  ( 5.376821459230018974, 0.2301511342434729712, 13.93958558162640493 ) ) ;
#38887=TOROIDAL_SURFACE ( 'NONE', #584, 14.49999999999999822, 0.5000000000000000000 ) ;
#38892=ADVANCED_FACE ( 'NONE', ( #24950 ), #93922, .T. ) ;
#38893=CIRCLE ( 'NONE', #85273, 14.49999999999999822 ) ;
#38902=ORIENTED_EDGE ( 'NONE', *, *, #67752, .F. ) ;
#38917=CARTESIAN_POINT ( 'NONE',  ( 12.50534872682732690, 4.484280952698287085E-16, -7.339363270777523596 ) ) ;
#38921=VECTOR ( 'NONE', #15253, 1000.000000000000000 ) ;
#38925=ORIENTED_EDGE ( 'NONE', *, *, #96003, .F. ) ;
#38930=ORIENTED_EDGE ( 'NONE', *, *, #77246, .T. ) ;
#38937=DIRECTION ( 'NONE',  ( -0.000000000000000000, 1.000000000000000000, 0.000000000000000000 ) ) ;
#38940=CARTESIAN_POINT ( 'NONE',  ( -6.382347221874242749, 0.5000000000000004441, -13.57444820018235987 ) ) ;
#38943=CARTESIAN_POINT ( 'NONE',  ( 11.62719953690064933, 14.63595249122790598, -9.476720473301801562 ) ) ;
#38947=LINE ( 'NONE', #92425, #77527 ) ;
#38960=LINE ( 'NONE', #69452, #7493 ) ;
#38961=DIRECTION ( 'NONE',  ( -0.04361938736533987893, 0.000000000000000000, 0.9990482215818576872 ) ) ;
#38964=CARTESIAN_POINT ( 'NONE',  ( 14.16423886937410082, -10.48791783175269643, -3.795296366450314096 ) ) ;
#38969=ORIENTED_EDGE ( 'NONE', *, *, #38300, .F. ) ;
#38974=DIRECTION ( 'NONE',  ( 0.000000000000000000, 0.000000000000000000, 1.000000000000000000 ) ) ;
#38980=CARTESIAN_POINT ( 'NONE',  ( 15.67879934938582664, 15.00000000000000000, -3.170591017105818921 ) ) ;
#38990=VERTEX_POINT ( 'NONE', #97384 ) ;
#38999=DIRECTION ( 'NONE',  ( -0.000000000000000000, -1.000000000000000000, -0.000000000000000000 ) ) ;
#39000=CARTESIAN_POINT ( 'NONE',  ( 10.82344394350224803, 0.04922511925147020351, 10.02492699998885328 ) ) ;
#39004=LINE ( 'NONE', #39500, #23922 ) ;
#39011=CARTESIAN_POINT ( 'NONE',  ( 0.000000000000000000, 15.00000000000000000, 0.000000000000000000 ) ) ;
#39015=CARTESIAN_POINT ( 'NONE',  ( -0.7166339456633684657, 15.00000000000000000, 15.98010739087745868 ) ) ;
#39029=DIRECTION ( 'NONE',  ( -0.000000000000000000, -1.000000000000000000, -0.000000000000000000 ) ) ;
#39031=VECTOR ( 'NONE', #74496, 1000.000000000000000 ) ;
#39032=CARTESIAN_POINT ( 'NONE',  ( 2.638427012816835227, 27.46726448433411960, 9.846743663894590881 ) ) ;
#39036=VERTEX_POINT ( 'NONE', #50880 ) ;
#39048=ORIENTED_EDGE ( 'NONE', *, *, #19779, .F. ) ;
#39059=VECTOR ( 'NONE', #82777, 1000.000000000000227 ) ;
#39065=ORIENTED_EDGE ( 'NONE', *, *, #8766, .T. ) ;
#39067=DIRECTION ( 'NONE',  ( -0.000000000000000000, -1.000000000000000000, -0.000000000000000000 ) ) ;
#39068=DIRECTION ( 'NONE',  ( 0.000000000000000000, 1.000000000000000000, 0.000000000000000000 ) ) ;
#39071=DIRECTION ( 'NONE',  ( 0.000000000000000000, 0.000000000000000000, 1.000000000000000000 ) ) ;
#39072=DIRECTION ( 'NONE',  ( 0.5075383629607025382, 0.000000000000000000, -0.8616291604415267091 ) ) ;
#39085=COLOUR_RGB ( '', 0.66274510, 0.83137255, 0.94901961) ;
#39087=AXIS2_PLACEMENT_3D ( 'NONE', #72888, #95911, #12392 ) ;
#39088=EDGE_CURVE ( 'NONE', #16656, #80097, #5876, .T. ) ;
#39094=CARTESIAN_POINT ( 'NONE',  ( 13.03370038005726705, 15.00000000000000000, -9.273621236547697322 ) ) ;
#39100=CARTESIAN_POINT ( 'NONE',  ( -10.88017736071110164, -2.144647989178493308, -2.915334737309917212 ) ) ;
#39106=DIRECTION ( 'NONE',  ( 0.000000000000000000, -1.000000000000000000, 0.000000000000000000 ) ) ;
#39107=B_SPLINE_CURVE_WITH_KNOTS ( 'NONE', 3,
 ( #79317, #78826, #10336, #71816, #33786, #64292 ),
 .UNSPECIFIED., .F., .F.,
 ( 4, 2, 4 ),
 ( 3.409110551496112395E-05, 0.0004400426677367850537, 0.0008459942299586089903 ),
 .UNSPECIFIED. ) ;
#39111=LINE ( 'NONE', #94554, #20116 ) ;
#39116=CARTESIAN_POINT ( 'NONE',  ( 9.402796353261127393, 0.5000000000000004441, -11.68706210897757103 ) ) ;
#39129=CARTESIAN_POINT ( 'NONE',  ( -14.03351048042393856, 15.00000000000000000, -2.474486531753901541 ) ) ;
#39132=DIRECTION ( 'NONE',  ( 0.9969173337331289630, 0.000000000000000000, -0.07845909572783234254 ) ) ;
#39134=ORIENTED_EDGE ( 'NONE', *, *, #82857, .T. ) ;
#39148=CARTESIAN_POINT ( 'NONE',  ( 4.923371831947295441, -10.65773551566587329, -8.527530157486179263 ) ) ;
#39153=VERTEX_POINT ( 'NONE', #54314 ) ;
#39159=DIRECTION ( 'NONE',  ( 0.000000000000000000, 1.000000000000000000, 0.000000000000000000 ) ) ;
#39167=EDGE_LOOP ( 'NONE', ( #47562, #26191, #78851, #6933 ) ) ;
#39176=EDGE_CURVE ( 'NONE', #29785, #87174, #62303, .T. ) ;
#39177=CARTESIAN_POINT ( 'NONE',  ( -9.898881779040587858, 0.000000000000000000, -10.25059215482589714 ) ) ;
#39178=ORIENTED_EDGE ( 'NONE', *, *, #11884, .F. ) ;
#39179=CARTESIAN_POINT ( 'NONE',  ( 4.838527690343618737, 0.5000000000000004441, -14.19819177887726624 ) ) ;
#39191=CARTESIAN_POINT ( 'NONE',  ( 0.000000000000000000, 14.49999999999999822, 0.000000000000000000 ) ) ;
#39203=EDGE_CURVE ( 'NONE', #83367, #77859, #7367, .T. ) ;
#39206=ORIENTED_EDGE ( 'NONE', *, *, #25638, .T. ) ;
#39207=ADVANCED_FACE ( 'NONE', ( #98384 ), #14373, .F. ) ;
#39208=CARTESIAN_POINT ( 'NONE',  ( 0.3093388210927642268, 15.00000000000000000, -14.99680997725065978 ) ) ;
#39212=CARTESIAN_POINT ( 'NONE',  ( 0.000000000000000000, 0.000000000000000000, 0.000000000000000000 ) ) ;
#39214=DIRECTION ( 'NONE',  ( 0.5519369853120676961, 0.000000000000000000, -0.8338858220671618859 ) ) ;
#39216=DIRECTION ( 'NONE',  ( 0.9981347984218662539, 0.000000000000000000, 0.06104853953487057033 ) ) ;
#39220=CARTESIAN_POINT ( 'NONE',  ( 7.082119434687054849, 28.47041550158063572, 12.26659068614894288 ) ) ;
#39226=VECTOR ( 'NONE', #76511, 1000.000000000000000 ) ;
#39231=VERTEX_POINT ( 'NONE', #44841 ) ;
#39241=VERTEX_POINT ( 'NONE', #75347 ) ;
#39250=CARTESIAN_POINT ( 'NONE',  ( -7.684764310694718326, 14.49999999999999112, -12.88194075009952222 ) ) ;
#39252=EDGE_CURVE ( 'NONE', #92402, #41037, #1503, .T. ) ;
#39256=ORIENTED_EDGE ( 'NONE', *, *, #55005, .F. ) ;
#39259=AXIS2_PLACEMENT_3D ( 'NONE', #31932, #22124, #52603 ) ;
#39270=CARTESIAN_POINT ( 'NONE',  ( -11.35178980618986877, 14.49999999999999112, 9.804941009311868072 ) ) ;
#39275=CARTESIAN_POINT ( 'NONE',  ( -4.838527690343713772, 15.00000000000000000, 14.19819177887723605 ) ) ;
#39291=EDGE_LOOP ( 'NONE', ( #42748, #46753, #8723, #36043 ) ) ;
#39294=DIRECTION ( 'NONE',  ( 0.000000000000000000, 0.000000000000000000, -1.000000000000000000 ) ) ;
#39300=AXIS2_PLACEMENT_3D ( 'NONE', #34821, #64326, #2888 ) ;
#39301=EDGE_LOOP ( 'NONE', ( #66801, #91521, #14148, #8970 ) ) ;
#39302=DIRECTION ( 'NONE',  ( -0.000000000000000000, -1.000000000000000000, -0.000000000000000000 ) ) ;
#39321=ADVANCED_FACE ( 'NONE', ( #46336 ), #380, .F. ) ;
#39329=CARTESIAN_POINT ( 'NONE',  ( -5.815502996285044190, 14.76930270348881002, 13.76292046016118675 ) ) ;
#39336=CARTESIAN_POINT ( 'NONE',  ( -5.806645064956352797, 3.422013106907373370E-16, -13.42464971017003528 ) ) ;
#39337=AXIS2_PLACEMENT_3D ( 'NONE', #47395, #2429, #31893 ) ;
#39344=VERTEX_POINT ( 'NONE', #76822 ) ;
#39355=ORIENTED_EDGE ( 'NONE', *, *, #53491, .F. ) ;
#39356=CARTESIAN_POINT ( 'NONE',  ( -2.815433093577222490, 14.63595249122788999, 14.73340885523749044 ) ) ;
#39357=CARTESIAN_POINT ( 'NONE',  ( -11.36220558718850882, 3.877685541201178108E-16, -9.008345252845398221 ) ) ;
#39363=DIRECTION ( 'NONE',  ( -0.9999619230641711987, 0.000000000000000000, -0.008726535498381204903 ) ) ;
#39368=CARTESIAN_POINT ( 'NONE',  ( -2.120353041430432128, 15.00000000000000000, -14.34413130794946234 ) ) ;
#39371=EDGE_CURVE ( 'NONE', #98693, #43481, #59902, .T. ) ;
#39376=CARTESIAN_POINT ( 'NONE',  ( 0.3093388210927633941, 0.5000000000000004441, 14.99680997725065978 ) ) ;
#39377=AXIS2_PLACEMENT_3D ( 'NONE', #32135, #78146, #70659 ) ;
#39386=ORIENTED_EDGE ( 'NONE', *, *, #60523, .T. ) ;
#39394=AXIS2_PLACEMENT_3D ( 'NONE', #40422, #62902, #79388 ) ;
#39405=ORIENTED_EDGE ( 'NONE', *, *, #56154, .T. ) ;
#39414=ADVANCED_FACE ( 'NONE', ( #40809 ), #48291, .T. ) ;
#39422=CARTESIAN_POINT ( 'NONE',  ( 3.420591144908469161, 0.3639311400139680908, 14.60477854057961267 ) ) ;
#39427=CARTESIAN_POINT ( 'NONE',  ( 10.14667048435145169, 15.00000000000000000, -10.35833375027041292 ) ) ;
#39434=FACE_OUTER_BOUND ( 'NONE', #94925, .T. ) ;
#39436=VERTEX_POINT ( 'NONE', #17327 ) ;
#39438=CARTESIAN_POINT ( 'NONE',  ( 11.25000000000000178, 2.618033628982651351, -2.373340393710807175E-15 ) ) ;
#39445=CARTESIAN_POINT ( 'NONE',  ( -13.96552416078070102, 0.04962884865031235576, 4.756200848674986048 ) ) ;
#39451=CARTESIAN_POINT ( 'NONE',  ( -3.843542995449462651, 14.76984992749125780, -14.43777707752884787 ) ) ;
#39454=AXIS2_PLACEMENT_3D ( 'NONE', #79472, #10971, #41492 ) ;
#39455=ORIENTED_EDGE ( 'NONE', *, *, #76596, .T. ) ;
#39457=CARTESIAN_POINT ( 'NONE',  ( 0.000000000000000000, 14.49999999999999822, 0.000000000000000000 ) ) ;
#39460=VECTOR ( 'NONE', #75079, 1000.000000000000000 ) ;
#39462=CARTESIAN_POINT ( 'NONE',  ( 10.36894250292378850, -5.071251165086031243, -10.36894250292379027 ) ) ;
#39470=DIRECTION ( 'NONE',  ( 0.000000000000000000, 0.000000000000000000, 1.000000000000000000 ) ) ;
#39479=CARTESIAN_POINT ( 'NONE',  ( -14.69266224296339729, 0.04962895675139352564, -1.335284760096340229 ) ) ;
#39488=ADVANCED_FACE ( 'NONE', ( #78800 ), #22582, .T. ) ;
#39493=VECTOR ( 'NONE', #53926, 1000.000000000000114 ) ;
#39496=CARTESIAN_POINT ( 'NONE',  ( 5.991992585808537441, 4.355491999677157623E-16, 13.20401548210299048 ) ) ;
#39499=CARTESIAN_POINT ( 'NONE',  ( 3.843478602184446036, 0.2306972965111899754, 14.43834224996325410 ) ) ;
#39500=CARTESIAN_POINT ( 'NONE',  ( -2.962741594152892510, -0.03417435944610275333, -13.93860331045676837 ) ) ;
#39518=CARTESIAN_POINT ( 'NONE',  ( -9.705452947461466806, 12.49999999999999289, -5.689172442861226031 ) ) ;
#39524=CARTESIAN_POINT ( 'NONE',  ( 0.1034006766821432000, 15.00000000000000000, 14.49963131600458688 ) ) ;
#39526=CARTESIAN_POINT ( 'NONE',  ( 9.065164099344512394, 14.49999999999999112, 11.95084933600776722 ) ) ;
#39527=CARTESIAN_POINT ( 'NONE',  ( 7.208316651077762316, 29.13393115100079100, -7.208316651077764980 ) ) ;
#39538=TOROIDAL_SURFACE ( 'NONE', #47512, 14.49999999999999822, 0.5000000000000000000 ) ;
#39539=CIRCLE ( 'NONE', #58638, 11.25000000000000178 ) ;
#39540=ADVANCED_FACE ( 'NONE', ( #3798 ), #78450, .T. ) ;
#39549=ORIENTED_EDGE ( 'NONE', *, *, #43152, .T. ) ;
#39559=VERTEX_POINT ( 'NONE', #34254 ) ;
#39560=EDGE_LOOP ( 'NONE', ( #74330, #22816, #62419 ) ) ;
#39561=LINE ( 'NONE', #71538, #47432 ) ;
#39573=ORIENTED_EDGE ( 'NONE', *, *, #55589, .F. ) ;
#39579=EDGE_CURVE ( 'NONE', #88333, #243, #87276, .T. ) ;
#39580=DIRECTION ( 'NONE',  ( 0.000000000000000000, 0.000000000000000000, 1.000000000000000000 ) ) ;
#39581=CIRCLE ( 'NONE', #77883, 15.00000000000000000 ) ;
#39584=ORIENTED_EDGE ( 'NONE', *, *, #63126, .T. ) ;
#39592=LINE ( 'NONE', #47571, #80554 ) ;
#39593=TOROIDAL_SURFACE ( 'NONE', #9250, 14.49999999999999822, 0.5000000000000000000 ) ;
#39597=CARTESIAN_POINT ( 'NONE',  ( 7.964842623401181321, 4.938685344154837509, 7.964842623401174215 ) ) ;
#39601=CARTESIAN_POINT ( 'NONE',  ( -13.34343830728408697, 14.49999999999999822, 6.852200678592504701 ) ) ;
#39608=CYLINDRICAL_SURFACE ( 'NONE', #44087, 15.00000000000000000 ) ;
#39612=CARTESIAN_POINT ( 'NONE',  ( 9.323033696085012423, 0.04962895454604582951, -11.43408728005512920 ) ) ;
#39625=EDGE_CURVE ( 'NONE', #81238, #86936, #77801, .T. ) ;
#39626=CARTESIAN_POINT ( 'NONE',  ( -13.55255535720589322, -0.03417435944610275333, -4.403492169843143067 ) ) ;
#39628=ORIENTED_EDGE ( 'NONE', *, *, #50484, .F. ) ;
#39629=ORIENTED_EDGE ( 'NONE', *, *, #26216, .T. ) ;
#39641=DIRECTION ( 'NONE',  ( -0.000000000000000000, -1.000000000000000000, -0.000000000000000000 ) ) ;
#39643=CARTESIAN_POINT ( 'NONE',  ( -7.208316651077756099, -13.36606884899921077, 7.208316651077766757 ) ) ;
#39644=ORIENTED_EDGE ( 'NONE', *, *, #67208, .F. ) ;
#39649=VERTEX_POINT ( 'NONE', #43253 ) ;
#39663=ORIENTED_EDGE ( 'NONE', *, *, #6279, .F. ) ;
#39667=CARTESIAN_POINT ( 'NONE',  ( 0.000000000000000000, 15.00000000000000000, 0.000000000000000000 ) ) ;
#39680=EDGE_LOOP ( 'NONE', ( #54516, #32006, #58031, #78017, #90534, #95708 ) ) ;
#39686=EDGE_CURVE ( 'NONE', #85753, #53420, #264, .T. ) ;
#39688=CARTESIAN_POINT ( 'NONE',  ( 14.47650479471825236, 0.3639311865616660091, -3.928206833722031721 ) ) ;
#39694=CARTESIAN_POINT ( 'NONE',  ( -11.62719953690052144, 0.3640475087720991820, -9.476720473301961434 ) ) ;
#39699=EDGE_CURVE ( 'NONE', #2288, #54272, #65249, .T. ) ;
#39700=CARTESIAN_POINT ( 'NONE',  ( -11.92686044187656513, 7.662123368507814725, 3.903127820947815962E-15 ) ) ;
#39701=ORIENTED_EDGE ( 'NONE', *, *, #57799, .F. ) ;
#39706=CARTESIAN_POINT ( 'NONE',  ( 14.11917416961168747, 14.76930270348881002, -4.887430353538946726 ) ) ;
#39707=DIRECTION ( 'NONE',  ( 0.000000000000000000, 0.000000000000000000, -1.000000000000000000 ) ) ;
#39708=CARTESIAN_POINT ( 'NONE',  ( 8.439016546559821919, 3.791394052158136007E-16, 11.79122553964979048 ) ) ;
#39712=CARTESIAN_POINT ( 'NONE',  ( -10.36894250292379205, 31.17874883491396432, -10.36894250292378672 ) ) ;
#39716=CARTESIAN_POINT ( 'NONE',  ( -0.3998276802501956606, -0.03417435944610275333, -15.99117050944549234 ) ) ;
#39721=EDGE_LOOP ( 'NONE', ( #24726, #11113, #94116, #16143, #86360, #56256 ) ) ;
#39731=VERTEX_POINT ( 'NONE', #27257 ) ;
#39734=CIRCLE ( 'NONE', #52488, 15.00000000000000000 ) ;
#39744=CIRCLE ( 'NONE', #50930, 15.00000000000000000 ) ;
#39746=EDGE_LOOP ( 'NONE', ( #62115, #67175, #49445, #17381 ) ) ;
#39754=CARTESIAN_POINT ( 'NONE',  ( 5.845017550302928022, -0.03417435944610275333, 14.89003580495037582 ) ) ;
#39756=DIRECTION ( 'NONE',  ( 0.000000000000000000, 0.000000000000000000, 1.000000000000000000 ) ) ;
#39769=CARTESIAN_POINT ( 'NONE',  ( 14.49120296996857249, 0.04922511925147129985, 2.766068805437629674 ) ) ;
#39772=EDGE_CURVE ( 'NONE', #86489, #44015, #4779, .T. ) ;
#39774=CARTESIAN_POINT ( 'NONE',  ( 9.382169495545415572, -2.751365330069575510, -9.382169495545422677 ) ) ;
#39775=EDGE_CURVE ( 'NONE', #22949, #77971, #14663, .T. ) ;
#39776=VERTEX_POINT ( 'NONE', #59236 ) ;
#39781=AXIS2_PLACEMENT_3D ( 'NONE', #32696, #2238, #10216 ) ;
#39783=LINE ( 'NONE', #55258, #32287 ) ;
#39784=CARTESIAN_POINT ( 'NONE',  ( -12.83294900548056994, 14.49999999999999112, -7.766300266068596692 ) ) ;
#39790=CARTESIAN_POINT ( 'NONE',  ( 0.000000000000000000, 15.00000000000000000, 0.000000000000000000 ) ) ;
#39791=DIRECTION ( 'NONE',  ( 0.000000000000000000, 0.000000000000000000, 1.000000000000000000 ) ) ;
#39795=AXIS2_PLACEMENT_3D ( 'NONE', #5203, #19209, #26701 ) ;
#39804=CARTESIAN_POINT ( 'NONE',  ( 12.34597252984332272, 0.04962896562384134375, 8.076773567935909171 ) ) ;
#39821=DIRECTION ( 'NONE',  ( 0.9914448613738104932, 0.000000000000000000, -0.1305261922200514901 ) ) ;
#39826=FACE_OUTER_BOUND ( 'NONE', #57052, .T. ) ;
#39860=CARTESIAN_POINT ( 'NONE',  ( -2.930023131210801157, 0.000000000000000000, 4.599215049682140233 ) ) ;
#39869=ORIENTED_EDGE ( 'NONE', *, *, #60444, .F. ) ;
#39872=ORIENTED_EDGE ( 'NONE', *, *, #94394, .T. ) ;
#39875=ORIENTED_EDGE ( 'NONE', *, *, #44189, .F. ) ;
#39879=LINE ( 'NONE', #9881, #91511 ) ;
#39885=FACE_OUTER_BOUND ( 'NONE', #31002, .T. ) ;
#39889=CIRCLE ( 'NONE', #68654, 15.00000000000000000 ) ;
#39894=CARTESIAN_POINT ( 'NONE',  ( -13.95749458852084146, 0.2306972965111889207, 5.331641351772924864 ) ) ;
#39895=CARTESIAN_POINT ( 'NONE',  ( 6.382347221874381304, 14.49999999999999112, 13.57444820018236520 ) ) ;
#39899=DIRECTION ( 'NONE',  ( 0.000000000000000000, 0.000000000000000000, 1.000000000000000000 ) ) ;
#39903=ORIENTED_EDGE ( 'NONE', *, *, #9513, .T. ) ;
#39904=CARTESIAN_POINT ( 'NONE',  ( 0.000000000000000000, 0.5000000000000004441, 0.000000000000000000 ) ) ;
#39906=EDGE_CURVE ( 'NONE', #89546, #71139, #49107, .T. ) ;
#39914=FACE_OUTER_BOUND ( 'NONE', #70242, .T. ) ;
#39915=DIRECTION ( 'NONE',  ( -0.9537169507482258224, 0.000000000000000000, -0.3007057995042767273 ) ) ;
#39918=FACE_OUTER_BOUND ( 'NONE', #42936, .T. ) ;
#39920=ORIENTED_EDGE ( 'NONE', *, *, #88957, .T. ) ;
#39922=CARTESIAN_POINT ( 'NONE',  ( -0.9082943533638192513, 4.617951328659527895E-16, 14.47152380945584582 ) ) ;
#39934=CARTESIAN_POINT ( 'NONE',  ( 13.48255862861920562, 15.00000000000000000, 5.335786055104250636 ) ) ;
#39942=CARTESIAN_POINT ( 'NONE',  ( -14.16423886937410437, -3.404584498419356731, -3.795296366450299885 ) ) ;
#39945=ORIENTED_EDGE ( 'NONE', *, *, #31738, .T. ) ;
#39947=CARTESIAN_POINT ( 'NONE',  ( -12.83294900548055573, 14.63606878838274206, -7.766300266068574487 ) ) ;
#39948=CARTESIAN_POINT ( 'NONE',  ( -0.7117905103455194338, 0.000000000000000000, 5.406585696355428183 ) ) ;
#39949=LINE ( 'NONE', #24468, #15353 ) ;
#39952=CARTESIAN_POINT ( 'NONE',  ( 14.35840480524197282, 15.00000000000000000, 4.340070442838948495 ) ) ;
#39956=DIRECTION ( 'NONE',  ( 0.9890158633619168249, 0.000000000000000000, 0.1478094111296113511 ) ) ;
#39959=DIRECTION ( 'NONE',  ( 0.000000000000000000, 0.000000000000000000, 1.000000000000000000 ) ) ;
#39965=CARTESIAN_POINT ( 'NONE',  ( 14.40939250469964961, 3.793246902777681429E-16, 1.618458416365853747 ) ) ;
#39967=ORIENTED_EDGE ( 'NONE', *, *, #22255, .F. ) ;
#39971=CARTESIAN_POINT ( 'NONE',  ( 12.60874940350942985, 3.897725180921639224E-16, 7.160268045227119238 ) ) ;
#39982=CARTESIAN_POINT ( 'NONE',  ( 3.836325488036083087, 0.5000000000000004441, 14.50112432709425114 ) ) ;
#39990=VERTEX_POINT ( 'NONE', #68248 ) ;
#39994=ORIENTED_EDGE ( 'NONE', *, *, #15254, .F. ) ;
#40001=CARTESIAN_POINT ( 'NONE',  ( -9.997910040112669705, 15.00000000000000000, 10.50199004140708325 ) ) ;
#40008=EDGE_CURVE ( 'NONE', #8159, #95321, #90230, .T. ) ;
#40010=CARTESIAN_POINT ( 'NONE',  ( -12.81628187352647252, -40.66803199673623936, 3.434112377981066722 ) ) ;
#40025=VECTOR ( 'NONE', #18442, 1000.000000000000000 ) ;
#40027=ORIENTED_EDGE ( 'NONE', *, *, #7823, .T. ) ;
#40029=AXIS2_PLACEMENT_3D ( 'NONE', #8496, #38999, #69986 ) ;
#40031=CARTESIAN_POINT ( 'NONE',  ( 0.000000000000000000, 0.5000000000000004441, 0.000000000000000000 ) ) ;
#40034=AXIS2_PLACEMENT_3D ( 'NONE', #42227, #29173, #58180 ) ;
#40035=EDGE_CURVE ( 'NONE', #9509, #75439, #52636, .T. ) ;
#40048=DIRECTION ( 'NONE',  ( -0.000000000000000000, -1.000000000000000000, -0.000000000000000000 ) ) ;
#40049=LINE ( 'NONE', #2077, #94477 ) ;
#40052=ORIENTED_EDGE ( 'NONE', *, *, #92212, .T. ) ;
#40057=CARTESIAN_POINT ( 'NONE',  ( 7.684764310694891520, 14.49999999999999112, -12.88194075009941564 ) ) ;
#40061=CIRCLE ( 'NONE', #17661, 14.49999999999999822 ) ;
#40063=VERTEX_POINT ( 'NONE', #45731 ) ;
#40068=EDGE_CURVE ( 'NONE', #85555, #59552, #82009, .T. ) ;
#40076=CARTESIAN_POINT ( 'NONE',  ( 7.964842623401177768, 1.188685344154840395, -7.964842623401181321 ) ) ;
#40078=CARTESIAN_POINT ( 'NONE',  ( 4.856044144387705153, 15.00000000000000888, -13.79699902221158858 ) ) ;
#40081=FACE_OUTER_BOUND ( 'NONE', #81467, .T. ) ;
#40083=PLANE ( 'NONE',  #20886 ) ;
#40088=ADVANCED_FACE ( 'NONE', ( #71190 ), #33167, .F. ) ;
#40109=EDGE_LOOP ( 'NONE', ( #88204, #55291, #54929, #24946 ) ) ;
#40122=CARTESIAN_POINT ( 'NONE',  ( -8.839000071697160621, 14.95037109469996395, 11.81225584161635211 ) ) ;
#40125=CARTESIAN_POINT ( 'NONE',  ( -9.846743663894596210, -9.199402182332550026, -2.638427012816824124 ) ) ;
#40127=EDGE_LOOP ( 'NONE', ( #11691, #79511, #19012, #66138, #14959, #94767 ) ) ;
#40128=PLANE ( 'NONE',  #85838 ) ;
#40129=CARTESIAN_POINT ( 'NONE',  ( 1.983216688680936812, -0.03417435944610275333, -14.11131997956737649 ) ) ;
#40130=ORIENTED_EDGE ( 'NONE', *, *, #80819, .F. ) ;
#40137=DIRECTION ( 'NONE',  ( 0.000000000000000000, 1.000000000000000000, 0.000000000000000000 ) ) ;
#40139=TOROIDAL_SURFACE ( 'NONE', #19359, 14.49999999999999822, 0.5000000000000000000 ) ;
#40143=ORIENTED_EDGE ( 'NONE', *, *, #88343, .T. ) ;
#40152=CARTESIAN_POINT ( 'NONE',  ( 1.354709868695545216, 14.49999999999999112, 14.93870011653158336 ) ) ;
#40156=ORIENTED_EDGE ( 'NONE', *, *, #82857, .F. ) ;
#40159=CARTESIAN_POINT ( 'NONE',  ( -11.48952521350012113, 4.018634162980579609E-16, -8.845383562533903898 ) ) ;
#40161=AXIS2_PLACEMENT_3D ( 'NONE', #1011, #77969, #84498 ) ;
#40177=ORIENTED_EDGE ( 'NONE', *, *, #37160, .T. ) ;
#40183=CARTESIAN_POINT ( 'NONE',  ( -4.880290883660339141, 0.000000000000000000, -2.433223276543861502 ) ) ;
#40186=CARTESIAN_POINT ( 'NONE',  ( -5.991992585808713301, 15.00000000000000000, 13.20401548210291054 ) ) ;
#40188=CARTESIAN_POINT ( 'NONE',  ( -10.88017736071109987, -36.72798132251182324, 2.915334737309934532 ) ) ;
#40208=DIRECTION ( 'NONE',  ( -0.000000000000000000, -1.000000000000000000, -0.000000000000000000 ) ) ;
#40227=ORIENTED_EDGE ( 'NONE', *, *, #56131, .T. ) ;
#40228=AXIS2_PLACEMENT_3D ( 'NONE', #84324, #32272, #31783 ) ;
#40229=ORIENTED_EDGE ( 'NONE', *, *, #59300, .T. ) ;
#40249=ORIENTED_EDGE ( 'NONE', *, *, #68460, .F. ) ;
#40251=CIRCLE ( 'NONE', #11473, 14.49999999999999822 ) ;
#40258=LINE ( 'NONE', #18739, #74532 ) ;
#40259=VERTEX_POINT ( 'NONE', #47185 ) ;
#40260=EDGE_CURVE ( 'NONE', #76878, #1436, #60483, .T. ) ;
#40262=CARTESIAN_POINT ( 'NONE',  ( -9.382169495545422677, -11.50136533006958217, -9.382169495545417348 ) ) ;
#40263=ORIENTED_EDGE ( 'NONE', *, *, #48530, .F. ) ;
#40265=ORIENTED_EDGE ( 'NONE', *, *, #92002, .F. ) ;
#40269=DIRECTION ( 'NONE',  ( -0.7716245833877234395, 0.000000000000000000, 0.6360782202777597316 ) ) ;
#40272=B_SPLINE_CURVE_WITH_KNOTS ( 'NONE', 3,
 ( #5581, #91024, #89059, #7053, #20574, #81547 ),
 .UNSPECIFIED., .F., .F.,
 ( 4, 2, 4 ),
 ( 0.0002800421825936756258, 0.0006862478247299506375, 0.001092453466866225758 ),
 .UNSPECIFIED. ) ;
#40277=CYLINDRICAL_SURFACE ( 'NONE', #61101, 15.00000000000000000 ) ;
#40281=CARTESIAN_POINT ( 'NONE',  ( 11.61621867929611973, 15.00000000000000000, -10.99731149103385874 ) ) ;
#40304=AXIS2_PLACEMENT_3D ( 'NONE', #68091, #27609, #66096 ) ;
#40317=DIRECTION ( 'NONE',  ( 0.9588197348681964938, 0.000000000000000000, -0.2840153447039108214 ) ) ;
#40322=CIRCLE ( 'NONE', #33861, 15.00000000000000000 ) ;
#40338=CARTESIAN_POINT ( 'NONE',  ( 0.000000000000000000, 0.5000000000000004441, 0.000000000000000000 ) ) ;
#40339=FACE_OUTER_BOUND ( 'NONE', #39301, .T. ) ;
#40354=AXIS2_PLACEMENT_3D ( 'NONE', #87361, #41401, #71867 ) ;
#40360=CARTESIAN_POINT ( 'NONE',  ( -14.43100913236846061, 15.00000000000000000, -1.412789942453363423 ) ) ;
#40371=ORIENTED_EDGE ( 'NONE', *, *, #13791, .F. ) ;
#40374=EDGE_LOOP ( 'NONE', ( #9493, #92712, #63225, #59372 ) ) ;
#40381=CARTESIAN_POINT ( 'NONE',  ( 3.115783986955557694, 15.00000000000000000, -14.16128137375397955 ) ) ;
#40386=AXIS2_PLACEMENT_3D ( 'NONE', #35721, #41282, #87241 ) ;
#40391=ORIENTED_EDGE ( 'NONE', *, *, #33254, .T. ) ;
#40394=CARTESIAN_POINT ( 'NONE',  ( -14.49440716394874151, 15.00000000000000000, 0.4026921475165272657 ) ) ;
#40395=AXIS2_PLACEMENT_3D ( 'NONE', #13759, #43261, #82745 ) ;
#40404=DIRECTION ( 'NONE',  ( 0.000000000000000000, 1.000000000000000000, 0.000000000000000000 ) ) ;
#40408=ORIENTED_EDGE ( 'NONE', *, *, #27082, .T. ) ;
#40410=PLANE ( 'NONE',  #35648 ) ;
#40416=DIRECTION ( 'NONE',  ( 8.881784197001252323E-16, 0.000000000000000000, 1.000000000000000000 ) ) ;
#40417=DIRECTION ( 'NONE',  ( -0.000000000000000000, 1.000000000000000000, 0.000000000000000000 ) ) ;
#40419=EDGE_CURVE ( 'NONE', #58682, #91405, #57954, .T. ) ;
#40422=CARTESIAN_POINT ( 'NONE',  ( 0.000000000000000000, 14.49999999999999822, 0.000000000000000000 ) ) ;
#40424=VERTEX_POINT ( 'NONE', #87648 ) ;
#40427=CARTESIAN_POINT ( 'NONE',  ( -1.847237859018534323, 14.95037103927854538, -14.63711110085123757 ) ) ;
#40437=CARTESIAN_POINT ( 'NONE',  ( 12.60589901313228189, 14.49999999999999112, -8.129656208642064286 ) ) ;
#40438=CARTESIAN_POINT ( 'NONE',  ( -3.420591144908647241, 0.5000000000000004441, 14.60477854057953451 ) ) ;
#40441=DIRECTION ( 'NONE',  ( 0.000000000000000000, 0.000000000000000000, 1.000000000000000000 ) ) ;
#40444=CARTESIAN_POINT ( 'NONE',  ( 13.75801628063878645, 15.00000000000000000, 4.578972376164554881 ) ) ;
#40445=CARTESIAN_POINT ( 'NONE',  ( -12.26659068614894110, -2.779584498419355842, 7.082119434687058401 ) ) ;
#40448=ADVANCED_FACE ( 'NONE', ( #80653 ), #80370, .T. ) ;
#40449=VERTEX_POINT ( 'NONE', #72636 ) ;
#40451=CARTESIAN_POINT ( 'NONE',  ( -12.79413655343686784, 14.76984915707685531, -7.715718893783058974 ) ) ;
#40456=EDGE_CURVE ( 'NONE', #53389, #33104, #43135, .T. ) ;
#40461=CARTESIAN_POINT ( 'NONE',  ( 14.26295192185810201, 0.04922511925148844586, 3.770186020345128952 ) ) ;
#40481=CARTESIAN_POINT ( 'NONE',  ( -5.806616290881239095, 15.00000000000000533, -13.42355087257370272 ) ) ;
#40492=ORIENTED_EDGE ( 'NONE', *, *, #37056, .T. ) ;
#40495=EDGE_CURVE ( 'NONE', #79187, #40528, #56398, .T. ) ;
#40497=CARTESIAN_POINT ( 'NONE',  ( 3.840373378095567336, 13.17686044187654559, -11.29165764256138260 ) ) ;
#40499=VERTEX_POINT ( 'NONE', #65632 ) ;
#40513=CARTESIAN_POINT ( 'NONE',  ( 4.923371831947301658, 27.67559781766745886, 8.527530157486175710 ) ) ;
#40514=VERTEX_POINT ( 'NONE', #66636 ) ;
#40515=CARTESIAN_POINT ( 'NONE',  ( 5.795997163830165277, -0.03417435944610275333, -13.01802277140705932 ) ) ;
#40524=VERTEX_POINT ( 'NONE', #64635 ) ;
#40527=TOROIDAL_SURFACE ( 'NONE', #72401, 14.49999999999999822, 0.5000000000000000000 ) ;
#40528=VERTEX_POINT ( 'NONE', #4169 ) ;
#40530=CARTESIAN_POINT ( 'NONE',  ( 10.69820648722788015, 1.823139558123380688, 5.272416709312279792 ) ) ;
#40533=CARTESIAN_POINT ( 'NONE',  ( -9.997910040112461871, 4.266261872180168263E-16, -10.50199004140731773 ) ) ;
#40539=ORIENTED_EDGE ( 'NONE', *, *, #60292, .F. ) ;
#40543=VERTEX_POINT ( 'NONE', #50646 ) ;
#40550=DIRECTION ( 'NONE',  ( 0.000000000000000000, 1.000000000000000000, 0.000000000000000000 ) ) ;
#40551=ORIENTED_EDGE ( 'NONE', *, *, #1167, .F. ) ;
#40561=EDGE_CURVE ( 'NONE', #94977, #77859, #23550, .T. ) ;
#40563=B_SPLINE_CURVE_WITH_KNOTS ( 'NONE', 3,
 ( #81867, #27390, #80896, #58368, #34391, #49896 ),
 .UNSPECIFIED., .F., .F.,
 ( 4, 2, 4 ),
 ( 3.409110551494655498E-05, 0.0004400426677367912337, 0.0008459942299586359869 ),
 .UNSPECIFIED. ) ;
#40571=EDGE_CURVE ( 'NONE', #51581, #78512, #5151, .T. ) ;
#40576=CARTESIAN_POINT ( 'NONE',  ( -5.440088680355558814, 2.230352010821508468, -9.422509992056136596 ) ) ;
#40582=LINE ( 'NONE', #72046, #67203 ) ;
#40586=CARTESIAN_POINT ( 'NONE',  ( 8.731067818237031375, 12.81330936912750929, -8.731067818237036704 ) ) ;
#40593=ORIENTED_EDGE ( 'NONE', *, *, #76902, .T. ) ;
#40597=CARTESIAN_POINT ( 'NONE',  ( -12.50534872682737664, 4.247830340245585198E-16, 7.339363270777436554 ) ) ;
#40603=CARTESIAN_POINT ( 'NONE',  ( 13.30156849913886496, 14.76930270348881002, -6.804875469488061768 ) ) ;
#40605=EDGE_CURVE ( 'NONE', #21360, #45156, #65136, .T. ) ;
#40607=FACE_OUTER_BOUND ( 'NONE', #71151, .T. ) ;
#40608=ORIENTED_EDGE ( 'NONE', *, *, #33056, .T. ) ;
#40609=EDGE_LOOP ( 'NONE', ( #47739, #10701, #71314, #90062, #1073, #91666 ) ) ;
#40619=CARTESIAN_POINT ( 'NONE',  ( 12.60589901313221439, 0.5000000000000004441, -8.129656208642048298 ) ) ;
#40622=CARTESIAN_POINT ( 'NONE',  ( 7.208316651077764980, -7.116068848999210772, 7.208316651077762316 ) ) ;
#40625=CARTESIAN_POINT ( 'NONE',  ( -2.962741594153171842, 15.00000000000000000, 13.93860331045670975 ) ) ;
#40627=DIRECTION ( 'NONE',  ( 0.2503800040544389427, 0.000000000000000000, 0.9681476403781082984 ) ) ;
#40633=CARTESIAN_POINT ( 'NONE',  ( -13.61464873478159454, 14.63595249122789177, -6.296136897218026718 ) ) ;
#40635=LINE ( 'NONE', #87101, #73339 ) ;
#40637=ORIENTED_EDGE ( 'NONE', *, *, #25771, .T. ) ;
#40641=ORIENTED_EDGE ( 'NONE', *, *, #32120, .F. ) ;
#40648=LINE ( 'NONE', #64103, #45650 ) ;
#40661=CARTESIAN_POINT ( 'NONE',  ( -2.815433093577223378, 15.00000000000000000, 14.73340885523747978 ) ) ;
#40666=CARTESIAN_POINT ( 'NONE',  ( -7.684764310694718326, 14.49999999999999112, -12.88194075009952222 ) ) ;
#40668=ADVANCED_FACE ( 'NONE', ( #83492 ), #50035, .T. ) ;
#40674=EDGE_LOOP ( 'NONE', ( #42479, #58820, #25025, #34596, #28286, #40265 ) ) ;
#40681=EDGE_CURVE ( 'NONE', #11914, #97132, #8474, .T. ) ;
#40683=CARTESIAN_POINT ( 'NONE',  ( 0.000000000000000000, 0.5000000000000004441, 0.000000000000000000 ) ) ;
#40685=CARTESIAN_POINT ( 'NONE',  ( 2.915334737309921209, -33.39464798917849464, -10.88017736071110164 ) ) ;
#40688=DIRECTION ( 'NONE',  ( 0.000000000000000000, 1.000000000000000000, -0.000000000000000000 ) ) ;
#40696=ORIENTED_EDGE ( 'NONE', *, *, #49054, .F. ) ;
#40702=CARTESIAN_POINT ( 'NONE',  ( -13.40508947812791796, 15.00000000000000000, -5.527528931052510863 ) ) ;
#40713=DIRECTION ( 'NONE',  ( -0.8038568606172203923, 0.000000000000000000, 0.5948227867513371514 ) ) ;
#40715=VECTOR ( 'NONE', #19907, 1000.000000000000000 ) ;
#40720=VERTEX_POINT ( 'NONE', #92454 ) ;
#40733=CARTESIAN_POINT ( 'NONE',  ( 10.84451454130507209, 4.631809541732465460E-16, -9.625305416630832056 ) ) ;
#40734=DIRECTION ( 'NONE',  ( -4.174438572590589223E-14, 0.000000000000000000, 1.000000000000000000 ) ) ;
#40738=ORIENTED_EDGE ( 'NONE', *, *, #67752, .T. ) ;
#40742=ORIENTED_EDGE ( 'NONE', *, *, #63487, .F. ) ;
#40751=CARTESIAN_POINT ( 'NONE',  ( -12.81628187352647608, -10.87636533006957507, 3.903127820947815962E-15 ) ) ;
#40756=ORIENTED_EDGE ( 'NONE', *, *, #88215, .T. ) ;
#40766=DIRECTION ( 'NONE',  ( 0.000000000000000000, 0.000000000000000000, 1.000000000000000000 ) ) ;
#40767=VECTOR ( 'NONE', #68257, 1000.000000000000000 ) ;
#40787=CARTESIAN_POINT ( 'NONE',  ( 13.95692576442265853, 14.76984994696949727, -5.331646315825722127 ) ) ;
#40791=AXIS2_PLACEMENT_3D ( 'NONE', #92004, #23533, #46500 ) ;
#40796=B_SPLINE_CURVE_WITH_KNOTS ( 'NONE', 3,
 ( #90114, #76105, #22628, #66635, #89627, #14135 ),
 .UNSPECIFIED., .F., .F.,
 ( 4, 2, 4 ),
 ( 3.409110551496111039E-05, 0.0004400426677367849995, 0.0008459942299586088819 ),
 .UNSPECIFIED. ) ;
#40797=AXIS2_PLACEMENT_3D ( 'NONE', #67224, #42747, #88235 ) ;
#40805=LINE ( 'NONE', #26273, #63799 ) ;
#40806=DIRECTION ( 'NONE',  ( 0.000000000000000000, 0.000000000000000000, -1.000000000000000000 ) ) ;
#40808=DIRECTION ( 'NONE',  ( -0.000000000000000000, -1.000000000000000000, -0.000000000000000000 ) ) ;
#40809=FACE_OUTER_BOUND ( 'NONE', #89386, .T. ) ;
#40815=ORIENTED_EDGE ( 'NONE', *, *, #73229, .T. ) ;
#40818=LINE ( 'NONE', #41808, #85061 ) ;
#40819=CARTESIAN_POINT ( 'NONE',  ( -13.14228782657345107, 15.00000000000000000, 7.230509711182143917 ) ) ;
#40840=VECTOR ( 'NONE', #43241, 1000.000000000000114 ) ;
#40843=AXIS2_PLACEMENT_3D ( 'NONE', #5316, #95310, #42812 ) ;
#40864=AXIS2_PLACEMENT_3D ( 'NONE', #30506, #8027, #23036 ) ;
#40865=ORIENTED_EDGE ( 'NONE', *, *, #63561, .F. ) ;
#40866=VECTOR ( 'NONE', #17869, 1000.000000000000000 ) ;
#40869=VECTOR ( 'NONE', #68346, 1000.000000000000000 ) ;
#40871=CARTESIAN_POINT ( 'NONE',  ( 13.07751017357383994, 15.00000000000000000, -6.263284095430508458 ) ) ;
#40878=ORIENTED_EDGE ( 'NONE', *, *, #32567, .F. ) ;
#40886=DIRECTION ( 'NONE',  ( 0.6087614290087296487, 0.000000000000000000, -0.7933533402912281707 ) ) ;
#40890=AXIS2_PLACEMENT_3D ( 'NONE', #2957, #95407, #48425 ) ;
#40902=CARTESIAN_POINT ( 'NONE',  ( -1.780824192092595792, 0.3639308653492316359, 14.89391369643515617 ) ) ;
#40905=VECTOR ( 'NONE', #16919, 1000.000000000000114 ) ;
#40910=CARTESIAN_POINT ( 'NONE',  ( 4.096035146093440993, 4.852245006323173772E-16, 13.90943910019262120 ) ) ;
#40913=CARTESIAN_POINT ( 'NONE',  ( 1.548803529117991573, 0.000000000000000000, 5.228673087012104759 ) ) ;
#40922=DIRECTION ( 'NONE',  ( -0.000000000000000000, 1.000000000000000000, -0.000000000000000000 ) ) ;
#40925=EDGE_CURVE ( 'NONE', #23291, #66530, #79912, .T. ) ;
#40935=DIRECTION ( 'NONE',  ( 0.000000000000000000, 1.000000000000000000, 0.000000000000000000 ) ) ;
#40936=CARTESIAN_POINT ( 'NONE',  ( -1.983216688681034068, 0.000000000000000000, 14.11131997956736406 ) ) ;
#40937=CARTESIAN_POINT ( 'NONE',  ( -5.204170427930421283E-15, 5.553748834913975863, -14.16423886937410082 ) ) ;
#40938=VECTOR ( 'NONE', #74335, 1000.000000000000227 ) ;
#40941=ORIENTED_EDGE ( 'NONE', *, *, #14836, .F. ) ;
#40948=CARTESIAN_POINT ( 'NONE',  ( 3.469446951953614189E-15, 10.93830936912750573, 11.92686044187656513 ) ) ;
#40965=VECTOR ( 'NONE', #12249, 1000.000000000000000 ) ;
#40968=TOROIDAL_SURFACE ( 'NONE', #56929, 14.49999999999999822, 0.5000000000000000000 ) ;
#40983=ORIENTED_EDGE ( 'NONE', *, *, #61474, .T. ) ;
#41003=CARTESIAN_POINT ( 'NONE',  ( -11.09922568453594316, -25.45969866340290721, 6.408140936763246920 ) ) ;
#41017=ORIENTED_EDGE ( 'NONE', *, *, #75348, .T. ) ;
#41028=CARTESIAN_POINT ( 'NONE',  ( -4.841308736149794179, 0.2301500557980292461, 14.13449535775529675 ) ) ;
#41033=LINE ( 'NONE', #26023, #98119 ) ;
#41036=ORIENTED_EDGE ( 'NONE', *, *, #56910, .F. ) ;
#41037=VERTEX_POINT ( 'NONE', #77153 ) ;
#41055=CARTESIAN_POINT ( 'NONE',  ( -3.795296366450300773, -27.15458449841936428, 14.16423886937410437 ) ) ;
#41060=CIRCLE ( 'NONE', #77733, 15.00000000000000000 ) ;
#41068=CARTESIAN_POINT ( 'NONE',  ( -10.70613742633244669, 4.850979303660538556E-16, -9.778988772285387654 ) ) ;
#41072=CARTESIAN_POINT ( 'NONE',  ( -10.88017736071109987, 3.272018677488170990, 2.915334737309934532 ) ) ;
#41075=CARTESIAN_POINT ( 'NONE',  ( 0.000000000000000000, 0.5000000000000004441, 0.000000000000000000 ) ) ;
#41094=DIRECTION ( 'NONE',  ( -0.000000000000000000, -1.000000000000000000, -0.000000000000000000 ) ) ;
#41098=AXIS2_PLACEMENT_3D ( 'NONE', #97115, #60062, #83572 ) ;
#41102=DIRECTION ( 'NONE',  ( -0.000000000000000000, 1.000000000000000000, -0.000000000000000000 ) ) ;
#41108=CARTESIAN_POINT ( 'NONE',  ( 0.000000000000000000, 0.5000000000000004441, 0.000000000000000000 ) ) ;
#41110=ORIENTED_EDGE ( 'NONE', *, *, #16039, .T. ) ;
#41123=CARTESIAN_POINT ( 'NONE',  ( 8.527530157486175710, 8.925597817667455303, -4.923371831947298993 ) ) ;
#41125=FACE_OUTER_BOUND ( 'NONE', #14831, .T. ) ;
#41127=DIRECTION ( 'NONE',  ( 0.000000000000000000, 1.000000000000000000, 0.000000000000000000 ) ) ;
#41128=ORIENTED_EDGE ( 'NONE', *, *, #47526, .F. ) ;
#41135=CARTESIAN_POINT ( 'NONE',  ( 12.25993886608605443, 15.00000000000000000, -8.642563219313617040 ) ) ;
#41139=CARTESIAN_POINT ( 'NONE',  ( -11.09922568453594316, 29.54030133659710344, 6.408140936763246920 ) ) ;
#41142=EDGE_LOOP ( 'NONE', ( #2634, #56059, #28458, #20230 ) ) ;
#41149=AXIS2_PLACEMENT_3D ( 'NONE', #18659, #41666, #11147 ) ;
#41150=CARTESIAN_POINT ( 'NONE',  ( 0.000000000000000000, 35.00000000000000000, 0.000000000000000000 ) ) ;
#41155=VERTEX_POINT ( 'NONE', #57595 ) ;
#41158=CARTESIAN_POINT ( 'NONE',  ( 0.000000000000000000, 14.49999999999999822, 0.000000000000000000 ) ) ;
#41162=EDGE_CURVE ( 'NONE', #59403, #26337, #89085, .T. ) ;
#41167=DIRECTION ( 'NONE',  ( 0.000000000000000000, 0.000000000000000000, 1.000000000000000000 ) ) ;
#41175=VECTOR ( 'NONE', #37144, 1000.000000000000000 ) ;
#41178=LINE ( 'NONE', #72134, #28106 ) ;
#41179=ORIENTED_EDGE ( 'NONE', *, *, #213, .T. ) ;
#41187=CARTESIAN_POINT ( 'NONE',  ( 2.174473938468991285, 0.000000000000000000, -5.000947681547184942 ) ) ;
#41188=DIRECTION ( 'NONE',  ( 0.000000000000000000, 0.000000000000000000, 1.000000000000000000 ) ) ;
#41191=CARTESIAN_POINT ( 'NONE',  ( 10.36894250292378850, 29.92874883491397853, -10.36894250292379027 ) ) ;
#41209=FACE_OUTER_BOUND ( 'NONE', #34197, .T. ) ;
#41215=ORIENTED_EDGE ( 'NONE', *, *, #84673, .T. ) ;
#41225=EDGE_CURVE ( 'NONE', #50127, #70139, #96608, .T. ) ;
#41229=ORIENTED_EDGE ( 'NONE', *, *, #76441, .F. ) ;
#41230=DIRECTION ( 'NONE',  ( 0.000000000000000000, 0.000000000000000000, 1.000000000000000000 ) ) ;
#41242=DIRECTION ( 'NONE',  ( -0.000000000000000000, -1.000000000000000000, -0.000000000000000000 ) ) ;
#41245=B_SPLINE_CURVE_WITH_KNOTS ( 'NONE', 3,
 ( #86929, #56918, #42912, #49912, #56443, #72407 ),
 .UNSPECIFIED., .F., .F.,
 ( 4, 2, 4 ),
 ( 0.0002800267093156154179, 0.0006862322000234324405, 0.001092437690731249463 ),
 .UNSPECIFIED. ) ;
#41250=DIRECTION ( 'NONE',  ( 0.8788171126619646056, 0.000000000000000000, 0.4771587602596096267 ) ) ;
#41251=ORIENTED_EDGE ( 'NONE', *, *, #20881, .T. ) ;
#41252=EDGE_CURVE ( 'NONE', #95502, #59148, #26611, .T. ) ;
#41254=EDGE_LOOP ( 'NONE', ( #1198, #44048, #67777, #97189, #98826, #29550 ) ) ;
#41261=CARTESIAN_POINT ( 'NONE',  ( 14.99847009497948136, 0.3639309181704115104, 0.2142307401081242346 ) ) ;
#41263=CARTESIAN_POINT ( 'NONE',  ( 9.382169495545419124, -4.001365330069578619, 9.382169495545417348 ) ) ;
#41276=CARTESIAN_POINT ( 'NONE',  ( -8.209432707284950226, 15.00000000000000000, 12.55409154915480485 ) ) ;
#41279=DIRECTION ( 'NONE',  ( 0.000000000000000000, 0.000000000000000000, -1.000000000000000000 ) ) ;
#41282=DIRECTION ( 'NONE',  ( -0.5372996083468249973, 0.000000000000000000, 0.8433914458128849434 ) ) ;
#41285=CARTESIAN_POINT ( 'NONE',  ( 14.02068044289375415, 15.00000000000000000, 5.331089937175756965 ) ) ;
#41289=DIRECTION ( 'NONE',  ( 0.000000000000000000, 1.000000000000000000, 0.000000000000000000 ) ) ;
#41293=CARTESIAN_POINT ( 'NONE',  ( 9.876730923139305673, 0.3640475087720985714, -11.28938378619063343 ) ) ;
#41300=SURFACE_STYLE_USAGE ( .BOTH. , #48274 ) ;
#41313=CARTESIAN_POINT ( 'NONE',  ( 1.683889348827612823E-15, 15.00000000000000000, -13.75000000000001776 ) ) ;
#41320=VECTOR ( 'NONE', #50941, 1000.000000000000000 ) ;
#41322=DIRECTION ( 'NONE',  ( -0.000000000000000000, -1.000000000000000000, -0.000000000000000000 ) ) ;
#41323=ORIENTED_EDGE ( 'NONE', *, *, #39775, .F. ) ;
#41342=CARTESIAN_POINT ( 'NONE',  ( -12.87890026492945239, 0.04922511925147124434, 7.195834080858260151 ) ) ;
#41343=CARTESIAN_POINT ( 'NONE',  ( -7.618485323809105481, 1.609362599783170644E-16, -12.48587314215772892 ) ) ;
#41346=FACE_OUTER_BOUND ( 'NONE', #26858, .T. ) ;
#41349=DIRECTION ( 'NONE',  ( -0.000000000000000000, -1.000000000000000000, -0.000000000000000000 ) ) ;
#41360=ADVANCED_FACE ( 'NONE', ( #6090 ), #82074, .F. ) ;
#41361=ADVANCED_FACE ( 'NONE', ( #37087 ), #66311, .T. ) ;
#41370=ORIENTED_EDGE ( 'NONE', *, *, #84035, .F. ) ;
#41374=CARTESIAN_POINT ( 'NONE',  ( 13.21272562211574986, 15.00000000000000178, -6.271554226548150091 ) ) ;
#41380=CARTESIAN_POINT ( 'NONE',  ( 0.000000000000000000, 0.5000000000000004441, 0.000000000000000000 ) ) ;
#41401=DIRECTION ( 'NONE',  ( 0.000000000000000000, 1.000000000000000000, 0.000000000000000000 ) ) ;
#41402=VERTEX_POINT ( 'NONE', #14730 ) ;
#41411=DIRECTION ( 'NONE',  ( 0.000000000000000000, 1.000000000000000000, 0.000000000000000000 ) ) ;
#41415=DIRECTION ( 'NONE',  ( 0.000000000000000000, 0.000000000000000000, 1.000000000000000000 ) ) ;
#41419=DIRECTION ( 'NONE',  ( -0.000000000000000000, -1.000000000000000000, -0.000000000000000000 ) ) ;
#41421=EDGE_LOOP ( 'NONE', ( #44550, #48852, #68639, #69559, #29442, #48536 ) ) ;
#41433=DIRECTION ( 'NONE',  ( 0.000000000000000000, 0.000000000000000000, 1.000000000000000000 ) ) ;
#41437=ORIENTED_EDGE ( 'NONE', *, *, #86987, .F. ) ;
#41439=ADVANCED_FACE ( 'NONE', ( #7216 ), #55109, .T. ) ;
#41443=CARTESIAN_POINT ( 'NONE',  ( 3.469446951953614189E-15, 3.053748834913973198, 14.16423886937410259 ) ) ;
#41453=DIRECTION ( 'NONE',  ( 0.7132504491541897806, 0.000000000000000000, -0.7009092642998425715 ) ) ;
#41458=CARTESIAN_POINT ( 'NONE',  ( 12.67147417979175827, 0.04962887043496324452, -7.555862176155505594 ) ) ;
#41468=ADVANCED_FACE ( 'NONE', ( #95506 ), #72987, .F. ) ;
#41471=ADVANCED_FACE ( 'NONE', ( #4517 ), #32762, .T. ) ;
#41475=CARTESIAN_POINT ( 'NONE',  ( -10.64017930668197209, 14.49999999999999112, -10.57291749337233000 ) ) ;
#41478=FACE_OUTER_BOUND ( 'NONE', #7137, .T. ) ;
#41480=LINE ( 'NONE', #26441, #28002 ) ;
#41488=VERTEX_POINT ( 'NONE', #11020 ) ;
#41492=DIRECTION ( 'NONE',  ( 0.000000000000000000, 0.000000000000000000, -1.000000000000000000 ) ) ;
#41499=CARTESIAN_POINT ( 'NONE',  ( 9.876730923139298568, 0.5000000000000004441, -11.28938378619063165 ) ) ;
#41501=ADVANCED_FACE ( 'NONE', ( #3534 ), #34981, .F. ) ;
#41502=CARTESIAN_POINT ( 'NONE',  ( -10.58981376305275468, 15.00000000000000000, -9.535111140613857117 ) ) ;
#41504=CARTESIAN_POINT ( 'NONE',  ( 12.81628187352647608, -28.37636533006957507, -2.602085213965210642E-15 ) ) ;
#41514=DIRECTION ( 'NONE',  ( 0.000000000000000000, 0.000000000000000000, 1.000000000000000000 ) ) ;
#41516=VERTEX_POINT ( 'NONE', #49999 ) ;
#41527=CARTESIAN_POINT ( 'NONE',  ( 0.000000000000000000, 0.5000000000000004441, 0.000000000000000000 ) ) ;
#41530=VERTEX_POINT ( 'NONE', #73473 ) ;
#41531=B_SPLINE_CURVE_WITH_KNOTS ( 'NONE', 3,
 ( #95583, #11584, #79095, #42100, #50569, #50075 ),
 .UNSPECIFIED., .F., .F.,
 ( 4, 2, 4 ),
 ( 0.0002800003244075575958, 0.0006862055569968510474, 0.001092410789586144553 ),
 .UNSPECIFIED. ) ;
#41532=CARTESIAN_POINT ( 'NONE',  ( 14.56311970191025296, 0.2301500865527682516, 3.337330457605979905 ) ) ;
#41537=CARTESIAN_POINT ( 'NONE',  ( 2.393480905993052854, 0.5000000000000004441, 14.80781041047752922 ) ) ;
#41539=CIRCLE ( 'NONE', #24053, 14.49999999999999822 ) ;
#41546=EDGE_LOOP ( 'NONE', ( #13379, #60050, #98272, #87711, #46045, #51566 ) ) ;
#41553=EDGE_CURVE ( 'NONE', #63527, #50188, #47418, .T. ) ;
#41554=TOROIDAL_SURFACE ( 'NONE', #97436, 14.49999999999999822, 0.5000000000000000000 ) ;
#41558=CARTESIAN_POINT ( 'NONE',  ( -14.16423886937409726, -32.98791783175269643, 3.795296366450320757 ) ) ;
#41568=DIRECTION ( 'NONE',  ( -0.000000000000000000, -1.000000000000000000, -0.000000000000000000 ) ) ;
#41570=CARTESIAN_POINT ( 'NONE',  ( 4.873787042390699931, 0.000000000000000000, 13.39061984619922718 ) ) ;
#41573=CARTESIAN_POINT ( 'NONE',  ( -10.88017736071110164, 12.85535201082150181, -2.915334737309917212 ) ) ;
#41580=B_SPLINE_CURVE_WITH_KNOTS ( 'NONE', 3,
 ( #48726, #70271, #1788, #79231, #41261, #62746 ),
 .UNSPECIFIED., .F., .F.,
 ( 4, 2, 4 ),
 ( 0.0002800154274912481246, 0.0006862208078174526597, 0.001092426188143657195 ),
 .UNSPECIFIED. ) ;
#41582=DIRECTION ( 'NONE',  ( 0.000000000000000000, 1.000000000000000000, -0.000000000000000000 ) ) ;
#41583=EDGE_CURVE ( 'NONE', #10027, #17080, #12001, .T. ) ;
#41586=EDGE_CURVE ( 'NONE', #63236, #48866, #88488, .T. ) ;
#41595=CARTESIAN_POINT ( 'NONE',  ( 14.35840480524199947, 0.5000000000000004441, -4.340070442838851683 ) ) ;
#41601=CARTESIAN_POINT ( 'NONE',  ( -8.470640952599010731, 14.99999999999807443, -11.92295067085447968 ) ) ;
#41614=ADVANCED_FACE ( 'NONE', ( #5002 ), #96680, .T. ) ;
#41615=CYLINDRICAL_SURFACE ( 'NONE', #95545, 15.00000000000000000 ) ;
#41618=CARTESIAN_POINT ( 'NONE',  ( 7.208316651077764980, 2.883931151000783455, 7.208316651077762316 ) ) ;
#41622=DIRECTION ( 'NONE',  ( 0.000000000000000000, 1.000000000000000000, 0.000000000000000000 ) ) ;
#41623=CIRCLE ( 'NONE', #17638, 14.49999999999999822 ) ;
#41630=B_SPLINE_CURVE_WITH_KNOTS ( 'NONE', 3,
 ( #42332, #72805, #46998, #4347, #77491, #2027 ),
 .UNSPECIFIED., .F., .F.,
 ( 4, 2, 4 ),
 ( 0.0002800111042658719098, 0.0006862164422996730332, 0.001092421780333474157 ),
 .UNSPECIFIED. ) ;
#41646=VERTEX_POINT ( 'NONE', #80989 ) ;
#41649=CARTESIAN_POINT ( 'NONE',  ( -15.08495336817617982, -0.03417435944610275333, 5.321802168063332950 ) ) ;
#41653=LINE ( 'NONE', #40661, #9094 ) ;
#41656=DIRECTION ( 'NONE',  ( 0.000000000000000000, 1.000000000000000000, 0.000000000000000000 ) ) ;
#41657=ORIENTED_EDGE ( 'NONE', *, *, #39775, .T. ) ;
#41666=DIRECTION ( 'NONE',  ( 0.000000000000000000, 1.000000000000000000, 0.000000000000000000 ) ) ;
#41668=ADVANCED_FACE ( 'NONE', ( #88987 ), #48749, .T. ) ;
#41669=VERTEX_POINT ( 'NONE', #50979 ) ;
#41672=CIRCLE ( 'NONE', #154, 14.49999999999999822 ) ;
#41679=CARTESIAN_POINT ( 'NONE',  ( 10.88017736071110164, -19.64464798917849464, 2.915334737309921209 ) ) ;
#41695=LINE ( 'NONE', #71205, #5658 ) ;
#41700=ORIENTED_EDGE ( 'NONE', *, *, #17841, .T. ) ;
#41701=DIRECTION ( 'NONE',  ( 0.000000000000000000, 1.000000000000000000, 0.000000000000000000 ) ) ;
#41709=DIRECTION ( 'NONE',  ( -0.1822355254921381451, 0.000000000000000000, -0.9832549075639562819 ) ) ;
#41715=ORIENTED_EDGE ( 'NONE', *, *, #56679, .F. ) ;
#41717=CARTESIAN_POINT ( 'NONE',  ( 6.090257717040516106, -3.095058389267212256E-15, 13.29726560978572714 ) ) ;
#41729=PLANE ( 'NONE',  #77908 ) ;
#41732=CARTESIAN_POINT ( 'NONE',  ( 4.923371831947295441, -30.65773551566587685, -8.527530157486179263 ) ) ;
#41734=EDGE_LOOP ( 'NONE', ( #10479, #94371, #4293, #62399 ) ) ;
#41736=VECTOR ( 'NONE', #72727, 1000.000000000000114 ) ;
#41747=CARTESIAN_POINT ( 'NONE',  ( -3.434112377981067610, 3.081968003263759304, -12.81628187352647252 ) ) ;
#41754=AXIS2_PLACEMENT_3D ( 'NONE', #82144, #36663, #21665 ) ;
#41756=CARTESIAN_POINT ( 'NONE',  ( 14.47650479471819551, 0.5000000000000004441, 3.928206833722108549 ) ) ;
#41759=DIRECTION ( 'NONE',  ( 0.000000000000000000, 0.000000000000000000, 1.000000000000000000 ) ) ;
#41762=CARTESIAN_POINT ( 'NONE',  ( 0.000000000000000000, 14.49999999999999822, 0.000000000000000000 ) ) ;
#41765=DIRECTION ( 'NONE',  ( 0.000000000000000000, 0.000000000000000000, 1.000000000000000000 ) ) ;
#41771=CARTESIAN_POINT ( 'NONE',  ( -14.26139399674453578, 15.00000000000000000, -2.619664342929994838 ) ) ;
#41776=CARTESIAN_POINT ( 'NONE',  ( 14.02068044289383231, 14.63606918466297557, -5.331089937175661930 ) ) ;
#41784=VERTEX_POINT ( 'NONE', #43960 ) ;
#41793=CARTESIAN_POINT ( 'NONE',  ( 14.40939250469963895, 15.00000000000000000, -1.618458416365745389 ) ) ;
#41798=DIRECTION ( 'NONE',  ( 0.000000000000000000, 1.000000000000000000, 0.000000000000000000 ) ) ;
#41801=CIRCLE ( 'NONE', #94457, 15.00000000000000000 ) ;
#41804=ORIENTED_EDGE ( 'NONE', *, *, #54038, .F. ) ;
#41805=EDGE_CURVE ( 'NONE', #26148, #32242, #88737, .T. ) ;
#41808=CARTESIAN_POINT ( 'NONE',  ( -10.93781366033354097, 15.00000000000000000, 10.26470809774057713 ) ) ;
#41811=CARTESIAN_POINT ( 'NONE',  ( 5.377205135395861646, 14.76930270348882601, 13.94000429068785074 ) ) ;
#41818=ORIENTED_EDGE ( 'NONE', *, *, #32320, .T. ) ;
#41834=FACE_OUTER_BOUND ( 'NONE', #45801, .T. ) ;
#41851=ORIENTED_EDGE ( 'NONE', *, *, #7131, .T. ) ;
#41855=ORIENTED_EDGE ( 'NONE', *, *, #71251, .F. ) ;
#41858=CIRCLE ( 'NONE', #88146, 14.49999999999999822 ) ;
#41859=CARTESIAN_POINT ( 'NONE',  ( -9.509319644403765537, 13.17686044187662020, 7.198808227794258663 ) ) ;
#41860=LINE ( 'NONE', #49335, #56837 ) ;
#41867=EDGE_LOOP ( 'NONE', ( #17864, #62609, #604, #66434 ) ) ;
#41869=ORIENTED_EDGE ( 'NONE', *, *, #72813, .F. ) ;
#41882=ORIENTED_EDGE ( 'NONE', *, *, #930, .F. ) ;
#41885=AXIS2_PLACEMENT_3D ( 'NONE', #73215, #26738, #41765 ) ;
#41886=VECTOR ( 'NONE', #40269, 1000.000000000000114 ) ;
#41888=VECTOR ( 'NONE', #4094, 1000.000000000000000 ) ;
#41899=CARTESIAN_POINT ( 'NONE',  ( 4.431036607602466759, 0.5000000000000004441, 14.33059365769913818 ) ) ;
#41900=EDGE_CURVE ( 'NONE', #39436, #15469, #59287, .T. ) ;
#41907=CARTESIAN_POINT ( 'NONE',  ( -13.95692576442134758, 14.76984994697213516, 5.331646315825635973 ) ) ;
#41919=CARTESIAN_POINT ( 'NONE',  ( 14.02068044289376303, 14.63595249122788999, 5.331089937175756077 ) ) ;
#41920=EDGE_CURVE ( 'NONE', #48512, #27481, #54503, .T. ) ;
#41921=DIRECTION ( 'NONE',  ( 0.000000000000000000, 0.000000000000000000, -1.000000000000000000 ) ) ;
#41944=CARTESIAN_POINT ( 'NONE',  ( -14.02068044289389626, 14.49999999999999112, 5.331089937175563342 ) ) ;
#41948=DIRECTION ( 'NONE',  ( -6.217248937900876626E-15, 0.000000000000000000, 1.000000000000000000 ) ) ;
#41949=CARTESIAN_POINT ( 'NONE',  ( 4.873787042390789637, -0.03417435944610275333, -13.39061984619918988 ) ) ;
#41951=ORIENTED_EDGE ( 'NONE', *, *, #18200, .F. ) ;
#41967=VERTEX_POINT ( 'NONE', #46920 ) ;
#41972=CARTESIAN_POINT ( 'NONE',  ( 6.189644032515776217, 0.04922511925147198680, -13.39157970158797006 ) ) ;
#41986=DIRECTION ( 'NONE',  ( -0.8788171126619678253, 0.000000000000000000, 0.4771587602596037425 ) ) ;
#41989=CARTESIAN_POINT ( 'NONE',  ( 9.382169495545415572, -32.75136533006958217, -9.382169495545422677 ) ) ;
#41990=ORIENTED_EDGE ( 'NONE', *, *, #98339, .F. ) ;
#41998=CARTESIAN_POINT ( 'NONE',  ( -14.91937968691864036, 0.2306972965111904195, -0.8063277559920134507 ) ) ;
#42002=VERTEX_POINT ( 'NONE', #78905 ) ;
#42004=CARTESIAN_POINT ( 'NONE',  ( -7.551349515323269479, 15.00000000000000000, 12.08468537022900868 ) ) ;
#42010=B_SPLINE_CURVE_WITH_KNOTS ( 'NONE', 3,
 ( #93524, #71038, #33017, #41532, #56996, #94504 ),
 .UNSPECIFIED., .F., .F.,
 ( 4, 2, 4 ),
 ( 0.0002800026249563246535, 0.0006862078800502478294, 0.001092413135144171005 ),
 .UNSPECIFIED. ) ;
#42012=EDGE_CURVE ( 'NONE', #54920, #5711, #38947, .T. ) ;
#42021=CARTESIAN_POINT ( 'NONE',  ( 5.803070148808231465, 15.00000000000000000, 13.28812917035392260 ) ) ;
#42028=DIRECTION ( 'NONE',  ( 0.000000000000000000, 0.000000000000000000, 1.000000000000000000 ) ) ;
#42034=ORIENTED_EDGE ( 'NONE', *, *, #91679, .F. ) ;
#42044=CARTESIAN_POINT ( 'NONE',  ( 12.26659068614894466, -35.27958449841936073, -7.082119434687053960 ) ) ;
#42047=ORIENTED_EDGE ( 'NONE', *, *, #76649, .T. ) ;
#42056=EDGE_CURVE ( 'NONE', #23318, #62480, #23317, .T. ) ;
#42060=CARTESIAN_POINT ( 'NONE',  ( -7.964842623401172439, 8.688685344154842838, 7.964842623401183097 ) ) ;
#42064=EDGE_CURVE ( 'NONE', #20489, #34423, #82310, .T. ) ;
#42066=AXIS2_PLACEMENT_3D ( 'NONE', #63622, #94128, #50474 ) ;
#42074=DIRECTION ( 'NONE',  ( 0.000000000000000000, 1.000000000000000000, 0.000000000000000000 ) ) ;
#42088=ORIENTED_EDGE ( 'NONE', *, *, #2629, .T. ) ;
#42093=CARTESIAN_POINT ( 'NONE',  ( 0.000000000000000000, 14.49999999999999822, 0.000000000000000000 ) ) ;
#42095=CARTESIAN_POINT ( 'NONE',  ( -10.82078848414227146, -0.03417435944610275333, 11.78082904627290795 ) ) ;
#42096=CARTESIAN_POINT ( 'NONE',  ( -13.48255862861919852, 3.931018169630358772E-16, -5.335786055104346559 ) ) ;
#42099=AXIS2_PLACEMENT_3D ( 'NONE', #55658, #85658, #17177 ) ;
#42100=CARTESIAN_POINT ( 'NONE',  ( -4.841308736149450453, 14.76984994419931674, -14.13449535775674626 ) ) ;
#42102=CARTESIAN_POINT ( 'NONE',  ( 7.208316651077762316, 4.133931151000787452, -7.208316651077764980 ) ) ;
#42103=EDGE_CURVE ( 'NONE', #3422, #65076, #26010, .T. ) ;
#42104=VERTEX_POINT ( 'NONE', #17436 ) ;
#42109=ORIENTED_EDGE ( 'NONE', *, *, #32257, .F. ) ;
#42115=CARTESIAN_POINT ( 'NONE',  ( 11.48952521350024192, 4.570664323179305100E-16, -8.845383562533745803 ) ) ;
#42116=EDGE_CURVE ( 'NONE', #63236, #89545, #9927, .T. ) ;
#42118=VERTEX_POINT ( 'NONE', #31908 ) ;
#42121=VERTEX_POINT ( 'NONE', #62409 ) ;
#42137=DIRECTION ( 'NONE',  ( 0.4461978131098069400, 0.000000000000000000, -0.8949343616020258851 ) ) ;
#42138=EDGE_LOOP ( 'NONE', ( #69765, #73655, #7311, #11707, #86197, #6197 ) ) ;
#42139=CARTESIAN_POINT ( 'NONE',  ( -1.915564264621230972, 4.378229052359348391E-16, -14.37291249357993372 ) ) ;
#42146=CARTESIAN_POINT ( 'NONE',  ( -7.313705784284680433, 0.5000000000000004441, 13.09617149020738935 ) ) ;
#42150=CARTESIAN_POINT ( 'NONE',  ( 11.81378540890930751, 15.00000000000000000, 7.968498874458199488 ) ) ;
#42154=VECTOR ( 'NONE', #34176, 1000.000000000000114 ) ;
#42163=AXIS2_PLACEMENT_3D ( 'NONE', #96646, #87639, #80644 ) ;
#42169=CARTESIAN_POINT ( 'NONE',  ( 5.440088680355549045, -23.60298132251182324, -9.422509992056141925 ) ) ;
#42175=CARTESIAN_POINT ( 'NONE',  ( 14.29484424893245453, 14.76984993772165744, -4.345072767107134304 ) ) ;
#42196=LINE ( 'NONE', #88163, #51138 ) ;
#42199=LINE ( 'NONE', #95176, #78646 ) ;
#42202=DIRECTION ( 'NONE',  ( -0.5075383629606967650, 0.000000000000000000, -0.8616291604415300398 ) ) ;
#42214=CARTESIAN_POINT ( 'NONE',  ( -2.826948239413729080, 0.2306972965111893925, -14.67127868811028968 ) ) ;
#42216=CARTESIAN_POINT ( 'NONE',  ( -8.527530157486182816, -39.40773551566587685, -4.923371831947288335 ) ) ;
#42217=ORIENTED_EDGE ( 'NONE', *, *, #98591, .F. ) ;
#42219=CARTESIAN_POINT ( 'NONE',  ( 0.000000000000000000, 14.49999999999999822, 0.000000000000000000 ) ) ;
#42227=CARTESIAN_POINT ( 'NONE',  ( 0.000000000000000000, 0.000000000000000000, 0.000000000000000000 ) ) ;
#42231=CARTESIAN_POINT ( 'NONE',  ( 9.382169495545415572, 7.248634669930418717, -9.382169495545422677 ) ) ;
#42232=ORIENTED_EDGE ( 'NONE', *, *, #76596, .F. ) ;
#42244=ADVANCED_FACE ( 'NONE', ( #26883 ), #49871, .F. ) ;
#42248=EDGE_CURVE ( 'NONE', #71871, #54278, #12090, .T. ) ;
#42256=CARTESIAN_POINT ( 'NONE',  ( 3.836325488036083087, 15.00000000000000000, 14.50112432709425114 ) ) ;
#42261=AXIS2_PLACEMENT_3D ( 'NONE', #93122, #32117, #92152 ) ;
#42266=CARTESIAN_POINT ( 'NONE',  ( 14.99847009497950800, 14.49999999999999112, 0.2142307401081135487 ) ) ;
#42268=ORIENTED_EDGE ( 'NONE', *, *, #92818, .T. ) ;
#42269=CARTESIAN_POINT ( 'NONE',  ( -9.742785792574940373, 2.505135511184877206, -5.624999999999991118 ) ) ;
#42274=B_SPLINE_CURVE_WITH_KNOTS ( 'NONE', 3,
 ( #42423, #87906, #19420, #95925, #3934, #10934 ),
 .UNSPECIFIED., .F., .F.,
 ( 4, 2, 4 ),
 ( 3.409110551496114428E-05, 0.0004400426677367863006, 0.0008459942299586114840 ),
 .UNSPECIFIED. ) ;
#42281=EDGE_CURVE ( 'NONE', #10227, #38291, #92569, .T. ) ;
#42286=ORIENTED_EDGE ( 'NONE', *, *, #87259, .T. ) ;
#42291=CIRCLE ( 'NONE', #3979, 15.00000000000000000 ) ;
#42302=DIRECTION ( 'NONE',  ( -0.9799247046208282574, 0.000000000000000000, -0.1993679344172039347 ) ) ;
#42311=ORIENTED_EDGE ( 'NONE', *, *, #27259, .F. ) ;
#42319=CARTESIAN_POINT ( 'NONE',  ( 9.898881779040729967, 15.00000000000000000, -10.25059215482576214 ) ) ;
#42323=DIRECTION ( 'NONE',  ( 0.000000000000000000, 1.000000000000000000, 0.000000000000000000 ) ) ;
#42327=VERTEX_POINT ( 'NONE', #94393 ) ;
#42332=CARTESIAN_POINT ( 'NONE',  ( -9.240973841163452107, 15.00000000000000000, -11.17382667070385160 ) ) ;
#42340=CARTESIAN_POINT ( 'NONE',  ( 14.56372689393330688, 14.95037103587380756, -2.356940382833013548 ) ) ;
#42348=VERTEX_POINT ( 'NONE', #72866 ) ;
#42349=AXIS2_PLACEMENT_3D ( 'NONE', #12977, #56524, #96505 ) ;
#42350=CYLINDRICAL_SURFACE ( 'NONE', #74937, 15.00000000000000000 ) ;
#42356=CARTESIAN_POINT ( 'NONE',  ( -8.758038983380448173, 2.271305648288091561, -7.488716559648692872 ) ) ;
#42359=ORIENTED_EDGE ( 'NONE', *, *, #68707, .T. ) ;
#42360=EDGE_CURVE ( 'NONE', #56243, #30649, #57863, .T. ) ;
#42375=CARTESIAN_POINT ( 'NONE',  ( 11.35178980618967337, 0.5000000000000004441, 9.804941009311999522 ) ) ;
#42381=CARTESIAN_POINT ( 'NONE',  ( 9.402796353261059892, 14.63606911086599283, 11.68706210897767761 ) ) ;
#42384=CARTESIAN_POINT ( 'NONE',  ( 11.25000000000000178, 7.618033628982655792, -2.373340393710807175E-15 ) ) ;
#42389=CARTESIAN_POINT ( 'NONE',  ( 7.684764310694878198, 0.5000000000000004441, -12.88194075009934991 ) ) ;
#42401=AXIS2_PLACEMENT_3D ( 'NONE', #39212, #69699, #1229 ) ;
#42403=EDGE_CURVE ( 'NONE', #38271, #37318, #21361, .T. ) ;
#42406=CARTESIAN_POINT ( 'NONE',  ( 14.49440716394873618, 15.00000000000000000, -0.4026921475166200803 ) ) ;
#42409=LINE ( 'NONE', #71912, #29492 ) ;
#42415=EDGE_LOOP ( 'NONE', ( #23069, #12132, #75640, #4018 ) ) ;
#42417=EDGE_CURVE ( 'NONE', #30382, #5711, #45638, .T. ) ;
#42422=CARTESIAN_POINT ( 'NONE',  ( 13.21236992757670059, -0.03417435944610275333, 5.338143956176803151 ) ) ;
#42423=CARTESIAN_POINT ( 'NONE',  ( 4.431036607602561794, 0.5000000000000004441, -14.33059365769911153 ) ) ;
#42428=LINE ( 'NONE', #73897, #2063 ) ;
#42440=ORIENTED_EDGE ( 'NONE', *, *, #54731, .T. ) ;
#42454=VERTEX_POINT ( 'NONE', #5385 ) ;
#42458=CARTESIAN_POINT ( 'NONE',  ( -8.375939845167836850, 15.00000000000000000, 11.52849216984293257 ) ) ;
#42464=EDGE_CURVE ( 'NONE', #91634, #25488, #5866, .T. ) ;
#42465=CARTESIAN_POINT ( 'NONE',  ( -6.898461952320517732, 4.837215022590613936E-16, 12.75387089053304557 ) ) ;
#42468=CARTESIAN_POINT ( 'NONE',  ( 12.81628187352647252, -33.16803199673624647, -3.434112377981059172 ) ) ;
#42475=CIRCLE ( 'NONE', #42401, 14.49999999999999822 ) ;
#42477=EDGE_CURVE ( 'NONE', #81875, #30157, #59835, .T. ) ;
#42479=ORIENTED_EDGE ( 'NONE', *, *, #54863, .T. ) ;
#42483=CARTESIAN_POINT ( 'NONE',  ( 8.375939845167682307, 0.000000000000000000, 11.52849216984304448 ) ) ;
#42485=B_SPLINE_CURVE_WITH_KNOTS ( 'NONE', 3,
 ( #32193, #62695, #3200, #25226, #47704, #33182 ),
 .UNSPECIFIED., .F., .F.,
 ( 4, 2, 4 ),
 ( 3.409110551494653465E-05, 0.0004400426677367932937, 0.0008459942299586401069 ),
 .UNSPECIFIED. ) ;
#42486=ORIENTED_EDGE ( 'NONE', *, *, #91572, .F. ) ;
#42496=VECTOR ( 'NONE', #36690, 1000.000000000000000 ) ;
#42497=CARTESIAN_POINT ( 'NONE',  ( 10.64017930668211598, 14.49999999999999112, -10.57291749337218256 ) ) ;
#42499=ORIENTED_EDGE ( 'NONE', *, *, #44238, .T. ) ;
#42502=AXIS2_PLACEMENT_3D ( 'NONE', #28208, #35203, #43207 ) ;
#42504=UNCERTAINTY_MEASURE_WITH_UNIT (LENGTH_MEASURE( 1.000000000000000082E-05 ), #86783, 'distance_accuracy_value', 'NONE');
#42505=CARTESIAN_POINT ( 'NONE',  ( 0.000000000000000000, 0.5000000000000004441, 0.000000000000000000 ) ) ;
#42519=CARTESIAN_POINT ( 'NONE',  ( -12.26659068614895354, -28.61291783175269643, -7.082119434687038861 ) ) ;
#42522=ORIENTED_EDGE ( 'NONE', *, *, #64906, .F. ) ;
#42523=DIRECTION ( 'NONE',  ( -0.9969173337331284079, 0.000000000000000000, 0.07845909572783860142 ) ) ;
#42528=CARTESIAN_POINT ( 'NONE',  ( -14.64921366071931530, 14.95037108083259625, -1.748670679920710569 ) ) ;
#42532=CARTESIAN_POINT ( 'NONE',  ( 5.440088680355549045, 11.39701867748817854, -9.422509992056141925 ) ) ;
#42535=VECTOR ( 'NONE', #63557, 1000.000000000000000 ) ;
#42540=DIRECTION ( 'NONE',  ( -0.000000000000000000, -1.000000000000000000, -0.000000000000000000 ) ) ;
#42549=ORIENTED_EDGE ( 'NONE', *, *, #98116, .T. ) ;
#42550=CARTESIAN_POINT ( 'NONE',  ( -15.86177583122253765, -0.03417435944610275333, 2.069169861586545700 ) ) ;
#42552=CARTESIAN_POINT ( 'NONE',  ( 5.056330833737696651, 15.00000000000000000, -13.58983143751348521 ) ) ;
#42563=FACE_OUTER_BOUND ( 'NONE', #58808, .T. ) ;
#42566=ORIENTED_EDGE ( 'NONE', *, *, #26120, .T. ) ;
#42579=CARTESIAN_POINT ( 'NONE',  ( 10.19513985507834342, 0.3639309290920412776, -11.00268709613220786 ) ) ;
#42581=CARTESIAN_POINT ( 'NONE',  ( -9.846743663894590881, -3.782735515665876846, 2.638427012816840111 ) ) ;
#42582=ORIENTED_EDGE ( 'NONE', *, *, #11493, .T. ) ;
#42586=ORIENTED_EDGE ( 'NONE', *, *, #68231, .T. ) ;
#42600=EDGE_CURVE ( 'NONE', #89676, #59403, #82840, .T. ) ;
#42602=VERTEX_POINT ( 'NONE', #60336 ) ;
#42615=VERTEX_POINT ( 'NONE', #73855 ) ;
#42616=CARTESIAN_POINT ( 'NONE',  ( -14.62617646268090077, 14.49999999999999112, -3.327906561567068433 ) ) ;
#42621=CARTESIAN_POINT ( 'NONE',  ( 14.62617646268087768, 15.00000000000000000, -3.327906561566883692 ) ) ;
#42622=VERTEX_POINT ( 'NONE', #14360 ) ;
#42623=CARTESIAN_POINT ( 'NONE',  ( -6.898461952320517732, 4.837215022590613936E-16, 12.75387089053304557 ) ) ;
#42628=CARTESIAN_POINT ( 'NONE',  ( -14.09394518620614711, 4.304378373471060795E-16, 3.407449058785263940 ) ) ;
#42640=DIRECTION ( 'NONE',  ( -0.3338068592337649076, 0.000000000000000000, -0.9426414910921805390 ) ) ;
#42648=CARTESIAN_POINT ( 'NONE',  ( -5.204170427930421283E-15, -23.18631465584515894, -10.88017736071110342 ) ) ;
#42652=DIRECTION ( 'NONE',  ( 0.4924235601034769871, 0.000000000000000000, -0.8703556959398941473 ) ) ;
#42655=AXIS2_PLACEMENT_3D ( 'NONE', #13477, #20490, #57493 ) ;
#42663=DIRECTION ( 'NONE',  ( 0.000000000000000000, 0.000000000000000000, 1.000000000000000000 ) ) ;
#42665=DIRECTION ( 'NONE',  ( 0.000000000000000000, 1.000000000000000000, 0.000000000000000000 ) ) ;
#42667=ORIENTED_EDGE ( 'NONE', *, *, #13044, .F. ) ;
#42673=DIRECTION ( 'NONE',  ( 0.7826081568524191345, 0.000000000000000000, -0.6225146366376130835 ) ) ;
#42678=ORIENTED_EDGE ( 'NONE', *, *, #62762, .F. ) ;
#42681=EDGE_CURVE ( 'NONE', #88686, #30837, #44116, .T. ) ;
#42683=EDGE_LOOP ( 'NONE', ( #70781, #95721, #35430, #25596 ) ) ;
#42701=CARTESIAN_POINT ( 'NONE',  ( 8.527530157486175710, -36.07440218233254114, -4.923371831947298993 ) ) ;
#42704=ORIENTED_EDGE ( 'NONE', *, *, #94550, .F. ) ;
#42706=ORIENTED_EDGE ( 'NONE', *, *, #77720, .F. ) ;
#42713=CARTESIAN_POINT ( 'NONE',  ( 3.469446951953614189E-15, 5.373634669930425822, 12.81628187352647608 ) ) ;
#42721=VECTOR ( 'NONE', #61745, 1000.000000000000000 ) ;
#42727=VECTOR ( 'NONE', #38692, 1000.000000000000000 ) ;
#42729=VECTOR ( 'NONE', #49319, 1000.000000000000114 ) ;
#42731=VERTEX_POINT ( 'NONE', #47292 ) ;
#42733=CARTESIAN_POINT ( 'NONE',  ( 10.64017930668205736, 0.5000000000000004441, -10.57291749337215592 ) ) ;
#42743=DIRECTION ( 'NONE',  ( 0.000000000000000000, 1.000000000000000000, 0.000000000000000000 ) ) ;
#42745=B_SPLINE_CURVE_WITH_KNOTS ( 'NONE', 3,
 ( #91375, #70735, #52881, #86219, #17731, #90377 ),
 .UNSPECIFIED., .F., .F.,
 ( 4, 2, 4 ),
 ( 0.0002800518438787976978, 0.0006862575805824382581, 0.001092463317286078818 ),
 .UNSPECIFIED. ) ;
#42747=DIRECTION ( 'NONE',  ( -0.000000000000000000, -1.000000000000000000, -0.000000000000000000 ) ) ;
#42748=ORIENTED_EDGE ( 'NONE', *, *, #36474, .F. ) ;
#42753=CARTESIAN_POINT ( 'NONE',  ( 14.62232599144295264, 15.00000000000000888, 0.3548652576989754781 ) ) ;
#42756=CARTESIAN_POINT ( 'NONE',  ( -3.897244926436033374, 3.994152527635309729E-16, -13.96644127841335958 ) ) ;
#42760=DIRECTION ( 'NONE',  ( 0.000000000000000000, 0.000000000000000000, 1.000000000000000000 ) ) ;
#42768=FACE_OUTER_BOUND ( 'NONE', #26296, .T. ) ;
#42771=DIRECTION ( 'NONE',  ( -0.000000000000000000, 1.000000000000000000, -0.000000000000000000 ) ) ;
#42777=ORIENTED_EDGE ( 'NONE', *, *, #86726, .F. ) ;
#42780=CARTESIAN_POINT ( 'NONE',  ( -10.58521204051718101, -0.03417435944610275333, -11.99294302885424024 ) ) ;
#42781=CARTESIAN_POINT ( 'NONE',  ( -2.913501739333568707, 15.00000000000000000, -14.20427779279538960 ) ) ;
#42789=CARTESIAN_POINT ( 'NONE',  ( -11.35178980618963784, 0.3639309078821091892, -9.804941009312090117 ) ) ;
#42796=CARTESIAN_POINT ( 'NONE',  ( 8.564643372776625796, 0.3639308585234187210, -12.31449893000744211 ) ) ;
#42799=CARTESIAN_POINT ( 'NONE',  ( 10.64017930668198453, 0.5000000000000004441, 10.57291749337222875 ) ) ;
#42805=ADVANCED_FACE ( 'NONE', ( #32288 ), #48909, .T. ) ;
#42806=VERTEX_POINT ( 'NONE', #38832 ) ;
#42812=DIRECTION ( 'NONE',  ( 0.000000000000000000, 0.000000000000000000, 1.000000000000000000 ) ) ;
#42814=EDGE_CURVE ( 'NONE', #31058, #71952, #77299, .T. ) ;
#42826=CARTESIAN_POINT ( 'NONE',  ( 13.07751017357383994, 15.00000000000000000, -6.263284095430508458 ) ) ;
#42827=CARTESIAN_POINT ( 'NONE',  ( 4.792102989642838651, 15.00000000000000000, 15.26149223938176291 ) ) ;
#42828=VERTEX_POINT ( 'NONE', #69821 ) ;
#42831=CARTESIAN_POINT ( 'NONE',  ( -11.92686044187656513, 12.66212336850781206, 3.903127820947815962E-15 ) ) ;
#42839=ORIENTED_EDGE ( 'NONE', *, *, #89400, .T. ) ;
#42851=B_SPLINE_CURVE_WITH_KNOTS ( 'NONE', 3,
 ( #76025, #75532, #7556, #45025, #38045, #29521 ),
 .UNSPECIFIED., .F., .F.,
 ( 4, 2, 4 ),
 ( 3.409110551477859173E-05, 0.0004400426677366043172, 0.0008459942299584299885 ),
 .UNSPECIFIED. ) ;
#42855=EDGE_LOOP ( 'NONE', ( #43703, #62537, #37359, #45408, #82679, #66484 ) ) ;
#42864=CARTESIAN_POINT ( 'NONE',  ( -14.47650479471827722, 0.3639311865617156361, 3.928206833721935354 ) ) ;
#42866=VECTOR ( 'NONE', #22287, 1000.000000000000227 ) ;
#42874=CARTESIAN_POINT ( 'NONE',  ( -7.595945211628163385, 4.385640548506873962E-16, -12.35117874301652030 ) ) ;
#42877=CARTESIAN_POINT ( 'NONE',  ( 8.439016546559892973, 15.00000000000000000, -11.79122553964970876 ) ) ;
#42879=CARTESIAN_POINT ( 'NONE',  ( 7.595945211628331251, 3.826527677142797770E-16, -12.35117874301642082 ) ) ;
#42887=EDGE_LOOP ( 'NONE', ( #30509, #25929, #95062, #70627 ) ) ;
#42892=CARTESIAN_POINT ( 'NONE',  ( 0.000000000000000000, 15.00000000000000000, 0.000000000000000000 ) ) ;
#42894=CARTESIAN_POINT ( 'NONE',  ( 14.97687855664614176, 14.49999999999999112, 0.8325315005901842147 ) ) ;
#42895=ORIENTED_EDGE ( 'NONE', *, *, #18000, .T. ) ;
#42899=CARTESIAN_POINT ( 'NONE',  ( -8.235571585149871865, 7.296802177851538396, -8.235571585149866536 ) ) ;
#42902=CARTESIAN_POINT ( 'NONE',  ( -6.898461952320240620, 15.00000000000000000, -12.75387089053316636 ) ) ;
#42912=CARTESIAN_POINT ( 'NONE',  ( -1.236355250167479491, 14.95037107271117627, 14.70131747622448515 ) ) ;
#42936=EDGE_LOOP ( 'NONE', ( #95733, #41855, #78262, #97441 ) ) ;
#42940=CARTESIAN_POINT ( 'NONE',  ( -12.60589901313231564, 14.63606915354311155, 8.129656208641970139 ) ) ;
#42942=CIRCLE ( 'NONE', #17408, 14.49999999999999822 ) ;
#42947=B_SPLINE_CURVE_WITH_KNOTS ( 'NONE', 3,
 ( #28650, #90625, #90131, #59140, #21661, #82641 ),
 .UNSPECIFIED., .F., .F.,
 ( 4, 2, 4 ),
 ( 0.0002800392683747309061, 0.0006862448819834952689, 0.001092450495592259523 ),
 .UNSPECIFIED. ) ;
#42954=PLANE ( 'NONE',  #65753 ) ;
#42955=CARTESIAN_POINT ( 'NONE',  ( -14.17193700899788134, -0.03417435944610275333, -1.489530601564206247 ) ) ;
#42957=VERTEX_POINT ( 'NONE', #35239 ) ;
#42959=CARTESIAN_POINT ( 'NONE',  ( -12.81628187352647963, -26.08469866340290721, -3.434112377981046293 ) ) ;
#42969=DIRECTION ( 'NONE',  ( 0.5224985647159551272, 0.000000000000000000, -0.8526401643540884034 ) ) ;
#42972=DIRECTION ( 'NONE',  ( -0.9969173337331274087, 0.000000000000000000, -0.07845909572785238206 ) ) ;
#42983=CARTESIAN_POINT ( 'NONE',  ( -2.913501739333569152, 4.140530414402051497E-16, -14.20427779279538960 ) ) ;
#42986=VERTEX_POINT ( 'NONE', #97868 ) ;
#42987=DIRECTION ( 'NONE',  ( -0.1822355254921514123, 0.000000000000000000, 0.9832549075639538394 ) ) ;
#42990=DIRECTION ( 'NONE',  ( 0.5664062369248313855, 0.000000000000000000, -0.8241261886220165866 ) ) ;
#42997=DIRECTION ( 'NONE',  ( 0.000000000000000000, 1.000000000000000000, 0.000000000000000000 ) ) ;
#42998=VERTEX_POINT ( 'NONE', #29328 ) ;
#43005=VECTOR ( 'NONE', #68548, 1000.000000000000000 ) ;
#43006=FACE_OUTER_BOUND ( 'NONE', #17972, .T. ) ;
#43007=ADVANCED_FACE ( 'NONE', ( #98862 ), #91317, .F. ) ;
#43009=CARTESIAN_POINT ( 'NONE',  ( -10.36894250292378317, -27.57125116508602503, 10.36894250292379560 ) ) ;
#43013=CYLINDRICAL_SURFACE ( 'NONE', #82693, 15.00000000000000000 ) ;
#43014=EDGE_CURVE ( 'NONE', #65339, #19933, #47234, .T. ) ;
#43025=CARTESIAN_POINT ( 'NONE',  ( -7.964842623401179544, 17.43868534415483751, -7.964842623401174215 ) ) ;
#43034=DIRECTION ( 'NONE',  ( 0.000000000000000000, 1.000000000000000000, 0.000000000000000000 ) ) ;
#43041=CARTESIAN_POINT ( 'NONE',  ( 8.731067818237042033, 9.537123368507819166, 8.731067818237033151 ) ) ;
#43044=VERTEX_POINT ( 'NONE', #9800 ) ;
#43054=AXIS2_PLACEMENT_3D ( 'NONE', #53833, #37366, #84345 ) ;
#43065=CARTESIAN_POINT ( 'NONE',  ( 13.48086198287162141, -0.03417435944610275333, 8.610676897597548063 ) ) ;
#43070=DIRECTION ( 'NONE',  ( 0.000000000000000000, 0.000000000000000000, 1.000000000000000000 ) ) ;
#43071=CARTESIAN_POINT ( 'NONE',  ( 9.846743663894594434, 3.508931151000788340, -2.168404344971008868E-15 ) ) ;
#43073=ORIENTED_EDGE ( 'NONE', *, *, #51830, .T. ) ;
#43082=ORIENTED_EDGE ( 'NONE', *, *, #54749, .F. ) ;
#43085=ORIENTED_EDGE ( 'NONE', *, *, #53278, .T. ) ;
#43087=VERTEX_POINT ( 'NONE', #94267 ) ;
#43092=VECTOR ( 'NONE', #12825, 1000.000000000000000 ) ;
#43093=CARTESIAN_POINT ( 'NONE',  ( -6.382347221874564269, 14.49999999999999112, 13.57444820018227993 ) ) ;
#43094=VECTOR ( 'NONE', #78983, 1000.000000000000000 ) ;
#43095=CARTESIAN_POINT ( 'NONE',  ( 10.04755927614745481, 15.00000000000000533, 10.62803196998863697 ) ) ;
#43096=VERTEX_POINT ( 'NONE', #24325 ) ;
#43098=ORIENTED_EDGE ( 'NONE', *, *, #57228, .F. ) ;
#43100=CARTESIAN_POINT ( 'NONE',  ( 4.856044144387611894, -2.574980159653071059E-16, 13.79699902221164720 ) ) ;
#43103=CIRCLE ( 'NONE', #51099, 15.00000000000000000 ) ;
#43115=DIRECTION ( 'NONE',  ( 0.000000000000000000, 0.000000000000000000, 1.000000000000000000 ) ) ;
#43120=EDGE_CURVE ( 'NONE', #8841, #952, #8759, .T. ) ;
#43121=VERTEX_POINT ( 'NONE', #63761 ) ;
#43131=CARTESIAN_POINT ( 'NONE',  ( 9.422509992056141925, -19.01964798917849109, -5.440088680355554374 ) ) ;
#43135=LINE ( 'NONE', #28135, #53180 ) ;
#43144=FACE_OUTER_BOUND ( 'NONE', #68794, .T. ) ;
#43148=CIRCLE ( 'NONE', #89475, 14.49999999999999822 ) ;
#43150=ORIENTED_EDGE ( 'NONE', *, *, #47408, .T. ) ;
#43152=EDGE_CURVE ( 'NONE', #3873, #47878, #96120, .T. ) ;
#43153=DIRECTION ( 'NONE',  ( 0.000000000000000000, 1.000000000000000000, 0.000000000000000000 ) ) ;
#43168=ORIENTED_EDGE ( 'NONE', *, *, #52270, .F. ) ;
#43170=DIRECTION ( 'NONE',  ( 0.000000000000000000, 0.000000000000000000, 1.000000000000000000 ) ) ;
#43187=ORIENTED_EDGE ( 'NONE', *, *, #72783, .T. ) ;
#43188=ORIENTED_EDGE ( 'NONE', *, *, #51539, .T. ) ;
#43194=AXIS2_PLACEMENT_3D ( 'NONE', #14731, #22717, #82212 ) ;
#43196=CARTESIAN_POINT ( 'NONE',  ( -6.408140936763246032, 8.290301336597091009, -11.09922568453594316 ) ) ;
#43197=VERTEX_POINT ( 'NONE', #72735 ) ;
#43207=DIRECTION ( 'NONE',  ( 0.000000000000000000, 0.000000000000000000, 1.000000000000000000 ) ) ;
#43208=CARTESIAN_POINT ( 'NONE',  ( -3.192513988408218761, 15.00000000000000533, 14.27292421863748473 ) ) ;
#43209=DIRECTION ( 'NONE',  ( -0.000000000000000000, -1.000000000000000000, -0.000000000000000000 ) ) ;
#43210=FACE_OUTER_BOUND ( 'NONE', #29045, .T. ) ;
#43214=AXIS2_PLACEMENT_3D ( 'NONE', #46361, #76849, #76368 ) ;
#43219=CARTESIAN_POINT ( 'NONE',  ( -9.876730923139378504, 0.5000000000000004441, 11.28938378619056415 ) ) ;
#43226=EDGE_CURVE ( 'NONE', #27622, #45246, #74687, .T. ) ;
#43236=ORIENTED_EDGE ( 'NONE', *, *, #24390, .F. ) ;
#43241=DIRECTION ( 'NONE',  ( -0.02617694830787626811, 0.000000000000000000, 0.9996573249755572599 ) ) ;
#43248=CARTESIAN_POINT ( 'NONE',  ( -7.082119434687044190, 7.637082168247301794, 12.26659068614894998 ) ) ;
#43252=AXIS2_PLACEMENT_3D ( 'NONE', #68112, #27628, #36116 ) ;
#43253=CARTESIAN_POINT ( 'NONE',  ( -8.439016546559740206, 3.923478264313957572E-16, -11.79122553964984910 ) ) ;
#43261=DIRECTION ( 'NONE',  ( -0.008726535498374266009, 0.000000000000000000, 0.9999619230641713097 ) ) ;
#43275=CARTESIAN_POINT ( 'NONE',  ( -13.61464873478178284, 14.49999999999999112, 6.296136897217746942 ) ) ;
#43285=VERTEX_POINT ( 'NONE', #57740 ) ;
#43297=DIRECTION ( 'NONE',  ( -0.8338858220671696575, 0.000000000000000000, 0.5519369853120560387 ) ) ;
#43303=ORIENTED_EDGE ( 'NONE', *, *, #21978, .F. ) ;
#43305=ORIENTED_EDGE ( 'NONE', *, *, #23736, .T. ) ;
#43319=EDGE_CURVE ( 'NONE', #68457, #71952, #73436, .T. ) ;
#43321=CARTESIAN_POINT ( 'NONE',  ( 2.258855624577643439, 14.95037108984192997, -14.57926203528950637 ) ) ;
#43329=EDGE_LOOP ( 'NONE', ( #50725, #54381, #82282, #66982, #9946, #3748 ) ) ;
#43336=ORIENTED_EDGE ( 'NONE', *, *, #25222, .T. ) ;
#43337=CARTESIAN_POINT ( 'NONE',  ( -5.378451019861605786, 0.000000000000000000, 0.9000440264802068713 ) ) ;
#43340=CARTESIAN_POINT ( 'NONE',  ( 4.862001128006681050, 15.00000000000000000, 13.66056166602463229 ) ) ;
#43344=CARTESIAN_POINT ( 'NONE',  ( -14.42525372082714696, 0.2301507929055852109, 3.890283033989091255 ) ) ;
#43348=AXIS2_PLACEMENT_3D ( 'NONE', #80461, #36436, #28914 ) ;
#43349=CARTESIAN_POINT ( 'NONE',  ( 9.402796353261066997, 14.49999999999999112, 11.68706210897770070 ) ) ;
#43351=EDGE_CURVE ( 'NONE', #40063, #51377, #35737, .T. ) ;
#43356=ADVANCED_FACE ( 'NONE', ( #5745 ), #36235, .F. ) ;
#43357=CIRCLE ( 'NONE', #17823, 15.00000000000000000 ) ;
#43363=DIRECTION ( 'NONE',  ( 3.552713678800501560E-14, 0.000000000000000000, 1.000000000000000000 ) ) ;
#43370=LINE ( 'NONE', #43856, #84288 ) ;
#43373=ORIENTED_EDGE ( 'NONE', *, *, #89400, .F. ) ;
#43376=ADVANCED_FACE ( 'NONE', ( #6724 ), #7726, .F. ) ;
#43379=CARTESIAN_POINT ( 'NONE',  ( -11.25000000000000178, 7.713468844518206247, -3.014428414850123250 ) ) ;
#43383=B_SPLINE_CURVE_WITH_KNOTS ( 'NONE', 3,
 ( #30666, #61175, #92171, #38201, #7705, #38683 ),
 .UNSPECIFIED., .F., .F.,
 ( 4, 2, 4 ),
 ( 0.0002800056097769410175, 0.0006862108940652281337, 0.001092416178353515250 ),
 .UNSPECIFIED. ) ;
#43385=CARTESIAN_POINT ( 'NONE',  ( 0.000000000000000000, 0.5000000000000004441, 0.000000000000000000 ) ) ;
#43387=CARTESIAN_POINT ( 'NONE',  ( 0.000000000000000000, 14.49999999999999822, 0.000000000000000000 ) ) ;
#43389=CARTESIAN_POINT ( 'NONE',  ( 12.83294900548063744, 15.00000000000000000, -7.766300266068363101 ) ) ;
#43393=DIRECTION ( 'NONE',  ( 0.000000000000000000, 0.000000000000000000, 1.000000000000000000 ) ) ;
#43394=DIRECTION ( 'NONE',  ( 0.9588197348681928300, -0.000000000000000000, 0.2840153447039234780 ) ) ;
#43399=CYLINDRICAL_SURFACE ( 'NONE', #67490, 15.00000000000000000 ) ;
#43421=CARTESIAN_POINT ( 'NONE',  ( -13.40508947812159235, 3.877950237245923868E-16, -5.527528931046294502 ) ) ;
#43424=VERTEX_POINT ( 'NONE', #44217 ) ;
#43433=CARTESIAN_POINT ( 'NONE',  ( 8.564643372776551189, 14.49999999999999112, 12.31449893000752915 ) ) ;
#43437=CARTESIAN_POINT ( 'NONE',  ( 2.602060718268817574, 0.000000000000000000, 4.792399674598875947 ) ) ;
#43439=CARTESIAN_POINT ( 'NONE',  ( 3.434112377981054287, -12.33469866340291432, -12.81628187352647608 ) ) ;
#43465=ORIENTED_EDGE ( 'NONE', *, *, #4559, .T. ) ;
#43467=CARTESIAN_POINT ( 'NONE',  ( 2.621477372531582528, 15.00000000000000000, 15.77990027919563154 ) ) ;
#43468=EDGE_CURVE ( 'NONE', #40449, #38087, #82663, .T. ) ;
#43477=CARTESIAN_POINT ( 'NONE',  ( 11.35178980618967337, 0.5000000000000004441, 9.804941009311999522 ) ) ;
#43481=VERTEX_POINT ( 'NONE', #8212 ) ;
#43483=CARTESIAN_POINT ( 'NONE',  ( 5.419894505350582925, 0.5000000000000004441, -13.98659156302458761 ) ) ;
#43488=DIRECTION ( 'NONE',  ( 0.000000000000000000, 0.000000000000000000, 1.000000000000000000 ) ) ;
#43490=CARTESIAN_POINT ( 'NONE',  ( 10.36894250292379027, -21.32125116508603213, 10.36894250292378672 ) ) ;
#43508=CARTESIAN_POINT ( 'NONE',  ( 7.964842623401181321, 19.93868534415484106, 7.964842623401174215 ) ) ;
#43511=PLANE ( 'NONE',  #47201 ) ;
#43513=EDGE_CURVE ( 'NONE', #42986, #31058, #83215, .T. ) ;
#43551=CARTESIAN_POINT ( 'NONE',  ( 12.25993886608609351, 14.49999999999999112, -8.642563219313673883 ) ) ;
#43553=CARTESIAN_POINT ( 'NONE',  ( -4.923371831947292776, 21.84226448433413026, 8.527530157486181039 ) ) ;
#43554=ORIENTED_EDGE ( 'NONE', *, *, #65705, .F. ) ;
#43565=AXIS2_PLACEMENT_3D ( 'NONE', #49305, #96306, #58268 ) ;
#43570=AXIS2_PLACEMENT_3D ( 'NONE', #70437, #78912, #86903 ) ;
#43575=ORIENTED_EDGE ( 'NONE', *, *, #70369, .T. ) ;
#43579=VECTOR ( 'NONE', #73342, 1000.000000000000000 ) ;
#43580=ADVANCED_FACE ( 'NONE', ( #75213 ), #69900, .T. ) ;
#43581=DIRECTION ( 'NONE',  ( 0.9799247046208295897, 0.000000000000000000, -0.1993679344171971901 ) ) ;
#43583=CARTESIAN_POINT ( 'NONE',  ( -5.073789285385991832, 0.000000000000000000, 1.998618750576336867 ) ) ;
#43584=CARTESIAN_POINT ( 'NONE',  ( 10.19513985507827236, 14.63606907090794351, 11.00268709613227891 ) ) ;
#43585=VERTEX_POINT ( 'NONE', #22233 ) ;
#43591=ADVANCED_FACE ( 'NONE', ( #7225 ), #68230, .F. ) ;
#43592=VECTOR ( 'NONE', #11831, 1000.000000000000000 ) ;
#43594=ORIENTED_EDGE ( 'NONE', *, *, #52040, .F. ) ;
#43595=CARTESIAN_POINT ( 'NONE',  ( -11.36476366739559651, 12.94173722837749452, 2.760244389056020431 ) ) ;
#43600=VERTEX_POINT ( 'NONE', #45710 ) ;
#43601=DIRECTION ( 'NONE',  ( 0.000000000000000000, 1.000000000000000000, 0.000000000000000000 ) ) ;
#43603=DIRECTION ( 'NONE',  ( 0.6225146366376079765, 0.000000000000000000, 0.7826081568524232424 ) ) ;
#43607=FACE_OUTER_BOUND ( 'NONE', #4346, .T. ) ;
#43610=DIRECTION ( 'NONE',  ( 1.776356839400250465E-15, 0.000000000000000000, 1.000000000000000000 ) ) ;
#43611=AXIS2_PLACEMENT_3D ( 'NONE', #79872, #47892, #71406 ) ;
#43619=CARTESIAN_POINT ( 'NONE',  ( 11.48952521350015488, 15.00000000000000000, 8.845383562533813304 ) ) ;
#43625=CARTESIAN_POINT ( 'NONE',  ( 9.422509992056141925, -24.01964798917849109, -5.440088680355554374 ) ) ;
#43629=CARTESIAN_POINT ( 'NONE',  ( 10.84451454130498149, 15.00000000000000000, 9.625305416630897781 ) ) ;
#43631=EDGE_CURVE ( 'NONE', #84722, #21240, #98639, .T. ) ;
#43641=ORIENTED_EDGE ( 'NONE', *, *, #2869, .T. ) ;
#43644=EDGE_CURVE ( 'NONE', #42998, #55876, #47533, .T. ) ;
#43650=CARTESIAN_POINT ( 'NONE',  ( -14.24131928502211863, 0.000000000000000000, 0.4973178280104966764 ) ) ;
#43658=VERTEX_POINT ( 'NONE', #85676 ) ;
#43674=CARTESIAN_POINT ( 'NONE',  ( 8.527530157486175710, -31.07440218233254470, -4.923371831947298993 ) ) ;
#43675=ORIENTED_EDGE ( 'NONE', *, *, #80278, .F. ) ;
#43676=CARTESIAN_POINT ( 'NONE',  ( 13.61464873478166204, 0.3639308181217354443, 6.296136897217934347 ) ) ;
#43682=AXIS2_PLACEMENT_3D ( 'NONE', #38240, #83234, #97771 ) ;
#43683=DIRECTION ( 'NONE',  ( -0.000000000000000000, -1.000000000000000000, -0.000000000000000000 ) ) ;
#43688=CARTESIAN_POINT ( 'NONE',  ( 9.382169495545419124, 10.99863466993041783, 9.382169495545417348 ) ) ;
#43693=ORIENTED_EDGE ( 'NONE', *, *, #35087, .F. ) ;
#43703=ORIENTED_EDGE ( 'NONE', *, *, #67149, .T. ) ;
#43705=VECTOR ( 'NONE', #1276, 1000.000000000000000 ) ;
#43706=CARTESIAN_POINT ( 'NONE',  ( 14.24131928502211686, 15.00000000000000000, -0.4973178280105898241 ) ) ;
#43707=CARTESIAN_POINT ( 'NONE',  ( -9.402796353260967521, 0.3640475087720753677, -11.68706210897770426 ) ) ;
#43710=EDGE_CURVE ( 'NONE', #30649, #22949, #66172, .T. ) ;
#43716=CARTESIAN_POINT ( 'NONE',  ( -4.873787042390612001, 15.00000000000000000, -13.39061984619925916 ) ) ;
#43721=CARTESIAN_POINT ( 'NONE',  ( -1.829604203029787435, -0.03417435944610275333, 15.89119079541584334 ) ) ;
#43731=CARTESIAN_POINT ( 'NONE',  ( -11.25000000000000178, 5.118033628982653127, 3.674383000693412496E-15 ) ) ;
#43737=CARTESIAN_POINT ( 'NONE',  ( -2.913501739333854701, 4.099883984707052505E-16, 14.20427779279533098 ) ) ;
#43741=CARTESIAN_POINT ( 'NONE',  ( -7.082119434687044190, 2.637082168247310676, 12.26659068614894998 ) ) ;
#43750=ORIENTED_EDGE ( 'NONE', *, *, #66277, .T. ) ;
#43753=DIRECTION ( 'NONE',  ( -0.000000000000000000, -1.000000000000000000, -0.000000000000000000 ) ) ;
#43761=CARTESIAN_POINT ( 'NONE',  ( -14.42956166534410656, 14.99999999999807443, 2.386684097923415404 ) ) ;
#43773=ORIENTED_EDGE ( 'NONE', *, *, #75556, .T. ) ;
#43785=AXIS2_PLACEMENT_3D ( 'NONE', #49631, #4660, #59108 ) ;
#43787=ORIENTED_EDGE ( 'NONE', *, *, #63640, .T. ) ;
#43795=ORIENTED_EDGE ( 'NONE', *, *, #95894, .T. ) ;
#43798=FACE_OUTER_BOUND ( 'NONE', #76762, .T. ) ;
#43799=EDGE_CURVE ( 'NONE', #22448, #40720, #18562, .T. ) ;
#43804=ORIENTED_EDGE ( 'NONE', *, *, #60392, .F. ) ;
#43808=PLANE ( 'NONE',  #17893 ) ;
#43814=CIRCLE ( 'NONE', #82142, 15.00000000000000000 ) ;
#43826=CARTESIAN_POINT ( 'NONE',  ( 10.58171042697168929, 0.2301503269722701694, 10.54749450092408658 ) ) ;
#43830=PLANE ( 'NONE',  #37590 ) ;
#43835=CARTESIAN_POINT ( 'NONE',  ( 9.281709892946398810, 15.00000000000000178, 11.30302492080712540 ) ) ;
#43843=CARTESIAN_POINT ( 'NONE',  ( 0.000000000000000000, 15.00000000000000000, 0.000000000000000000 ) ) ;
#43844=CIRCLE ( 'NONE', #792, 15.00000000000000000 ) ;
#43846=DIRECTION ( 'NONE',  ( 0.000000000000000000, 1.000000000000000000, 0.000000000000000000 ) ) ;
#43850=DIRECTION ( 'NONE',  ( -0.000000000000000000, 1.000000000000000000, 0.000000000000000000 ) ) ;
#43856=CARTESIAN_POINT ( 'NONE',  ( -3.836325488036278930, 15.00000000000000000, 14.50112432709419785 ) ) ;
#43858=CARTESIAN_POINT ( 'NONE',  ( 14.99847009497948669, 14.63606908182952715, -0.2142307401080164042 ) ) ;
#43883=LINE ( 'NONE', #74379, #66677 ) ;
#43887=EDGE_CURVE ( 'NONE', #13064, #73542, #41178, .T. ) ;
#43895=ORIENTED_EDGE ( 'NONE', *, *, #77030, .F. ) ;
#43899=CARTESIAN_POINT ( 'NONE',  ( 11.62719953690058361, 15.00000000000000000, 9.476720473301874392 ) ) ;
#43904=VECTOR ( 'NONE', #22294, 1000.000000000000000 ) ;
#43908=DIRECTION ( 'NONE',  ( -0.1650476058606810681, 0.000000000000000000, 0.9862856015372308827 ) ) ;
#43909=EDGE_LOOP ( 'NONE', ( #49883, #38255, #27330, #55749 ) ) ;
#43918=CARTESIAN_POINT ( 'NONE',  ( 0.000000000000000000, 0.5000000000000004441, 0.000000000000000000 ) ) ;
#43921=DIRECTION ( 'NONE',  ( -0.6494480483301851015, 0.000000000000000000, 0.7604059656000297096 ) ) ;
#43924=ORIENTED_EDGE ( 'NONE', *, *, #62672, .T. ) ;
#43926=CARTESIAN_POINT ( 'NONE',  ( 11.09922568453595026, -23.79303199673624292, 6.408140936763232709 ) ) ;
#43936=CYLINDRICAL_SURFACE ( 'NONE', #81794, 15.00000000000000000 ) ;
#43942=ORIENTED_EDGE ( 'NONE', *, *, #51950, .T. ) ;
#43949=CARTESIAN_POINT ( 'NONE',  ( 14.29730467489529389, 15.00000000000000000, 2.416004766803322656 ) ) ;
#43954=ORIENTED_EDGE ( 'NONE', *, *, #47299, .F. ) ;
#43960=CARTESIAN_POINT ( 'NONE',  ( 12.98685442714194949, 4.417933709739653524E-16, 6.449155920601044478 ) ) ;
#43967=CARTESIAN_POINT ( 'NONE',  ( 14.88232117145530431, 0.3640475087720976277, 1.875237731503244243 ) ) ;
#43968=AXIS2_PLACEMENT_3D ( 'NONE', #4025, #5501, #35974 ) ;
#43979=CARTESIAN_POINT ( 'NONE',  ( 7.082119434687054849, -16.52958449841936073, 12.26659068614894288 ) ) ;
#43985=VERTEX_POINT ( 'NONE', #66106 ) ;
#43992=DIRECTION ( 'NONE',  ( 0.000000000000000000, 0.000000000000000000, -1.000000000000000000 ) ) ;
#43994=CARTESIAN_POINT ( 'NONE',  ( 12.60589901313216110, 15.00000000000000000, 8.129656208642140669 ) ) ;
#43996=CARTESIAN_POINT ( 'NONE',  ( -5.440088680355558814, 27.23035201082150891, -9.422509992056136596 ) ) ;
#44002=ADVANCED_FACE ( 'NONE', ( #4153 ), #95636, .F. ) ;
#44012=CARTESIAN_POINT ( 'NONE',  ( 3.195792623639471142, 11.20379003517448346, -11.92686044187660066 ) ) ;
#44015=VERTEX_POINT ( 'NONE', #50124 ) ;
#44025=DIRECTION ( 'NONE',  ( 0.000000000000000000, 1.000000000000000000, 0.000000000000000000 ) ) ;
#44036=VECTOR ( 'NONE', #2376, 1000.000000000000114 ) ;
#44044=CARTESIAN_POINT ( 'NONE',  ( 4.746257547686181688, 0.000000000000000000, 2.685303318749109547 ) ) ;
#44047=CARTESIAN_POINT ( 'NONE',  ( 7.208316651077764980, 12.88393115100078390, 7.208316651077762316 ) ) ;
#44048=ORIENTED_EDGE ( 'NONE', *, *, #66946, .F. ) ;
#44049=ORIENTED_EDGE ( 'NONE', *, *, #97728, .F. ) ;
#44051=VERTEX_POINT ( 'NONE', #33630 ) ;
#44057=CIRCLE ( 'NONE', #39300, 14.49999999999999822 ) ;
#44062=B_SPLINE_CURVE_WITH_KNOTS ( 'NONE', 3,
 ( #21282, #59760, #90254, #37284, #90753, #67774 ),
 .UNSPECIFIED., .F., .F.,
 ( 4, 2, 4 ),
 ( 0.0002800003243993108831, 0.0006862055569927221887, 0.001092410789586133494 ),
 .UNSPECIFIED. ) ;
#44064=ORIENTED_EDGE ( 'NONE', *, *, #52783, .T. ) ;
#44070=DIRECTION ( 'NONE',  ( -0.8703556959399010307, 0.000000000000000000, 0.4924235601034648302 ) ) ;
#44073=EDGE_LOOP ( 'NONE', ( #8073, #78541, #59896, #66811 ) ) ;
#44076=CARTESIAN_POINT ( 'NONE',  ( 14.04391541078762984, 15.00000000000000000, -3.608107528142820986 ) ) ;
#44078=DIRECTION ( 'NONE',  ( -0.6626200482157408311, 0.000000000000000000, 0.7489557207889990798 ) ) ;
#44080=DIRECTION ( 'NONE',  ( 2.309263891220325920E-14, 0.000000000000000000, 1.000000000000000000 ) ) ;
#44082=CARTESIAN_POINT ( 'NONE',  ( 0.000000000000000000, 14.49999999999999822, 0.000000000000000000 ) ) ;
#44083=VERTEX_POINT ( 'NONE', #35622 ) ;
#44084=CARTESIAN_POINT ( 'NONE',  ( -10.32896413005680536, 4.271642702460845875, -5.963430220938272797 ) ) ;
#44087=AXIS2_PLACEMENT_3D ( 'NONE', #84606, #48556, #85589 ) ;
#44093=DIRECTION ( 'NONE',  ( 0.1132032137679039180, -0.000000000000000000, 0.9935718556765877896 ) ) ;
#44103=CARTESIAN_POINT ( 'NONE',  ( 13.30119215211372641, 14.76984893004598476, 6.804450086558370359 ) ) ;
#44107=CARTESIAN_POINT ( 'NONE',  ( 3.469446951953614189E-15, -10.68631465584515894, 10.88017736071110342 ) ) ;
#44110=DIRECTION ( 'NONE',  ( -0.000000000000000000, -1.000000000000000000, -0.000000000000000000 ) ) ;
#44114=VECTOR ( 'NONE', #11769, 1000.000000000000000 ) ;
#44116=CIRCLE ( 'NONE', #68062, 14.49999999999999822 ) ;
#44132=CARTESIAN_POINT ( 'NONE',  ( 3.927832320392154575, -0.03417435944610275333, 13.69797916712106733 ) ) ;
#44134=DIRECTION ( 'NONE',  ( 0.000000000000000000, 0.000000000000000000, 1.000000000000000000 ) ) ;
#44136=VECTOR ( 'NONE', #7228, 1000.000000000000000 ) ;
#44137=ORIENTED_EDGE ( 'NONE', *, *, #74390, .F. ) ;
#44138=CARTESIAN_POINT ( 'NONE',  ( -14.82269085861167035, 14.63595249122789177, -2.299529454047154697 ) ) ;
#44142=ORIENTED_EDGE ( 'NONE', *, *, #97816, .F. ) ;
#44160=CARTESIAN_POINT ( 'NONE',  ( 4.923371831947301658, -17.32440218233254470, 8.527530157486175710 ) ) ;
#44164=B_SPLINE_CURVE_WITH_KNOTS ( 'NONE', 3,
 ( #9176, #39694, #77175, #10169, #16195, #23713 ),
 .UNSPECIFIED., .F., .F.,
 ( 4, 2, 4 ),
 ( 3.409110551496062250E-05, 0.0004400426677367845658, 0.0008459942299586084482 ),
 .UNSPECIFIED. ) ;
#44165=ORIENTED_EDGE ( 'NONE', *, *, #49690, .F. ) ;
#44166=VECTOR ( 'NONE', #28160, 999.9999999999998863 ) ;
#44167=LINE ( 'NONE', #52663, #37727 ) ;
#44172=DIRECTION ( 'NONE',  ( 0.000000000000000000, 0.000000000000000000, -1.000000000000000000 ) ) ;
#44175=CARTESIAN_POINT ( 'NONE',  ( 11.09922568453594671, 27.04030133659709989, -6.408140936763241591 ) ) ;
#44178=VERTEX_POINT ( 'NONE', #26156 ) ;
#44182=ADVANCED_FACE ( 'NONE', ( #56650 ), #33125, .T. ) ;
#44186=PLANE ( 'NONE',  #84714 ) ;
#44189=EDGE_CURVE ( 'NONE', #2722, #19871, #34125, .T. ) ;
#44191=DIRECTION ( 'NONE',  ( -0.000000000000000000, -1.000000000000000000, -0.000000000000000000 ) ) ;
#44192=CARTESIAN_POINT ( 'NONE',  ( -14.88232117145532385, 15.00000000000000000, 1.875237731503040628 ) ) ;
#44194=AXIS2_PLACEMENT_3D ( 'NONE', #39191, #22223, #14726 ) ;
#44199=ADVANCED_FACE ( 'NONE', ( #57134 ), #19144, .F. ) ;
#44200=VERTEX_POINT ( 'NONE', #52592 ) ;
#44202=CARTESIAN_POINT ( 'NONE',  ( -14.35840480524203144, 0.5000000000000004441, 4.340070442838751319 ) ) ;
#44206=CARTESIAN_POINT ( 'NONE',  ( -4.180366052181437198, 14.99999999999798206, 14.01545757926889557 ) ) ;
#44210=CYLINDRICAL_SURFACE ( 'NONE', #40797, 15.00000000000000000 ) ;
#44215=CIRCLE ( 'NONE', #71371, 14.49999999999999822 ) ;
#44217=CARTESIAN_POINT ( 'NONE',  ( -13.07751017357372447, 15.00000000000000000, -6.263284095430686094 ) ) ;
#44220=CARTESIAN_POINT ( 'NONE',  ( -9.705452947461587598, 2.500000000000008438, -5.689172442861014645 ) ) ;
#44226=CARTESIAN_POINT ( 'NONE',  ( -13.78891971893212443, 0.5000000000000004441, 5.904717858191433244 ) ) ;
#44232=CARTESIAN_POINT ( 'NONE',  ( 3.795296366450314540, 23.26208216824728936, 14.16423886937410082 ) ) ;
#44234=CIRCLE ( 'NONE', #1165, 14.49999999999999822 ) ;
#44238=EDGE_CURVE ( 'NONE', #61056, #77111, #60587, .T. ) ;
#44249=AXIS2_PLACEMENT_3D ( 'NONE', #62334, #69862, #887 ) ;
#44267=TOROIDAL_SURFACE ( 'NONE', #57041, 14.49999999999999822, 0.5000000000000000000 ) ;
#44268=ORIENTED_EDGE ( 'NONE', *, *, #62519, .T. ) ;
#44270=FACE_OUTER_BOUND ( 'NONE', #27668, .T. ) ;
#44271=EDGE_CURVE ( 'NONE', #42121, #94488, #45146, .T. ) ;
#44278=CARTESIAN_POINT ( 'NONE',  ( 0.000000000000000000, 15.00000000000000000, 0.000000000000000000 ) ) ;
#44284=EDGE_CURVE ( 'NONE', #1757, #32864, #18035, .T. ) ;
#44288=ORIENTED_EDGE ( 'NONE', *, *, #8687, .T. ) ;
#44295=ORIENTED_EDGE ( 'NONE', *, *, #75311, .F. ) ;
#44303=EDGE_LOOP ( 'NONE', ( #96615, #85731, #12318, #86459, #44926, #90014 ) ) ;
#44305=CARTESIAN_POINT ( 'NONE',  ( 2.120353041430647068, 15.00000000000000000, -14.34413130794945523 ) ) ;
#44321=DIRECTION ( 'NONE',  ( 8.659560562354946417E-17, 0.7071067811865465735, -0.7071067811865485719 ) ) ;
#44340=EDGE_CURVE ( 'NONE', #91116, #75439, #83596, .T. ) ;
#44346=AXIS2_PLACEMENT_3D ( 'NONE', #87695, #50695, #65185 ) ;
#44352=AXIS2_PLACEMENT_3D ( 'NONE', #96899, #81859, #51870 ) ;
#44357=CARTESIAN_POINT ( 'NONE',  ( 3.195792623639526653, 3.229976035794172695, -11.92686044187656336 ) ) ;
#44358=AXIS2_PLACEMENT_3D ( 'NONE', #62602, #17629, #38646 ) ;
#44368=FACE_OUTER_BOUND ( 'NONE', #9278, .T. ) ;
#44369=CARTESIAN_POINT ( 'NONE',  ( -2.258855624577434718, 0.04962891015807079781, -14.57926203528953657 ) ) ;
#44382=DIRECTION ( 'NONE',  ( -0.000000000000000000, 1.000000000000000000, -0.000000000000000000 ) ) ;
#44387=DIRECTION ( 'NONE',  ( -0.000000000000000000, -1.000000000000000000, -0.000000000000000000 ) ) ;
#44388=DIRECTION ( 'NONE',  ( 0.000000000000000000, 0.000000000000000000, 1.000000000000000000 ) ) ;
#44400=EDGE_CURVE ( 'NONE', #24676, #87709, #90077, .T. ) ;
#44411=ORIENTED_EDGE ( 'NONE', *, *, #74873, .F. ) ;
#44418=PLANE ( 'NONE',  #83331 ) ;
#44422=ORIENTED_EDGE ( 'NONE', *, *, #55341, .T. ) ;
#44424=CARTESIAN_POINT ( 'NONE',  ( 6.408140936763243367, -24.20969866340290721, 11.09922568453594494 ) ) ;
#44435=AXIS2_PLACEMENT_3D ( 'NONE', #29526, #74546, #28057 ) ;
#44443=VERTEX_POINT ( 'NONE', #24583 ) ;
#44449=CARTESIAN_POINT ( 'NONE',  ( -8.375939845167836850, 0.000000000000000000, 11.52849216984293257 ) ) ;
#44462=CARTESIAN_POINT ( 'NONE',  ( -14.52844422123122747, -2.748198397366576661E-15, 1.683098224408205557 ) ) ;
#44469=CARTESIAN_POINT ( 'NONE',  ( 14.64885433385999214, 0.04922511925147109862, 1.748475581354309583 ) ) ;
#44471=VERTEX_POINT ( 'NONE', #17074 ) ;
#44480=CARTESIAN_POINT ( 'NONE',  ( 10.36894250292378850, -15.07125116508603213, -10.36894250292379027 ) ) ;
#44481=CIRCLE ( 'NONE', #84402, 15.00000000000000000 ) ;
#44486=ORIENTED_EDGE ( 'NONE', *, *, #64388, .T. ) ;
#44490=CARTESIAN_POINT ( 'NONE',  ( 3.420591144908583736, 14.49999999999999112, -14.60477854057961800 ) ) ;
#44493=CARTESIAN_POINT ( 'NONE',  ( -0.8060400322138528972, 0.000000000000000000, -5.393339789881751223 ) ) ;
#44497=CARTESIAN_POINT ( 'NONE',  ( 5.440088680355556150, 24.73035201082151957, 9.422509992056138373 ) ) ;
#44502=CARTESIAN_POINT ( 'NONE',  ( -14.76100041229773296, 0.2306972965111885321, 2.313205896730730071 ) ) ;
#44517=DIRECTION ( 'NONE',  ( 0.2164396139381103701, 0.000000000000000000, -0.9762960071199316969 ) ) ;
#44528=CARTESIAN_POINT ( 'NONE',  ( 6.189940676892116578, 14.95037117674007021, -13.39186120659003265 ) ) ;
#44534=ORIENTED_EDGE ( 'NONE', *, *, #6237, .T. ) ;
#44539=CARTESIAN_POINT ( 'NONE',  ( -4.431036607602381494, 14.63595249122789177, -14.33059365769917726 ) ) ;
#44548=CARTESIAN_POINT ( 'NONE',  ( -4.923371831947292776, 16.84226448433412315, 8.527530157486181039 ) ) ;
#44550=ORIENTED_EDGE ( 'NONE', *, *, #28799, .T. ) ;
#44552=VERTEX_POINT ( 'NONE', #10060 ) ;
#44566=ORIENTED_EDGE ( 'NONE', *, *, #12569, .T. ) ;
#44569=VECTOR ( 'NONE', #27162, 1000.000000000000000 ) ;
#44575=ADVANCED_FACE ( 'NONE', ( #32546 ), #31558, .F. ) ;
#44578=ORIENTED_EDGE ( 'NONE', *, *, #92796, .T. ) ;
#44579=DIRECTION ( 'NONE',  ( 0.000000000000000000, 0.000000000000000000, 1.000000000000000000 ) ) ;
#44580=LINE ( 'NONE', #607, #1446 ) ;
#44585=CARTESIAN_POINT ( 'NONE',  ( 0.000000000000000000, 0.5000000000000004441, 0.000000000000000000 ) ) ;
#44588=ORIENTED_EDGE ( 'NONE', *, *, #7044, .T. ) ;
#44592=CARTESIAN_POINT ( 'NONE',  ( -13.07734668325347016, 15.00000000000000711, 6.551438809692819554 ) ) ;
#44600=EDGE_CURVE ( 'NONE', #39231, #70759, #48284, .T. ) ;
#44611=CARTESIAN_POINT ( 'NONE',  ( 13.34343830728403724, 14.49999999999999112, 6.852200678592740068 ) ) ;
#44616=CARTESIAN_POINT ( 'NONE',  ( 7.964842623401181321, -15.06131465584516071, 7.964842623401174215 ) ) ;
#44620=DIRECTION ( 'NONE',  ( 0.8433914458128849434, -0.000000000000000000, 0.5372996083468249973 ) ) ;
#44622=FACE_OUTER_BOUND ( 'NONE', #51095, .T. ) ;
#44635=ADVANCED_FACE ( 'NONE', ( #69087 ), #85684, .T. ) ;
#44642=LINE ( 'NONE', #52633, #80984 ) ;
#44648=ORIENTED_EDGE ( 'NONE', *, *, #50981, .T. ) ;
#44663=CARTESIAN_POINT ( 'NONE',  ( 2.638427012816835227, -22.53273551566587685, 9.846743663894590881 ) ) ;
#44665=DIRECTION ( 'NONE',  ( -0.9681476403781067441, 0.000000000000000000, -0.2503800040544454375 ) ) ;
#44666=ORIENTED_EDGE ( 'NONE', *, *, #38242, .F. ) ;
#44668=VECTOR ( 'NONE', #65327, 1000.000000000000000 ) ;
#44678=CARTESIAN_POINT ( 'NONE',  ( 11.09922568453595026, 16.20696800326376064, 6.408140936763232709 ) ) ;
#44679=ORIENTED_EDGE ( 'NONE', *, *, #39686, .F. ) ;
#44682=VERTEX_POINT ( 'NONE', #34012 ) ;
#44691=ADVANCED_FACE ( 'NONE', ( #72508 ), #71772, .F. ) ;
#44694=DIRECTION ( 'NONE',  ( -0.7253743710122820820, 0.000000000000000000, -0.6883545756937599069 ) ) ;
#44695=CARTESIAN_POINT ( 'NONE',  ( -0.7166339456633684657, -0.03417435944610275333, 15.98010739087745868 ) ) ;
#44714=CARTESIAN_POINT ( 'NONE',  ( -5.279540384298797129, 0.000000000000000000, 1.365381980696670716 ) ) ;
#44715=EDGE_CURVE ( 'NONE', #9889, #41155, #51511, .T. ) ;
#44717=ORIENTED_EDGE ( 'NONE', *, *, #47408, .F. ) ;
#44718=EDGE_CURVE ( 'NONE', #38990, #71871, #54455, .T. ) ;
#44719=LINE ( 'NONE', #1225, #90464 ) ;
#44723=CARTESIAN_POINT ( 'NONE',  ( 10.58981376305288613, 15.00000000000000000, -9.535111140613709679 ) ) ;
#44727=CARTESIAN_POINT ( 'NONE',  ( 0.000000000000000000, 15.00000000000000000, 0.000000000000000000 ) ) ;
#44730=CARTESIAN_POINT ( 'NONE',  ( -1.780824192092587577, 14.49999999999999112, 14.89391369643518637 ) ) ;
#44731=CARTESIAN_POINT ( 'NONE',  ( -5.204170427930421283E-15, 20.55374883491398208, -14.16423886937410082 ) ) ;
#44742=DIRECTION ( 'NONE',  ( 0.000000000000000000, 0.000000000000000000, 1.000000000000000000 ) ) ;
#44746=ORIENTED_EDGE ( 'NONE', *, *, #4039, .T. ) ;
#44749=CARTESIAN_POINT ( 'NONE',  ( 0.000000000000000000, 14.49999999999999822, 0.000000000000000000 ) ) ;
#44754=EDGE_CURVE ( 'NONE', #85704, #17506, #8477, .T. ) ;
#44758=DIRECTION ( 'NONE',  ( -0.000000000000000000, -1.000000000000000000, -0.000000000000000000 ) ) ;
#44764=LINE ( 'NONE', #60752, #12527 ) ;
#44777=VERTEX_POINT ( 'NONE', #53972 ) ;
#44779=EDGE_LOOP ( 'NONE', ( #92267, #3002, #14350, #36649 ) ) ;
#44787=AXIS2_PLACEMENT_3D ( 'NONE', #34169, #2739, #11687 ) ;
#44790=VECTOR ( 'NONE', #57413, 1000.000000000000000 ) ;
#44795=CARTESIAN_POINT ( 'NONE',  ( 13.96521320569122437, 0.04922511925147349254, 4.755935267939266353 ) ) ;
#44799=CIRCLE ( 'NONE', #35010, 14.49999999999999822 ) ;
#44805=DIRECTION ( 'NONE',  ( -0.000000000000000000, 1.000000000000000000, -0.000000000000000000 ) ) ;
#44824=EDGE_CURVE ( 'NONE', #3422, #44200, #25470, .T. ) ;
#44839=VERTEX_POINT ( 'NONE', #15982 ) ;
#44840=ORIENTED_EDGE ( 'NONE', *, *, #57607, .F. ) ;
#44841=CARTESIAN_POINT ( 'NONE',  ( 0.3093388210927633941, 14.49999999999999822, 14.99680997725065978 ) ) ;
#44843=CARTESIAN_POINT ( 'NONE',  ( 5.963430220938279902, 3.021642702460851204, -10.32896413005680181 ) ) ;
#44849=ORIENTED_EDGE ( 'NONE', *, *, #24772, .T. ) ;
#44853=DIRECTION ( 'NONE',  ( 0.000000000000000000, 1.000000000000000000, 0.000000000000000000 ) ) ;
#44863=CARTESIAN_POINT ( 'NONE',  ( -11.10136736363520527, 14.95077488074852745, -9.716261771425058313 ) ) ;
#44867=CARTESIAN_POINT ( 'NONE',  ( -13.14228782657345462, 0.3640475087720987379, 7.230509711182144805 ) ) ;
#44872=CARTESIAN_POINT ( 'NONE',  ( -2.827051895225887179, 0.2301501044984908817, 14.67071941139710312 ) ) ;
#44873=CARTESIAN_POINT ( 'NONE',  ( -3.420591144908390113, 14.49999999999999112, -14.60477854057966063 ) ) ;
#44884=CARTESIAN_POINT ( 'NONE',  ( 0.000000000000000000, 15.00000000000000000, 0.000000000000000000 ) ) ;
#44893=AXIS2_PLACEMENT_3D ( 'NONE', #86909, #25448, #85939 ) ;
#44909=DIRECTION ( 'NONE',  ( -0.000000000000000000, -1.000000000000000000, -0.000000000000000000 ) ) ;
#44911=ORIENTED_EDGE ( 'NONE', *, *, #19140, .F. ) ;
#44913=CARTESIAN_POINT ( 'NONE',  ( -9.382169495545413795, -20.25136533006958217, 9.382169495545428006 ) ) ;
#44917=CARTESIAN_POINT ( 'NONE',  ( 3.166711953933263768, 0.000000000000000000, -4.439566422914428045 ) ) ;
#44922=ADVANCED_FACE ( 'NONE', ( #47936 ), #94248, .T. ) ;
#44926=ORIENTED_EDGE ( 'NONE', *, *, #11446, .T. ) ;
#44931=CARTESIAN_POINT ( 'NONE',  ( 0.4278561937608483801, 0.000000000000000000, -5.436428395565743088 ) ) ;
#44936=ADVANCED_FACE ( 'NONE', ( #46469 ), #32007, .T. ) ;
#44939=CARTESIAN_POINT ( 'NONE',  ( 14.82269085861167568, 14.63595249122790598, 2.299529454047060550 ) ) ;
#44942=LINE ( 'NONE', #7466, #10010 ) ;
#44947=DIRECTION ( 'NONE',  ( -0.000000000000000000, -1.000000000000000000, -0.000000000000000000 ) ) ;
#44955=B_SPLINE_CURVE_WITH_KNOTS ( 'NONE', 3,
 ( #81344, #80364, #72845, #43826, #5365, #35844 ),
 .UNSPECIFIED., .F., .F.,
 ( 4, 2, 4 ),
 ( 0.0002800206007755490657, 0.0006862260317144062332, 0.001092431462653263401 ),
 .UNSPECIFIED. ) ;
#44971=CARTESIAN_POINT ( 'NONE',  ( 10.36894250292379027, -26.32125116508603568, 10.36894250292378672 ) ) ;
#44976=ORIENTED_EDGE ( 'NONE', *, *, #52091, .F. ) ;
#44981=DIRECTION ( 'NONE',  ( 0.000000000000000000, 1.000000000000000000, 0.000000000000000000 ) ) ;
#44983=DIRECTION ( 'NONE',  ( 0.000000000000000000, 1.000000000000000000, 0.000000000000000000 ) ) ;
#44985=CARTESIAN_POINT ( 'NONE',  ( 5.440088680355556150, 29.73035201082152668, 9.422509992056138373 ) ) ;
#44990=LINE ( 'NONE', #31462, #74314 ) ;
#44991=ORIENTED_EDGE ( 'NONE', *, *, #32163, .T. ) ;
#44995=LINE ( 'NONE', #52499, #14623 ) ;
#45002=DIRECTION ( 'NONE',  ( 0.000000000000000000, 1.000000000000000000, 0.000000000000000000 ) ) ;
#45020=ORIENTED_EDGE ( 'NONE', *, *, #48004, .T. ) ;
#45025=CARTESIAN_POINT ( 'NONE',  ( 2.258648100792295832, 0.04922511925147383949, -14.57890972981273769 ) ) ;
#45032=CARTESIAN_POINT ( 'NONE',  ( 0.000000000000000000, 14.49999999999999822, 0.000000000000000000 ) ) ;
#45033=CARTESIAN_POINT ( 'NONE',  ( -9.846743663894596210, 20.80059781766745175, -2.638427012816824124 ) ) ;
#45034=ORIENTED_EDGE ( 'NONE', *, *, #70557, .F. ) ;
#45037=EDGE_CURVE ( 'NONE', #33071, #41488, #69731, .T. ) ;
#45046=EDGE_CURVE ( 'NONE', #15789, #70022, #42274, .T. ) ;
#45048=EDGE_CURVE ( 'NONE', #38087, #40514, #41245, .T. ) ;
#45052=ORIENTED_EDGE ( 'NONE', *, *, #25575, .F. ) ;
#45054=VERTEX_POINT ( 'NONE', #94426 ) ;
#45060=EDGE_CURVE ( 'NONE', #69579, #40063, #10447, .T. ) ;
#45064=AXIS2_PLACEMENT_3D ( 'NONE', #27716, #20724, #51214 ) ;
#45065=ORIENTED_EDGE ( 'NONE', *, *, #20687, .T. ) ;
#45067=VERTEX_POINT ( 'NONE', #41944 ) ;
#45068=CARTESIAN_POINT ( 'NONE',  ( 2.621477372531582528, -0.03417435944610275333, 15.77990027919563154 ) ) ;
#45072=ADVANCED_FACE ( 'NONE', ( #25941 ), #35399, .T. ) ;
#45075=EDGE_LOOP ( 'NONE', ( #37813, #25264, #43168, #39994 ) ) ;
#45076=FACE_OUTER_BOUND ( 'NONE', #56618, .T. ) ;
#45080=ORIENTED_EDGE ( 'NONE', *, *, #59954, .F. ) ;
#45088=EDGE_CURVE ( 'NONE', #92052, #2779, #2989, .T. ) ;
#45089=CARTESIAN_POINT ( 'NONE',  ( 5.418184704451244116, 0.000000000000000000, -0.6173241701923083413 ) ) ;
#45090=ORIENTED_EDGE ( 'NONE', *, *, #28363, .T. ) ;
#45097=DIRECTION ( 'NONE',  ( -0.000000000000000000, -1.000000000000000000, -0.000000000000000000 ) ) ;
#45098=TOROIDAL_SURFACE ( 'NONE', #2034, 14.49999999999999822, 0.5000000000000000000 ) ;
#45101=CARTESIAN_POINT ( 'NONE',  ( 2.915334737309921209, -13.39464798917849109, -10.88017736071110164 ) ) ;
#45106=FACE_OUTER_BOUND ( 'NONE', #13185, .T. ) ;
#45109=TOROIDAL_SURFACE ( 'NONE', #13135, 14.49999999999999822, 0.5000000000000000000 ) ;
#45117=EDGE_LOOP ( 'NONE', ( #10630, #13574, #91200, #68446 ) ) ;
#45119=CARTESIAN_POINT ( 'NONE',  ( 14.47650479471827722, 14.49999999999999112, -3.928206833722049929 ) ) ;
#45132=CARTESIAN_POINT ( 'NONE',  ( -14.82269085861172364, 14.49999999999999112, -2.299529454047143595 ) ) ;
#45134=EDGE_LOOP ( 'NONE', ( #35077, #39386, #29470, #74189 ) ) ;
#45135=ORIENTED_EDGE ( 'NONE', *, *, #3915, .F. ) ;
#45146=CIRCLE ( 'NONE', #96261, 15.00000000000000000 ) ;
#45151=CIRCLE ( 'NONE', #35586, 14.49999999999999822 ) ;
#45152=CARTESIAN_POINT ( 'NONE',  ( 3.469446951953614189E-15, -27.74106884899921255, 9.846743663894594434 ) ) ;
#45155=VECTOR ( 'NONE', #22379, 1000.000000000000114 ) ;
#45156=VERTEX_POINT ( 'NONE', #19910 ) ;
#45169=CARTESIAN_POINT ( 'NONE',  ( 12.81628187352647252, 16.83196800326375708, -3.434112377981059172 ) ) ;
#45173=ORIENTED_EDGE ( 'NONE', *, *, #71254, .T. ) ;
#45175=ORIENTED_EDGE ( 'NONE', *, *, #63242, .F. ) ;
#45176=VECTOR ( 'NONE', #84479, 1000.000000000000114 ) ;
#45187=CARTESIAN_POINT ( 'NONE',  ( 7.264948169187460003, 0.2306972965111908080, -13.05597881399718929 ) ) ;
#45188=VERTEX_POINT ( 'NONE', #80911 ) ;
#45189=CIRCLE ( 'NONE', #49970, 15.00000000000000000 ) ;
#45190=CARTESIAN_POINT ( 'NONE',  ( -3.384479038598405154, 14.76984929998922347, 14.55223509985375863 ) ) ;
#45191=CARTESIAN_POINT ( 'NONE',  ( 1.087200977609890096, 0.000000000000000000, 5.343763529286935210 ) ) ;
#45193=ORIENTED_EDGE ( 'NONE', *, *, #80725, .T. ) ;
#45217=LINE ( 'NONE', #46209, #93622 ) ;
#45227=VECTOR ( 'NONE', #88847, 1000.000000000000000 ) ;
#45228=CARTESIAN_POINT ( 'NONE',  ( -14.16423886937410437, 21.59541550158063927, -3.795296366450299885 ) ) ;
#45235=B_SPLINE_CURVE_WITH_KNOTS ( 'NONE', 3,
 ( #675, #17141, #40122, #24143, #23164, #24637 ),
 .UNSPECIFIED., .F., .F.,
 ( 4, 2, 4 ),
 ( 0.0002800392683662262074, 0.0006862448819792434616, 0.001092450495592260824 ),
 .UNSPECIFIED. ) ;
#45236=ORIENTED_EDGE ( 'NONE', *, *, #34055, .T. ) ;
#45242=LINE ( 'NONE', #7258, #40767 ) ;
#45246=VERTEX_POINT ( 'NONE', #79915 ) ;
#45253=CARTESIAN_POINT ( 'NONE',  ( -12.11353679309445219, 0.04962889481943084935, 8.421373815019547848 ) ) ;
#45259=EDGE_CURVE ( 'NONE', #45656, #26776, #34403, .T. ) ;
#45261=EDGE_CURVE ( 'NONE', #60216, #46867, #76697, .T. ) ;
#45264=ORIENTED_EDGE ( 'NONE', *, *, #28572, .T. ) ;
#45266=CARTESIAN_POINT ( 'NONE',  ( 0.000000000000000000, 14.49999999999999822, 0.000000000000000000 ) ) ;
#45271=LINE ( 'NONE', #75766, #39059 ) ;
#45282=ORIENTED_EDGE ( 'NONE', *, *, #4099, .T. ) ;
#45284=ORIENTED_EDGE ( 'NONE', *, *, #69793, .F. ) ;
#45288=CARTESIAN_POINT ( 'NONE',  ( 7.313705784284532996, 0.3639312656126381662, 13.09617149020750837 ) ) ;
#45289=ORIENTED_EDGE ( 'NONE', *, *, #61081, .F. ) ;
#45291=ADVANCED_FACE ( 'NONE', ( #64892 ), #17950, .F. ) ;
#45292=TOROIDAL_SURFACE ( 'NONE', #13312, 14.49999999999999822, 0.5000000000000000000 ) ;
#45293=EDGE_CURVE ( 'NONE', #49707, #89457, #49414, .T. ) ;
#45294=ORIENTED_EDGE ( 'NONE', *, *, #86840, .F. ) ;
#45302=DIRECTION ( 'NONE',  ( 0.000000000000000000, 1.000000000000000000, 0.000000000000000000 ) ) ;
#45303=DIRECTION ( 'NONE',  ( 0.7132504491541897806, 0.000000000000000000, -0.7009092642998425715 ) ) ;
#45306=ORIENTED_EDGE ( 'NONE', *, *, #97575, .T. ) ;
#45308=DIRECTION ( 'NONE',  ( 0.000000000000000000, 1.000000000000000000, 0.000000000000000000 ) ) ;
#45323=DIRECTION ( 'NONE',  ( 0.000000000000000000, 0.000000000000000000, 1.000000000000000000 ) ) ;
#45328=ORIENTED_EDGE ( 'NONE', *, *, #49422, .T. ) ;
#45334=DIRECTION ( 'NONE',  ( -0.9890158633619157147, 0.000000000000000000, -0.1478094111296180124 ) ) ;
#45345=CARTESIAN_POINT ( 'NONE',  ( 9.399392868737743711, 4.718572659598065102E-16, 11.04089732309480532 ) ) ;
#45353=CARTESIAN_POINT ( 'NONE',  ( 3.166711953933172286, 0.000000000000000000, 4.439566422914491994 ) ) ;
#45354=DIRECTION ( 'NONE',  ( 0.000000000000000000, 0.000000000000000000, 1.000000000000000000 ) ) ;
#45362=FACE_OUTER_BOUND ( 'NONE', #68440, .T. ) ;
#45363=CARTESIAN_POINT ( 'NONE',  ( -14.75001642003105040, 0.04962894700187112096, -0.3071237627331344089 ) ) ;
#45369=DIRECTION ( 'NONE',  ( -0.000000000000000000, -1.000000000000000000, -0.000000000000000000 ) ) ;
#45374=CARTESIAN_POINT ( 'NONE',  ( -3.384800920123979484, 14.76930270348881180, -14.55270344038012453 ) ) ;
#45389=ORIENTED_EDGE ( 'NONE', *, *, #79926, .F. ) ;
#45390=EDGE_CURVE ( 'NONE', #54861, #54024, #90362, .T. ) ;
#45402=CARTESIAN_POINT ( 'NONE',  ( 5.279540384298776701, 0.000000000000000000, 1.365381980696741548 ) ) ;
#45403=CARTESIAN_POINT ( 'NONE',  ( 0.000000000000000000, 15.00000000000000000, 0.000000000000000000 ) ) ;
#45405=CARTESIAN_POINT ( 'NONE',  ( -14.16722289976678617, 0.5000000000000004441, -4.928467845925704083 ) ) ;
#45408=ORIENTED_EDGE ( 'NONE', *, *, #98249, .F. ) ;
#45410=CARTESIAN_POINT ( 'NONE',  ( -6.408140936763246032, -16.70969866340291077, -11.09922568453594316 ) ) ;
#45414=FACE_OUTER_BOUND ( 'NONE', #89320, .T. ) ;
#45425=CARTESIAN_POINT ( 'NONE',  ( -14.29730467489530632, 4.415605380435452030E-16, -2.416004766803409254 ) ) ;
#45427=ORIENTED_EDGE ( 'NONE', *, *, #93804, .F. ) ;
#45428=CARTESIAN_POINT ( 'NONE',  ( -12.21238578216017245, -2.320870275476780957E-16, 8.049595036947042814 ) ) ;
#45429=EDGE_CURVE ( 'NONE', #13614, #1450, #43148, .T. ) ;
#45436=PLANE ( 'NONE',  #2180 ) ;
#45437=EDGE_CURVE ( 'NONE', #59690, #84144, #60367, .T. ) ;
#45439=CARTESIAN_POINT ( 'NONE',  ( -8.209432707284749497, 14.49999999999999112, -12.55409154915501269 ) ) ;
#45442=ORIENTED_EDGE ( 'NONE', *, *, #3312, .T. ) ;
#45443=CARTESIAN_POINT ( 'NONE',  ( 9.742785792574933268, 3.034700295649320534, -5.625000000000003553 ) ) ;
#45445=TOROIDAL_SURFACE ( 'NONE', #3997, 14.49999999999999822, 0.5000000000000000000 ) ;
#45451=EDGE_CURVE ( 'NONE', #91405, #22543, #98409, .T. ) ;
#45455=CARTESIAN_POINT ( 'NONE',  ( -2.815433093576914736, 14.49999999999999112, -14.73340885523760413 ) ) ;
#45464=CARTESIAN_POINT ( 'NONE',  ( 11.48952521350825151, 15.00000000000000000, -8.845383562535966249 ) ) ;
#45467=CARTESIAN_POINT ( 'NONE',  ( -12.26659068614895354, -18.61291783175269288, -7.082119434687038861 ) ) ;
#45477=CARTESIAN_POINT ( 'NONE',  ( 5.991992585808519678, 15.00000000000000000, 13.20401548210297271 ) ) ;
#45479=CARTESIAN_POINT ( 'NONE',  ( 7.551349515323185990, -0.03417435944610275333, -12.08468537022906020 ) ) ;
#45482=CARTESIAN_POINT ( 'NONE',  ( 3.469446951953614189E-15, 24.31368534415484461, 10.88017736071110342 ) ) ;
#45487=DIRECTION ( 'NONE',  ( -0.000000000000000000, -1.000000000000000000, -0.000000000000000000 ) ) ;
#45495=EDGE_CURVE ( 'NONE', #23012, #97173, #6886, .T. ) ;
#45524=ADVANCED_FACE ( 'NONE', ( #36397 ), #68384, .F. ) ;
#45526=DIRECTION ( 'NONE',  ( -3.463895836830488406E-14, 0.000000000000000000, 1.000000000000000000 ) ) ;
#45527=CARTESIAN_POINT ( 'NONE',  ( 0.000000000000000000, 0.000000000000000000, 0.000000000000000000 ) ) ;
#45532=CARTESIAN_POINT ( 'NONE',  ( -6.869455772996959197, 15.00000000000000000, -14.44603661281848517 ) ) ;
#45536=CARTESIAN_POINT ( 'NONE',  ( -9.846743663894590881, 16.21726448433411960, 2.638427012816840111 ) ) ;
#45538=ORIENTED_EDGE ( 'NONE', *, *, #97672, .F. ) ;
#45563=FACE_OUTER_BOUND ( 'NONE', #28353, .T. ) ;
#45568=ORIENTED_EDGE ( 'NONE', *, *, #68407, .F. ) ;
#45589=ORIENTED_EDGE ( 'NONE', *, *, #80948, .F. ) ;
#45590=ORIENTED_EDGE ( 'NONE', *, *, #73141, .T. ) ;
#45602=CARTESIAN_POINT ( 'NONE',  ( -10.88017736071110164, -12.14464798917849642, -2.915334737309917212 ) ) ;
#45607=LINE ( 'NONE', #51133, #30404 ) ;
#45614=CARTESIAN_POINT ( 'NONE',  ( -7.109031286574684749, 0.04962885628204312394, -12.92745085449648101 ) ) ;
#45615=CIRCLE ( 'NONE', #23304, 14.49999999999999822 ) ;
#45620=PLANE ( 'NONE',  #70295 ) ;
#45632=TOROIDAL_SURFACE ( 'NONE', #24884, 14.49999999999999822, 0.5000000000000000000 ) ;
#45635=AXIS2_PLACEMENT_3D ( 'NONE', #73312, #6305, #96834 ) ;
#45637=ORIENTED_EDGE ( 'NONE', *, *, #85395, .T. ) ;
#45638=CIRCLE ( 'NONE', #28073, 14.49999999999999822 ) ;
#45642=EDGE_CURVE ( 'NONE', #28421, #18735, #41672, .T. ) ;
#45650=VECTOR ( 'NONE', #56626, 1000.000000000000000 ) ;
#45655=CARTESIAN_POINT ( 'NONE',  ( -7.208316651077756099, -18.36606884899920900, 7.208316651077766757 ) ) ;
#45656=VERTEX_POINT ( 'NONE', #91864 ) ;
#45657=CARTESIAN_POINT ( 'NONE',  ( 0.1034006766821536916, 15.00000000000000000, -14.49963131600461352 ) ) ;
#45658=ORIENTED_EDGE ( 'NONE', *, *, #26632, .T. ) ;
#45661=CARTESIAN_POINT ( 'NONE',  ( -0.7375392941519193224, 0.3639308982088595434, 14.98185688723474129 ) ) ;
#45666=DIRECTION ( 'NONE',  ( 0.1132032137679039180, 0.000000000000000000, 0.9935718556765877896 ) ) ;
#45667=DIRECTION ( 'NONE',  ( -0.000000000000000000, -1.000000000000000000, -0.000000000000000000 ) ) ;
#45669=CIRCLE ( 'NONE', #40890, 14.49999999999999822 ) ;
#45670=CARTESIAN_POINT ( 'NONE',  ( -11.09922568453594316, 19.54030133659709279, 6.408140936763246920 ) ) ;
#45671=ORIENTED_EDGE ( 'NONE', *, *, #4569, .T. ) ;
#45680=DIRECTION ( 'NONE',  ( 0.000000000000000000, 1.000000000000000000, 0.000000000000000000 ) ) ;
#45683=CIRCLE ( 'NONE', #7365, 15.00000000000000000 ) ;
#45691=CARTESIAN_POINT ( 'NONE',  ( -12.07856007377833407, 3.961594683405543780E-16, 8.022367888854752493 ) ) ;
#45695=ORIENTED_EDGE ( 'NONE', *, *, #34109, .T. ) ;
#45697=DIRECTION ( 'NONE',  ( 0.000000000000000000, 1.000000000000000000, 0.000000000000000000 ) ) ;
#45701=CARTESIAN_POINT ( 'NONE',  ( -9.402796353261225093, 14.49999999999999112, 11.68706210897757281 ) ) ;
#45710=CARTESIAN_POINT ( 'NONE',  ( 13.75801628063878645, 4.006593314786880238E-16, 4.578972376164555769 ) ) ;
#45714=ORIENTED_EDGE ( 'NONE', *, *, #71907, .F. ) ;
#45715=DIRECTION ( 'NONE',  ( 0.4305110968083047940, 0.000000000000000000, -0.9025852843498560762 ) ) ;
#45719=DIRECTION ( 'NONE',  ( -0.000000000000000000, -1.000000000000000000, -0.000000000000000000 ) ) ;
#45727=CARTESIAN_POINT ( 'NONE',  ( 7.082119434687047743, 20.13708216824730712, -12.26659068614894821 ) ) ;
#45729=EDGE_CURVE ( 'NONE', #63731, #74051, #47329, .T. ) ;
#45731=CARTESIAN_POINT ( 'NONE',  ( 9.898881779040729967, 0.000000000000000000, -10.25059215482576214 ) ) ;
#45735=VECTOR ( 'NONE', #12362, 999.9999999999998863 ) ;
#45745=FACE_OUTER_BOUND ( 'NONE', #62649, .T. ) ;
#45746=ADVANCED_FACE ( 'NONE', ( #31834 ), #30858, .F. ) ;
#45753=CARTESIAN_POINT ( 'NONE',  ( -11.96291822454869802, 4.725512573308054359E-16, -8.193813980849247613 ) ) ;
#45755=LINE ( 'NONE', #77223, #23478 ) ;
#45757=B_SPLINE_CURVE_WITH_KNOTS ( 'NONE', 3,
 ( #28347, #81348, #7714, #65346, #91689, #42375 ),
 .UNSPECIFIED., .F., .F.,
 ( 4, 2, 4 ),
 ( 0.0002800138956522161475, 0.0006862192609926581061, 0.001092424626333100010 ),
 .UNSPECIFIED. ) ;
#45766=ORIENTED_EDGE ( 'NONE', *, *, #11405, .F. ) ;
#45767=VERTEX_POINT ( 'NONE', #1869 ) ;
#45797=ORIENTED_EDGE ( 'NONE', *, *, #6438, .T. ) ;
#45801=EDGE_LOOP ( 'NONE', ( #44679, #98401, #12608, #34311 ) ) ;
#45804=CYLINDRICAL_SURFACE ( 'NONE', #88105, 15.00000000000000000 ) ;
#45805=CARTESIAN_POINT ( 'NONE',  ( 2.815433093577012880, 14.49999999999999112, 14.73340885523758281 ) ) ;
#45810=VECTOR ( 'NONE', #28542, 1000.000000000000114 ) ;
#45812=AXIS2_PLACEMENT_3D ( 'NONE', #49509, #3549, #57016 ) ;
#45813=PLANE ( 'NONE',  #8797 ) ;
#45823=DIRECTION ( 'NONE',  ( -0.000000000000000000, -1.000000000000000000, -0.000000000000000000 ) ) ;
#45829=CARTESIAN_POINT ( 'NONE',  ( 0.000000000000000000, 15.00000000000000000, 0.000000000000000000 ) ) ;
#45835=ORIENTED_EDGE ( 'NONE', *, *, #57984, .F. ) ;
#45836=VECTOR ( 'NONE', #80419, 1000.000000000000114 ) ;
#45838=DIRECTION ( 'NONE',  ( -0.04361938736532633420, 0.000000000000000000, -0.9990482215818581313 ) ) ;
#45847=LINE ( 'NONE', #75840, #65446 ) ;
#45855=EDGE_CURVE ( 'NONE', #44471, #15375, #8849, .T. ) ;
#45858=VECTOR ( 'NONE', #51726, 1000.000000000000114 ) ;
#45861=LINE ( 'NONE', #53852, #94975 ) ;
#45864=EDGE_CURVE ( 'NONE', #70611, #63731, #95987, .T. ) ;
#45869=ORIENTED_EDGE ( 'NONE', *, *, #53411, .T. ) ;
#45871=CARTESIAN_POINT ( 'NONE',  ( -4.289191146912808207E-15, 8.868033628982656680, -11.25000000000000178 ) ) ;
#45875=AXIS2_PLACEMENT_3D ( 'NONE', #83310, #69794, #54763 ) ;
#45877=CARTESIAN_POINT ( 'NONE',  ( -14.99847009497950800, 14.49999999999999112, -0.2142307401082109986 ) ) ;
#45883=CARTESIAN_POINT ( 'NONE',  ( -8.731067818237029599, 3.287123368507813836, 8.731067818237043809 ) ) ;
#45885=AXIS2_PLACEMENT_3D ( 'NONE', #33455, #63952, #86963 ) ;
#45890=EDGE_CURVE ( 'NONE', #8159, #31701, #17143, .T. ) ;
#45897=FACE_OUTER_BOUND ( 'NONE', #20194, .T. ) ;
#45920=CARTESIAN_POINT ( 'NONE',  ( 11.09922568453594671, -7.959698663402909879, -6.408140936763241591 ) ) ;
#45935=ORIENTED_EDGE ( 'NONE', *, *, #98486, .T. ) ;
#45948=PLANE ( 'NONE',  #77693 ) ;
#45951=CIRCLE ( 'NONE', #97075, 14.49999999999999822 ) ;
#45953=CARTESIAN_POINT ( 'NONE',  ( 11.24999999999999822, 2.559852905346091223, 0.8418318073276112035 ) ) ;
#45968=CARTESIAN_POINT ( 'NONE',  ( 5.302565485995484273, 0.000000000000000000, 1.273033341818867736 ) ) ;
#45970=CARTESIAN_POINT ( 'NONE',  ( 14.49154782522701446, 0.04962890019108410350, -2.766288502466956345 ) ) ;
#45973=CARTESIAN_POINT ( 'NONE',  ( 14.16423886937410437, -0.9045844984193566196, 3.795296366450304770 ) ) ;
#45978=ORIENTED_EDGE ( 'NONE', *, *, #32736, .F. ) ;
#45984=CARTESIAN_POINT ( 'NONE',  ( 12.80781515976310203, -0.03417435944610275333, 6.246788841744411513 ) ) ;
#45990=CARTESIAN_POINT ( 'NONE',  ( -14.88585913059880284, 0.2301501830257628445, -1.278057234794063302 ) ) ;
#45996=CARTESIAN_POINT ( 'NONE',  ( -1.820328553599931842, 0.000000000000000000, 5.140449258537799437 ) ) ;
#46007=FACE_OUTER_BOUND ( 'NONE', #62250, .T. ) ;
#46010=DIRECTION ( 'NONE',  ( -0.6225146366376129725, 0.000000000000000000, -0.7826081568524190235 ) ) ;
#46020=CARTESIAN_POINT ( 'NONE',  ( 9.399392868737814766, 15.00000000000000000, -11.04089732309474314 ) ) ;
#46023=ADVANCED_FACE ( 'NONE', ( #64290 ), #32816, .F. ) ;
#46027=ORIENTED_EDGE ( 'NONE', *, *, #53329, .T. ) ;
#46042=CARTESIAN_POINT ( 'NONE',  ( 9.846743663894594434, 28.50893115100078390, -2.168404344971008868E-15 ) ) ;
#46043=VERTEX_POINT ( 'NONE', #95803 ) ;
#46044=CARTESIAN_POINT ( 'NONE',  ( 11.62719953690064933, 14.49999999999999822, -9.476720473301794456 ) ) ;
#46045=ORIENTED_EDGE ( 'NONE', *, *, #33966, .T. ) ;
#46052=VERTEX_POINT ( 'NONE', #57781 ) ;
#46057=VERTEX_POINT ( 'NONE', #73281 ) ;
#46070=ORIENTED_EDGE ( 'NONE', *, *, #19318, .T. ) ;
#46071=FACE_OUTER_BOUND ( 'NONE', #1099, .T. ) ;
#46090=EDGE_CURVE ( 'NONE', #51581, #37077, #4024, .T. ) ;
#46092=VERTEX_POINT ( 'NONE', #94802 ) ;
#46101=CARTESIAN_POINT ( 'NONE',  ( -14.35840480524197815, 0.3639308199838639513, -4.340070442839035536 ) ) ;
#46103=VECTOR ( 'NONE', #47723, 1000.000000000000000 ) ;
#46106=CARTESIAN_POINT ( 'NONE',  ( -5.440088680355558814, -17.76964798917849109, -9.422509992056136596 ) ) ;
#46111=DIRECTION ( 'NONE',  ( 0.8788171126619711560, 0.000000000000000000, -0.4771587602595978028 ) ) ;
#46119=DIRECTION ( 'NONE',  ( 0.1822355254921448620, 0.000000000000000000, 0.9832549075639551717 ) ) ;
#46124=DIRECTION ( 'NONE',  ( 0.9969173337331278528, 0.000000000000000000, 0.07845909572784538766 ) ) ;
#46132=ADVANCED_FACE ( 'NONE', ( #79803 ), #52263, .F. ) ;
#46133=CARTESIAN_POINT ( 'NONE',  ( 5.817157072110800797, 0.5000000000000004441, -13.82608706751086558 ) ) ;
#46135=ORIENTED_EDGE ( 'NONE', *, *, #81136, .F. ) ;
#46141=DIRECTION ( 'NONE',  ( -1.509903313490212895E-14, 0.000000000000000000, 1.000000000000000000 ) ) ;
#46151=VECTOR ( 'NONE', #49661, 1000.000000000000000 ) ;
#46153=CARTESIAN_POINT ( 'NONE',  ( -7.208316651077756099, -28.36606884899921610, 7.208316651077766757 ) ) ;
#46156=ORIENTED_EDGE ( 'NONE', *, *, #1307, .T. ) ;
#46158=ORIENTED_EDGE ( 'NONE', *, *, #1387, .F. ) ;
#46159=CARTESIAN_POINT ( 'NONE',  ( 0.000000000000000000, 15.00000000000000000, 0.000000000000000000 ) ) ;
#46168=CARTESIAN_POINT ( 'NONE',  ( 3.434112377981060948, 20.58196800326374643, 12.81628187352647430 ) ) ;
#46170=ADVANCED_FACE ( 'NONE', ( #59756 ), #71987, .T. ) ;
#46173=ORIENTED_EDGE ( 'NONE', *, *, #77246, .F. ) ;
#46187=ORIENTED_EDGE ( 'NONE', *, *, #55600, .F. ) ;
#46190=EDGE_CURVE ( 'NONE', #32127, #83513, #72004, .T. ) ;
#46194=PLANE ( 'NONE',  #81049 ) ;
#46200=CARTESIAN_POINT ( 'NONE',  ( -13.21236992757665973, -0.03417435944610275333, -5.338143956176898186 ) ) ;
#46208=VERTEX_POINT ( 'NONE', #14782 ) ;
#46209=CARTESIAN_POINT ( 'NONE',  ( -1.780824192092292924, 15.00000000000000000, -14.89391369643515795 ) ) ;
#46213=EDGE_CURVE ( 'NONE', #24676, #8841, #4804, .T. ) ;
#46214=B_SPLINE_CURVE_WITH_KNOTS ( 'NONE', 3,
 ( #47314, #93809, #77814, #25339, #66759, #50262 ),
 .UNSPECIFIED., .F., .F.,
 ( 4, 2, 4 ),
 ( 3.409110551494646689E-05, 0.0004400426677367928058, 0.0008459942299586391311 ),
 .UNSPECIFIED. ) ;
#46215=CARTESIAN_POINT ( 'NONE',  ( 0.000000000000000000, 14.49999999999999822, 0.000000000000000000 ) ) ;
#46222=CARTESIAN_POINT ( 'NONE',  ( 12.26659068614894466, 19.72041550158062861, -7.082119434687053960 ) ) ;
#46241=ORIENTED_EDGE ( 'NONE', *, *, #79926, .T. ) ;
#46253=AXIS2_PLACEMENT_3D ( 'NONE', #94937, #55480, #2987 ) ;
#46258=ORIENTED_EDGE ( 'NONE', *, *, #39088, .F. ) ;
#46265=DIRECTION ( 'NONE',  ( 0.000000000000000000, 0.000000000000000000, 1.000000000000000000 ) ) ;
#46269=CARTESIAN_POINT ( 'NONE',  ( -11.62112565934141983, 15.00000000000000888, -8.881879596174913516 ) ) ;
#46274=LINE ( 'NONE', #39275, #21965 ) ;
#46282=EDGE_LOOP ( 'NONE', ( #78089, #87469, #10503, #17174 ) ) ;
#46287=ORIENTED_EDGE ( 'NONE', *, *, #33124, .T. ) ;
#46292=DIRECTION ( 'NONE',  ( 0.000000000000000000, 1.000000000000000000, 0.000000000000000000 ) ) ;
#46295=ORIENTED_EDGE ( 'NONE', *, *, #81489, .T. ) ;
#46314=AXIS2_PLACEMENT_3D ( 'NONE', #61889, #1425, #31877 ) ;
#46316=VECTOR ( 'NONE', #55731, 1000.000000000000114 ) ;
#46336=FACE_OUTER_BOUND ( 'NONE', #60330, .T. ) ;
#46337=CARTESIAN_POINT ( 'NONE',  ( 0.000000000000000000, 0.5000000000000004441, 0.000000000000000000 ) ) ;
#46342=VERTEX_POINT ( 'NONE', #56573 ) ;
#46353=ORIENTED_EDGE ( 'NONE', *, *, #45855, .F. ) ;
#46354=CARTESIAN_POINT ( 'NONE',  ( -2.863845842056022661, 14.95077488074853456, 14.47219703936410617 ) ) ;
#46355=DIRECTION ( 'NONE',  ( 0.000000000000000000, 1.000000000000000000, 0.000000000000000000 ) ) ;
#46361=CARTESIAN_POINT ( 'NONE',  ( 15.33206046421389601, -0.03417435944610275333, 4.561284726668865197 ) ) ;
#46377=VECTOR ( 'NONE', #37399, 1000.000000000000000 ) ;
#46385=AXIS2_PLACEMENT_3D ( 'NONE', #60182, #14207, #90678 ) ;
#46388=ADVANCED_FACE ( 'NONE', ( #63565 ), #30521, .T. ) ;
#46399=DIRECTION ( 'NONE',  ( -0.000000000000000000, -1.000000000000000000, -0.000000000000000000 ) ) ;
#46401=ORIENTED_EDGE ( 'NONE', *, *, #56714, .T. ) ;
#46411=ADVANCED_FACE ( 'NONE', ( #10578 ), #86416, .T. ) ;
#46420=ORIENTED_EDGE ( 'NONE', *, *, #19347, .F. ) ;
#46425=CARTESIAN_POINT ( 'NONE',  ( 14.69266224296806200, 14.95037104324574884, -1.335284760094769263 ) ) ;
#46429=CARTESIAN_POINT ( 'NONE',  ( -12.80781515976305762, 0.000000000000000000, -6.246788841744501219 ) ) ;
#46442=EDGE_CURVE ( 'NONE', #1044, #22386, #27042, .T. ) ;
#46455=CARTESIAN_POINT ( 'NONE',  ( -14.16423886937410437, -8.404584498419364280, -3.795296366450299885 ) ) ;
#46459=ORIENTED_EDGE ( 'NONE', *, *, #73699, .F. ) ;
#46467=CARTESIAN_POINT ( 'NONE',  ( 14.42571047809456175, 0.2306972965111693252, 3.890621016587945569 ) ) ;
#46469=FACE_OUTER_BOUND ( 'NONE', #30850, .T. ) ;
#46477=VECTOR ( 'NONE', #864, 1000.000000000000000 ) ;
#46488=DIRECTION ( 'NONE',  ( 0.000000000000000000, 0.000000000000000000, 1.000000000000000000 ) ) ;
#46489=CYLINDRICAL_SURFACE ( 'NONE', #22283, 15.00000000000000000 ) ;
#46500=DIRECTION ( 'NONE',  ( -2.042810365310288034E-14, 0.000000000000000000, 1.000000000000000000 ) ) ;
#46516=CARTESIAN_POINT ( 'NONE',  ( 8.838651438279482520, 14.95077488074853456, 11.81204219878344475 ) ) ;
#46517=CARTESIAN_POINT ( 'NONE',  ( 4.923371831947295441, 24.34226448433413026, -8.527530157486179263 ) ) ;
#46519=VECTOR ( 'NONE', #97562, 1000.000000000000000 ) ;
#46530=ORIENTED_EDGE ( 'NONE', *, *, #39088, .T. ) ;
#46534=ORIENTED_EDGE ( 'NONE', *, *, #2392, .F. ) ;
#46544=LINE ( 'NONE', #9039, #20315 ) ;
#46550=ORIENTED_EDGE ( 'NONE', *, *, #42281, .T. ) ;
#46552=DIRECTION ( 'NONE',  ( -0.9099612708765399960, 0.000000000000000000, -0.4146932426562462415 ) ) ;
#46554=LINE ( 'NONE', #23586, #22539 ) ;
#46557=DIRECTION ( 'NONE',  ( -0.000000000000000000, 1.000000000000000000, -0.000000000000000000 ) ) ;
#46564=EDGE_CURVE ( 'NONE', #25275, #26584, #22616, .T. ) ;
#46570=EDGE_LOOP ( 'NONE', ( #84668, #96604, #61866, #48029, #4616, #67376 ) ) ;
#46584=CARTESIAN_POINT ( 'NONE',  ( 10.88017736071109987, 0.7720186774881703240, -2.915334737309928315 ) ) ;
#46586=CARTESIAN_POINT ( 'NONE',  ( -0.1034006766821533585, 0.000000000000000000, -14.49963131600461175 ) ) ;
#46590=CARTESIAN_POINT ( 'NONE',  ( -14.56311970191023164, 0.2301500865527675577, -3.337330457606075829 ) ) ;
#46593=CARTESIAN_POINT ( 'NONE',  ( 7.771322705631503069, 15.00000000000000000, -12.24159072199917375 ) ) ;
#46597=CARTESIAN_POINT ( 'NONE',  ( 9.240973841163606650, 4.560084876699663581E-16, -11.17382667070372726 ) ) ;
#46599=ORIENTED_EDGE ( 'NONE', *, *, #19468, .T. ) ;
#46611=CARTESIAN_POINT ( 'NONE',  ( 0.000000000000000000, 14.49999999999999822, 0.000000000000000000 ) ) ;
#46615=VECTOR ( 'NONE', #88564, 1000.000000000000114 ) ;
#46628=CARTESIAN_POINT ( 'NONE',  ( -7.208316651077764980, -4.616068848999211660, -7.208316651077759651 ) ) ;
#46629=ORIENTED_EDGE ( 'NONE', *, *, #62428, .F. ) ;
#46638=DIRECTION ( 'NONE',  ( 0.3502073812594559410, 0.000000000000000000, 0.9366721892484018985 ) ) ;
#46639=CARTESIAN_POINT ( 'NONE',  ( -2.393480905993275343, 14.63606894034134420, 14.80781041047753810 ) ) ;
#46641=EDGE_CURVE ( 'NONE', #37440, #63858, #43357, .T. ) ;
#46643=VERTEX_POINT ( 'NONE', #59022 ) ;
#46644=VECTOR ( 'NONE', #2573, 1000.000000000000227 ) ;
#46647=TOROIDAL_SURFACE ( 'NONE', #37097, 14.49999999999999822, 0.5000000000000000000 ) ;
#46649=EDGE_LOOP ( 'NONE', ( #56720, #13596, #78465, #13706, #25544, #85446 ) ) ;
#46655=AXIS2_PLACEMENT_3D ( 'NONE', #38855, #1851, #77811 ) ;
#46659=AXIS2_PLACEMENT_3D ( 'NONE', #33772, #2841, #72765 ) ;
#46662=DIRECTION ( 'NONE',  ( 0.000000000000000000, 0.000000000000000000, 1.000000000000000000 ) ) ;
#46673=CARTESIAN_POINT ( 'NONE',  ( 0.000000000000000000, 14.49999999999999822, 0.000000000000000000 ) ) ;
#46686=ORIENTED_EDGE ( 'NONE', *, *, #46851, .T. ) ;
#46694=CARTESIAN_POINT ( 'NONE',  ( 10.32896413005680181, 5.578790035174474582, -5.963430220938285231 ) ) ;
#46699=CARTESIAN_POINT ( 'NONE',  ( -10.88017736071109987, -31.72798132251182679, 2.915334737309934532 ) ) ;
#46707=ORIENTED_EDGE ( 'NONE', *, *, #97575, .F. ) ;
#46721=CARTESIAN_POINT ( 'NONE',  ( 14.17193700899789022, -0.03417435944610275333, 1.489530601564113654 ) ) ;
#46722=DIRECTION ( 'NONE',  ( -0.000000000000000000, -1.000000000000000000, -0.000000000000000000 ) ) ;
#46729=DIRECTION ( 'NONE',  ( 0.000000000000000000, 0.000000000000000000, 1.000000000000000000 ) ) ;
#46734=VERTEX_POINT ( 'NONE', #84002 ) ;
#46735=ORIENTED_EDGE ( 'NONE', *, *, #6509, .F. ) ;
#46736=CARTESIAN_POINT ( 'NONE',  ( -11.62719953690071506, 15.00000000000000000, 9.476720473301710967 ) ) ;
#46744=ADVANCED_FACE ( 'NONE', ( #59518 ), #38540, .T. ) ;
#46748=CARTESIAN_POINT ( 'NONE',  ( -11.29168986245629469, 14.76984976272667360, 9.783658503027758968 ) ) ;
#46753=ORIENTED_EDGE ( 'NONE', *, *, #31843, .F. ) ;
#46755=ORIENTED_EDGE ( 'NONE', *, *, #25222, .F. ) ;
#46758=ORIENTED_EDGE ( 'NONE', *, *, #76347, .F. ) ;
#46774=DIRECTION ( 'NONE',  ( 0.8038568606172162845, -0.000000000000000000, 0.5948227867513425915 ) ) ;
#46778=ORIENTED_EDGE ( 'NONE', *, *, #7546, .F. ) ;
#46781=DIRECTION ( 'NONE',  ( 0.000000000000000000, 0.000000000000000000, 1.000000000000000000 ) ) ;
#46784=TOROIDAL_SURFACE ( 'NONE', #59565, 14.49999999999999822, 0.5000000000000000000 ) ;
#46787=CARTESIAN_POINT ( 'NONE',  ( 3.014428414850136129, 11.57636696231598350, 11.25000000000000000 ) ) ;
#46798=CARTESIAN_POINT ( 'NONE',  ( 12.60589901313216110, 0.5000000000000004441, 8.129656208642140669 ) ) ;
#46805=CARTESIAN_POINT ( 'NONE',  ( 0.000000000000000000, 0.5000000000000004441, 0.000000000000000000 ) ) ;
#46810=DIRECTION ( 'NONE',  ( 0.8338858220671618859, 0.000000000000000000, 0.5519369853120676961 ) ) ;
#46813=CARTESIAN_POINT ( 'NONE',  ( 9.399392868737718842, 15.00000000000000000, 11.04089732309479110 ) ) ;
#46819=DIRECTION ( 'NONE',  ( -0.000000000000000000, -1.000000000000000000, -0.000000000000000000 ) ) ;
#46824=FACE_OUTER_BOUND ( 'NONE', #71652, .T. ) ;
#46827=DIRECTION ( 'NONE',  ( 0.02617694830786938473, -0.000000000000000000, 0.9996573249755573709 ) ) ;
#46841=CARTESIAN_POINT ( 'NONE',  ( 9.820177974736397530, 14.76984956101181368, -11.25994418464053126 ) ) ;
#46846=PLANE ( 'NONE',  #44249 ) ;
#46847=CARTESIAN_POINT ( 'NONE',  ( 0.000000000000000000, 15.00000000000000000, 0.000000000000000000 ) ) ;
#46851=EDGE_CURVE ( 'NONE', #33104, #93159, #94392, .T. ) ;
#46855=ADVANCED_FACE ( 'NONE', ( #46007 ), #82019, .T. ) ;
#46864=AXIS2_PLACEMENT_3D ( 'NONE', #12913, #27910, #50915 ) ;
#46867=VERTEX_POINT ( 'NONE', #76497 ) ;
#46868=VECTOR ( 'NONE', #95236, 1000.000000000000114 ) ;
#46881=CYLINDRICAL_SURFACE ( 'NONE', #52500, 15.00000000000000000 ) ;
#46884=ORIENTED_EDGE ( 'NONE', *, *, #65715, .T. ) ;
#46885=EDGE_CURVE ( 'NONE', #31483, #48866, #71359, .T. ) ;
#46893=EDGE_CURVE ( 'NONE', #68696, #50677, #64049, .T. ) ;
#46895=CARTESIAN_POINT ( 'NONE',  ( -13.21236992757677164, 15.00000000000000000, 5.338143956176621074 ) ) ;
#46896=ORIENTED_EDGE ( 'NONE', *, *, #71907, .T. ) ;
#46900=DIRECTION ( 'NONE',  ( 0.5075383629606904368, 0.000000000000000000, 0.8616291604415338146 ) ) ;
#46904=CARTESIAN_POINT ( 'NONE',  ( 0.000000000000000000, 15.00000000000000000, 0.000000000000000000 ) ) ;
#46905=DIRECTION ( 'NONE',  ( -2.930988785010413267E-14, 0.000000000000000000, 1.000000000000000000 ) ) ;
#46907=CARTESIAN_POINT ( 'NONE',  ( 14.94699059465108171, 14.49999999999999112, -1.259949270174796965 ) ) ;
#46908=DIRECTION ( 'NONE',  ( -0.3007057995042767273, 0.000000000000000000, 0.9537169507482258224 ) ) ;
#46910=CARTESIAN_POINT ( 'NONE',  ( 12.80781515976314822, -0.03417435944610275333, -6.246788841744324472 ) ) ;
#46914=CARTESIAN_POINT ( 'NONE',  ( 11.12471383767373467, 2.500000000000004885, 1.674288514525068328 ) ) ;
#46920=CARTESIAN_POINT ( 'NONE',  ( 14.35840480524197282, 0.5000000000000004441, 4.340070442838948495 ) ) ;
#46928=CARTESIAN_POINT ( 'NONE',  ( -3.420591144908650350, 0.3640475087720806968, 14.60477854057954339 ) ) ;
#46934=ADVANCED_FACE ( 'NONE', ( #53990 ), #16990, .T. ) ;
#46938=CARTESIAN_POINT ( 'NONE',  ( -7.082119434687058401, -9.029584498419360727, -12.26659068614894110 ) ) ;
#46942=ORIENTED_EDGE ( 'NONE', *, *, #33284, .F. ) ;
#46944=LINE ( 'NONE', #984, #56632 ) ;
#46955=DIRECTION ( 'NONE',  ( 0.000000000000000000, 0.000000000000000000, 1.000000000000000000 ) ) ;
#46970=EDGE_CURVE ( 'NONE', #25526, #42104, #51296, .T. ) ;
#46975=DIRECTION ( 'NONE',  ( -0.000000000000000000, -1.000000000000000000, -0.000000000000000000 ) ) ;
#46976=VERTEX_POINT ( 'NONE', #54474 ) ;
#46978=DIRECTION ( 'NONE',  ( -0.000000000000000000, -1.000000000000000000, -0.000000000000000000 ) ) ;
#46991=ORIENTED_EDGE ( 'NONE', *, *, #67143, .F. ) ;
#46998=CARTESIAN_POINT ( 'NONE',  ( -9.323033696084856103, 14.95037104545394868, -11.43408728005525710 ) ) ;
#47004=DIRECTION ( 'NONE',  ( -0.02617694830786282401, 0.000000000000000000, -0.9996573249755575929 ) ) ;
#47006=CIRCLE ( 'NONE', #714, 15.00000000000000000 ) ;
#47008=CARTESIAN_POINT ( 'NONE',  ( 3.469446951953614189E-15, 27.25893115100078035, 9.846743663894594434 ) ) ;
#47009=ORIENTED_EDGE ( 'NONE', *, *, #1307, .F. ) ;
#47018=EDGE_LOOP ( 'NONE', ( #13418, #56119, #40742, #96954 ) ) ;
#47022=ORIENTED_EDGE ( 'NONE', *, *, #15600, .F. ) ;
#47030=AXIS2_PLACEMENT_3D ( 'NONE', #17254, #54727, #78727 ) ;
#47035=ORIENTED_EDGE ( 'NONE', *, *, #25575, .T. ) ;
#47045=EDGE_LOOP ( 'NONE', ( #16045, #46187, #14664, #23508 ) ) ;
#47047=AXIS2_PLACEMENT_3D ( 'NONE', #23982, #63434, #69473 ) ;
#47051=ADVANCED_FACE ( 'NONE', ( #13937 ), #35927, .F. ) ;
#47069=CARTESIAN_POINT ( 'NONE',  ( -5.440088680355547268, 3.897018677488178540, 9.422509992056143702 ) ) ;
#47076=DIRECTION ( 'NONE',  ( 0.7716245833877107829, 0.000000000000000000, 0.6360782202777751637 ) ) ;
#47082=CARTESIAN_POINT ( 'NONE',  ( -7.264509831664514472, 0.2301509507469247651, -13.05561747642799375 ) ) ;
#47101=ORIENTED_EDGE ( 'NONE', *, *, #80278, .T. ) ;
#47115=CARTESIAN_POINT ( 'NONE',  ( 9.846743663894594434, -16.49106884899920900, -2.168404344971008868E-15 ) ) ;
#47117=DIRECTION ( 'NONE',  ( 0.8870108331782213806, 0.000000000000000000, -0.4617486132350345773 ) ) ;
#47119=ORIENTED_EDGE ( 'NONE', *, *, #68527, .T. ) ;
#47126=B_SPLINE_CURVE_WITH_KNOTS ( 'NONE', 3,
 ( #32522, #33978, #11010, #2555, #56028, #55535 ),
 .UNSPECIFIED., .F., .F.,
 ( 4, 2, 4 ),
 ( 0.0002800808511812512844, 0.0006862868719359046989, 0.001092492892690558005 ),
 .UNSPECIFIED. ) ;
#47129=CARTESIAN_POINT ( 'NONE',  ( -6.408140936763232709, 29.95696800326377840, 11.09922568453595026 ) ) ;
#47134=ORIENTED_EDGE ( 'NONE', *, *, #43799, .F. ) ;
#47136=CARTESIAN_POINT ( 'NONE',  ( -0.4278561937608865717, 0.000000000000000000, 5.436428395565740423 ) ) ;
#47140=CARTESIAN_POINT ( 'NONE',  ( 14.97687855664614531, 14.49999999999999112, -0.8325315005900779664 ) ) ;
#47143=CARTESIAN_POINT ( 'NONE',  ( 0.3093388210927641713, 0.3627605259888580513, -14.99680997725065978 ) ) ;
#47147=ORIENTED_EDGE ( 'NONE', *, *, #21041, .T. ) ;
#47152=ORIENTED_EDGE ( 'NONE', *, *, #70361, .T. ) ;
#47153=CARTESIAN_POINT ( 'NONE',  ( 14.15281240980447031, -3.205596188883898450E-15, -3.688687068602698016 ) ) ;
#47163=EDGE_CURVE ( 'NONE', #69512, #23460, #27450, .T. ) ;
#47167=B_SPLINE_CURVE_WITH_KNOTS ( 'NONE', 3,
 ( #55682, #17692, #64137, #2706, #94159, #48657 ),
 .UNSPECIFIED., .F., .F.,
 ( 4, 2, 4 ),
 ( 0.0002800245631444417513, 0.0006862300328522872098, 0.001092435502560132722 ),
 .UNSPECIFIED. ) ;
#47168=ORIENTED_EDGE ( 'NONE', *, *, #2304, .F. ) ;
#47170=CARTESIAN_POINT ( 'NONE',  ( 0.000000000000000000, 14.49999999999999822, 0.000000000000000000 ) ) ;
#47174=CARTESIAN_POINT ( 'NONE',  ( -12.60589901313210071, 15.00000000000000000, -8.129656208642224158 ) ) ;
#47181=CARTESIAN_POINT ( 'NONE',  ( -14.16423886937409726, 32.01208216824730357, 3.795296366450320757 ) ) ;
#47185=CARTESIAN_POINT ( 'NONE',  ( -14.40939250469964783, 15.00000000000000000, 1.618458416365647023 ) ) ;
#47192=AXIS2_PLACEMENT_3D ( 'NONE', #48403, #1948, #16934 ) ;
#47199=DIRECTION ( 'NONE',  ( -0.6626200482157305061, 0.000000000000000000, -0.7489557207890082946 ) ) ;
#47200=CARTESIAN_POINT ( 'NONE',  ( 14.88232117145535760, 14.49999999999999112, 1.875237731503272887 ) ) ;
#47201=AXIS2_PLACEMENT_3D ( 'NONE', #98029, #20530, #52985 ) ;
#47206=VERTEX_POINT ( 'NONE', #68414 ) ;
#47209=DIRECTION ( 'NONE',  ( 0.000000000000000000, 0.000000000000000000, 1.000000000000000000 ) ) ;
#47212=CARTESIAN_POINT ( 'NONE',  ( 0.04758788293968784638, 0.000000000000000000, 5.453031268574421553 ) ) ;
#47216=CARTESIAN_POINT ( 'NONE',  ( -10.58981376305275468, 0.000000000000000000, -9.535111140613857117 ) ) ;
#47218=ORIENTED_EDGE ( 'NONE', *, *, #95142, .T. ) ;
#47220=LINE ( 'NONE', #46736, #2283 ) ;
#47234=B_SPLINE_CURVE_WITH_KNOTS ( 'NONE', 3,
 ( #7841, #68832, #364, #10782, #3284, #32778 ),
 .UNSPECIFIED., .F., .F.,
 ( 4, 2, 4 ),
 ( 3.409110551496121881E-05, 0.0004400426677367866800, 0.0008459942299586121345 ),
 .UNSPECIFIED. ) ;
#47237=ADVANCED_FACE ( 'NONE', ( #31376 ), #98441, .F. ) ;
#47249=ORIENTED_EDGE ( 'NONE', *, *, #45293, .T. ) ;
#47253=VERTEX_POINT ( 'NONE', #25863 ) ;
#47254=EDGE_CURVE ( 'NONE', #29544, #11914, #56360, .T. ) ;
#47259=CARTESIAN_POINT ( 'NONE',  ( 1.915564264621337776, 15.00000000000000000, 14.37291249357991774 ) ) ;
#47263=ORIENTED_EDGE ( 'NONE', *, *, #47583, .F. ) ;
#47264=ORIENTED_EDGE ( 'NONE', *, *, #27686, .T. ) ;
#47272=DIRECTION ( 'NONE',  ( 0.000000000000000000, 0.000000000000000000, -1.000000000000000000 ) ) ;
#47288=( NAMED_UNIT ( * ) SI_UNIT ( $, .STERADIAN. ) SOLID_ANGLE_UNIT ( ) );
#47291=ADVANCED_FACE ( 'NONE', ( #13824 ), #43808, .F. ) ;
#47292=CARTESIAN_POINT ( 'NONE',  ( 5.817157072110800797, 0.5000000000000004441, -13.82608706751086558 ) ) ;
#47299=EDGE_CURVE ( 'NONE', #18731, #58682, #14150, .T. ) ;
#47300=DIRECTION ( 'NONE',  ( -0.9366721892483995671, 0.000000000000000000, 0.3502073812594621027 ) ) ;
#47301=CIRCLE ( 'NONE', #26542, 14.49999999999999822 ) ;
#47302=DIRECTION ( 'NONE',  ( 0.000000000000000000, 0.000000000000000000, 1.000000000000000000 ) ) ;
#47308=B_SPLINE_CURVE_WITH_KNOTS ( 'NONE', 3,
 ( #70915, #32893, #2925, #69927, #18892, #78397 ),
 .UNSPECIFIED., .F., .F.,
 ( 4, 2, 4 ),
 ( 3.409110551496121881E-05, 0.0004400426677367872763, 0.0008459942299586133271 ),
 .UNSPECIFIED. ) ;
#47309=EDGE_CURVE ( 'NONE', #76280, #43600, #57829, .T. ) ;
#47314=CARTESIAN_POINT ( 'NONE',  ( 3.420591144908486481, 14.49999999999999112, 14.60477854057964109 ) ) ;
#47320=EDGE_CURVE ( 'NONE', #30635, #48953, #56234, .T. ) ;
#47322=LINE ( 'NONE', #31826, #8543 ) ;
#47323=CARTESIAN_POINT ( 'NONE',  ( -14.94699059465102664, 15.00000000000000000, 1.259949270174715696 ) ) ;
#47328=CARTESIAN_POINT ( 'NONE',  ( 14.35840480524197282, 0.5000000000000004441, 4.340070442838948495 ) ) ;
#47329=LINE ( 'NONE', #62830, #27302 ) ;
#47337=AXIS2_PLACEMENT_3D ( 'NONE', #50761, #82233, #26768 ) ;
#47354=ORIENTED_EDGE ( 'NONE', *, *, #51256, .F. ) ;
#47357=ORIENTED_EDGE ( 'NONE', *, *, #10646, .T. ) ;
#47359=EDGE_CURVE ( 'NONE', #39036, #36269, #3493, .T. ) ;
#47362=EDGE_LOOP ( 'NONE', ( #37923, #52097, #58587, #44648, #69898, #87523 ) ) ;
#47363=VECTOR ( 'NONE', #89833, 1000.000000000000000 ) ;
#47366=CIRCLE ( 'NONE', #36167, 14.49999999999999822 ) ;
#47372=CARTESIAN_POINT ( 'NONE',  ( -14.22792531055123888, 15.00000000000000711, 3.387425595041007043 ) ) ;
#47390=VERTEX_POINT ( 'NONE', #38794 ) ;
#47395=CARTESIAN_POINT ( 'NONE',  ( 0.000000000000000000, 0.000000000000000000, 0.000000000000000000 ) ) ;
#47396=DIRECTION ( 'NONE',  ( 0.000000000000000000, 0.000000000000000000, 1.000000000000000000 ) ) ;
#47402=DIRECTION ( 'NONE',  ( 0.000000000000000000, 1.000000000000000000, 0.000000000000000000 ) ) ;
#47408=EDGE_CURVE ( 'NONE', #46208, #70611, #62259, .T. ) ;
#47412=ADVANCED_FACE ( 'NONE', ( #37818 ), #59341, .T. ) ;
#47418=B_SPLINE_CURVE_WITH_KNOTS ( 'NONE', 3,
 ( #87506, #57496, #19018, #87990, #49496, #41537 ),
 .UNSPECIFIED., .F., .F.,
 ( 4, 2, 4 ),
 ( 0.0002800364959418014067, 0.0006862420824208874913, 0.001092447668899973467 ),
 .UNSPECIFIED. ) ;
#47423=CARTESIAN_POINT ( 'NONE',  ( 13.95749458852077218, 14.76930270348881002, 5.331641351773115822 ) ) ;
#47425=CARTESIAN_POINT ( 'NONE',  ( 5.056330833731752072, 3.901243639414221473E-16, -13.58983143750699973 ) ) ;
#47427=ORIENTED_EDGE ( 'NONE', *, *, #66413, .T. ) ;
#47430=DIRECTION ( 'NONE',  ( 0.000000000000000000, 0.000000000000000000, 1.000000000000000000 ) ) ;
#47432=VECTOR ( 'NONE', #79516, 1000.000000000000227 ) ;
#47434=CARTESIAN_POINT ( 'NONE',  ( 7.082119434687054849, -11.52958449841935717, 12.26659068614894288 ) ) ;
#47438=ORIENTED_EDGE ( 'NONE', *, *, #61114, .F. ) ;
#47443=CARTESIAN_POINT ( 'NONE',  ( -10.58981376305275468, -0.03417435944610275333, -9.535111140613857117 ) ) ;
#47447=ADVANCED_FACE ( 'NONE', ( #24291 ), #54757, .F. ) ;
#47450=CARTESIAN_POINT ( 'NONE',  ( -14.03351048042393856, 15.00000000000000000, -2.474486531753901541 ) ) ;
#47458=EDGE_LOOP ( 'NONE', ( #23250, #87138, #82552, #30766 ) ) ;
#47461=ADVANCED_FACE ( 'NONE', ( #91288 ), #45804, .T. ) ;
#47465=AXIS2_PLACEMENT_3D ( 'NONE', #12901, #66894, #13400 ) ;
#47468=FACE_OUTER_BOUND ( 'NONE', #26601, .T. ) ;
#47473=CARTESIAN_POINT ( 'NONE',  ( 7.551349515323100725, 15.00000000000000000, 12.08468537022911349 ) ) ;
#47491=DIRECTION ( 'NONE',  ( 0.000000000000000000, 0.000000000000000000, 1.000000000000000000 ) ) ;
#47500=CARTESIAN_POINT ( 'NONE',  ( -9.846743663894590881, 26.21726448433411960, 2.638427012816840111 ) ) ;
#47502=ORIENTED_EDGE ( 'NONE', *, *, #15946, .T. ) ;
#47505=AXIS2_PLACEMENT_3D ( 'NONE', #24341, #46819, #37868 ) ;
#47511=EDGE_CURVE ( 'NONE', #84080, #10597, #69785, .T. ) ;
#47512=AXIS2_PLACEMENT_3D ( 'NONE', #17904, #95366, #87857 ) ;
#47520=ORIENTED_EDGE ( 'NONE', *, *, #24059, .F. ) ;
#47524=B_SPLINE_CURVE_WITH_KNOTS ( 'NONE', 3,
 ( #50334, #36330, #74313, #65334, #73824, #81816 ),
 .UNSPECIFIED., .F., .F.,
 ( 4, 2, 4 ),
 ( 3.409110551496077836E-05, 0.0004400426677367842406, 0.0008459942299586076893 ),
 .UNSPECIFIED. ) ;
#47526=EDGE_CURVE ( 'NONE', #1162, #43600, #89217, .T. ) ;
#47532=ORIENTED_EDGE ( 'NONE', *, *, #25263, .F. ) ;
#47533=( BOUNDED_CURVE ( )  B_SPLINE_CURVE ( 2, ( #53695, #84218, #38706, #97256, #13732, #86663, #39700, #10663, #69206, #8689, #55161, #77669, #10175 ),
 .UNSPECIFIED., .F., .F. ) 
 B_SPLINE_CURVE_WITH_KNOTS ( ( 3, 2, 2, 2, 2, 2, 3 ),
 ( 0.5999999999999999778, 0.6055555555555555136, 0.6111111111111111605, 0.6166666666666666963, 0.6222222222222223431, 0.6277777777777778789, 0.6333333333333334147 ),
 .UNSPECIFIED. ) 
 CURVE ( )  GEOMETRIC_REPRESENTATION_ITEM ( )  RATIONAL_B_SPLINE_CURVE ( ( 1.000000000000000000, 0.9659258262890682012, 1.000000000000000000, 0.9659258262890682012, 1.000000000000000000, 0.9659258262890682012, 1.000000000000000000, 0.9659258262890682012, 1.000000000000000000, 0.9659258262890682012, 1.000000000000000000, 0.9659258262890675351, 1.000000000000000666 ) ) 
 REPRESENTATION_ITEM ( '' )  );
#47534=EDGE_CURVE ( 'NONE', #15285, #51412, #91402, .T. ) ;
#47535=B_SPLINE_CURVE_WITH_KNOTS ( 'NONE', 3,
 ( #59334, #43835, #50861, #12850, #42381, #43349 ),
 .UNSPECIFIED., .F., .F.,
 ( 4, 2, 4 ),
 ( 0.0002800111042658766803, 0.0006862164422996869110, 0.001092421780333497142 ),
 .UNSPECIFIED. ) ;
#47538=VERTEX_POINT ( 'NONE', #22322 ) ;
#47541=EDGE_CURVE ( 'NONE', #36269, #73854, #76122, .T. ) ;
#47550=VERTEX_POINT ( 'NONE', #77759 ) ;
#47561=EDGE_LOOP ( 'NONE', ( #16274, #86734, #66071, #27098 ) ) ;
#47562=ORIENTED_EDGE ( 'NONE', *, *, #58886, .F. ) ;
#47568=LINE ( 'NONE', #39094, #32036 ) ;
#47571=CARTESIAN_POINT ( 'NONE',  ( -14.62617646268089899, 15.00000000000000000, 3.327906561566782440 ) ) ;
#47575=CARTESIAN_POINT ( 'NONE',  ( -2.915334737309934532, 7.022018677488174099, -10.88017736071109987 ) ) ;
#47582=PLANE ( 'NONE',  #56013 ) ;
#47583=EDGE_CURVE ( 'NONE', #93734, #63206, #86259, .T. ) ;
#47587=FACE_OUTER_BOUND ( 'NONE', #95341, .T. ) ;
#47588=DIRECTION ( 'NONE',  ( 0.000000000000000000, 1.000000000000000000, 0.000000000000000000 ) ) ;
#47595=ORIENTED_EDGE ( 'NONE', *, *, #50795, .T. ) ;
#47609=VERTEX_POINT ( 'NONE', #17772 ) ;
#47622=CARTESIAN_POINT ( 'NONE',  ( -8.527530157486173934, -13.57440218233254470, 4.923371831947302546 ) ) ;
#47623=EDGE_CURVE ( 'NONE', #94129, #74647, #39783, .T. ) ;
#47624=ORIENTED_EDGE ( 'NONE', *, *, #58886, .T. ) ;
#47625=CARTESIAN_POINT ( 'NONE',  ( 0.000000000000000000, 15.00000000000000000, 0.000000000000000000 ) ) ;
#47627=VERTEX_POINT ( 'NONE', #10754 ) ;
#47633=DIRECTION ( 'NONE',  ( 0.9366721892484018985, 0.000000000000000000, -0.3502073812594559410 ) ) ;
#47638=ORIENTED_EDGE ( 'NONE', *, *, #55589, .T. ) ;
#47640=ORIENTED_EDGE ( 'NONE', *, *, #13652, .T. ) ;
#47652=LINE ( 'NONE', #71637, #26579 ) ;
#47655=CARTESIAN_POINT ( 'NONE',  ( 0.000000000000000000, 0.5000000000000004441, 0.000000000000000000 ) ) ;
#47659=CARTESIAN_POINT ( 'NONE',  ( -14.71525861348286313, 0.3640475087720981273, -2.908807992686782029 ) ) ;
#47662=DIRECTION ( 'NONE',  ( 0.9099612708765483227, 0.000000000000000000, -0.4146932426562279783 ) ) ;
#47664=LINE ( 'NONE', #10649, #15552 ) ;
#47675=EDGE_CURVE ( 'NONE', #4350, #82368, #3561, .T. ) ;
#47683=DIRECTION ( 'NONE',  ( -0.000000000000000000, -1.000000000000000000, -0.000000000000000000 ) ) ;
#47688=CARTESIAN_POINT ( 'NONE',  ( -9.422509992056136596, -36.51964798917849464, 5.440088680355559703 ) ) ;
#47699=VERTEX_POINT ( 'NONE', #79638 ) ;
#47704=CARTESIAN_POINT ( 'NONE',  ( -2.189666204609083788, 15.00000000000000888, -14.46180170876169413 ) ) ;
#47708=VERTEX_POINT ( 'NONE', #48637 ) ;
#47723=DIRECTION ( 'NONE',  ( -0.000000000000000000, 1.000000000000000000, 0.000000000000000000 ) ) ;
#47732=CARTESIAN_POINT ( 'NONE',  ( 0.000000000000000000, 0.000000000000000000, 0.000000000000000000 ) ) ;
#47733=CARTESIAN_POINT ( 'NONE',  ( -12.00809552683946357, 14.49999999999999822, -8.989195838243713155 ) ) ;
#47737=ORIENTED_EDGE ( 'NONE', *, *, #23888, .F. ) ;
#47738=CARTESIAN_POINT ( 'NONE',  ( 0.000000000000000000, 14.49999999999999822, 0.000000000000000000 ) ) ;
#47739=ORIENTED_EDGE ( 'NONE', *, *, #60765, .F. ) ;
#47749=CARTESIAN_POINT ( 'NONE',  ( 12.60589901313222505, 14.49999999999999112, 8.129656208642151327 ) ) ;
#47750=CARTESIAN_POINT ( 'NONE',  ( -9.382169495545422677, -6.501365330069580395, -9.382169495545417348 ) ) ;
#47759=DIRECTION ( 'NONE',  ( 0.000000000000000000, 1.000000000000000000, 0.000000000000000000 ) ) ;
#47761=PLANE ( 'NONE',  #81485 ) ;
#47763=ORIENTED_EDGE ( 'NONE', *, *, #29122, .T. ) ;
#47764=EDGE_CURVE ( 'NONE', #75142, #84080, #73829, .T. ) ;
#47765=CARTESIAN_POINT ( 'NONE',  ( 0.000000000000000000, 0.5000000000000004441, 0.000000000000000000 ) ) ;
#47767=DIRECTION ( 'NONE',  ( -0.000000000000000000, 1.000000000000000000, -0.000000000000000000 ) ) ;
#47771=CARTESIAN_POINT ( 'NONE',  ( -4.838527690343430443, 15.00000000000000000, -14.19819177887733375 ) ) ;
#47781=DIRECTION ( 'NONE',  ( -0.000000000000000000, -1.000000000000000000, -0.000000000000000000 ) ) ;
#47799=FACE_OUTER_BOUND ( 'NONE', #72098, .T. ) ;
#47807=CARTESIAN_POINT ( 'NONE',  ( -6.767445849361338084, 14.63595249122788999, 13.38662304974494077 ) ) ;
#47810=B_SPLINE_CURVE_WITH_KNOTS ( 'NONE', 3,
 ( #57724, #58204, #88227, #58717, #20731, #36726 ),
 .UNSPECIFIED., .F., .F.,
 ( 4, 2, 4 ),
 ( 3.409110551496127980E-05, 0.0004400426677367858127, 0.0008459942299586103998 ),
 .UNSPECIFIED. ) ;
#47811=CARTESIAN_POINT ( 'NONE',  ( -8.564643372776451713, 0.3640475087720985714, -12.31449893000753093 ) ) ;
#47817=CARTESIAN_POINT ( 'NONE',  ( -2.826948239414023067, 14.76930270348881180, 14.67127868811023639 ) ) ;
#47818=CARTESIAN_POINT ( 'NONE',  ( 1.983216688680843109, 15.00000000000000000, 14.11131997956739070 ) ) ;
#47837=DIRECTION ( 'NONE',  ( 0.9636304532086191754, 0.000000000000000000, 0.2672383760782702788 ) ) ;
#47849=EDGE_LOOP ( 'NONE', ( #27108, #28689, #46173, #84983 ) ) ;
#47851=EDGE_CURVE ( 'NONE', #23913, #45067, #10166, .T. ) ;
#47853=EDGE_LOOP ( 'NONE', ( #72962, #6569, #55141, #57572, #52659, #48732 ) ) ;
#47857=DIRECTION ( 'NONE',  ( 0.000000000000000000, 1.000000000000000000, 0.000000000000000000 ) ) ;
#47867=CARTESIAN_POINT ( 'NONE',  ( -14.47650479471824880, 15.00000000000000000, 3.928206833721914482 ) ) ;
#47874=VECTOR ( 'NONE', #49241, 1000.000000000000000 ) ;
#47875=EDGE_CURVE ( 'NONE', #39231, #51116, #34116, .T. ) ;
#47877=FACE_OUTER_BOUND ( 'NONE', #90096, .T. ) ;
#47878=VERTEX_POINT ( 'NONE', #56161 ) ;
#47881=EDGE_CURVE ( 'NONE', #42118, #16779, #18159, .T. ) ;
#47883=EDGE_LOOP ( 'NONE', ( #47152, #96208, #13144, #15031, #41882, #58828 ) ) ;
#47892=DIRECTION ( 'NONE',  ( -0.07845909572783862918, 0.000000000000000000, -0.9969173337331285190 ) ) ;
#47900=CARTESIAN_POINT ( 'NONE',  ( -1.780824192092282265, 14.63606913465075365, -14.89391369643520058 ) ) ;
#47910=CARTESIAN_POINT ( 'NONE',  ( 12.34597252984337956, 14.95037103437615755, -8.076773567935822129 ) ) ;
#47911=CARTESIAN_POINT ( 'NONE',  ( -3.384800920124265033, 0.2306972965111788454, 14.55270344038004815 ) ) ;
#47915=CARTESIAN_POINT ( 'NONE',  ( 10.82344394350231198, 14.95077488074853456, -10.02492699998876979 ) ) ;
#47920=CARTESIAN_POINT ( 'NONE',  ( -14.16423886937409726, -2.987917831752693765, 3.795296366450320757 ) ) ;
#47923=VERTEX_POINT ( 'NONE', #72123 ) ;
#47932=ADVANCED_FACE ( 'NONE', ( #56641 ), #54631, .T. ) ;
#47936=FACE_OUTER_BOUND ( 'NONE', #3555, .T. ) ;
#47943=VECTOR ( 'NONE', #52809, 1000.000000000000000 ) ;
#47947=CARTESIAN_POINT ( 'NONE',  ( -11.36220558719268325, 15.00000000000000000, -9.008345252852777207 ) ) ;
#47971=EDGE_LOOP ( 'NONE', ( #15113, #59763, #43085, #29754, #70137, #42678 ) ) ;
#47976=CIRCLE ( 'NONE', #8093, 14.49999999999999822 ) ;
#47977=CARTESIAN_POINT ( 'NONE',  ( 0.3093388210927642268, 0.5000000000000004441, -14.99680997725065978 ) ) ;
#47982=EDGE_CURVE ( 'NONE', #93214, #25445, #1062, .T. ) ;
#47984=DIRECTION ( 'NONE',  ( 0.000000000000000000, 0.000000000000000000, 1.000000000000000000 ) ) ;
#47988=CARTESIAN_POINT ( 'NONE',  ( 9.846743663894590881, 28.30059781766746951, 2.638427012816828565 ) ) ;
#47989=EDGE_LOOP ( 'NONE', ( #46459, #71738, #66292, #85037 ) ) ;
#48004=EDGE_CURVE ( 'NONE', #53609, #22386, #82590, .T. ) ;
#48005=ORIENTED_EDGE ( 'NONE', *, *, #81318, .T. ) ;
#48007=DIRECTION ( 'NONE',  ( 0.000000000000000000, 0.000000000000000000, 1.000000000000000000 ) ) ;
#48018=ORIENTED_EDGE ( 'NONE', *, *, #67474, .T. ) ;
#48020=DIRECTION ( 'NONE',  ( -0.000000000000000000, -1.000000000000000000, -0.000000000000000000 ) ) ;
#48028=FACE_OUTER_BOUND ( 'NONE', #9648, .T. ) ;
#48029=ORIENTED_EDGE ( 'NONE', *, *, #50484, .T. ) ;
#48034=EDGE_CURVE ( 'NONE', #46342, #46043, #20616, .T. ) ;
#48036=CARTESIAN_POINT ( 'NONE',  ( 0.1034006766821432000, 15.00000000000000000, 14.49963131600458688 ) ) ;
#48051=CARTESIAN_POINT ( 'NONE',  ( 5.440088680355549045, -3.602981322511821016, -9.422509992056141925 ) ) ;
#48055=DIRECTION ( 'NONE',  ( 0.000000000000000000, 0.000000000000000000, 1.000000000000000000 ) ) ;
#48060=TOROIDAL_SURFACE ( 'NONE', #65691, 14.49999999999999822, 0.5000000000000000000 ) ;
#48067=CARTESIAN_POINT ( 'NONE',  ( -8.606322355891181886, 15.00000000000000000, -11.66967075398817322 ) ) ;
#48084=CARTESIAN_POINT ( 'NONE',  ( -9.402796353261216211, 0.3639308891339976815, 11.68706210897754083 ) ) ;
#48088=ORIENTED_EDGE ( 'NONE', *, *, #55233, .T. ) ;
#48098=ADVANCED_FACE ( 'NONE', ( #36096 ), #53065, .T. ) ;
#48103=CARTESIAN_POINT ( 'NONE',  ( 8.527530157486179263, -11.90773551566587329, 4.923371831947292776 ) ) ;
#48106=FACE_OUTER_BOUND ( 'NONE', #26825, .T. ) ;
#48113=EDGE_CURVE ( 'NONE', #18352, #97076, #67601, .T. ) ;
#48115=CIRCLE ( 'NONE', #14592, 14.49999999999999822 ) ;
#48116=DIRECTION ( 'NONE',  ( -0.000000000000000000, -1.000000000000000000, -0.000000000000000000 ) ) ;
#48122=ADVANCED_FACE ( 'NONE', ( #58601 ), #28601, .F. ) ;
#48132=FACE_OUTER_BOUND ( 'NONE', #98246, .T. ) ;
#48133=CONICAL_SURFACE ( 'NONE', #294, 13.74999999999999467, 0.7853981633974458365 ) ;
#48141=B_SPLINE_CURVE_WITH_KNOTS ( 'NONE', 3,
 ( #85686, #70691, #16702, #20012, #17693, #73006 ),
 .UNSPECIFIED., .F., .F.,
 ( 4, 2, 4 ),
 ( 0.0002800015744458473265, 0.0006862068192651732488, 0.001092412064084499279 ),
 .UNSPECIFIED. ) ;
#48150=AXIS2_PLACEMENT_3D ( 'NONE', #13101, #29567, #6590 ) ;
#48156=CARTESIAN_POINT ( 'NONE',  ( 0.000000000000000000, 14.49999999999999822, 0.000000000000000000 ) ) ;
#48157=ORIENTED_EDGE ( 'NONE', *, *, #68322, .F. ) ;
#48159=CARTESIAN_POINT ( 'NONE',  ( 3.927832320392154575, 0.000000000000000000, 13.69797916712106733 ) ) ;
#48163=CARTESIAN_POINT ( 'NONE',  ( 13.86186289918443215, 15.00000000000000888, -4.667665767314964853 ) ) ;
#48165=CARTESIAN_POINT ( 'NONE',  ( -14.48718990079891888, 15.00000000000000000, -0.6093675230842395818 ) ) ;
#48169=CARTESIAN_POINT ( 'NONE',  ( -5.440088680355558814, -37.76964798917849464, -9.422509992056136596 ) ) ;
#48173=EDGE_CURVE ( 'NONE', #82904, #44178, #6106, .T. ) ;
#48180=CIRCLE ( 'NONE', #91370, 14.49999999999999822 ) ;
#48181=VERTEX_POINT ( 'NONE', #81592 ) ;
#48192=VERTEX_POINT ( 'NONE', #51607 ) ;
#48202=VERTEX_POINT ( 'NONE', #13103 ) ;
#48203=AXIS2_PLACEMENT_3D ( 'NONE', #43918, #73433, #65935 ) ;
#48206=ORIENTED_EDGE ( 'NONE', *, *, #23390, .F. ) ;
#48208=ORIENTED_EDGE ( 'NONE', *, *, #33440, .F. ) ;
#48210=CARTESIAN_POINT ( 'NONE',  ( -5.378451019861586246, 0.000000000000000000, -0.9000440264803170054 ) ) ;
#48214=CARTESIAN_POINT ( 'NONE',  ( 0.000000000000000000, 15.00000000000000000, -11.25000000000000178 ) ) ;
#48217=CARTESIAN_POINT ( 'NONE',  ( 11.35178980618974087, 0.5000000000000004441, -9.804941009311923139 ) ) ;
#48218=ADVANCED_FACE ( 'NONE', ( #82091 ), #9977, .T. ) ;
#48220=FACE_OUTER_BOUND ( 'NONE', #3346, .T. ) ;
#48221=AXIS2_PLACEMENT_3D ( 'NONE', #15903, #29898, #7913 ) ;
#48230=VERTEX_POINT ( 'NONE', #83084 ) ;
#48236=DIRECTION ( 'NONE',  ( 0.4924235601034648302, -0.000000000000000000, 0.8703556959399010307 ) ) ;
#48237=VERTEX_POINT ( 'NONE', #5620 ) ;
#48239=B_SPLINE_CURVE_WITH_KNOTS ( 'NONE', 3,
 ( #83292, #53279, #38296, #61270, #23795, #83785 ),
 .UNSPECIFIED., .F., .F.,
 ( 4, 2, 4 ),
 ( 3.409110551485654587E-05, 0.0004400426677367037386, 0.0008459942299585509855 ),
 .UNSPECIFIED. ) ;
#48240=CARTESIAN_POINT ( 'NONE',  ( -9.382169495545422677, -1.501365330069578619, -9.382169495545417348 ) ) ;
#48243=VERTEX_POINT ( 'NONE', #90575 ) ;
#48245=ORIENTED_EDGE ( 'NONE', *, *, #81318, .F. ) ;
#48248=CARTESIAN_POINT ( 'NONE',  ( 14.88232117145534339, 0.3639310251205937208, -1.875237731503157645 ) ) ;
#48254=DIRECTION ( 'NONE',  ( -0.000000000000000000, -1.000000000000000000, -0.000000000000000000 ) ) ;
#48272=CIRCLE ( 'NONE', #5180, 15.00000000000000000 ) ;
#48274=SURFACE_SIDE_STYLE ('',( #70312 ) ) ;
#48283=CARTESIAN_POINT ( 'NONE',  ( -5.817157072110894944, 14.49999999999999112, 13.82608706751089755 ) ) ;
#48284=B_SPLINE_CURVE_WITH_KNOTS ( 'NONE', 3,
 ( #77549, #63047, #93543, #62543, #25564, #48036 ),
 .UNSPECIFIED., .F., .F.,
 ( 4, 2, 4 ),
 ( 3.409110551496215394E-05, 0.0004400426677368006120, 0.0008459942299586391311 ),
 .UNSPECIFIED. ) ;
#48288=TOROIDAL_SURFACE ( 'NONE', #6773, 14.49999999999999822, 0.5000000000000000000 ) ;
#48290=CARTESIAN_POINT ( 'NONE',  ( -5.810202895580280469, 0.04922511925147063372, -13.56051778013773479 ) ) ;
#48291=CYLINDRICAL_SURFACE ( 'NONE', #6578, 15.00000000000000000 ) ;
#48295=AXIS2_PLACEMENT_3D ( 'NONE', #92435, #16453, #10307 ) ;
#48297=ORIENTED_EDGE ( 'NONE', *, *, #38242, .T. ) ;
#48305=PLANE ( 'NONE',  #46659 ) ;
#48308=EDGE_LOOP ( 'NONE', ( #1089, #25066, #36079, #77436 ) ) ;
#48348=TOROIDAL_SURFACE ( 'NONE', #30710, 14.49999999999999822, 0.5000000000000000000 ) ;
#48359=ORIENTED_EDGE ( 'NONE', *, *, #311, .T. ) ;
#48362=ORIENTED_EDGE ( 'NONE', *, *, #96197, .T. ) ;
#48364=CIRCLE ( 'NONE', #54714, 14.49999999999999822 ) ;
#48368=CARTESIAN_POINT ( 'NONE',  ( 6.382347221874338672, 14.63595249122789177, 13.57444820018232434 ) ) ;
#48373=DIRECTION ( 'NONE',  ( -0.000000000000000000, -1.000000000000000000, -0.000000000000000000 ) ) ;
#48377=ORIENTED_EDGE ( 'NONE', *, *, #78386, .F. ) ;
#48378=VECTOR ( 'NONE', #51312, 1000.000000000000000 ) ;
#48394=ORIENTED_EDGE ( 'NONE', *, *, #26632, .F. ) ;
#48395=AXIS2_PLACEMENT_3D ( 'NONE', #16300, #92774, #60311 ) ;
#48403=CARTESIAN_POINT ( 'NONE',  ( 0.000000000000000000, 0.5000000000000004441, 0.000000000000000000 ) ) ;
#48418=CARTESIAN_POINT ( 'NONE',  ( 3.469446951953614189E-15, 13.05374883491396787, 14.16423886937410259 ) ) ;
#48425=DIRECTION ( 'NONE',  ( -1.776356839400250465E-15, 0.000000000000000000, 1.000000000000000000 ) ) ;
#48427=CIRCLE ( 'NONE', #26106, 15.00000000000000000 ) ;
#48439=AXIS2_PLACEMENT_3D ( 'NONE', #30003, #67033, #91002 ) ;
#48441=LINE ( 'NONE', #56922, #13860 ) ;
#48447=LINE ( 'NONE', #77460, #16175 ) ;
#48455=DIRECTION ( 'NONE',  ( -0.000000000000000000, -1.000000000000000000, -0.000000000000000000 ) ) ;
#48465=ORIENTED_EDGE ( 'NONE', *, *, #57686, .T. ) ;
#48483=CARTESIAN_POINT ( 'NONE',  ( -5.204170427930421283E-15, -27.12636533006957507, -12.81628187352647608 ) ) ;
#48484=VERTEX_POINT ( 'NONE', #84078 ) ;
#48494=AXIS2_PLACEMENT_3D ( 'NONE', #4203, #2747, #41230 ) ;
#48496=ORIENTED_EDGE ( 'NONE', *, *, #3302, .T. ) ;
#48499=EDGE_CURVE ( 'NONE', #20656, #38087, #19024, .T. ) ;
#48504=CARTESIAN_POINT ( 'NONE',  ( -10.64017930668191170, 0.5000000000000004441, -10.57291749337230158 ) ) ;
#48506=CARTESIAN_POINT ( 'NONE',  ( -4.856092091438414471, -2.729140156053354904E-15, 13.79590085420550061 ) ) ;
#48509=VERTEX_POINT ( 'NONE', #49501 ) ;
#48512=VERTEX_POINT ( 'NONE', #12008 ) ;
#48530=EDGE_CURVE ( 'NONE', #7679, #37275, #19510, .T. ) ;
#48532=CARTESIAN_POINT ( 'NONE',  ( -5.204170427930421283E-15, -39.44625116508603213, -14.16423886937410082 ) ) ;
#48535=ORIENTED_EDGE ( 'NONE', *, *, #61373, .T. ) ;
#48536=ORIENTED_EDGE ( 'NONE', *, *, #81374, .F. ) ;
#48548=CARTESIAN_POINT ( 'NONE',  ( -2.915334737309917656, 4.105352010821503583, 10.88017736071110164 ) ) ;
#48553=FACE_OUTER_BOUND ( 'NONE', #37530, .T. ) ;
#48556=DIRECTION ( 'NONE',  ( -0.000000000000000000, -1.000000000000000000, -0.000000000000000000 ) ) ;
#48563=CARTESIAN_POINT ( 'NONE',  ( 0.000000000000000000, 0.000000000000000000, 0.000000000000000000 ) ) ;
#48578=CARTESIAN_POINT ( 'NONE',  ( -8.564643372776458818, 14.63606914147517735, -12.31449893000756468 ) ) ;
#48592=CARTESIAN_POINT ( 'NONE',  ( 0.000000000000000000, 0.000000000000000000, 0.000000000000000000 ) ) ;
#48594=CARTESIAN_POINT ( 'NONE',  ( -7.208316651077764980, -14.61606884899921077, -7.208316651077759651 ) ) ;
#48600=ORIENTED_EDGE ( 'NONE', *, *, #65382, .F. ) ;
#48608=CARTESIAN_POINT ( 'NONE',  ( -9.820177974736479243, 14.76984956101180835, 11.25994418464046198 ) ) ;
#48615=ORIENTED_EDGE ( 'NONE', *, *, #80844, .F. ) ;
#48621=EDGE_LOOP ( 'NONE', ( #6673, #70736, #79119, #4452 ) ) ;
#48625=VERTEX_POINT ( 'NONE', #4031 ) ;
#48629=DIRECTION ( 'NONE',  ( 0.000000000000000000, 1.000000000000000000, 0.000000000000000000 ) ) ;
#48634=CARTESIAN_POINT ( 'NONE',  ( 7.993487411949270260, 0.04962888323599794205, 12.40005926694712990 ) ) ;
#48637=CARTESIAN_POINT ( 'NONE',  ( 6.689969769698871360, 15.00000000000000000, 12.58200319823975022 ) ) ;
#48638=ORIENTED_EDGE ( 'NONE', *, *, #95617, .F. ) ;
#48645=B_SPLINE_CURVE_WITH_KNOTS ( 'NONE', 3,
 ( #74435, #21455, #82936, #21957, #14453, #27463 ),
 .UNSPECIFIED., .F., .F.,
 ( 4, 2, 4 ),
 ( 3.409110551496048698E-05, 0.0004400426677367984978, 0.0008459942299586365290 ),
 .UNSPECIFIED. ) ;
#48649=ADVANCED_FACE ( 'NONE', ( #48028 ), #89820, .T. ) ;
#48650=EDGE_CURVE ( 'NONE', #75691, #73066, #67500, .T. ) ;
#48657=CARTESIAN_POINT ( 'NONE',  ( 10.93781366033347169, 0.5000000000000004441, -10.26470809774065351 ) ) ;
#48661=CARTESIAN_POINT ( 'NONE',  ( 3.469446951953614189E-15, -35.68631465584515894, 10.88017736071110342 ) ) ;
#48664=DIRECTION ( 'NONE',  ( 0.000000000000000000, 0.000000000000000000, 1.000000000000000000 ) ) ;
#48680=CARTESIAN_POINT ( 'NONE',  ( 14.40939250469964961, 15.00000000000000000, 1.618458416365853747 ) ) ;
#48685=EDGE_CURVE ( 'NONE', #33923, #34058, #5261, .T. ) ;
#48686=CARTESIAN_POINT ( 'NONE',  ( 12.35505582470273644, 15.00000000000000000, -10.16021613965630443 ) ) ;
#48697=EDGE_LOOP ( 'NONE', ( #38342, #28858, #3814, #4222, #10180, #7072 ) ) ;
#48698=ORIENTED_EDGE ( 'NONE', *, *, #20227, .T. ) ;
#48699=DIRECTION ( 'NONE',  ( 0.000000000000000000, 0.000000000000000000, 1.000000000000000000 ) ) ;
#48713=DIRECTION ( 'NONE',  ( 0.000000000000000000, 1.000000000000000000, 0.000000000000000000 ) ) ;
#48718=CARTESIAN_POINT ( 'NONE',  ( 0.9940297508536876103, -0.03417435944610275333, 14.21528771620250353 ) ) ;
#48726=CARTESIAN_POINT ( 'NONE',  ( 14.49440716394873263, 4.853942851202206293E-16, 0.4026921475167233311 ) ) ;
#48727=AXIS2_PLACEMENT_3D ( 'NONE', #24232, #32192, #86693 ) ;
#48728=CARTESIAN_POINT ( 'NONE',  ( 6.408140936763236262, -2.543031996736243361, -11.09922568453595026 ) ) ;
#48732=ORIENTED_EDGE ( 'NONE', *, *, #32163, .F. ) ;
#48737=LINE ( 'NONE', #35709, #19186 ) ;
#48740=EDGE_CURVE ( 'NONE', #54629, #23697, #60557, .T. ) ;
#48743=CARTESIAN_POINT ( 'NONE',  ( 0.000000000000000000, 0.5000000000000004441, 0.000000000000000000 ) ) ;
#48745=CARTESIAN_POINT ( 'NONE',  ( 1.847340224724850932, 14.95077488074853456, -14.63671528203490979 ) ) ;
#48748=PLANE ( 'NONE',  #1998 ) ;
#48749=TOROIDAL_SURFACE ( 'NONE', #43968, 14.49999999999999822, 0.5000000000000000000 ) ;
#48755=CARTESIAN_POINT ( 'NONE',  ( 14.29730467489532408, 4.491438197698105257E-16, 2.416004766803315995 ) ) ;
#48758=EDGE_CURVE ( 'NONE', #60661, #47206, #87992, .T. ) ;
#48764=AXIS2_PLACEMENT_3D ( 'NONE', #93976, #24516, #85993 ) ;
#48768=EDGE_CURVE ( 'NONE', #62241, #86312, #74901, .T. ) ;
#48771=VERTEX_POINT ( 'NONE', #65986 ) ;
#48779=CARTESIAN_POINT ( 'NONE',  ( 14.94699059465100888, 0.5000000000000004441, 1.259949270174915981 ) ) ;
#48782=CARTESIAN_POINT ( 'NONE',  ( 6.382347221874334231, 15.00000000000000000, 13.57444820018231724 ) ) ;
#48791=FACE_OUTER_BOUND ( 'NONE', #61987, .T. ) ;
#48799=VERTEX_POINT ( 'NONE', #58481 ) ;
#48801=LINE ( 'NONE', #33777, #7948 ) ;
#48807=CARTESIAN_POINT ( 'NONE',  ( -7.674335239599113123, 0.2306972965111898366, -12.81961907869226991 ) ) ;
#48829=ORIENTED_EDGE ( 'NONE', *, *, #70118, .F. ) ;
#48832=ORIENTED_EDGE ( 'NONE', *, *, #40681, .F. ) ;
#48850=ORIENTED_EDGE ( 'NONE', *, *, #22611, .F. ) ;
#48852=ORIENTED_EDGE ( 'NONE', *, *, #57142, .F. ) ;
#48856=CARTESIAN_POINT ( 'NONE',  ( -13.48255862861931043, 4.084149796850864849E-16, 5.335786055104065007 ) ) ;
#48857=CARTESIAN_POINT ( 'NONE',  ( 6.091055032734291608, 15.00000000000000888, 13.29802223412760753 ) ) ;
#48866=VERTEX_POINT ( 'NONE', #36490 ) ;
#48875=CARTESIAN_POINT ( 'NONE',  ( -13.14228782657330896, 14.63595249122789177, -7.230509711182420141 ) ) ;
#48878=FACE_OUTER_BOUND ( 'NONE', #28591, .T. ) ;
#48906=CARTESIAN_POINT ( 'NONE',  ( 10.36894250292378850, -0.07125116508603752952, -10.36894250292379027 ) ) ;
#48909=TOROIDAL_SURFACE ( 'NONE', #87234, 14.49999999999999822, 0.5000000000000000000 ) ;
#48910=VERTEX_POINT ( 'NONE', #69943 ) ;
#48913=LINE ( 'NONE', #17458, #82178 ) ;
#48924=CARTESIAN_POINT ( 'NONE',  ( 12.83294900548066053, 0.3639312116172450096, -7.766300266068392411 ) ) ;
#48936=CIRCLE ( 'NONE', #95251, 14.49999999999999822 ) ;
#48943=ORIENTED_EDGE ( 'NONE', *, *, #47163, .T. ) ;
#48953=VERTEX_POINT ( 'NONE', #67974 ) ;
#48954=AXIS2_PLACEMENT_3D ( 'NONE', #39667, #62628, #4495 ) ;
#48958=ORIENTED_EDGE ( 'NONE', *, *, #81770, .F. ) ;
#48959=CARTESIAN_POINT ( 'NONE',  ( 12.74305857943745046, -3.163668057994810583E-15, 7.177950183686947483 ) ) ;
#48962=CYLINDRICAL_SURFACE ( 'NONE', #39454, 11.25000000000000178 ) ;
#48964=LINE ( 'NONE', #10973, #25308 ) ;
#48968=B_SPLINE_CURVE_WITH_KNOTS ( 'NONE', 3,
 ( #76383, #37910, #75890, #63209, #7898, #6904 ),
 .UNSPECIFIED., .F., .F.,
 ( 4, 2, 4 ),
 ( 3.409110551494651432E-05, 0.0004400426677367925347, 0.0008459942299586384806 ),
 .UNSPECIFIED. ) ;
#48970=AXIS2_PLACEMENT_3D ( 'NONE', #97561, #30504, #29024 ) ;
#48973=CARTESIAN_POINT ( 'NONE',  ( 0.000000000000000000, 14.49999999999999822, 0.000000000000000000 ) ) ;
#48975=CARTESIAN_POINT ( 'NONE',  ( 3.469446951953614189E-15, -29.62636533006957862, 12.81628187352647608 ) ) ;
#48984=EDGE_CURVE ( 'NONE', #82368, #79612, #55778, .T. ) ;
#48985=CYLINDRICAL_SURFACE ( 'NONE', #68223, 15.00000000000000000 ) ;
#48987=VECTOR ( 'NONE', #84681, 1000.000000000000000 ) ;
#49001=LINE ( 'NONE', #94499, #93487 ) ;
#49006=CARTESIAN_POINT ( 'NONE',  ( 5.815488105659666118, 14.76984994604921475, 13.76235181012722286 ) ) ;
#49010=ORIENTED_EDGE ( 'NONE', *, *, #48034, .T. ) ;
#49011=CARTESIAN_POINT ( 'NONE',  ( -12.22506292814027873, 14.76930270348881002, 8.589871424854626625 ) ) ;
#49020=ORIENTED_EDGE ( 'NONE', *, *, #88474, .F. ) ;
#49031=CARTESIAN_POINT ( 'NONE',  ( 14.16423886937410259, -35.69625116508602503, -2.602085213965210642E-15 ) ) ;
#49035=VERTEX_POINT ( 'NONE', #75957 ) ;
#49036=CIRCLE ( 'NONE', #2817, 11.25000000000000178 ) ;
#49043=CARTESIAN_POINT ( 'NONE',  ( -9.402796353260967521, 15.00000000000000000, -11.68706210897770248 ) ) ;
#49045=CARTESIAN_POINT ( 'NONE',  ( -6.767445849361338972, 0.3639308223168559175, 13.38662304974495854 ) ) ;
#49050=CARTESIAN_POINT ( 'NONE',  ( -10.88017736071110164, 17.85535201082151247, -2.915334737309917212 ) ) ;
#49053=LINE ( 'NONE', #43389, #31841 ) ;
#49054=EDGE_CURVE ( 'NONE', #2122, #18620, #50568, .T. ) ;
#49055=CARTESIAN_POINT ( 'NONE',  ( 0.000000000000000000, 15.00000000000000000, 0.000000000000000000 ) ) ;
#49056=PLANE ( 'NONE',  #75187 ) ;
#49060=CARTESIAN_POINT ( 'NONE',  ( 8.731067818237036704, 11.56330936912750573, 8.731067818237033151 ) ) ;
#49062=AXIS2_PLACEMENT_3D ( 'NONE', #63524, #32536, #63034 ) ;
#49078=CARTESIAN_POINT ( 'NONE',  ( -5.448048636097846398, 0.000000000000000000, 0.2378669404634123075 ) ) ;
#49094=FACE_OUTER_BOUND ( 'NONE', #21069, .T. ) ;
#49095=CARTESIAN_POINT ( 'NONE',  ( -4.923371831947292776, 1.842264484334124486, 8.527530157486181039 ) ) ;
#49098=CARTESIAN_POINT ( 'NONE',  ( 0.000000000000000000, 14.49999999999999822, 0.000000000000000000 ) ) ;
#49099=ORIENTED_EDGE ( 'NONE', *, *, #29211, .T. ) ;
#49105=CARTESIAN_POINT ( 'NONE',  ( -9.876730923139437124, 14.49999999999999112, 11.28938378619059613 ) ) ;
#49107=B_SPLINE_CURVE_WITH_KNOTS ( 'NONE', 3,
 ( #98269, #16218, #98766, #259, #36756, #60720 ),
 .UNSPECIFIED., .F., .F.,
 ( 4, 2, 4 ),
 ( 0.0002800170536516726491, 0.0006862224498868382903, 0.001092427846122004040 ),
 .UNSPECIFIED. ) ;
#49108=B_SPLINE_CURVE_WITH_KNOTS ( 'NONE', 3,
 ( #55303, #63772, #61817, #48290, #39336, #85813 ),
 .UNSPECIFIED., .F., .F.,
 ( 4, 2, 4 ),
 ( 3.409110551496102908E-05, 0.0004400426677367863006, 0.0008459942299586115924 ),
 .UNSPECIFIED. ) ;
#49111=ORIENTED_EDGE ( 'NONE', *, *, #22611, .T. ) ;
#49125=EDGE_LOOP ( 'NONE', ( #92532, #5608, #45637, #41370, #39629, #61755 ) ) ;
#49130=ADVANCED_FACE ( 'NONE', ( #71427 ), #18038, .T. ) ;
#49136=DIRECTION ( 'NONE',  ( 0.000000000000000000, 1.000000000000000000, 0.000000000000000000 ) ) ;
#49149=ORIENTED_EDGE ( 'NONE', *, *, #47254, .F. ) ;
#49156=LINE ( 'NONE', #41187, #96486 ) ;
#49160=CARTESIAN_POINT ( 'NONE',  ( 5.440088680355556150, -20.26964798917849109, 9.422509992056138373 ) ) ;
#49166=ADVANCED_FACE ( 'NONE', ( #71895 ), #16940, .F. ) ;
#49176=CARTESIAN_POINT ( 'NONE',  ( 14.52844422123120616, 15.00000000000000533, 1.683098224408404953 ) ) ;
#49189=DIRECTION ( 'NONE',  ( 0.7253743710122775301, 0.000000000000000000, 0.6883545756937645699 ) ) ;
#49192=CIRCLE ( 'NONE', #95522, 14.49999999999999822 ) ;
#49193=CARTESIAN_POINT ( 'NONE',  ( -4.838527690343428667, 0.3640475087720985714, -14.19819177887734440 ) ) ;
#49196=DIRECTION ( 'NONE',  ( 0.000000000000000000, 1.000000000000000000, 0.000000000000000000 ) ) ;
#49201=CARTESIAN_POINT ( 'NONE',  ( 13.21236992757673789, -0.03417435944610275333, -5.338143956176714333 ) ) ;
#49206=DIRECTION ( 'NONE',  ( 0.06104853953486361756, 0.000000000000000000, -0.9981347984218665870 ) ) ;
#49211=CARTESIAN_POINT ( 'NONE',  ( 4.923371831947295441, -35.65773551566588395, -8.527530157486179263 ) ) ;
#49219=VECTOR ( 'NONE', #28288, 1000.000000000000114 ) ;
#49220=DIRECTION ( 'NONE',  ( -0.8526401643540884034, 0.000000000000000000, -0.5224985647159552382 ) ) ;
#49222=CIRCLE ( 'NONE', #63619, 14.49999999999999822 ) ;
#49226=EDGE_CURVE ( 'NONE', #26337, #97969, #81971, .T. ) ;
#49227=CARTESIAN_POINT ( 'NONE',  ( -3.434112377981047626, -9.834698663402914320, 12.81628187352647963 ) ) ;
#49231=ORIENTED_EDGE ( 'NONE', *, *, #63487, .T. ) ;
#49239=ORIENTED_EDGE ( 'NONE', *, *, #10295, .F. ) ;
#49241=DIRECTION ( 'NONE',  ( 0.000000000000000000, 1.000000000000000000, 0.000000000000000000 ) ) ;
#49249=VECTOR ( 'NONE', #2355, 1000.000000000000000 ) ;
#49256=CARTESIAN_POINT ( 'NONE',  ( -14.15369600240084225, 7.013432803265604835E-16, -3.689340892730420762 ) ) ;
#49265=CARTESIAN_POINT ( 'NONE',  ( -12.60874940350953111, 15.00000000000000000, 7.160268045226944267 ) ) ;
#49278=CARTESIAN_POINT ( 'NONE',  ( -12.00809552683965187, 0.5000000000000004441, 8.989195838243462688 ) ) ;
#49280=EDGE_CURVE ( 'NONE', #16647, #60661, #65908, .T. ) ;
#49281=AXIS2_PLACEMENT_3D ( 'NONE', #9780, #54766, #17292 ) ;
#49294=ORIENTED_EDGE ( 'NONE', *, *, #1437, .F. ) ;
#49305=CARTESIAN_POINT ( 'NONE',  ( 0.000000000000000000, 0.5000000000000004441, 0.000000000000000000 ) ) ;
#49319=DIRECTION ( 'NONE',  ( -0.9636304532086248376, 0.000000000000000000, 0.2672383760782501838 ) ) ;
#49322=VECTOR ( 'NONE', #34160, 1000.000000000000000 ) ;
#49327=VERTEX_POINT ( 'NONE', #85432 ) ;
#49328=CARTESIAN_POINT ( 'NONE',  ( -10.70613742633263321, 15.00000000000000000, 9.778988772285140740 ) ) ;
#49330=ORIENTED_EDGE ( 'NONE', *, *, #52075, .T. ) ;
#49332=EDGE_CURVE ( 'NONE', #65562, #14583, #3366, .T. ) ;
#49335=CARTESIAN_POINT ( 'NONE',  ( 0.000000000000000000, 35.00000000000000000, -11.92686044187656513 ) ) ;
#49343=EDGE_LOOP ( 'NONE', ( #45935, #67596, #90576, #48698, #23023, #84200 ) ) ;
#49345=VERTEX_POINT ( 'NONE', #78416 ) ;
#49353=EDGE_CURVE ( 'NONE', #87486, #44443, #10422, .T. ) ;
#49357=DIRECTION ( 'NONE',  ( 0.000000000000000000, 0.000000000000000000, 1.000000000000000000 ) ) ;
#49362=ORIENTED_EDGE ( 'NONE', *, *, #17959, .F. ) ;
#49370=FACE_OUTER_BOUND ( 'NONE', #37083, .T. ) ;
#49376=EDGE_CURVE ( 'NONE', #65168, #85153, #37914, .T. ) ;
#49394=AXIS2_PLACEMENT_3D ( 'NONE', #41075, #66885, #96416 ) ;
#49412=EDGE_CURVE ( 'NONE', #23105, #3928, #33922, .T. ) ;
#49414=LINE ( 'NONE', #20414, #55947 ) ;
#49419=DIRECTION ( 'NONE',  ( -0.9990482215818579093, 0.000000000000000000, 0.04361938736533305799 ) ) ;
#49422=EDGE_CURVE ( 'NONE', #65076, #23913, #33991, .T. ) ;
#49429=CARTESIAN_POINT ( 'NONE',  ( -5.815488105659576412, 14.76984994604921475, -13.76235181012726549 ) ) ;
#49437=AXIS2_PLACEMENT_3D ( 'NONE', #95419, #65398, #74374 ) ;
#49445=ORIENTED_EDGE ( 'NONE', *, *, #80497, .F. ) ;
#49448=EDGE_CURVE ( 'NONE', #67150, #75159, #5392, .T. ) ;
#49451=DIRECTION ( 'NONE',  ( 1.776356839400250465E-15, 0.000000000000000000, 1.000000000000000000 ) ) ;
#49456=EDGE_CURVE ( 'NONE', #51188, #43096, #85128, .T. ) ;
#49460=CARTESIAN_POINT ( 'NONE',  ( 12.81628187352647252, -38.16803199673624647, -3.434112377981059172 ) ) ;
#49489=CARTESIAN_POINT ( 'NONE',  ( 5.810213597521703299, 14.95037102642602278, 13.56092647078875224 ) ) ;
#49493=FACE_OUTER_BOUND ( 'NONE', #25727, .T. ) ;
#49496=CARTESIAN_POINT ( 'NONE',  ( 2.393480905993071062, 0.3639310596586424751, 14.80781041047755942 ) ) ;
#49501=CARTESIAN_POINT ( 'NONE',  ( 14.99847009497950800, 14.49999999999999112, -0.2142307401080081053 ) ) ;
#49508=VECTOR ( 'NONE', #41986, 1000.000000000000227 ) ;
#49509=CARTESIAN_POINT ( 'NONE',  ( 0.000000000000000000, 15.00000000000000000, 0.000000000000000000 ) ) ;
#49511=CARTESIAN_POINT ( 'NONE',  ( -10.36894250292379205, -38.82125116508603924, -10.36894250292378672 ) ) ;
#49527=CARTESIAN_POINT ( 'NONE',  ( 5.440088680355549045, 16.39701867748817676, -9.422509992056141925 ) ) ;
#49540=CARTESIAN_POINT ( 'NONE',  ( -9.011287250621620615, 14.76930270348882068, -11.91783356064799726 ) ) ;
#49554=EDGE_LOOP ( 'NONE', ( #5447, #36077, #86062, #46758 ) ) ;
#49562=LINE ( 'NONE', #65551, #41888 ) ;
#49571=CARTESIAN_POINT ( 'NONE',  ( 8.527530157486175710, -1.074402182332540034, -4.923371831947298993 ) ) ;
#49575=VECTOR ( 'NONE', #88705, 1000.000000000000000 ) ;
#49583=VERTEX_POINT ( 'NONE', #36864 ) ;
#49586=ORIENTED_EDGE ( 'NONE', *, *, #82899, .F. ) ;
#49593=B_SPLINE_CURVE_WITH_KNOTS ( 'NONE', 3,
 ( #45405, #38417, #60902, #30895, #53399, #84893 ),
 .UNSPECIFIED., .F., .F.,
 ( 4, 2, 4 ),
 ( 3.409110551495941633E-05, 0.0004400426677367835358, 0.0008459942299586075808 ),
 .UNSPECIFIED. ) ;
#49597=VECTOR ( 'NONE', #71164, 1000.000000000000000 ) ;
#49599=VERTEX_POINT ( 'NONE', #53834 ) ;
#49606=CYLINDRICAL_SURFACE ( 'NONE', #71564, 11.92686044187656513 ) ;
#49610=CARTESIAN_POINT ( 'NONE',  ( 0.000000000000000000, 0.5000000000000004441, 0.000000000000000000 ) ) ;
#49629=CARTESIAN_POINT ( 'NONE',  ( 10.44173051747104708, 12.78704354326105275, -4.918064008119704233 ) ) ;
#49631=CARTESIAN_POINT ( 'NONE',  ( 0.000000000000000000, 0.5000000000000004441, 0.000000000000000000 ) ) ;
#49636=CARTESIAN_POINT ( 'NONE',  ( 5.440088680355556150, -30.26964798917849109, 9.422509992056138373 ) ) ;
#49640=DIRECTION ( 'NONE',  ( 0.000000000000000000, 0.000000000000000000, 1.000000000000000000 ) ) ;
#49647=B_SPLINE_CURVE_WITH_KNOTS ( 'NONE', 3,
 ( #57141, #19151, #26645, #96145, #88129, #19641, #3669, #55681, #4159, #87637, #49629, #34626, #94158, #50134, #79655, #11153, #80138, #71665, #56657, #11648, #3175, #17691, #25684, #33640 ),
 .UNSPECIFIED., .F., .F.,
 ( 4, 2, 2, 2, 2, 2, 2, 2, 2, 2, 2, 4 ),
 ( 0.000000000000000000, 0.002011827134370535418, 0.003017740701555803127, 0.004023654268741070836, 0.006035481403111603652, 0.007041394970296870927, 0.008047308537482138202, 0.01005913567185267796, 0.01106504923903794783, 0.01207096280622321945, 0.01408278994059376787, 0.01609461707496431804 ),
 .UNSPECIFIED. ) ;
#49652=DIRECTION ( 'NONE',  ( 0.6755902076156591329, 0.000000000000000000, -0.7372773368101250835 ) ) ;
#49657=DIRECTION ( 'NONE',  ( 0.000000000000000000, 0.000000000000000000, 1.000000000000000000 ) ) ;
#49661=DIRECTION ( 'NONE',  ( -0.000000000000000000, 1.000000000000000000, -0.000000000000000000 ) ) ;
#49665=CARTESIAN_POINT ( 'NONE',  ( 10.93781366033347169, 15.00000000000000000, -10.26470809774065351 ) ) ;
#49667=ADVANCED_FACE ( 'NONE', ( #95279 ), #9830, .F. ) ;
#49670=ORIENTED_EDGE ( 'NONE', *, *, #36258, .F. ) ;
#49672=VERTEX_POINT ( 'NONE', #87285 ) ;
#49674=VECTOR ( 'NONE', #7988, 1000.000000000000000 ) ;
#49675=CARTESIAN_POINT ( 'NONE',  ( 6.382347221874359988, 0.3639313913011580359, 13.57444820018234388 ) ) ;
#49688=CARTESIAN_POINT ( 'NONE',  ( 0.000000000000000000, 15.00000000000000000, 0.000000000000000000 ) ) ;
#49690=EDGE_CURVE ( 'NONE', #28000, #39649, #15239, .T. ) ;
#49691=CARTESIAN_POINT ( 'NONE',  ( -7.208316651077764980, -34.61606884899921965, -7.208316651077759651 ) ) ;
#49692=ORIENTED_EDGE ( 'NONE', *, *, #61077, .F. ) ;
#49693=LINE ( 'NONE', #4221, #23614 ) ;
#49700=AXIS2_PLACEMENT_3D ( 'NONE', #37519, #90005, #83505 ) ;
#49704=CARTESIAN_POINT ( 'NONE',  ( -11.09922568453595382, 8.706968003263760636, -6.408140936763226492 ) ) ;
#49707=VERTEX_POINT ( 'NONE', #56314 ) ;
#49716=EDGE_CURVE ( 'NONE', #26946, #89452, #30794, .T. ) ;
#49726=EDGE_CURVE ( 'NONE', #93626, #12985, #46214, .T. ) ;
#49738=CARTESIAN_POINT ( 'NONE',  ( 9.876730923139298568, 0.5000000000000004441, -11.28938378619063165 ) ) ;
#49746=VERTEX_POINT ( 'NONE', #72764 ) ;
#49751=CARTESIAN_POINT ( 'NONE',  ( 9.399392868737718842, 15.00000000000000000, 11.04089732309479110 ) ) ;
#49758=CARTESIAN_POINT ( 'NONE',  ( 0.000000000000000000, 15.00000000000000000, 0.000000000000000000 ) ) ;
#49771=EDGE_CURVE ( 'NONE', #25131, #48799, #94027, .T. ) ;
#49773=CARTESIAN_POINT ( 'NONE',  ( -6.715867195167532167, 15.00000000000000000, 12.85095824508320028 ) ) ;
#49776=CARTESIAN_POINT ( 'NONE',  ( 11.03499054390001533, 2.041642599432720750, 4.094770669169175648 ) ) ;
#49779=FACE_OUTER_BOUND ( 'NONE', #68764, .T. ) ;
#49782=ORIENTED_EDGE ( 'NONE', *, *, #95410, .T. ) ;
#49788=DIRECTION ( 'NONE',  ( 0.9981347984218670311, 0.000000000000000000, -0.06104853953485662316 ) ) ;
#49793=TOROIDAL_SURFACE ( 'NONE', #81691, 14.49999999999999822, 0.5000000000000000000 ) ;
#49797=DIRECTION ( 'NONE',  ( 0.8616291604415301508, 0.000000000000000000, -0.5075383629606968761 ) ) ;
#49812=ORIENTED_EDGE ( 'NONE', *, *, #61474, .F. ) ;
#49813=B_SPLINE_CURVE_WITH_KNOTS ( 'NONE', 3,
 ( #9779, #2796, #71752, #93268, #10273, #93761 ),
 .UNSPECIFIED., .F., .F.,
 ( 4, 2, 4 ),
 ( 3.409110551496109007E-05, 0.0004400426677367863006, 0.0008459942299586115924 ),
 .UNSPECIFIED. ) ;
#49817=CARTESIAN_POINT ( 'NONE',  ( 0.000000000000000000, 0.000000000000000000, 0.000000000000000000 ) ) ;
#49822=LINE ( 'NONE', #80332, #65941 ) ;
#49838=LINE ( 'NONE', #19838, #43092 ) ;
#49846=DIRECTION ( 'NONE',  ( 0.000000000000000000, 0.000000000000000000, -1.000000000000000000 ) ) ;
#49847=ORIENTED_EDGE ( 'NONE', *, *, #63640, .F. ) ;
#49851=ORIENTED_EDGE ( 'NONE', *, *, #32507, .F. ) ;
#49853=VECTOR ( 'NONE', #30841, 1000.000000000000000 ) ;
#49859=DIRECTION ( 'NONE',  ( 0.000000000000000000, 0.000000000000000000, 1.000000000000000000 ) ) ;
#49863=ORIENTED_EDGE ( 'NONE', *, *, #25425, .F. ) ;
#49867=DIRECTION ( 'NONE',  ( -0.6225146366376236307, 0.000000000000000000, 0.7826081568524105858 ) ) ;
#49871=PLANE ( 'NONE',  #7322 ) ;
#49873=CARTESIAN_POINT ( 'NONE',  ( 12.67122524790590710, 14.95077488074853456, -7.555537761805753760 ) ) ;
#49883=ORIENTED_EDGE ( 'NONE', *, *, #19548, .F. ) ;
#49889=DIRECTION ( 'NONE',  ( 0.000000000000000000, 0.000000000000000000, 1.000000000000000000 ) ) ;
#49896=CARTESIAN_POINT ( 'NONE',  ( -14.09394518620605297, 15.00000000000000000, -3.407449058785551710 ) ) ;
#49901=CARTESIAN_POINT ( 'NONE',  ( -5.963430220938290560, 8.854976035794180689, -10.32896413005679648 ) ) ;
#49908=CARTESIAN_POINT ( 'NONE',  ( 1.820328553599968036, 0.000000000000000000, -5.140449258537787891 ) ) ;
#49912=CARTESIAN_POINT ( 'NONE',  ( -1.326261724323127389, 14.76984959128327901, 14.88164196614432377 ) ) ;
#49916=DIRECTION ( 'NONE',  ( -0.000000000000000000, -1.000000000000000000, -0.000000000000000000 ) ) ;
#49920=AXIS2_PLACEMENT_3D ( 'NONE', #37109, #67605, #98112 ) ;
#49927=CARTESIAN_POINT ( 'NONE',  ( -4.850115630859779259, 14.95077488074853456, 13.93278430610803831 ) ) ;
#49940=ORIENTED_EDGE ( 'NONE', *, *, #1410, .F. ) ;
#49944=ADVANCED_FACE ( 'NONE', ( #96287 ), #66303, .T. ) ;
#49945=CARTESIAN_POINT ( 'NONE',  ( -13.78891971893200186, 0.3640475087720986824, -5.904717858191729007 ) ) ;
#49952=CARTESIAN_POINT ( 'NONE',  ( -10.58981376305295008, 15.00000000000000000, 9.535111140613638625 ) ) ;
#49959=AXIS2_PLACEMENT_3D ( 'NONE', #25939, #93445, #24478 ) ;
#49961=CARTESIAN_POINT ( 'NONE',  ( -11.09922568453595382, -36.29303199673623936, -6.408140936763226492 ) ) ;
#49969=DIRECTION ( 'NONE',  ( -0.000000000000000000, -1.000000000000000000, -0.000000000000000000 ) ) ;
#49970=AXIS2_PLACEMENT_3D ( 'NONE', #15814, #37337, #7820 ) ;
#49972=ORIENTED_EDGE ( 'NONE', *, *, #57106, .F. ) ;
#49977=VERTEX_POINT ( 'NONE', #50774 ) ;
#49979=CARTESIAN_POINT ( 'NONE',  ( -12.60589901313228012, 0.3640475087720979053, 8.129656208641964810 ) ) ;
#49986=DIRECTION ( 'NONE',  ( -0.9953961983671785196, 0.000000000000000000, -0.09584575252022721481 ) ) ;
#49991=DIRECTION ( 'NONE',  ( -0.9366721892483947931, 0.000000000000000000, -0.3502073812594747038 ) ) ;
#49997=AXIS2_PLACEMENT_3D ( 'NONE', #50606, #90076, #21602 ) ;
#49998=AXIS2_PLACEMENT_3D ( 'NONE', #35867, #19392, #81853 ) ;
#49999=CARTESIAN_POINT ( 'NONE',  ( -10.58981376305295008, 0.000000000000000000, 9.535111140613638625 ) ) ;
#50003=PLANE ( 'NONE',  #65776 ) ;
#50017=CARTESIAN_POINT ( 'NONE',  ( 10.36894250292378850, -30.07125116508602858, -10.36894250292379027 ) ) ;
#50021=ORIENTED_EDGE ( 'NONE', *, *, #20687, .F. ) ;
#50028=CARTESIAN_POINT ( 'NONE',  ( 7.313705784284503686, 0.5000000000000004441, 13.09617149020748705 ) ) ;
#50030=CARTESIAN_POINT ( 'NONE',  ( -14.97687855664613465, 14.49999999999999112, -0.8325315005902816923 ) ) ;
#50032=CARTESIAN_POINT ( 'NONE',  ( 10.88017736071110164, 20.35535201082150536, 2.915334737309921209 ) ) ;
#50035=TOROIDAL_SURFACE ( 'NONE', #54802, 14.49999999999999822, 0.5000000000000000000 ) ;
#50042=B_SPLINE_CURVE_WITH_KNOTS ( 'NONE', 3,
 ( #16111, #8608, #85099, #62576, #9098, #23636 ),
 .UNSPECIFIED., .F., .F.,
 ( 4, 2, 4 ),
 ( 3.409110551496111039E-05, 0.0004400426677367854874, 0.0008459942299586098577 ),
 .UNSPECIFIED. ) ;
#50052=DIRECTION ( 'NONE',  ( 0.000000000000000000, 0.000000000000000000, 1.000000000000000000 ) ) ;
#50060=CARTESIAN_POINT ( 'NONE',  ( -8.375939845167836850, 15.00000000000000000, 11.52849216984293257 ) ) ;
#50064=CARTESIAN_POINT ( 'NONE',  ( 13.48255862861927312, 3.989652714533045580E-16, -5.335786055104159153 ) ) ;
#50075=CARTESIAN_POINT ( 'NONE',  ( -4.838527690343426002, 14.49999999999999112, -14.19819177887740302 ) ) ;
#50078=CARTESIAN_POINT ( 'NONE',  ( -4.923371831947292776, 6.842264484334122265, 8.527530157486181039 ) ) ;
#50082=LINE ( 'NONE', #81071, #82906 ) ;
#50088=DIRECTION ( 'NONE',  ( 0.9099612708765425495, 0.000000000000000000, 0.4146932426562403018 ) ) ;
#50096=ORIENTED_EDGE ( 'NONE', *, *, #52821, .F. ) ;
#50103=ADVANCED_FACE ( 'NONE', ( #60243 ), #82747, .T. ) ;
#50104=CARTESIAN_POINT ( 'NONE',  ( 10.19513985507828302, 14.49999999999999112, 11.00268709613230200 ) ) ;
#50106=VERTEX_POINT ( 'NONE', #21773 ) ;
#50108=CARTESIAN_POINT ( 'NONE',  ( 13.14228782657334804, 0.5000000000000004441, 7.230509711182329546 ) ) ;
#50110=VERTEX_POINT ( 'NONE', #31707 ) ;
#50111=CARTESIAN_POINT ( 'NONE',  ( -4.547378612396795639, 0.000000000000000000, 3.009844244835475635 ) ) ;
#50115=CARTESIAN_POINT ( 'NONE',  ( 12.25993886608603489, 14.49999999999999112, 8.642563219313760925 ) ) ;
#50117=CARTESIAN_POINT ( 'NONE',  ( -7.108715748589260919, 0.04922511925147068923, 12.92719074505362542 ) ) ;
#50124=CARTESIAN_POINT ( 'NONE',  ( 11.22915323889580463, 15.00000000000000000, -8.773176023390609757 ) ) ;
#50125=EDGE_CURVE ( 'NONE', #76878, #5586, #36651, .T. ) ;
#50127=VERTEX_POINT ( 'NONE', #90737 ) ;
#50134=CARTESIAN_POINT ( 'NONE',  ( 9.508231703811905078, 12.87087484978187746, -6.715038726106763001 ) ) ;
#50140=CARTESIAN_POINT ( 'NONE',  ( 2.915334737309928315, -25.47798132251181968, 10.88017736071109987 ) ) ;
#50146=CARTESIAN_POINT ( 'NONE',  ( 14.35840480524204388, 14.63606918001612556, -4.340070442838849019 ) ) ;
#50154=UNCERTAINTY_MEASURE_WITH_UNIT (LENGTH_MEASURE( 1.000000000000000082E-05 ), #94015, 'distance_accuracy_value', 'NONE');
#50164=FACE_OUTER_BOUND ( 'NONE', #9257, .T. ) ;
#50167=CARTESIAN_POINT ( 'NONE',  ( 7.993154516101047768, 0.04922511925147154271, -12.39982181464614541 ) ) ;
#50185=DIRECTION ( 'NONE',  ( 0.000000000000000000, 1.000000000000000000, 0.000000000000000000 ) ) ;
#50187=CARTESIAN_POINT ( 'NONE',  ( 7.208316651077764980, -37.11606884899919834, 7.208316651077762316 ) ) ;
#50188=VERTEX_POINT ( 'NONE', #22265 ) ;
#50200=CARTESIAN_POINT ( 'NONE',  ( 12.81628187352647608, 1.623634669930422492, -2.602085213965210642E-15 ) ) ;
#50201=ORIENTED_EDGE ( 'NONE', *, *, #91343, .F. ) ;
#50213=CARTESIAN_POINT ( 'NONE',  ( -12.58848565468362857, 15.00000000000000888, 7.447709424579771031 ) ) ;
#50214=LINE ( 'NONE', #71271, #32280 ) ;
#50219=CARTESIAN_POINT ( 'NONE',  ( 11.39601241150452182, 15.00000000000000000, 11.22534175661874301 ) ) ;
#50225=CARTESIAN_POINT ( 'NONE',  ( -14.04391541078760675, 4.104531544909319036E-16, -3.608107528143027043 ) ) ;
#50235=CARTESIAN_POINT ( 'NONE',  ( -2.393480905993257579, 0.3640475087720981273, 14.80781041047750435 ) ) ;
#50236=ADVANCED_FACE ( 'NONE', ( #45745 ), #50384, .T. ) ;
#50239=CARTESIAN_POINT ( 'NONE',  ( -11.25000000000000178, 4.909700295649315649, -3.014428414850122806 ) ) ;
#50245=DIRECTION ( 'NONE',  ( 0.000000000000000000, 0.000000000000000000, 1.000000000000000000 ) ) ;
#50247=DIRECTION ( 'NONE',  ( -0.000000000000000000, -1.000000000000000000, -0.000000000000000000 ) ) ;
#50255=PLANE ( 'NONE',  #7468 ) ;
#50262=CARTESIAN_POINT ( 'NONE',  ( 3.115783986955448892, 15.00000000000000000, 14.16128137375397600 ) ) ;
#50263=VECTOR ( 'NONE', #81478, 1000.000000000000000 ) ;
#50267=ORIENTED_EDGE ( 'NONE', *, *, #82865, .T. ) ;
#50274=CARTESIAN_POINT ( 'NONE',  ( -13.61464873478175797, 14.63606918187687000, 6.296136897217746053 ) ) ;
#50275=EDGE_CURVE ( 'NONE', #77529, #97699, #45242, .T. ) ;
#50283=ADVANCED_FACE ( 'NONE', ( #83741 ), #76241, .F. ) ;
#50302=VERTEX_POINT ( 'NONE', #85712 ) ;
#50305=ORIENTED_EDGE ( 'NONE', *, *, #19506, .T. ) ;
#50307=DIRECTION ( 'NONE',  ( -0.000000000000000000, -1.000000000000000000, -0.000000000000000000 ) ) ;
#50309=ORIENTED_EDGE ( 'NONE', *, *, #39176, .T. ) ;
#50312=DIRECTION ( 'NONE',  ( 0.000000000000000000, 1.000000000000000000, 0.000000000000000000 ) ) ;
#50318=ORIENTED_EDGE ( 'NONE', *, *, #44271, .T. ) ;
#50320=ORIENTED_EDGE ( 'NONE', *, *, #76910, .T. ) ;
#50321=AXIS2_PLACEMENT_3D ( 'NONE', #98095, #53052, #84060 ) ;
#50327=LINE ( 'NONE', #33834, #44668 ) ;
#50331=B_SPLINE_CURVE_WITH_KNOTS ( 'NONE', 3,
 ( #14993, #83472, #68967, #91951, #37492, #29961 ),
 .UNSPECIFIED., .F., .F.,
 ( 4, 2, 4 ),
 ( 3.409110551494637202E-05, 0.0004400426677367925347, 0.0008459942299586386974 ),
 .UNSPECIFIED. ) ;
#50334=CARTESIAN_POINT ( 'NONE',  ( -8.209432707284950226, 0.5000000000000004441, 12.55409154915480485 ) ) ;
#50335=EDGE_CURVE ( 'NONE', #49345, #65924, #42485, .T. ) ;
#50336=AXIS2_PLACEMENT_3D ( 'NONE', #45829, #22345, #16807 ) ;
#50340=ORIENTED_EDGE ( 'NONE', *, *, #42064, .F. ) ;
#50341=DIRECTION ( 'NONE',  ( 0.000000000000000000, 1.000000000000000000, 0.000000000000000000 ) ) ;
#50347=DIRECTION ( 'NONE',  ( 0.000000000000000000, 0.000000000000000000, 1.000000000000000000 ) ) ;
#50349=CARTESIAN_POINT ( 'NONE',  ( 9.876730923139357188, 14.49999999999999112, -11.28938378619066363 ) ) ;
#50355=ORIENTED_EDGE ( 'NONE', *, *, #60315, .F. ) ;
#50356=DIRECTION ( 'NONE',  ( 1.000000000000000000, 0.000000000000000000, 0.000000000000000000 ) ) ;
#50358=AXIS2_PLACEMENT_3D ( 'NONE', #56201, #77702, #32690 ) ;
#50365=EDGE_CURVE ( 'NONE', #85655, #4847, #60360, .T. ) ;
#50371=CARTESIAN_POINT ( 'NONE',  ( -2.933660812630105141, 15.00000000000000000, 15.72485391577587954 ) ) ;
#50377=VECTOR ( 'NONE', #83718, 1000.000000000000114 ) ;
#50379=CARTESIAN_POINT ( 'NONE',  ( 0.000000000000000000, 0.000000000000000000, 0.000000000000000000 ) ) ;
#50382=CARTESIAN_POINT ( 'NONE',  ( -0.3093388210927672244, 0.3640475087720984049, 14.99680997725066867 ) ) ;
#50383=ORIENTED_EDGE ( 'NONE', *, *, #91679, .T. ) ;
#50384=TOROIDAL_SURFACE ( 'NONE', #12068, 14.49999999999999822, 0.5000000000000000000 ) ;
#50386=DIRECTION ( 'NONE',  ( 0.000000000000000000, 1.000000000000000000, 0.000000000000000000 ) ) ;
#50388=CARTESIAN_POINT ( 'NONE',  ( 0.000000000000000000, 0.000000000000000000, 0.000000000000000000 ) ) ;
#50391=CARTESIAN_POINT ( 'NONE',  ( -8.731067818237036704, 9.063309369127512838, -8.731067818237033151 ) ) ;
#50395=FACE_OUTER_BOUND ( 'NONE', #19813, .T. ) ;
#50401=CARTESIAN_POINT ( 'NONE',  ( 8.209432707284861408, 15.00000000000000000, -12.55409154915486170 ) ) ;
#50410=ADVANCED_FACE ( 'NONE', ( #41209 ), #71689, .F. ) ;
#50432=ORIENTED_EDGE ( 'NONE', *, *, #94928, .F. ) ;
#50436=CIRCLE ( 'NONE', #80774, 15.00000000000000000 ) ;
#50437=CARTESIAN_POINT ( 'NONE',  ( -8.502626202121433607, 14.95077488074853456, 12.05617882333531554 ) ) ;
#50444=FACE_OUTER_BOUND ( 'NONE', #83401, .T. ) ;
#50446=EDGE_CURVE ( 'NONE', #27786, #4847, #41695, .T. ) ;
#50448=CARTESIAN_POINT ( 'NONE',  ( -3.434112377981067610, -26.91803199673625002, -12.81628187352647252 ) ) ;
#50459=EDGE_CURVE ( 'NONE', #43985, #76019, #66383, .T. ) ;
#50462=ORIENTED_EDGE ( 'NONE', *, *, #17647, .T. ) ;
#50467=ORIENTED_EDGE ( 'NONE', *, *, #17959, .T. ) ;
#50469=CARTESIAN_POINT ( 'NONE',  ( 5.963430220938279902, 8.021642702460848540, -10.32896413005680181 ) ) ;
#50474=DIRECTION ( 'NONE',  ( 0.000000000000000000, 0.000000000000000000, 1.000000000000000000 ) ) ;
#50476=LINE ( 'NONE', #80980, #85081 ) ;
#50478=CIRCLE ( 'NONE', #55263, 15.00000000000000000 ) ;
#50480=ORIENTED_EDGE ( 'NONE', *, *, #96429, .T. ) ;
#50482=LINE ( 'NONE', #80985, #56564 ) ;
#50484=EDGE_CURVE ( 'NONE', #27552, #12702, #70220, .T. ) ;
#50486=VERTEX_POINT ( 'NONE', #79182 ) ;
#50491=DIRECTION ( 'NONE',  ( 0.000000000000000000, 1.000000000000000000, 0.000000000000000000 ) ) ;
#50498=CARTESIAN_POINT ( 'NONE',  ( -11.49638213510188756, 14.95077488074853456, 9.245501498401852203 ) ) ;
#50499=ORIENTED_EDGE ( 'NONE', *, *, #12228, .F. ) ;
#50506=CARTESIAN_POINT ( 'NONE',  ( 14.43100913237647731, 15.00000000000000000, -1.412789942450803027 ) ) ;
#50509=CARTESIAN_POINT ( 'NONE',  ( -12.26659068614894110, -27.77958449841936073, 7.082119434687058401 ) ) ;
#50513=ORIENTED_EDGE ( 'NONE', *, *, #6804, .F. ) ;
#50514=CARTESIAN_POINT ( 'NONE',  ( 8.375939845167756914, -0.03417435944610275333, -11.52849216984298941 ) ) ;
#50521=CARTESIAN_POINT ( 'NONE',  ( -6.767445849361333643, 0.5000000000000004441, 13.38662304974491946 ) ) ;
#50524=CARTESIAN_POINT ( 'NONE',  ( 3.469446951953614189E-15, 9.313685344154846391, 10.88017736071110342 ) ) ;
#50527=ORIENTED_EDGE ( 'NONE', *, *, #10881, .T. ) ;
#50528=VECTOR ( 'NONE', #72964, 1000.000000000000227 ) ;
#50530=DIRECTION ( 'NONE',  ( 1.563194018672220156E-13, 0.000000000000000000, 1.000000000000000000 ) ) ;
#50539=DIRECTION ( 'NONE',  ( -0.7826081568524105858, 0.000000000000000000, -0.6225146366376238527 ) ) ;
#50542=VERTEX_POINT ( 'NONE', #9214 ) ;
#50545=CARTESIAN_POINT ( 'NONE',  ( 0.000000000000000000, 0.5000000000000004441, 0.000000000000000000 ) ) ;
#50552=FACE_OUTER_BOUND ( 'NONE', #40374, .T. ) ;
#50568=( BOUNDED_CURVE ( )  B_SPLINE_CURVE ( 2, ( #68472, #8447, #13589, #30445, #98499, #60945, #22981, #29954, #53948, #966, #60459, #90949, #15481 ),
 .UNSPECIFIED., .F., .T. ) 
 B_SPLINE_CURVE_WITH_KNOTS ( ( 3, 2, 2, 2, 2, 2, 3 ),
 ( 0.6666666666666666297, 0.6722222222222222765, 0.6777777777777778123, 0.6833333333333333481, 0.6888888888888888840, 0.6944444444444444198, 0.6999999999999999556 ),
 .UNSPECIFIED. ) 
 CURVE ( )  GEOMETRIC_REPRESENTATION_ITEM ( )  RATIONAL_B_SPLINE_CURVE ( ( 1.000000000000000000, 0.9659258262890684232, 1.000000000000000000, 0.9659258262890684232, 1.000000000000000000, 0.9659258262890684232, 1.000000000000000000, 0.9659258262890684232, 1.000000000000000000, 0.9659258262890684232, 1.000000000000000000, 0.9659258262890684232, 1.000000000000000000 ) ) 
 REPRESENTATION_ITEM ( '' )  );
#50569=CARTESIAN_POINT ( 'NONE',  ( -4.838527690343427778, 14.63606918327098327, -14.19819177887737638 ) ) ;
#50571=CARTESIAN_POINT ( 'NONE',  ( -14.62617646268096827, 14.49999999999999112, 3.327906561566773558 ) ) ;
#50572=CARTESIAN_POINT ( 'NONE',  ( 4.923371831947301658, -2.324402182332541145, 8.527530157486175710 ) ) ;
#50573=ORIENTED_EDGE ( 'NONE', *, *, #88343, .F. ) ;
#50576=EDGE_CURVE ( 'NONE', #24815, #80599, #78197, .T. ) ;
#50577=ORIENTED_EDGE ( 'NONE', *, *, #16669, .F. ) ;
#50584=VECTOR ( 'NONE', #35547, 1000.000000000000000 ) ;
#50585=EDGE_CURVE ( 'NONE', #47609, #18352, #53535, .T. ) ;
#50586=AXIS2_PLACEMENT_3D ( 'NONE', #28497, #13497, #74479 ) ;
#50589=ORIENTED_EDGE ( 'NONE', *, *, #35057, .T. ) ;
#50602=VERTEX_POINT ( 'NONE', #27647 ) ;
#50606=CARTESIAN_POINT ( 'NONE',  ( 0.000000000000000000, 14.49999999999999822, 0.000000000000000000 ) ) ;
#50608=EDGE_CURVE ( 'NONE', #11604, #28932, #65641, .T. ) ;
#50609=DIRECTION ( 'NONE',  ( 0.000000000000000000, 1.000000000000000000, 0.000000000000000000 ) ) ;
#50610=CARTESIAN_POINT ( 'NONE',  ( -11.57731665747925831, 12.81546821322845986, 0.2203853198082409703 ) ) ;
#50611=DIRECTION ( 'NONE',  ( 0.3007057995042701770, 0.000000000000000000, 0.9537169507482278208 ) ) ;
#50612=CARTESIAN_POINT ( 'NONE',  ( -3.270351084886603310, 0.04962888917231444985, -14.38617789677966385 ) ) ;
#50615=CARTESIAN_POINT ( 'NONE',  ( 6.767445849361153343, 15.00000000000000000, 13.38662304974501360 ) ) ;
#50617=DIRECTION ( 'NONE',  ( 0.000000000000000000, 1.000000000000000000, 0.000000000000000000 ) ) ;
#50619=DIRECTION ( 'NONE',  ( -0.7826081568524232424, -0.000000000000000000, 0.6225146366376079765 ) ) ;
#50622=CARTESIAN_POINT ( 'NONE',  ( 0.000000000000000000, 15.00000000000000000, 0.000000000000000000 ) ) ;
#50627=EDGE_LOOP ( 'NONE', ( #69778, #83643, #47520, #48615 ) ) ;
#50637=AXIS2_PLACEMENT_3D ( 'NONE', #12105, #25288, #34591 ) ;
#50641=CARTESIAN_POINT ( 'NONE',  ( 9.422509992056141925, -29.01964798917849109, -5.440088680355554374 ) ) ;
#50645=CARTESIAN_POINT ( 'NONE',  ( -0.9082943533608713871, 15.00000000000000000, -14.47152380946376660 ) ) ;
#50646=CARTESIAN_POINT ( 'NONE',  ( 12.50534872682730914, 15.00000000000000000, -7.339363270777500503 ) ) ;
#50649=CARTESIAN_POINT ( 'NONE',  ( 0.000000000000000000, 15.00000000000000000, 0.000000000000000000 ) ) ;
#50655=DIRECTION ( 'NONE',  ( 0.8141155183563107967, 0.000000000000000000, 0.5807029557109515405 ) ) ;
#50659=ORIENTED_EDGE ( 'NONE', *, *, #60997, .F. ) ;
#50661=LINE ( 'NONE', #87663, #38148 ) ;
#50672=EDGE_CURVE ( 'NONE', #61531, #27349, #20150, .T. ) ;
#50673=VERTEX_POINT ( 'NONE', #74123 ) ;
#50676=ORIENTED_EDGE ( 'NONE', *, *, #31276, .F. ) ;
#50677=VERTEX_POINT ( 'NONE', #58133 ) ;
#50678=CARTESIAN_POINT ( 'NONE',  ( 3.014428414850134796, 9.380135511184867880, 11.24999999999999822 ) ) ;
#50693=CARTESIAN_POINT ( 'NONE',  ( 9.846743663894590881, -36.28273551566587685, -2.638427012816833894 ) ) ;
#50695=DIRECTION ( 'NONE',  ( -0.000000000000000000, -1.000000000000000000, -0.000000000000000000 ) ) ;
#50701=VECTOR ( 'NONE', #44093, 1000.000000000000114 ) ;
#50702=DIRECTION ( 'NONE',  ( -0.000000000000000000, -1.000000000000000000, -0.000000000000000000 ) ) ;
#50703=AXIS2_PLACEMENT_3D ( 'NONE', #282, #59752, #60251 ) ;
#50705=ADVANCED_FACE ( 'NONE', ( #26667 ), #19172, .F. ) ;
#50707=CARTESIAN_POINT ( 'NONE',  ( -9.382169495545422677, 8.498634669930423158, -9.382169495545417348 ) ) ;
#50708=ADVANCED_FACE ( 'NONE', ( #43144 ), #31185, .T. ) ;
#50719=DIRECTION ( 'NONE',  ( 0.2334453638559155775, 0.000000000000000000, -0.9723699203976741146 ) ) ;
#50725=ORIENTED_EDGE ( 'NONE', *, *, #25344, .T. ) ;
#50726=CARTESIAN_POINT ( 'NONE',  ( 0.000000000000000000, 15.00000000000000000, 0.000000000000000000 ) ) ;
#50728=CARTESIAN_POINT ( 'NONE',  ( 0.000000000000000000, 15.00000000000000000, 0.000000000000000000 ) ) ;
#50730=CARTESIAN_POINT ( 'NONE',  ( 10.58981376305288613, 0.000000000000000000, -9.535111140613709679 ) ) ;
#50733=PLANE ( 'NONE',  #40386 ) ;
#50734=EDGE_CURVE ( 'NONE', #77766, #50974, #58057, .T. ) ;
#50740=CARTESIAN_POINT ( 'NONE',  ( -14.94699059465099822, 14.49999999999999822, -1.259949270175015013 ) ) ;
#50741=LINE ( 'NONE', #28223, #38521 ) ;
#50744=DIRECTION ( 'NONE',  ( 0.000000000000000000, 0.000000000000000000, 1.000000000000000000 ) ) ;
#50750=CARTESIAN_POINT ( 'NONE',  ( 14.93928340878672500, 14.76930270348881180, 0.2363597353050709837 ) ) ;
#50752=ORIENTED_EDGE ( 'NONE', *, *, #40035, .T. ) ;
#50761=CARTESIAN_POINT ( 'NONE',  ( 0.000000000000000000, 15.00000000000000000, 0.000000000000000000 ) ) ;
#50762=CARTESIAN_POINT ( 'NONE',  ( -14.16423886937410437, 1.595415501580629503, -3.795296366450299885 ) ) ;
#50765=CARTESIAN_POINT ( 'NONE',  ( -11.75209714983983567, 0.04922511925149412187, 8.918201205061931702 ) ) ;
#50774=CARTESIAN_POINT ( 'NONE',  ( 14.26139399674455710, 4.125707382711286748E-16, 2.619664342929903356 ) ) ;
#50775=CARTESIAN_POINT ( 'NONE',  ( -11.48952521350009448, 15.00000000000000000, -8.845383562533896793 ) ) ;
#50778=ORIENTED_EDGE ( 'NONE', *, *, #60374, .F. ) ;
#50781=DIRECTION ( 'NONE',  ( -0.5519369853120501546, 0.000000000000000000, -0.8338858220671735433 ) ) ;
#50786=VECTOR ( 'NONE', #44078, 1000.000000000000114 ) ;
#50789=CARTESIAN_POINT ( 'NONE',  ( 14.19749592853504438, -0.03417435944610275333, -7.369430493279943484 ) ) ;
#50792=CARTESIAN_POINT ( 'NONE',  ( -11.48952521350030587, 15.00000000000000000, 8.845383562533664090 ) ) ;
#50795=EDGE_CURVE ( 'NONE', #88686, #10324, #58643, .T. ) ;
#50798=CIRCLE ( 'NONE', #25276, 15.00000000000000000 ) ;
#50810=CARTESIAN_POINT ( 'NONE',  ( -8.564643372776465924, 14.49999999999999112, -12.31449893000758955 ) ) ;
#50815=ORIENTED_EDGE ( 'NONE', *, *, #82984, .F. ) ;
#50824=ADVANCED_FACE ( 'NONE', ( #12158 ), #69538, .T. ) ;
#50827=ADVANCED_FACE ( 'NONE', ( #73139 ), #95158, .F. ) ;
#50837=DIRECTION ( 'NONE',  ( 0.9862856015372297724, 0.000000000000000000, 0.1650476058606878682 ) ) ;
#50840=ORIENTED_EDGE ( 'NONE', *, *, #71792, .T. ) ;
#50852=CARTESIAN_POINT ( 'NONE',  ( -6.898461952320517732, 15.00000000000000000, 12.75387089053304557 ) ) ;
#50859=ORIENTED_EDGE ( 'NONE', *, *, #80288, .F. ) ;
#50860=AXIS2_PLACEMENT_3D ( 'NONE', #54990, #54500, #16529 ) ;
#50861=CARTESIAN_POINT ( 'NONE',  ( 9.323033696084937816, 14.95037104545395046, 11.43408728005520203 ) ) ;
#50865=CARTESIAN_POINT ( 'NONE',  ( 14.82269085861168811, 0.5000000000000004441, -2.299529454046961519 ) ) ;
#50878=VERTEX_POINT ( 'NONE', #92849 ) ;
#50880=CARTESIAN_POINT ( 'NONE',  ( 14.29730467489533652, 3.971653163193037558E-16, -2.416004766803220516 ) ) ;
#50887=LINE ( 'NONE', #35879, #808 ) ;
#50890=CARTESIAN_POINT ( 'NONE',  ( -3.195792623639522212, 10.72997603579417536, 11.92686044187656691 ) ) ;
#50892=DIRECTION ( 'NONE',  ( 0.000000000000000000, 0.000000000000000000, 1.000000000000000000 ) ) ;
#50899=PLANE ( 'NONE',  #11119 ) ;
#50904=CARTESIAN_POINT ( 'NONE',  ( 14.88232117145530786, 14.49999999999999822, -1.875237731503139438 ) ) ;
#50915=DIRECTION ( 'NONE',  ( 0.000000000000000000, 0.000000000000000000, 1.000000000000000000 ) ) ;
#50918=PLANE ( 'NONE',  #83972 ) ;
#50924=EDGE_LOOP ( 'NONE', ( #21307, #88524, #88966, #8883, #86248, #69040 ) ) ;
#50928=FACE_OUTER_BOUND ( 'NONE', #46649, .T. ) ;
#50930=AXIS2_PLACEMENT_3D ( 'NONE', #82419, #81925, #35441 ) ;
#50931=ORIENTED_EDGE ( 'NONE', *, *, #71792, .F. ) ;
#50941=DIRECTION ( 'NONE',  ( -0.000000000000000000, 1.000000000000000000, -0.000000000000000000 ) ) ;
#50943=EDGE_CURVE ( 'NONE', #14583, #31163, #53604, .T. ) ;
#50945=CARTESIAN_POINT ( 'NONE',  ( -9.399392868737642459, 15.00000000000000000, -11.04089732309485861 ) ) ;
#50947=CARTESIAN_POINT ( 'NONE',  ( 12.81628187352647252, -13.16803199673624825, -3.434112377981059172 ) ) ;
#50955=CARTESIAN_POINT ( 'NONE',  ( -13.07661834287492120, -3.167479706257454935E-15, 6.550615570651588726 ) ) ;
#50962=ORIENTED_EDGE ( 'NONE', *, *, #40419, .F. ) ;
#50974=VERTEX_POINT ( 'NONE', #40360 ) ;
#50975=CARTESIAN_POINT ( 'NONE',  ( 0.2078314800211761848, 0.04962894115304285203, 14.75174957775520213 ) ) ;
#50977=ORIENTED_EDGE ( 'NONE', *, *, #5834, .F. ) ;
#50979=CARTESIAN_POINT ( 'NONE',  ( 2.913501739333762774, 15.00000000000000000, -14.20427779279532565 ) ) ;
#50981=EDGE_CURVE ( 'NONE', #765, #61749, #23889, .T. ) ;
#50983=DIRECTION ( 'NONE',  ( 0.000000000000000000, 1.000000000000000000, 0.000000000000000000 ) ) ;
#50994=DIRECTION ( 'NONE',  ( 0.000000000000000000, 1.000000000000000000, 0.000000000000000000 ) ) ;
#50996=CARTESIAN_POINT ( 'NONE',  ( -3.795296366450300773, -22.15458449841936073, 14.16423886937410437 ) ) ;
#51012=CARTESIAN_POINT ( 'NONE',  ( -9.422509992056145478, 17.64701867748817676, -5.440088680355541939 ) ) ;
#51023=EDGE_CURVE ( 'NONE', #1044, #42348, #1391, .T. ) ;
#51043=ADVANCED_FACE ( 'NONE', ( #78837 ), #16869, .F. ) ;
#51046=VERTEX_POINT ( 'NONE', #84866 ) ;
#51052=CARTESIAN_POINT ( 'NONE',  ( 4.431036607602561794, 0.5000000000000004441, -14.33059365769911153 ) ) ;
#51057=DIRECTION ( 'NONE',  ( 0.000000000000000000, 0.000000000000000000, 1.000000000000000000 ) ) ;
#51060=CARTESIAN_POINT ( 'NONE',  ( 12.34086200392826882, 0.000000000000000000, -7.124999999999971578 ) ) ;
#51061=CARTESIAN_POINT ( 'NONE',  ( 9.846743663894594434, 8.508931151000792781, -2.168404344971008868E-15 ) ) ;
#51063=ORIENTED_EDGE ( 'NONE', *, *, #58713, .F. ) ;
#51065=ORIENTED_EDGE ( 'NONE', *, *, #82436, .F. ) ;
#51083=AXIS2_PLACEMENT_3D ( 'NONE', #66387, #72902, #43393 ) ;
#51088=CARTESIAN_POINT ( 'NONE',  ( 1.236355250167264774, 0.04962892728884438220, 14.70131747622448337 ) ) ;
#51089=AXIS2_PLACEMENT_3D ( 'NONE', #44884, #14414, #85733 ) ;
#51094=B_SPLINE_CURVE_WITH_KNOTS ( 'NONE', 3,
 ( #33433, #40481, #26437, #49429, #70978, #25957 ),
 .UNSPECIFIED., .F., .F.,
 ( 4, 2, 4 ),
 ( 0.0002800001862105926565, 0.0006862054174524929908, 0.001092410648694393163 ),
 .UNSPECIFIED. ) ;
#51095=EDGE_LOOP ( 'NONE', ( #87662, #8768, #25611, #29058, #92157, #31187 ) ) ;
#51097=CARTESIAN_POINT ( 'NONE',  ( 14.42571047809459195, 14.76930270348883134, -3.890621016587847869 ) ) ;
#51099=AXIS2_PLACEMENT_3D ( 'NONE', #5757, #59227, #28737 ) ;
#51109=PLANE ( 'NONE',  #94604 ) ;
#51112=CARTESIAN_POINT ( 'NONE',  ( 0.000000000000000000, 0.000000000000000000, 0.000000000000000000 ) ) ;
#51116=VERTEX_POINT ( 'NONE', #39376 ) ;
#51129=CARTESIAN_POINT ( 'NONE',  ( 3.469446951953614189E-15, -25.68631465584515894, 10.88017736071110342 ) ) ;
#51133=CARTESIAN_POINT ( 'NONE',  ( 2.930023131210769627, 0.000000000000000000, -4.599215049682158885 ) ) ;
#51138=VECTOR ( 'NONE', #56691, 1000.000000000000227 ) ;
#51139=EDGE_CURVE ( 'NONE', #61703, #93127, #2868, .T. ) ;
#51143=DIRECTION ( 'NONE',  ( 0.8526401643540847397, 0.000000000000000000, 0.5224985647159611224 ) ) ;
#51144=EDGE_CURVE ( 'NONE', #23745, #11622, #45615, .T. ) ;
#51151=ORIENTED_EDGE ( 'NONE', *, *, #33090, .T. ) ;
#51161=CYLINDRICAL_SURFACE ( 'NONE', #20820, 15.00000000000000000 ) ;
#51167=ORIENTED_EDGE ( 'NONE', *, *, #82402, .T. ) ;
#51169=CARTESIAN_POINT ( 'NONE',  ( -5.428133280998936883, 0.000000000000000000, -0.5226697871168243248 ) ) ;
#51185=CARTESIAN_POINT ( 'NONE',  ( -8.527530157486182816, -34.40773551566587685, -4.923371831947288335 ) ) ;
#51188=VERTEX_POINT ( 'NONE', #16375 ) ;
#51193=DIRECTION ( 'NONE',  ( -1.776356839400250780E-14, 0.000000000000000000, 1.000000000000000000 ) ) ;
#51198=CARTESIAN_POINT ( 'NONE',  ( 11.09922568453594671, 12.04030133659709456, -6.408140936763241591 ) ) ;
#51211=CARTESIAN_POINT ( 'NONE',  ( 13.34343830728403724, 14.49999999999999112, 6.852200678592740068 ) ) ;
#51212=TOROIDAL_SURFACE ( 'NONE', #25678, 14.49999999999999822, 0.5000000000000000000 ) ;
#51214=DIRECTION ( 'NONE',  ( 0.000000000000000000, 0.000000000000000000, 1.000000000000000000 ) ) ;
#51215=CARTESIAN_POINT ( 'NONE',  ( -12.25993886608611660, 0.5000000000000004441, 8.642563219313529999 ) ) ;
#51218=AXIS2_PLACEMENT_3D ( 'NONE', #33069, #61239, #71585 ) ;
#51220=VERTEX_POINT ( 'NONE', #72306 ) ;
#51222=CARTESIAN_POINT ( 'NONE',  ( 0.8060400322138880913, 0.000000000000000000, 5.393339789881745894 ) ) ;
#51226=CARTESIAN_POINT ( 'NONE',  ( 14.24131928502211686, 15.00000000000000000, -0.4973178280105898241 ) ) ;
#51230=EDGE_CURVE ( 'NONE', #35164, #7679, #18280, .T. ) ;
#51234=CARTESIAN_POINT ( 'NONE',  ( -12.74305857943755882, 15.00000000000000178, 7.177950183686771624 ) ) ;
#51236=ORIENTED_EDGE ( 'NONE', *, *, #37081, .F. ) ;
#51247=CARTESIAN_POINT ( 'NONE',  ( -10.36894250292379205, 11.17874883491397675, -10.36894250292378672 ) ) ;
#51256=EDGE_CURVE ( 'NONE', #54489, #41784, #87799, .T. ) ;
#51257=VECTOR ( 'NONE', #72398, 1000.000000000000000 ) ;
#51258=EDGE_LOOP ( 'NONE', ( #42895, #76499, #1362, #94405 ) ) ;
#51261=FACE_OUTER_BOUND ( 'NONE', #65424, .T. ) ;
#51268=VERTEX_POINT ( 'NONE', #3337 ) ;
#51270=CARTESIAN_POINT ( 'NONE',  ( -11.10175276307583658, 0.04962894967561114201, -9.716398248524834358 ) ) ;
#51271=PLANE ( 'NONE',  #50703 ) ;
#51292=DIRECTION ( 'NONE',  ( 0.000000000000000000, 1.000000000000000000, 0.000000000000000000 ) ) ;
#51296=CIRCLE ( 'NONE', #40161, 14.49999999999999822 ) ;
#51297=CARTESIAN_POINT ( 'NONE',  ( -14.43100913236851568, 4.866596497322921311E-16, 1.412789942453065883 ) ) ;
#51299=EDGE_CURVE ( 'NONE', #58998, #58863, #71173, .T. ) ;
#51306=ORIENTED_EDGE ( 'NONE', *, *, #5216, .T. ) ;
#51310=EDGE_LOOP ( 'NONE', ( #19448, #75087, #38693, #76667 ) ) ;
#51312=DIRECTION ( 'NONE',  ( 0.000000000000000000, 1.000000000000000000, 0.000000000000000000 ) ) ;
#51317=ORIENTED_EDGE ( 'NONE', *, *, #75291, .F. ) ;
#51319=ORIENTED_EDGE ( 'NONE', *, *, #77114, .F. ) ;
#51321=CARTESIAN_POINT ( 'NONE',  ( 3.541595367958687568, 0.000000000000000000, -4.146675399920591865 ) ) ;
#51324=PLANE ( 'NONE',  #52661 ) ;
#51328=B_SPLINE_CURVE_WITH_KNOTS ( 'NONE', 3,
 ( #86569, #87050, #95541, #27031, #57530, #88024 ),
 .UNSPECIFIED., .F., .F.,
 ( 4, 2, 4 ),
 ( 0.0002800086601590408698, 0.0006862139742845935111, 0.001092419288410146315 ),
 .UNSPECIFIED. ) ;
#51330=VECTOR ( 'NONE', #7885, 1000.000000000000227 ) ;
#51331=ORIENTED_EDGE ( 'NONE', *, *, #41586, .F. ) ;
#51338=CARTESIAN_POINT ( 'NONE',  ( 0.000000000000000000, 0.5000000000000004441, 0.000000000000000000 ) ) ;
#51341=DIRECTION ( 'NONE',  ( -3.996802888650562914E-14, 0.000000000000000000, 1.000000000000000000 ) ) ;
#51345=DIRECTION ( 'NONE',  ( 0.000000000000000000, 0.000000000000000000, 1.000000000000000000 ) ) ;
#51346=DIRECTION ( 'NONE',  ( 0.4461978131098069400, 0.000000000000000000, -0.8949343616020258851 ) ) ;
#51352=AXIS2_PLACEMENT_3D ( 'NONE', #37036, #68026, #8506 ) ;
#51365=CARTESIAN_POINT ( 'NONE',  ( -10.82361996477984789, 0.04962893104176982484, 10.02529603627126953 ) ) ;
#51375=EDGE_CURVE ( 'NONE', #79612, #1475, #43814, .T. ) ;
#51376=DIRECTION ( 'NONE',  ( -0.4924235601034707144, 0.000000000000000000, 0.8703556959398975890 ) ) ;
#51377=VERTEX_POINT ( 'NONE', #42319 ) ;
#51381=CARTESIAN_POINT ( 'NONE',  ( 12.34086200392826882, -0.03417435944610275333, -7.124999999999971578 ) ) ;
#51389=VERTEX_POINT ( 'NONE', #73786 ) ;
#51402=CARTESIAN_POINT ( 'NONE',  ( 0.000000000000000000, 0.000000000000000000, 0.000000000000000000 ) ) ;
#51412=VERTEX_POINT ( 'NONE', #27298 ) ;
#51413=CARTESIAN_POINT ( 'NONE',  ( 13.64884605730314426, -0.03417435944610275333, -8.341846182955777067 ) ) ;
#51436=AXIS2_PLACEMENT_3D ( 'NONE', #29791, #60303, #90796 ) ;
#51439=EDGE_LOOP ( 'NONE', ( #93043, #64603, #42440, #63830, #44422, #98315 ) ) ;
#51442=CARTESIAN_POINT ( 'NONE',  ( -6.408140936763232709, -15.04303199673624469, 11.09922568453595026 ) ) ;
#51443=VECTOR ( 'NONE', #74360, 1000.000000000000000 ) ;
#51464=CARTESIAN_POINT ( 'NONE',  ( 14.82269085861167390, 14.49999999999999822, 2.299529454047062327 ) ) ;
#51471=CARTESIAN_POINT ( 'NONE',  ( 0.000000000000000000, 0.000000000000000000, 0.000000000000000000 ) ) ;
#51476=CARTESIAN_POINT ( 'NONE',  ( 11.49638213510176499, 0.04922511925147023820, 9.245501498402024509 ) ) ;
#51486=CARTESIAN_POINT ( 'NONE',  ( 5.240416992896808068, 0.04922511925147525502, -13.79072622793301761 ) ) ;
#51494=CARTESIAN_POINT ( 'NONE',  ( 3.795296366450306547, -19.65458449841936428, -14.16423886937410259 ) ) ;
#51502=CARTESIAN_POINT ( 'NONE',  ( 10.93781366033343083, 14.49999999999999112, 10.26470809774079029 ) ) ;
#51506=CARTESIAN_POINT ( 'NONE',  ( 0.000000000000000000, 0.5000000000000004441, 0.000000000000000000 ) ) ;
#51511=LINE ( 'NONE', #82003, #85459 ) ;
#51515=CARTESIAN_POINT ( 'NONE',  ( -14.43063482171897149, -2.270048298641522937E-16, 2.386446184882927035 ) ) ;
#51516=EDGE_LOOP ( 'NONE', ( #9764, #25959, #65414, #77359, #51317, #39178 ) ) ;
#51527=DIRECTION ( 'NONE',  ( -3.819167204710539130E-14, 0.000000000000000000, 1.000000000000000000 ) ) ;
#51539=EDGE_CURVE ( 'NONE', #97117, #83990, #83945, .T. ) ;
#51559=B_SPLINE_CURVE_WITH_KNOTS ( 'NONE', 3,
 ( #57715, #58706, #88216, #19723, #50213, #12219 ),
 .UNSPECIFIED., .F., .F.,
 ( 4, 2, 4 ),
 ( 3.409110551494643978E-05, 0.0004400426677367937273, 0.0008459942299586410827 ),
 .UNSPECIFIED. ) ;
#51560=CARTESIAN_POINT ( 'NONE',  ( -13.21236992757677164, 15.00000000000000000, 5.338143956176621074 ) ) ;
#51564=CARTESIAN_POINT ( 'NONE',  ( -9.846743663894596210, 15.80059781766745353, -2.638427012816824124 ) ) ;
#51566=ORIENTED_EDGE ( 'NONE', *, *, #6348, .F. ) ;
#51567=LINE ( 'NONE', #38056, #43005 ) ;
#51581=VERTEX_POINT ( 'NONE', #27795 ) ;
#51590=B_SPLINE_CURVE_WITH_KNOTS ( 'NONE', 3,
 ( #37041, #36549, #44528, #98559, #61007, #91008 ),
 .UNSPECIFIED., .F., .F.,
 ( 4, 2, 4 ),
 ( 0.0002800858945027140997, 0.0006862919646584248693, 0.001092498034814135639 ),
 .UNSPECIFIED. ) ;
#51597=ORIENTED_EDGE ( 'NONE', *, *, #31761, .T. ) ;
#51599=ADVANCED_FACE ( 'NONE', ( #87316 ), #89778, .T. ) ;
#51600=LINE ( 'NONE', #66595, #6970 ) ;
#51607=CARTESIAN_POINT ( 'NONE',  ( 14.47650479471822216, 0.5000000000000004441, -3.928206833722012625 ) ) ;
#51608=ORIENTED_EDGE ( 'NONE', *, *, #44718, .F. ) ;
#51619=CARTESIAN_POINT ( 'NONE',  ( 0.000000000000000000, 0.000000000000000000, 0.000000000000000000 ) ) ;
#51631=CARTESIAN_POINT ( 'NONE',  ( 12.60589901313221439, 0.5000000000000004441, -8.129656208642048298 ) ) ;
#51636=CARTESIAN_POINT ( 'NONE',  ( -7.964842623401179544, -12.56131465584515894, -7.964842623401174215 ) ) ;
#51639=CARTESIAN_POINT ( 'NONE',  ( 14.61146088927472420, 2.439454888092384977E-16, 0.6660010753335569023 ) ) ;
#51651=VERTEX_POINT ( 'NONE', #14798 ) ;
#51654=CYLINDRICAL_SURFACE ( 'NONE', #11078, 15.00000000000000000 ) ;
#51659=CARTESIAN_POINT ( 'NONE',  ( -14.26139399674453578, 3.905478766663822759E-16, -2.619664342929995282 ) ) ;
#51665=ORIENTED_EDGE ( 'NONE', *, *, #72713, .T. ) ;
#51670=CARTESIAN_POINT ( 'NONE',  ( 12.98685442714199390, 3.839196892837649736E-16, -6.449155920600954772 ) ) ;
#51685=CARTESIAN_POINT ( 'NONE',  ( 9.846743663894594434, -26.49106884899921255, -2.168404344971008868E-15 ) ) ;
#51687=CARTESIAN_POINT ( 'NONE',  ( 13.34989199099675439, 0.04962897297196695173, 6.279943681065537575 ) ) ;
#51698=CARTESIAN_POINT ( 'NONE',  ( 6.408140936763236262, 12.45696800326375531, -11.09922568453595026 ) ) ;
#51700=EDGE_CURVE ( 'NONE', #33002, #71459, #7784, .T. ) ;
#51707=PLANE ( 'NONE',  #38773 ) ;
#51711=PLANE ( 'NONE',  #23322 ) ;
#51713=DIRECTION ( 'NONE',  ( 0.000000000000000000, 0.000000000000000000, 1.000000000000000000 ) ) ;
#51717=EDGE_CURVE ( 'NONE', #16296, #88170, #45271, .T. ) ;
#51723=FACE_OUTER_BOUND ( 'NONE', #79979, .T. ) ;
#51724=ORIENTED_EDGE ( 'NONE', *, *, #96791, .T. ) ;
#51726=DIRECTION ( 'NONE',  ( -0.9890158633619177131, 0.000000000000000000, 0.1478094111296046342 ) ) ;
#51730=CARTESIAN_POINT ( 'NONE',  ( -4.431036607602684363, 14.63606876205412632, 14.33059365769911508 ) ) ;
#51743=CARTESIAN_POINT ( 'NONE',  ( 0.000000000000000000, 15.00000000000000000, -14.25000000000000000 ) ) ;
#51744=EDGE_CURVE ( 'NONE', #56319, #85753, #10289, .T. ) ;
#51750=CARTESIAN_POINT ( 'NONE',  ( 14.16423886937410437, 4.095415501580630391, 3.795296366450304770 ) ) ;
#51769=CARTESIAN_POINT ( 'NONE',  ( -1.114591949024815731, 15.00000000000000000, -14.45709807627963350 ) ) ;
#51774=CARTESIAN_POINT ( 'NONE',  ( -12.03768810259491140, -3.868822986584015221E-15, 8.306778944023246680 ) ) ;
#51781=VERTEX_POINT ( 'NONE', #77731 ) ;
#51783=LINE ( 'NONE', #53754, #30077 ) ;
#51792=CARTESIAN_POINT ( 'NONE',  ( 0.000000000000000000, 15.00000000000000000, 0.000000000000000000 ) ) ;
#51801=ORIENTED_EDGE ( 'NONE', *, *, #45088, .T. ) ;
#51802=ADVANCED_FACE ( 'NONE', ( #2755 ), #24748, .F. ) ;
#51805=CARTESIAN_POINT ( 'NONE',  ( 0.000000000000000000, 0.000000000000000000, 0.000000000000000000 ) ) ;
#51808=ORIENTED_EDGE ( 'NONE', *, *, #86071, .F. ) ;
#51816=EDGE_CURVE ( 'NONE', #5586, #47253, #51822, .T. ) ;
#51819=DIRECTION ( 'NONE',  ( -0.000000000000000000, 1.000000000000000000, -0.000000000000000000 ) ) ;
#51822=CIRCLE ( 'NONE', #5514, 15.00000000000000000 ) ;
#51823=ADVANCED_FACE ( 'NONE', ( #77241 ), #90132, .T. ) ;
#51830=EDGE_CURVE ( 'NONE', #5117, #39559, #85247, .T. ) ;
#51832=PLANE ( 'NONE',  #91399 ) ;
#51835=DIRECTION ( 'NONE',  ( 0.9170600743851183845, 0.000000000000000000, 0.3987490689252592979 ) ) ;
#51843=ORIENTED_EDGE ( 'NONE', *, *, #35665, .F. ) ;
#51845=FACE_OUTER_BOUND ( 'NONE', #279, .T. ) ;
#51849=LINE ( 'NONE', #57372, #82385 ) ;
#51853=ORIENTED_EDGE ( 'NONE', *, *, #90191, .T. ) ;
#51858=ADVANCED_FACE ( 'NONE', ( #70251 ), #3942, .T. ) ;
#51862=DIRECTION ( 'NONE',  ( -0.5075383629607084224, 0.000000000000000000, 0.8616291604415231564 ) ) ;
#51870=DIRECTION ( 'NONE',  ( 0.000000000000000000, 0.000000000000000000, 1.000000000000000000 ) ) ;
#51871=EDGE_CURVE ( 'NONE', #9609, #79224, #22122, .T. ) ;
#51875=LINE ( 'NONE', #90845, #88002 ) ;
#51876=ORIENTED_EDGE ( 'NONE', *, *, #61286, .T. ) ;
#51888=LINE ( 'NONE', #89878, #11083 ) ;
#51898=CARTESIAN_POINT ( 'NONE',  ( -2.913501739333854701, 4.099883984707052505E-16, 14.20427779279533098 ) ) ;
#51899=CARTESIAN_POINT ( 'NONE',  ( -10.32896413005679470, 3.078790035174472361, 5.963430220938290560 ) ) ;
#51901=CIRCLE ( 'NONE', #26334, 15.00000000000000000 ) ;
#51904=CARTESIAN_POINT ( 'NONE',  ( 9.240973841163533820, 15.00000000000000000, 11.17382667070378943 ) ) ;
#51933=DIRECTION ( 'NONE',  ( 0.000000000000000000, 0.000000000000000000, 1.000000000000000000 ) ) ;
#51935=LINE ( 'NONE', #75412, #55650 ) ;
#51939=ORIENTED_EDGE ( 'NONE', *, *, #31843, .T. ) ;
#51941=CARTESIAN_POINT ( 'NONE',  ( 12.81628187352647252, -18.16803199673624292, -3.434112377981059172 ) ) ;
#51945=CARTESIAN_POINT ( 'NONE',  ( 0.000000000000000000, 15.00000000000000000, 0.000000000000000000 ) ) ;
#51950=EDGE_CURVE ( 'NONE', #74051, #46208, #66220, .T. ) ;
#51951=AXIS2_PLACEMENT_3D ( 'NONE', #41527, #71530, #78521 ) ;
#51971=ORIENTED_EDGE ( 'NONE', *, *, #20069, .T. ) ;
#51977=EDGE_CURVE ( 'NONE', #19380, #80716, #80555, .T. ) ;
#51979=CARTESIAN_POINT ( 'NONE',  ( 11.62719953690058539, 0.3640475087720986269, 9.476720473301883274 ) ) ;
#51985=DIRECTION ( 'NONE',  ( 0.000000000000000000, 0.000000000000000000, 1.000000000000000000 ) ) ;
#51996=CARTESIAN_POINT ( 'NONE',  ( -3.795296366450322534, -19.23791783175269998, -14.16423886937409904 ) ) ;
#52000=VERTEX_POINT ( 'NONE', #76750 ) ;
#52007=FACE_OUTER_BOUND ( 'NONE', #1164, .T. ) ;
#52009=CARTESIAN_POINT ( 'NONE',  ( -6.767445849361066301, 0.5000000000000004441, -13.38662304974505801 ) ) ;
#52010=DIRECTION ( 'NONE',  ( -0.5664062369248369366, 0.000000000000000000, 0.8241261886220129229 ) ) ;
#52015=CARTESIAN_POINT ( 'NONE',  ( -14.82269085861171298, 0.3640475087720979608, 2.299529454046859822 ) ) ;
#52019=CARTESIAN_POINT ( 'NONE',  ( 12.25993886608599581, 0.5000000000000004441, 8.642563219313704082 ) ) ;
#52036=LINE ( 'NONE', #58041, #50584 ) ;
#52040=EDGE_CURVE ( 'NONE', #73542, #3919, #787, .T. ) ;
#52042=ORIENTED_EDGE ( 'NONE', *, *, #78535, .F. ) ;
#52049=CARTESIAN_POINT ( 'NONE',  ( -10.09777502097891499, 14.95077488074853456, 10.75551206493373257 ) ) ;
#52057=CARTESIAN_POINT ( 'NONE',  ( -3.469446951953614189E-15, 9.758931151000794557, -9.846743663894594434 ) ) ;
#52058=VERTEX_POINT ( 'NONE', #23778 ) ;
#52059=ORIENTED_EDGE ( 'NONE', *, *, #97004, .F. ) ;
#52060=CARTESIAN_POINT ( 'NONE',  ( 1.175037534397233241, 15.00000000000000711, -14.57833316477036689 ) ) ;
#52061=ORIENTED_EDGE ( 'NONE', *, *, #34522, .T. ) ;
#52068=AXIS2_PLACEMENT_3D ( 'NONE', #72436, #3964, #81423 ) ;
#52071=TOROIDAL_SURFACE ( 'NONE', #21744, 14.49999999999999822, 0.5000000000000000000 ) ;
#52075=EDGE_CURVE ( 'NONE', #23697, #85150, #27903, .T. ) ;
#52079=ORIENTED_EDGE ( 'NONE', *, *, #58486, .F. ) ;
#52084=CARTESIAN_POINT ( 'NONE',  ( -14.97687855664607248, 0.5000000000000004441, -0.8325315005902533816 ) ) ;
#52086=ORIENTED_EDGE ( 'NONE', *, *, #38436, .T. ) ;
#52088=ORIENTED_EDGE ( 'NONE', *, *, #30883, .F. ) ;
#52090=ORIENTED_EDGE ( 'NONE', *, *, #73027, .F. ) ;
#52091=EDGE_CURVE ( 'NONE', #8762, #42622, #6191, .T. ) ;
#52092=CARTESIAN_POINT ( 'NONE',  ( -11.54609836565341929, 12.78764854742128598, -0.3568064872451662262 ) ) ;
#52093=CYLINDRICAL_SURFACE ( 'NONE', #53781, 15.00000000000000000 ) ;
#52094=DIRECTION ( 'NONE',  ( 0.000000000000000000, 0.000000000000000000, 1.000000000000000000 ) ) ;
#52097=ORIENTED_EDGE ( 'NONE', *, *, #22814, .F. ) ;
#52100=CARTESIAN_POINT ( 'NONE',  ( -13.34343830728409053, 14.63595249122790598, 6.852200678592508254 ) ) ;
#52105=CARTESIAN_POINT ( 'NONE',  ( -11.48952521350030587, 4.186587853438871531E-16, 8.845383562533662314 ) ) ;
#52109=ORIENTED_EDGE ( 'NONE', *, *, #4559, .F. ) ;
#52115=FACE_OUTER_BOUND ( 'NONE', #43909, .T. ) ;
#52118=CARTESIAN_POINT ( 'NONE',  ( -0.9082943533638283551, 15.00000000000000000, 14.47152380945581918 ) ) ;
#52121=CARTESIAN_POINT ( 'NONE',  ( 5.440088680355556150, -10.26964798917848931, 9.422509992056138373 ) ) ;
#52123=CARTESIAN_POINT ( 'NONE',  ( 14.62232599144297396, 2.134523027080836854E-16, -0.3548652576988654550 ) ) ;
#52139=DIRECTION ( 'NONE',  ( 0.000000000000000000, 1.000000000000000000, 0.000000000000000000 ) ) ;
#52145=FACE_OUTER_BOUND ( 'NONE', #29485, .T. ) ;
#52149=EDGE_LOOP ( 'NONE', ( #47009, #29514, #77272, #62578 ) ) ;
#52150=CARTESIAN_POINT ( 'NONE',  ( -14.29730467489527967, 15.00000000000000000, -2.416004766803415471 ) ) ;
#52152=ORIENTED_EDGE ( 'NONE', *, *, #73420, .T. ) ;
#52154=CARTESIAN_POINT ( 'NONE',  ( -9.402796353261203777, 0.5000000000000004441, 11.68706210897750708 ) ) ;
#52162=LINE ( 'NONE', #95696, #70647 ) ;
#52170=CARTESIAN_POINT ( 'NONE',  ( -3.469446951953614189E-15, -30.24106884899920900, -9.846743663894594434 ) ) ;
#52171=ORIENTED_EDGE ( 'NONE', *, *, #95985, .T. ) ;
#52173=ORIENTED_EDGE ( 'NONE', *, *, #94394, .F. ) ;
#52174=VERTEX_POINT ( 'NONE', #29172 ) ;
#52176=DIRECTION ( 'NONE',  ( -0.3007057995042767273, 0.000000000000000000, 0.9537169507482258224 ) ) ;
#52184=CARTESIAN_POINT ( 'NONE',  ( -11.09922568453595382, 18.70696800326376774, -6.408140936763226492 ) ) ;
#52189=ORIENTED_EDGE ( 'NONE', *, *, #70129, .F. ) ;
#52195=LINE ( 'NONE', #22698, #53098 ) ;
#52198=FACE_OUTER_BOUND ( 'NONE', #83970, .T. ) ;
#52199=EDGE_LOOP ( 'NONE', ( #12063, #75944, #92749, #16287 ) ) ;
#52207=DIRECTION ( 'NONE',  ( 0.000000000000000000, 0.000000000000000000, 1.000000000000000000 ) ) ;
#52217=VECTOR ( 'NONE', #3426, 1000.000000000000000 ) ;
#52227=LINE ( 'NONE', #22236, #4267 ) ;
#52235=PLANE ( 'NONE',  #1676 ) ;
#52239=CARTESIAN_POINT ( 'NONE',  ( 12.26659068614894466, 14.72041550158064638, -7.082119434687053960 ) ) ;
#52246=ORIENTED_EDGE ( 'NONE', *, *, #79124, .F. ) ;
#52250=CARTESIAN_POINT ( 'NONE',  ( 15.94536257719940409, -0.03417435944610275333, 1.273895096820067296 ) ) ;
#52251=CARTESIAN_POINT ( 'NONE',  ( -11.62719953690071506, 0.5000000000000004441, 9.476720473301710967 ) ) ;
#52252=AXIS2_PLACEMENT_3D ( 'NONE', #61906, #2430, #46905 ) ;
#52258=CARTESIAN_POINT ( 'NONE',  ( -5.817157072110894944, 14.49999999999999112, 13.82608706751089755 ) ) ;
#52263=PLANE ( 'NONE',  #65618 ) ;
#52270=EDGE_CURVE ( 'NONE', #54861, #43424, #15064, .T. ) ;
#52273=CARTESIAN_POINT ( 'NONE',  ( 11.25000000000000355, 5.421802177851542837, -2.602085213965210642E-15 ) ) ;
#52279=EDGE_CURVE ( 'NONE', #32515, #50673, #34308, .T. ) ;
#52286=CIRCLE ( 'NONE', #45875, 15.00000000000000000 ) ;
#52290=EDGE_CURVE ( 'NONE', #40499, #38777, #51901, .T. ) ;
#52293=ORIENTED_EDGE ( 'NONE', *, *, #88420, .T. ) ;
#52298=DIRECTION ( 'NONE',  ( 0.000000000000000000, 0.000000000000000000, 1.000000000000000000 ) ) ;
#52305=CARTESIAN_POINT ( 'NONE',  ( 0.000000000000000000, 14.49999999999999822, 0.000000000000000000 ) ) ;
#52307=ADVANCED_FACE ( 'NONE', ( #17154 ), #92632, .F. ) ;
#52308=ORIENTED_EDGE ( 'NONE', *, *, #53329, .F. ) ;
#52310=DIRECTION ( 'NONE',  ( 0.000000000000000000, 1.000000000000000000, 0.000000000000000000 ) ) ;
#52315=B_SPLINE_CURVE_WITH_KNOTS ( 'NONE', 3,
 ( #47733, #69271, #77736, #17258, #46269, #71237 ),
 .UNSPECIFIED., .F., .F.,
 ( 4, 2, 4 ),
 ( 3.409110551326284999E-05, 0.0004400426677351060040, 0.0008459942299569491852 ),
 .UNSPECIFIED. ) ;
#52336=ORIENTED_EDGE ( 'NONE', *, *, #98148, .T. ) ;
#52353=TOROIDAL_SURFACE ( 'NONE', #9255, 14.49999999999999822, 0.5000000000000000000 ) ;
#52355=VECTOR ( 'NONE', #50609, 1000.000000000000000 ) ;
#52356=LINE ( 'NONE', #13370, #95392 ) ;
#52364=CARTESIAN_POINT ( 'NONE',  ( -5.625000000000007994, 7.088468844518210688, -9.742785792574931492 ) ) ;
#52370=ORIENTED_EDGE ( 'NONE', *, *, #74957, .T. ) ;
#52376=LINE ( 'NONE', #82880, #68721 ) ;
#52377=DIRECTION ( 'NONE',  ( 0.000000000000000000, 1.000000000000000000, 0.000000000000000000 ) ) ;
#52384=ADVANCED_FACE ( 'NONE', ( #9640 ), #63605, .F. ) ;
#52386=B_SPLINE_CURVE_WITH_KNOTS ( 'NONE', 3,
 ( #73873, #59359, #65874, #73375, #80400, #42894 ),
 .UNSPECIFIED., .F., .F.,
 ( 4, 2, 4 ),
 ( 0.0002800225282680458404, 0.0006862279780657128125, 0.001092433427863379785 ),
 .UNSPECIFIED. ) ;
#52387=EDGE_CURVE ( 'NONE', #97699, #59012, #10362, .T. ) ;
#52392=EDGE_CURVE ( 'NONE', #14084, #76878, #18356, .T. ) ;
#52408=CARTESIAN_POINT ( 'NONE',  ( 0.000000000000000000, 0.5000000000000004441, 0.000000000000000000 ) ) ;
#52411=ORIENTED_EDGE ( 'NONE', *, *, #87122, .T. ) ;
#52423=ORIENTED_EDGE ( 'NONE', *, *, #35000, .T. ) ;
#52426=CARTESIAN_POINT ( 'NONE',  ( -12.81628187352647963, -16.08469866340291077, -3.434112377981046293 ) ) ;
#52439=VERTEX_POINT ( 'NONE', #73565 ) ;
#52444=ORIENTED_EDGE ( 'NONE', *, *, #58022, .F. ) ;
#52449=CARTESIAN_POINT ( 'NONE',  ( 0.7375392941517004974, 14.49999999999999112, 14.98185688723477682 ) ) ;
#52451=DIRECTION ( 'NONE',  ( 0.000000000000000000, -0.000000000000000000, 1.000000000000000000 ) ) ;
#52455=CARTESIAN_POINT ( 'NONE',  ( -13.34343830728394309, 15.00000000000000000, -6.852200678592783589 ) ) ;
#52463=EDGE_CURVE ( 'NONE', #46092, #72566, #79607, .T. ) ;
#52467=DIRECTION ( 'NONE',  ( 0.000000000000000000, 0.000000000000000000, 1.000000000000000000 ) ) ;
#52476=CARTESIAN_POINT ( 'NONE',  ( -10.36894250292379205, -23.82125116508602858, -10.36894250292378672 ) ) ;
#52487=LINE ( 'NONE', #60482, #35860 ) ;
#52488=AXIS2_PLACEMENT_3D ( 'NONE', #64929, #87938, #81426 ) ;
#52491=CARTESIAN_POINT ( 'NONE',  ( -10.88017736071109987, 23.27201867748817676, 2.915334737309934532 ) ) ;
#52499=CARTESIAN_POINT ( 'NONE',  ( 13.21236992757670059, 15.00000000000000000, 5.338143956176803151 ) ) ;
#52500=AXIS2_PLACEMENT_3D ( 'NONE', #45403, #46399, #92871 ) ;
#52501=EDGE_CURVE ( 'NONE', #86688, #69641, #57094, .T. ) ;
#52508=CARTESIAN_POINT ( 'NONE',  ( 0.000000000000000000, 14.49999999999999822, 0.000000000000000000 ) ) ;
#52510=ORIENTED_EDGE ( 'NONE', *, *, #85065, .T. ) ;
#52526=VERTEX_POINT ( 'NONE', #42115 ) ;
#52540=DIRECTION ( 'NONE',  ( -0.000000000000000000, -1.000000000000000000, -0.000000000000000000 ) ) ;
#52541=CARTESIAN_POINT ( 'NONE',  ( 8.527530157486179263, 13.09226448433412848, 4.923371831947292776 ) ) ;
#52543=ORIENTED_EDGE ( 'NONE', *, *, #3396, .T. ) ;
#52544=APPLICATION_CONTEXT ( 'automotive_design' ) ;
#52546=ORIENTED_EDGE ( 'NONE', *, *, #21255, .T. ) ;
#52558=ORIENTED_EDGE ( 'NONE', *, *, #64785, .F. ) ;
#52568=VECTOR ( 'NONE', #60040, 1000.000000000000000 ) ;
#52573=VERTEX_POINT ( 'NONE', #27576 ) ;
#52582=ORIENTED_EDGE ( 'NONE', *, *, #58254, .F. ) ;
#52583=CARTESIAN_POINT ( 'NONE',  ( -11.92686044187655980, 4.896642702460838770, 3.195792623639539087 ) ) ;
#52585=CARTESIAN_POINT ( 'NONE',  ( 6.715867195167446901, 15.00000000000000000, -12.85095824508324469 ) ) ;
#52592=CARTESIAN_POINT ( 'NONE',  ( -13.55255535720598026, 0.000000000000000000, 4.403492169842870396 ) ) ;
#52594=EDGE_LOOP ( 'NONE', ( #41017, #55960, #84585, #12805, #30016, #43554 ) ) ;
#52603=DIRECTION ( 'NONE',  ( 0.000000000000000000, 0.000000000000000000, 1.000000000000000000 ) ) ;
#52608=CARTESIAN_POINT ( 'NONE',  ( 10.88017736071110519, -9.436314655845157162, -2.602085213965210642E-15 ) ) ;
#52612=CARTESIAN_POINT ( 'NONE',  ( 14.69227023463708548, 14.95077488074853456, 1.335400878252637646 ) ) ;
#52613=VECTOR ( 'NONE', #56321, 1000.000000000000227 ) ;
#52614=CARTESIAN_POINT ( 'NONE',  ( 2.120353041430552921, 4.509079855230530718E-16, 14.34413130794947122 ) ) ;
#52633=CARTESIAN_POINT ( 'NONE',  ( -0.3093388210927642268, 15.00000000000000000, 14.99680997725065978 ) ) ;
#52636=B_SPLINE_CURVE_WITH_KNOTS ( 'NONE', 3,
 ( #14758, #92211, #749, #22252, #7746, #53227 ),
 .UNSPECIFIED., .F., .F.,
 ( 4, 2, 4 ),
 ( 0.0002800484630364006439, 0.0006862541666483321437, 0.001092459870260263644 ),
 .UNSPECIFIED. ) ;
#52637=DIRECTION ( 'NONE',  ( 0.000000000000000000, 1.000000000000000000, -0.000000000000000000 ) ) ;
#52640=VERTEX_POINT ( 'NONE', #24054 ) ;
#52656=CARTESIAN_POINT ( 'NONE',  ( -2.638427012816840111, -20.03273551566587685, -9.846743663894590881 ) ) ;
#52658=CYLINDRICAL_SURFACE ( 'NONE', #90673, 15.00000000000000000 ) ;
#52659=ORIENTED_EDGE ( 'NONE', *, *, #19318, .F. ) ;
#52661=AXIS2_PLACEMENT_3D ( 'NONE', #52798, #76296, #45303 ) ;
#52663=CARTESIAN_POINT ( 'NONE',  ( 1.180296924652878499, 0.000000000000000000, 5.323975374878061828 ) ) ;
#52672=CARTESIAN_POINT ( 'NONE',  ( 3.434112377981060948, 15.58196800326375353, 12.81628187352647430 ) ) ;
#52683=LINE ( 'NONE', #97725, #71934 ) ;
#52689=CARTESIAN_POINT ( 'NONE',  ( -12.00809552683971759, 14.49999999999999112, 8.989195838243478676 ) ) ;
#52699=CARTESIAN_POINT ( 'NONE',  ( -11.49658347684252924, 14.95037108522090463, -9.245857368724228920 ) ) ;
#52710=DIRECTION ( 'NONE',  ( 0.000000000000000000, 1.000000000000000000, 0.000000000000000000 ) ) ;
#52713=DIRECTION ( 'NONE',  ( 0.000000000000000000, 1.000000000000000000, 0.000000000000000000 ) ) ;
#52717=CYLINDRICAL_SURFACE ( 'NONE', #23296, 15.00000000000000000 ) ;
#52718=DIRECTION ( 'NONE',  ( 0.000000000000000000, 1.000000000000000000, 0.000000000000000000 ) ) ;
#52719=AXIS2_PLACEMENT_3D ( 'NONE', #91617, #61108, #77096 ) ;
#52721=DIRECTION ( 'NONE',  ( -0.000000000000000000, -1.000000000000000000, -0.000000000000000000 ) ) ;
#52724=CARTESIAN_POINT ( 'NONE',  ( -3.795296366450322534, 20.76208216824731068, -14.16423886937409904 ) ) ;
#52731=CYLINDRICAL_SURFACE ( 'NONE', #77641, 11.25000000000000178 ) ;
#52734=EDGE_CURVE ( 'NONE', #51220, #40543, #90105, .T. ) ;
#52751=CARTESIAN_POINT ( 'NONE',  ( -12.22474924877152347, 0.2301506569030525307, 8.589397507024811418 ) ) ;
#52759=AXIS2_PLACEMENT_3D ( 'NONE', #21733, #76201, #15222 ) ;
#52761=DIRECTION ( 'NONE',  ( 0.7132504491541801217, 0.000000000000000000, 0.7009092642998523415 ) ) ;
#52779=ORIENTED_EDGE ( 'NONE', *, *, #80844, .T. ) ;
#52783=EDGE_CURVE ( 'NONE', #59056, #29326, #96656, .T. ) ;
#52784=ORIENTED_EDGE ( 'NONE', *, *, #63758, .F. ) ;
#52787=ORIENTED_EDGE ( 'NONE', *, *, #91387, .T. ) ;
#52790=CARTESIAN_POINT ( 'NONE',  ( 7.771322705631417804, 3.835866486557528145E-16, 12.24159072199922704 ) ) ;
#52792=AXIS2_PLACEMENT_3D ( 'NONE', #37527, #50539, #28528 ) ;
#52796=DIRECTION ( 'NONE',  ( 5.506706202140776441E-14, 0.000000000000000000, 1.000000000000000000 ) ) ;
#52798=CARTESIAN_POINT ( 'NONE',  ( -13.21236992757677164, -0.03417435944610275333, 5.338143956176621074 ) ) ;
#52800=AXIS2_PLACEMENT_3D ( 'NONE', #5212, #50702, #81196 ) ;
#52803=DIRECTION ( 'NONE',  ( 0.000000000000000000, 0.000000000000000000, -1.000000000000000000 ) ) ;
#52805=FACE_OUTER_BOUND ( 'NONE', #72487, .T. ) ;
#52809=DIRECTION ( 'NONE',  ( -0.000000000000000000, -1.000000000000000000, -0.000000000000000000 ) ) ;
#52821=EDGE_CURVE ( 'NONE', #3216, #31971, #36359, .T. ) ;
#52829=EDGE_CURVE ( 'NONE', #91269, #44178, #23375, .T. ) ;
#52841=ORIENTED_EDGE ( 'NONE', *, *, #39625, .T. ) ;
#52862=ORIENTED_EDGE ( 'NONE', *, *, #93509, .F. ) ;
#52869=CARTESIAN_POINT ( 'NONE',  ( 9.065164099344453774, 15.00000000000000000, 11.95084933600773169 ) ) ;
#52874=CARTESIAN_POINT ( 'NONE',  ( -2.863771337576625609, 0.04962896698837778592, 14.47259902956226618 ) ) ;
#52875=CARTESIAN_POINT ( 'NONE',  ( -1.909764518474497796, 0.000000000000000000, 5.107897229450579779 ) ) ;
#52881=CARTESIAN_POINT ( 'NONE',  ( -7.993487411953518418, 14.95037111676103869, 12.40005926694992766 ) ) ;
#52886=FACE_OUTER_BOUND ( 'NONE', #8996, .T. ) ;
#52889=VERTEX_POINT ( 'NONE', #95383 ) ;
#52907=ORIENTED_EDGE ( 'NONE', *, *, #54085, .F. ) ;
#52909=CARTESIAN_POINT ( 'NONE',  ( 3.469446951953614189E-15, -14.62636533006957151, 12.81628187352647608 ) ) ;
#52912=VECTOR ( 'NONE', #29589, 999.9999999999998863 ) ;
#52920=CARTESIAN_POINT ( 'NONE',  ( -9.820177974736244764, 0.2301504389881804946, -11.25994418464066271 ) ) ;
#52921=ORIENTED_EDGE ( 'NONE', *, *, #76902, .F. ) ;
#52927=ORIENTED_EDGE ( 'NONE', *, *, #77475, .F. ) ;
#52929=AXIS2_PLACEMENT_3D ( 'NONE', #46611, #166, #22653 ) ;
#52937=DIRECTION ( 'NONE',  ( -0.000000000000000000, 1.000000000000000000, -0.000000000000000000 ) ) ;
#52940=ORIENTED_EDGE ( 'NONE', *, *, #5001, .F. ) ;
#52946=ADVANCED_FACE ( 'NONE', ( #37362 ), #60825, .F. ) ;
#52956=DIRECTION ( 'NONE',  ( 0.000000000000000000, 1.000000000000000000, 0.000000000000000000 ) ) ;
#52964=CARTESIAN_POINT ( 'NONE',  ( 14.16423886937410259, -15.69625116508602680, -2.602085213965210642E-15 ) ) ;
#52971=CARTESIAN_POINT ( 'NONE',  ( 10.76445796113278419, 14.99999999999804601, 9.901260316216218271 ) ) ;
#52974=LINE ( 'NONE', #36510, #33683 ) ;
#52977=CARTESIAN_POINT ( 'NONE',  ( 13.55255535720591986, -0.03417435944610275333, 4.403492169843056914 ) ) ;
#52980=CARTESIAN_POINT ( 'NONE',  ( 2.915334737309928315, 29.52201867748817676, 10.88017736071109987 ) ) ;
#52985=DIRECTION ( 'NONE',  ( -0.8038568606172123987, 0.000000000000000000, -0.5948227867513479206 ) ) ;
#53010=AXIS2_PLACEMENT_3D ( 'NONE', #44585, #28098, #67599 ) ;
#53020=CARTESIAN_POINT ( 'NONE',  ( 3.843542995449403588, 14.76984992748860748, 14.43777707753016948 ) ) ;
#53027=CARTESIAN_POINT ( 'NONE',  ( 9.011287250621712985, 14.76930270348881002, 11.91783356064793686 ) ) ;
#53028=CARTESIAN_POINT ( 'NONE',  ( -3.469446951953614189E-15, 14.75893115100079100, -9.846743663894594434 ) ) ;
#53029=ORIENTED_EDGE ( 'NONE', *, *, #69915, .T. ) ;
#53030=ORIENTED_EDGE ( 'NONE', *, *, #61404, .T. ) ;
#53032=ORIENTED_EDGE ( 'NONE', *, *, #81374, .T. ) ;
#53042=ORIENTED_EDGE ( 'NONE', *, *, #94363, .T. ) ;
#53052=DIRECTION ( 'NONE',  ( 0.000000000000000000, 1.000000000000000000, 0.000000000000000000 ) ) ;
#53053=EDGE_CURVE ( 'NONE', #98886, #21745, #30820, .T. ) ;
#53055=FACE_OUTER_BOUND ( 'NONE', #9254, .T. ) ;
#53056=CARTESIAN_POINT ( 'NONE',  ( 14.26139399675174957, 15.00000000000000000, 2.619664342934486356 ) ) ;
#53057=AXIS2_PLACEMENT_3D ( 'NONE', #82696, #43209, #21214 ) ;
#53065=TOROIDAL_SURFACE ( 'NONE', #62621, 14.49999999999999822, 0.5000000000000000000 ) ;
#53068=DIRECTION ( 'NONE',  ( 0.000000000000000000, 0.000000000000000000, -1.000000000000000000 ) ) ;
#53074=EDGE_LOOP ( 'NONE', ( #50577, #61637, #9536, #43236 ) ) ;
#53084=VECTOR ( 'NONE', #79200, 1000.000000000000114 ) ;
#53086=ADVANCED_FACE ( 'NONE', ( #67351 ), #15225, .T. ) ;
#53087=ORIENTED_EDGE ( 'NONE', *, *, #43631, .T. ) ;
#53096=EDGE_CURVE ( 'NONE', #91322, #44682, #75836, .T. ) ;
#53098=VECTOR ( 'NONE', #30660, 1000.000000000000000 ) ;
#53102=CARTESIAN_POINT ( 'NONE',  ( -5.204170427930421283E-15, -13.18631465584516071, -10.88017736071110342 ) ) ;
#53107=DIRECTION ( 'NONE',  ( 0.000000000000000000, 0.000000000000000000, -1.000000000000000000 ) ) ;
#53111=VECTOR ( 'NONE', #19844, 1000.000000000000000 ) ;
#53151=CARTESIAN_POINT ( 'NONE',  ( -8.527530157486173934, -28.57440218233254470, 4.923371831947302546 ) ) ;
#53152=ORIENTED_EDGE ( 'NONE', *, *, #65118, .F. ) ;
#53154=AXIS2_PLACEMENT_3D ( 'NONE', #42780, #27267, #34770 ) ;
#53157=ORIENTED_EDGE ( 'NONE', *, *, #13791, .T. ) ;
#53158=LINE ( 'NONE', #67685, #42496 ) ;
#53164=EDGE_CURVE ( 'NONE', #50602, #89674, #83342, .T. ) ;
#53167=CARTESIAN_POINT ( 'NONE',  ( -6.408140936763232709, 14.95696800326375886, 11.09922568453595026 ) ) ;
#53171=VERTEX_POINT ( 'NONE', #31307 ) ;
#53177=CARTESIAN_POINT ( 'NONE',  ( 0.000000000000000000, 15.00000000000000000, 0.000000000000000000 ) ) ;
#53180=VECTOR ( 'NONE', #4671, 1000.000000000000114 ) ;
#53182=ORIENTED_EDGE ( 'NONE', *, *, #33793, .T. ) ;
#53187=CARTESIAN_POINT ( 'NONE',  ( 0.000000000000000000, 14.49999999999999822, 0.000000000000000000 ) ) ;
#53191=DIRECTION ( 'NONE',  ( -0.9099612708765398850, 0.000000000000000000, -0.4146932426562461860 ) ) ;
#53192=ADVANCED_FACE ( 'NONE', ( #32786 ), #16861, .T. ) ;
#53194=DIRECTION ( 'NONE',  ( -0.3173046564050833740, 0.000000000000000000, -0.9483236552062023206 ) ) ;
#53195=CARTESIAN_POINT ( 'NONE',  ( -5.991992585808429972, 15.00000000000000000, -13.20401548210301357 ) ) ;
#53196=FACE_OUTER_BOUND ( 'NONE', #62735, .T. ) ;
#53207=ORIENTED_EDGE ( 'NONE', *, *, #11057, .F. ) ;
#53208=B_SPLINE_CURVE_WITH_KNOTS ( 'NONE', 3,
 ( #85194, #63651, #56178, #9192, #78176, #9687 ),
 .UNSPECIFIED., .F., .F.,
 ( 4, 2, 4 ),
 ( 0.0002800065468393059492, 0.0006862118402932819439, 0.001092417133747257884 ),
 .UNSPECIFIED. ) ;
#53210=CIRCLE ( 'NONE', #64401, 13.74999999999999467 ) ;
#53220=DIRECTION ( 'NONE',  ( 0.6225146366376183016, 0.000000000000000000, -0.7826081568524148047 ) ) ;
#53223=CARTESIAN_POINT ( 'NONE',  ( -1.915564264621539392, 15.00000000000000000, 14.37291249357986445 ) ) ;
#53224=CARTESIAN_POINT ( 'NONE',  ( -12.26659068614895354, 26.38708216824731068, -7.082119434687038861 ) ) ;
#53227=CARTESIAN_POINT ( 'NONE',  ( 3.420591144908583736, 14.49999999999999112, -14.60477854057961800 ) ) ;
#53255=ORIENTED_EDGE ( 'NONE', *, *, #20020, .T. ) ;
#53256=ORIENTED_EDGE ( 'NONE', *, *, #86497, .T. ) ;
#53278=EDGE_CURVE ( 'NONE', #14929, #1780, #28123, .T. ) ;
#53279=CARTESIAN_POINT ( 'NONE',  ( 3.836325488036181675, 14.63595249122789177, -14.50112432709423693 ) ) ;
#53280=VERTEX_POINT ( 'NONE', #70318 ) ;
#53283=ORIENTED_EDGE ( 'NONE', *, *, #79035, .F. ) ;
#53292=CARTESIAN_POINT ( 'NONE',  ( 1.377727649040772586E-15, 15.00000000000000000, 11.25000000000000178 ) ) ;
#53299=CARTESIAN_POINT ( 'NONE',  ( -1.236172813752466570, 0.04922511925147319417, 14.70095156538447867 ) ) ;
#53313=PLANE ( 'NONE',  #98279 ) ;
#53329=EDGE_CURVE ( 'NONE', #87207, #67193, #71302, .T. ) ;
#53332=CARTESIAN_POINT ( 'NONE',  ( 0.000000000000000000, 15.00000000000000000, 0.000000000000000000 ) ) ;
#53333=CARTESIAN_POINT ( 'NONE',  ( -10.58981376305295008, -0.03417435944610275333, 9.535111140613638625 ) ) ;
#53345=LINE ( 'NONE', #67874, #32663 ) ;
#53353=VECTOR ( 'NONE', #17207, 1000.000000000000227 ) ;
#53354=CARTESIAN_POINT ( 'NONE',  ( 0.000000000000000000, 0.5000000000000004441, 0.000000000000000000 ) ) ;
#53355=CARTESIAN_POINT ( 'NONE',  ( 11.75209714983967935, 14.95077488074854166, 8.918201205062084469 ) ) ;
#53365=CARTESIAN_POINT ( 'NONE',  ( 14.64885433385999569, 14.95077488074853456, -1.748475581354204333 ) ) ;
#53366=LINE ( 'NONE', #13401, #69063 ) ;
#53381=EDGE_LOOP ( 'NONE', ( #35237, #21776, #75047, #98709, #94018, #97885 ) ) ;
#53389=VERTEX_POINT ( 'NONE', #20750 ) ;
#53399=CARTESIAN_POINT ( 'NONE',  ( -13.86186289918438952, 5.522654816098036239E-16, -4.667665767315160252 ) ) ;
#53401=ORIENTED_EDGE ( 'NONE', *, *, #28910, .F. ) ;
#53403=CARTESIAN_POINT ( 'NONE',  ( -12.81628187352647608, -0.8763653300695728454, 3.903127820947815962E-15 ) ) ;
#53411=EDGE_CURVE ( 'NONE', #7169, #69512, #88250, .T. ) ;
#53419=ADVANCED_FACE ( 'NONE', ( #65740 ), #8914, .T. ) ;
#53420=VERTEX_POINT ( 'NONE', #72744 ) ;
#53432=ORIENTED_EDGE ( 'NONE', *, *, #85870, .F. ) ;
#53447=DIRECTION ( 'NONE',  ( 0.000000000000000000, 0.000000000000000000, 1.000000000000000000 ) ) ;
#53452=CARTESIAN_POINT ( 'NONE',  ( 0.000000000000000000, 0.000000000000000000, 0.000000000000000000 ) ) ;
#53456=CARTESIAN_POINT ( 'NONE',  ( -12.26659068614894110, -7.779584498419360727, 7.082119434687058401 ) ) ;
#53469=CARTESIAN_POINT ( 'NONE',  ( 1.354709868695521013, 14.63595249122789177, 14.93870011653153540 ) ) ;
#53473=CARTESIAN_POINT ( 'NONE',  ( 10.88017736071109987, 25.77201867748818032, -2.915334737309928315 ) ) ;
#53490=CARTESIAN_POINT ( 'NONE',  ( -14.99847009497950800, 14.49999999999999112, -0.2142307401082109986 ) ) ;
#53491=EDGE_CURVE ( 'NONE', #67824, #78138, #95121, .T. ) ;
#53507=EDGE_CURVE ( 'NONE', #21503, #60570, #35242, .T. ) ;
#53510=ORIENTED_EDGE ( 'NONE', *, *, #63145, .F. ) ;
#53516=CARTESIAN_POINT ( 'NONE',  ( 0.000000000000000000, 2.500000000000005773, 0.000000000000000000 ) ) ;
#53524=CARTESIAN_POINT ( 'NONE',  ( -7.208316651077756099, 31.63393115100080166, 7.208316651077766757 ) ) ;
#53535=CIRCLE ( 'NONE', #2468, 15.00000000000000000 ) ;
#53541=ADVANCED_FACE ( 'NONE', ( #21245 ), #82352, .T. ) ;
#53549=CARTESIAN_POINT ( 'NONE',  ( 12.15129255554608534, -0.03417435944610275333, 10.40305174771247998 ) ) ;
#53552=ORIENTED_EDGE ( 'NONE', *, *, #36481, .T. ) ;
#53554=ORIENTED_EDGE ( 'NONE', *, *, #32943, .F. ) ;
#53556=CIRCLE ( 'NONE', #75909, 15.00000000000000000 ) ;
#53557=CARTESIAN_POINT ( 'NONE',  ( 0.000000000000000000, 15.00000000000000000, 0.000000000000000000 ) ) ;
#53572=CARTESIAN_POINT ( 'NONE',  ( 7.674335239599288983, 14.76930270348881180, -12.81961907869216333 ) ) ;
#53575=TOROIDAL_SURFACE ( 'NONE', #15287, 14.49999999999999822, 0.5000000000000000000 ) ;
#53577=B_SPLINE_CURVE_WITH_KNOTS ( 'NONE', 3,
 ( #46597, #53607, #39612, #1626, #23134, #39116 ),
 .UNSPECIFIED., .F., .F.,
 ( 4, 2, 4 ),
 ( 0.0002800111042666518849, 0.0006862164423004496472, 0.001092421780334247410 ),
 .UNSPECIFIED. ) ;
#53578=EDGE_LOOP ( 'NONE', ( #56698, #9610, #76390, #95833 ) ) ;
#53587=DIRECTION ( 'NONE',  ( 0.000000000000000000, 1.000000000000000000, 0.000000000000000000 ) ) ;
#53591=CARTESIAN_POINT ( 'NONE',  ( -2.915334737309917656, -5.894647989178490199, 10.88017736071110164 ) ) ;
#53597=DIRECTION ( 'NONE',  ( 0.4771587602595978028, 0.000000000000000000, 0.8788171126619711560 ) ) ;
#53600=B_SPLINE_CURVE_WITH_KNOTS ( 'NONE', 3,
 ( #81092, #12593, #32754, #80608, #17289, #43093 ),
 .UNSPECIFIED., .F., .F.,
 ( 4, 2, 4 ),
 ( 0.0002800858945027110639, 0.0006862919646584216167, 0.001092498034814132169 ),
 .UNSPECIFIED. ) ;
#53602=CARTESIAN_POINT ( 'NONE',  ( -12.25993886608593364, 15.00000000000000000, -8.642563219313787570 ) ) ;
#53604=CIRCLE ( 'NONE', #36048, 14.49999999999999822 ) ;
#53607=CARTESIAN_POINT ( 'NONE',  ( 9.281709892946475193, -3.106493334055145310E-15, -11.30302492080705967 ) ) ;
#53609=VERTEX_POINT ( 'NONE', #49751 ) ;
#53618=CARTESIAN_POINT ( 'NONE',  ( 0.7375392941517004974, 14.49999999999999112, 14.98185688723477682 ) ) ;
#53625=ORIENTED_EDGE ( 'NONE', *, *, #25776, .T. ) ;
#53632=DIRECTION ( 'NONE',  ( 0.09584575252022037306, -0.000000000000000000, 0.9953961983671790748 ) ) ;
#53641=B_SPLINE_CURVE_WITH_KNOTS ( 'NONE', 3,
 ( #62709, #24732, #17727, #8732, #55210, #39250 ),
 .UNSPECIFIED., .F., .F.,
 ( 4, 2, 4 ),
 ( 0.0002800032591452409876, 0.0006862085204420063315, 0.001092413781738771567 ),
 .UNSPECIFIED. ) ;
#53642=DIRECTION ( 'NONE',  ( -0.6494480483301799945, 0.000000000000000000, -0.7604059656000340395 ) ) ;
#53645=CARTESIAN_POINT ( 'NONE',  ( -3.469446951953614189E-15, -20.24106884899921255, -9.846743663894594434 ) ) ;
#53646=ORIENTED_EDGE ( 'NONE', *, *, #34055, .F. ) ;
#53659=CARTESIAN_POINT ( 'NONE',  ( -5.204170427930421283E-15, 17.87363466993041783, -12.81628187352647608 ) ) ;
#53660=ORIENTED_EDGE ( 'NONE', *, *, #95142, .F. ) ;
#53662=ADVANCED_FACE ( 'NONE', ( #12253 ), #79145, .T. ) ;
#53671=EDGE_CURVE ( 'NONE', #3928, #29178, #89242, .T. ) ;
#53673=LINE ( 'NONE', #217, #54080 ) ;
#53675=CARTESIAN_POINT ( 'NONE',  ( -9.065164099344370285, 0.5000000000000004441, -11.95084933600779564 ) ) ;
#53681=CARTESIAN_POINT ( 'NONE',  ( -9.065164099344613646, 15.00000000000000000, 11.95084933600761445 ) ) ;
#53682=CYLINDRICAL_SURFACE ( 'NONE', #15568, 15.00000000000000000 ) ;
#53683=ORIENTED_EDGE ( 'NONE', *, *, #16159, .F. ) ;
#53688=CARTESIAN_POINT ( 'NONE',  ( 0.000000000000000000, 0.000000000000000000, 0.000000000000000000 ) ) ;
#53695=CARTESIAN_POINT ( 'NONE',  ( -5.204170427930421283E-15, 6.412123368507812948, -11.92686044187656513 ) ) ;
#53697=VECTOR ( 'NONE', #79259, 1000.000000000000000 ) ;
#53698=ORIENTED_EDGE ( 'NONE', *, *, #8089, .T. ) ;
#53705=CARTESIAN_POINT ( 'NONE',  ( 13.74344568549453527, 14.76984872681200756, 5.860030649989749207 ) ) ;
#53712=CARTESIAN_POINT ( 'NONE',  ( 10.36894250292379027, 18.67874883491397142, 10.36894250292378672 ) ) ;
#53722=VECTOR ( 'NONE', #31411, 999.9999999999998863 ) ;
#53730=DIRECTION ( 'NONE',  ( 0.000000000000000000, 0.000000000000000000, 1.000000000000000000 ) ) ;
#53745=CARTESIAN_POINT ( 'NONE',  ( 5.810202895580367510, 0.04922511925147131373, 13.56051778013769393 ) ) ;
#53749=CARTESIAN_POINT ( 'NONE',  ( -5.073789285385954528, 0.000000000000000000, -1.998618750576442338 ) ) ;
#53750=EDGE_CURVE ( 'NONE', #57430, #26946, #67953, .T. ) ;
#53751=EDGE_LOOP ( 'NONE', ( #36218, #32077, #88112, #32108 ) ) ;
#53753=CARTESIAN_POINT ( 'NONE',  ( -14.97687855664608847, 0.5000000000000004441, 0.8325315005899532883 ) ) ;
#53754=CARTESIAN_POINT ( 'NONE',  ( 14.54804176595378706, 15.00000000000000000, 6.650705016170673112 ) ) ;
#53761=EDGE_CURVE ( 'NONE', #77766, #41488, #91712, .T. ) ;
#53762=AXIS2_PLACEMENT_3D ( 'NONE', #18446, #71456, #34907 ) ;
#53765=CARTESIAN_POINT ( 'NONE',  ( 4.698669664746514485, 0.000000000000000000, -2.767727949825255163 ) ) ;
#53769=VERTEX_POINT ( 'NONE', #6732 ) ;
#53773=CIRCLE ( 'NONE', #7459, 14.49999999999999822 ) ;
#53781=AXIS2_PLACEMENT_3D ( 'NONE', #82587, #98104, #94515 ) ;
#53785=EDGE_CURVE ( 'NONE', #17162, #93214, #248, .T. ) ;
#53787=ORIENTED_EDGE ( 'NONE', *, *, #72367, .F. ) ;
#53791=CARTESIAN_POINT ( 'NONE',  ( 8.564643372776536978, 15.00000000000000000, 12.31449893000746343 ) ) ;
#53795=AXIS2_PLACEMENT_3D ( 'NONE', #56355, #88320, #80325 ) ;
#53797=AXIS2_PLACEMENT_3D ( 'NONE', #96681, #28159, #36154 ) ;
#53799=ORIENTED_EDGE ( 'NONE', *, *, #52387, .T. ) ;
#53800=CIRCLE ( 'NONE', #45812, 14.49999999999999822 ) ;
#53807=DIRECTION ( 'NONE',  ( 0.9588197348681928300, 0.000000000000000000, 0.2840153447039234780 ) ) ;
#53812=LINE ( 'NONE', #84323, #38816 ) ;
#53816=DIRECTION ( 'NONE',  ( 0.000000000000000000, 1.000000000000000000, 0.000000000000000000 ) ) ;
#53827=VECTOR ( 'NONE', #97071, 1000.000000000000000 ) ;
#53833=CARTESIAN_POINT ( 'NONE',  ( 0.000000000000000000, 0.5000000000000004441, 0.000000000000000000 ) ) ;
#53834=CARTESIAN_POINT ( 'NONE',  ( -3.115783986955370732, 3.816680036666981737E-16, -14.16128137375401685 ) ) ;
#53839=EDGE_CURVE ( 'NONE', #43481, #21313, #22733, .T. ) ;
#53841=CARTESIAN_POINT ( 'NONE',  ( -13.14228782657329653, 0.5000000000000004441, -7.230509711182418364 ) ) ;
#53844=CIRCLE ( 'NONE', #36284, 14.49999999999999822 ) ;
#53847=ORIENTED_EDGE ( 'NONE', *, *, #17613, .F. ) ;
#53849=AXIS2_PLACEMENT_3D ( 'NONE', #26034, #79022, #33505 ) ;
#53852=CARTESIAN_POINT ( 'NONE',  ( -11.61621867929619611, 15.00000000000000000, 10.99731149103378058 ) ) ;
#53859=EDGE_LOOP ( 'NONE', ( #49294, #54874, #78104, #85678 ) ) ;
#53866=CARTESIAN_POINT ( 'NONE',  ( 9.876730923139357188, 14.49999999999999112, -11.28938378619066363 ) ) ;
#53878=AXIS2_PLACEMENT_3D ( 'NONE', #61492, #76013, #68030 ) ;
#53885=EDGE_CURVE ( 'NONE', #52058, #16281, #61686, .T. ) ;
#53905=EDGE_LOOP ( 'NONE', ( #28656, #60134, #20192, #798, #38668, #61233 ) ) ;
#53910=DIRECTION ( 'NONE',  ( 0.8141155183563107967, 0.000000000000000000, 0.5807029557109515405 ) ) ;
#53915=ADVANCED_FACE ( 'NONE', ( #21750 ), #52717, .T. ) ;
#53918=ORIENTED_EDGE ( 'NONE', *, *, #8830, .F. ) ;
#53922=ORIENTED_EDGE ( 'NONE', *, *, #3663, .T. ) ;
#53926=DIRECTION ( 'NONE',  ( 0.9366721892484018985, 0.000000000000000000, -0.3502073812594559410 ) ) ;
#53927=VECTOR ( 'NONE', #20392, 1000.000000000000000 ) ;
#53929=CARTESIAN_POINT ( 'NONE',  ( -9.065164099344613646, 0.5000000000000004441, 11.95084933600761445 ) ) ;
#53933=LINE ( 'NONE', #76922, #92998 ) ;
#53938=CARTESIAN_POINT ( 'NONE',  ( 11.25000000000000000, 2.826366962315984832, -3.014428414850133908 ) ) ;
#53948=CARTESIAN_POINT ( 'NONE',  ( -9.742785792574931492, 10.53470029564931920, 5.625000000000008882 ) ) ;
#53952=CARTESIAN_POINT ( 'NONE',  ( -7.684764310694971456, 14.49999999999999822, 12.88194075009929840 ) ) ;
#53958=CARTESIAN_POINT ( 'NONE',  ( -5.204170427930421283E-15, -4.446251165086026802, -14.16423886937410082 ) ) ;
#53969=DIRECTION ( 'NONE',  ( 0.000000000000000000, 0.000000000000000000, 1.000000000000000000 ) ) ;
#53972=CARTESIAN_POINT ( 'NONE',  ( 0.3093388210927642268, 14.49999999999999822, -14.99680997725065978 ) ) ;
#53982=DIRECTION ( 'NONE',  ( 0.04361938736534638067, 0.000000000000000000, -0.9990482215818573541 ) ) ;
#53989=FACE_OUTER_BOUND ( 'NONE', #33498, .T. ) ;
#53990=FACE_OUTER_BOUND ( 'NONE', #8921, .T. ) ;
#53998=AXIS2_PLACEMENT_3D ( 'NONE', #96086, #79600, #34566 ) ;
#54022=CARTESIAN_POINT ( 'NONE',  ( -9.846743663894594434, 31.00893115100078390, 3.469446951953614189E-15 ) ) ;
#54023=ORIENTED_EDGE ( 'NONE', *, *, #48685, .F. ) ;
#54024=VERTEX_POINT ( 'NONE', #33157 ) ;
#54033=ORIENTED_EDGE ( 'NONE', *, *, #70683, .F. ) ;
#54036=ORIENTED_EDGE ( 'NONE', *, *, #19580, .T. ) ;
#54038=EDGE_CURVE ( 'NONE', #15924, #82423, #53208, .T. ) ;
#54039=VERTEX_POINT ( 'NONE', #86671 ) ;
#54045=CARTESIAN_POINT ( 'NONE',  ( -4.391700990647259495, 0.2306972965111845908, 14.28114200970186687 ) ) ;
#54050=EDGE_LOOP ( 'NONE', ( #31591, #70075, #38651, #7519 ) ) ;
#54052=PLANE ( 'NONE',  #88025 ) ;
#54054=CARTESIAN_POINT ( 'NONE',  ( -2.393480905993287777, 14.49999999999999112, 14.80781041047755409 ) ) ;
#54058=ORIENTED_EDGE ( 'NONE', *, *, #1205, .F. ) ;
#54069=EDGE_CURVE ( 'NONE', #91634, #48230, #62671, .T. ) ;
#54076=CARTESIAN_POINT ( 'NONE',  ( -13.82671409943298357, 15.00000000000000000, 3.447387012295131115 ) ) ;
#54080=VECTOR ( 'NONE', #16178, 1000.000000000000000 ) ;
#54083=CARTESIAN_POINT ( 'NONE',  ( 10.88017736071110519, 0.5636853441548448362, -2.602085213965210642E-15 ) ) ;
#54085=EDGE_CURVE ( 'NONE', #12575, #14459, #74630, .T. ) ;
#54095=DIRECTION ( 'NONE',  ( 0.9832549075639526182, 0.000000000000000000, 0.1822355254921578793 ) ) ;
#54099=EDGE_CURVE ( 'NONE', #73183, #25080, #47167, .T. ) ;
#54101=CARTESIAN_POINT ( 'NONE',  ( -12.67147417979180979, 0.04962887043496414657, 7.555862176155415888 ) ) ;
#54127=CARTESIAN_POINT ( 'NONE',  ( 4.923371831947295441, -5.657735515665875070, -8.527530157486179263 ) ) ;
#54128=ORIENTED_EDGE ( 'NONE', *, *, #14370, .F. ) ;
#54130=EDGE_LOOP ( 'NONE', ( #5935, #24995, #39405, #21821, #94354, #89656 ) ) ;
#54139=AXIS2_PLACEMENT_3D ( 'NONE', #80585, #12079, #36063 ) ;
#54140=CARTESIAN_POINT ( 'NONE',  ( 0.000000000000000000, 15.00000000000000000, 0.000000000000000000 ) ) ;
#54144=CARTESIAN_POINT ( 'NONE',  ( 11.09922568453595026, 26.20696800326376064, 6.408140936763232709 ) ) ;
#54148=VERTEX_POINT ( 'NONE', #71666 ) ;
#54153=CARTESIAN_POINT ( 'NONE',  ( 6.767445849361252819, 14.49999999999999112, -13.38662304974503492 ) ) ;
#54156=AXIS2_PLACEMENT_3D ( 'NONE', #53557, #39068, #68085 ) ;
#54164=FACE_OUTER_BOUND ( 'NONE', #76034, .T. ) ;
#54166=CARTESIAN_POINT ( 'NONE',  ( -5.795997163830251431, -0.03417435944610275333, 13.01802277140702024 ) ) ;
#54170=DIRECTION ( 'NONE',  ( 0.000000000000000000, 0.000000000000000000, 1.000000000000000000 ) ) ;
#54180=CARTESIAN_POINT ( 'NONE',  ( 12.50534872682727716, 15.00000000000000000, 7.339363270777608861 ) ) ;
#54183=EDGE_CURVE ( 'NONE', #61835, #75327, #77188, .T. ) ;
#54184=EDGE_CURVE ( 'NONE', #11472, #44083, #42475, .T. ) ;
#54185=EDGE_LOOP ( 'NONE', ( #70050, #76037, #55411, #74347 ) ) ;
#54186=DIRECTION ( 'NONE',  ( 0.000000000000000000, 1.000000000000000000, 0.000000000000000000 ) ) ;
#54191=CARTESIAN_POINT ( 'NONE',  ( -7.674241358950961711, 0.2301500950314201710, 12.81905807005879439 ) ) ;
#54192=CARTESIAN_POINT ( 'NONE',  ( 10.32896413005680181, 4.745456701841142433, 5.963430220938278126 ) ) ;
#54196=CARTESIAN_POINT ( 'NONE',  ( 1.780824192092400615, 0.3640475087720986824, 14.89391369643515617 ) ) ;
#54197=CARTESIAN_POINT ( 'NONE',  ( 14.16423886937410259, 24.30374883491398563, -2.602085213965210642E-15 ) ) ;
#54205=ORIENTED_EDGE ( 'NONE', *, *, #45864, .F. ) ;
#54211=CARTESIAN_POINT ( 'NONE',  ( -11.59580422753466422, 0.2301505044262088240, 9.421229451859115755 ) ) ;
#54217=EDGE_CURVE ( 'NONE', #54527, #59040, #92683, .T. ) ;
#54219=CARTESIAN_POINT ( 'NONE',  ( 14.09394518620612224, 15.00000000000000000, -3.407449058785360752 ) ) ;
#54220=CIRCLE ( 'NONE', #4771, 15.00000000000000000 ) ;
#54223=LINE ( 'NONE', #47212, #98503 ) ;
#54229=B_SPLINE_CURVE_WITH_KNOTS ( 'NONE', 3,
 ( #84351, #92327, #68362, #8824, #23358, #53841 ),
 .UNSPECIFIED., .F., .F.,
 ( 4, 2, 4 ),
 ( 0.0002800020636817308482, 0.0006862073132860410825, 0.001092412562890351154 ),
 .UNSPECIFIED. ) ;
#54254=VERTEX_POINT ( 'NONE', #64625 ) ;
#54256=EDGE_LOOP ( 'NONE', ( #53510, #60506, #22914, #65456 ) ) ;
#54263=EDGE_LOOP ( 'NONE', ( #53255, #13819, #46550, #75393, #52582, #52090 ) ) ;
#54264=VERTEX_POINT ( 'NONE', #43619 ) ;
#54268=CARTESIAN_POINT ( 'NONE',  ( -8.209432707284690878, 15.00000000000000000, -12.55409154915497183 ) ) ;
#54272=VERTEX_POINT ( 'NONE', #12626 ) ;
#54278=VERTEX_POINT ( 'NONE', #66116 ) ;
#54279=CARTESIAN_POINT ( 'NONE',  ( 8.235571585149870089, 11.99303362898264602, 8.235571585149868312 ) ) ;
#54280=VERTEX_POINT ( 'NONE', #27629 ) ;
#54284=FACE_OUTER_BOUND ( 'NONE', #20173, .T. ) ;
#54293=CIRCLE ( 'NONE', #51089, 14.49999999999999822 ) ;
#54300=EDGE_CURVE ( 'NONE', #6506, #91280, #29120, .T. ) ;
#54314=CARTESIAN_POINT ( 'NONE',  ( 1.983216688680936812, 0.000000000000000000, -14.11131997956737649 ) ) ;
#54315=DIRECTION ( 'NONE',  ( 0.000000000000000000, 0.000000000000000000, 1.000000000000000000 ) ) ;
#54319=CARTESIAN_POINT ( 'NONE',  ( 14.71525861348289865, 0.5000000000000004441, -2.908807992686582633 ) ) ;
#54331=ORIENTED_EDGE ( 'NONE', *, *, #94597, .T. ) ;
#54333=EDGE_CURVE ( 'NONE', #26776, #10227, #55241, .T. ) ;
#54334=DIRECTION ( 'NONE',  ( -0.6087614290087242086, 0.000000000000000000, 0.7933533402912323895 ) ) ;
#54340=CARTESIAN_POINT ( 'NONE',  ( -14.49440716394870599, 15.00000000000000000, -0.4026921475168267484 ) ) ;
#54351=VECTOR ( 'NONE', #13153, 1000.000000000000000 ) ;
#54359=VECTOR ( 'NONE', #45369, 1000.000000000000000 ) ;
#54362=CIRCLE ( 'NONE', #84707, 15.00000000000000000 ) ;
#54367=TOROIDAL_SURFACE ( 'NONE', #14422, 14.49999999999999822, 0.5000000000000000000 ) ;
#54372=ORIENTED_EDGE ( 'NONE', *, *, #33783, .F. ) ;
#54378=DIRECTION ( 'NONE',  ( -3.907985046680550391E-14, 0.000000000000000000, 1.000000000000000000 ) ) ;
#54381=ORIENTED_EDGE ( 'NONE', *, *, #76973, .F. ) ;
#54383=VECTOR ( 'NONE', #68614, 1000.000000000000114 ) ;
#54387=DIRECTION ( 'NONE',  ( 0.000000000000000000, 1.000000000000000000, 0.000000000000000000 ) ) ;
#54393=B_SPLINE_CURVE_WITH_KNOTS ( 'NONE', 3,
 ( #8834, #85325, #69842, #60848, #31817, #15861 ),
 .UNSPECIFIED., .F., .F.,
 ( 4, 2, 4 ),
 ( 3.409110551494648722E-05, 0.0004400426677367915589, 0.0008459942299586366374 ),
 .UNSPECIFIED. ) ;
#54401=CARTESIAN_POINT ( 'NONE',  ( 3.384479038598206646, 0.2301507000107690937, 14.55223509985380304 ) ) ;
#54405=CARTESIAN_POINT ( 'NONE',  ( -13.61802159414294877, -2.748198397366576661E-15, -5.334603887713678105 ) ) ;
#54408=CARTESIAN_POINT ( 'NONE',  ( 12.60874940350947959, 15.00000000000000000, -7.160268045227033973 ) ) ;
#54413=ORIENTED_EDGE ( 'NONE', *, *, #9646, .T. ) ;
#54435=LINE ( 'NONE', #75963, #65658 ) ;
#54438=CARTESIAN_POINT ( 'NONE',  ( 10.36894250292378850, -10.07125116508603213, -10.36894250292379027 ) ) ;
#54443=EDGE_CURVE ( 'NONE', #49035, #16296, #55071, .T. ) ;
#54444=CARTESIAN_POINT ( 'NONE',  ( -6.336100170400736253, 0.2301512019179792756, -13.53056138701896316 ) ) ;
#54446=DIRECTION ( 'NONE',  ( 0.000000000000000000, 1.000000000000000000, 0.000000000000000000 ) ) ;
#54451=DIRECTION ( 'NONE',  ( 0.000000000000000000, 1.000000000000000000, 0.000000000000000000 ) ) ;
#54453=CARTESIAN_POINT ( 'NONE',  ( 14.47650479471819551, 0.5000000000000004441, 3.928206833722108549 ) ) ;
#54455=LINE ( 'NONE', #92456, #83124 ) ;
#54462=ORIENTED_EDGE ( 'NONE', *, *, #33632, .T. ) ;
#54464=TOROIDAL_SURFACE ( 'NONE', #11358, 14.49999999999999822, 0.5000000000000000000 ) ;
#54474=CARTESIAN_POINT ( 'NONE',  ( 1.983216688680843109, 0.000000000000000000, 14.11131997956739070 ) ) ;
#54475=ORIENTED_EDGE ( 'NONE', *, *, #6805, .T. ) ;
#54489=VERTEX_POINT ( 'NONE', #93076 ) ;
#54494=CARTESIAN_POINT ( 'NONE',  ( -5.625000000000007994, 12.08846884451820891, -9.742785792574931492 ) ) ;
#54495=DIRECTION ( 'NONE',  ( 0.000000000000000000, 0.000000000000000000, 1.000000000000000000 ) ) ;
#54500=DIRECTION ( 'NONE',  ( -0.000000000000000000, -1.000000000000000000, -0.000000000000000000 ) ) ;
#54503=B_SPLINE_CURVE_WITH_KNOTS ( 'NONE', 3,
 ( #98985, #44462, #74964, #6468, #20990, #36973 ),
 .UNSPECIFIED., .F., .F.,
 ( 4, 2, 4 ),
 ( 0.0002800313526655974386, 0.0006862368888107541701, 0.001092442424955911064 ),
 .UNSPECIFIED. ) ;
#54505=CARTESIAN_POINT ( 'NONE',  ( -8.527530157486173934, 31.42559781766746241, 4.923371831947302546 ) ) ;
#54514=ADVANCED_FACE ( 'NONE', ( #9585 ), #77092, .T. ) ;
#54516=ORIENTED_EDGE ( 'NONE', *, *, #8919, .T. ) ;
#54519=ORIENTED_EDGE ( 'NONE', *, *, #67082, .T. ) ;
#54527=VERTEX_POINT ( 'NONE', #33545 ) ;
#54535=CARTESIAN_POINT ( 'NONE',  ( 3.836325488036075981, 14.49999999999999112, 14.50112432709431687 ) ) ;
#54548=FACE_OUTER_BOUND ( 'NONE', #15708, .T. ) ;
#54568=CARTESIAN_POINT ( 'NONE',  ( -10.88017736071109987, -1.727981322511823015, 2.915334737309934532 ) ) ;
#54574=ADVANCED_FACE ( 'NONE', ( #47587 ), #39608, .T. ) ;
#54584=PLANE ( 'NONE',  #52719 ) ;
#54598=ORIENTED_EDGE ( 'NONE', *, *, #68322, .T. ) ;
#54613=CARTESIAN_POINT ( 'NONE',  ( -3.469446951953614189E-15, -5.241068848999205443, -9.846743663894594434 ) ) ;
#54614=ORIENTED_EDGE ( 'NONE', *, *, #64037, .T. ) ;
#54615=ORIENTED_EDGE ( 'NONE', *, *, #14741, .T. ) ;
#54623=CARTESIAN_POINT ( 'NONE',  ( -13.21382278599129023, 15.00000000000000711, -6.271621331965704371 ) ) ;
#54629=VERTEX_POINT ( 'NONE', #2114 ) ;
#54630=VECTOR ( 'NONE', #27226, 1000.000000000000114 ) ;
#54631=TOROIDAL_SURFACE ( 'NONE', #11533, 14.49999999999999822, 0.5000000000000000000 ) ;
#54633=ORIENTED_EDGE ( 'NONE', *, *, #7823, .F. ) ;
#54635=ORIENTED_EDGE ( 'NONE', *, *, #12002, .F. ) ;
#54641=EDGE_CURVE ( 'NONE', #54903, #87966, #39111, .T. ) ;
#54645=FACE_OUTER_BOUND ( 'NONE', #98583, .T. ) ;
#54648=ORIENTED_EDGE ( 'NONE', *, *, #91343, .T. ) ;
#54657=DIRECTION ( 'NONE',  ( -0.000000000000000000, -1.000000000000000000, -0.000000000000000000 ) ) ;
#54667=CARTESIAN_POINT ( 'NONE',  ( 12.79413655343692469, 14.76984915707685886, 7.715718893782970156 ) ) ;
#54677=CARTESIAN_POINT ( 'NONE',  ( 13.07751017357376888, 15.00000000000000000, 6.263284095430594611 ) ) ;
#54682=CARTESIAN_POINT ( 'NONE',  ( -7.082119434687044190, 27.63708216824731068, 12.26659068614894998 ) ) ;
#54687=EDGE_CURVE ( 'NONE', #49707, #39559, #9092, .T. ) ;
#54701=AXIS2_PLACEMENT_3D ( 'NONE', #90454, #42997, #35491 ) ;
#54705=ORIENTED_EDGE ( 'NONE', *, *, #79645, .T. ) ;
#54707=LINE ( 'NONE', #93698, #78098 ) ;
#54714=AXIS2_PLACEMENT_3D ( 'NONE', #32801, #93312, #33292 ) ;
#54717=AXIS2_PLACEMENT_3D ( 'NONE', #55608, #63091, #27057 ) ;
#54727=DIRECTION ( 'NONE',  ( 0.000000000000000000, 1.000000000000000000, 0.000000000000000000 ) ) ;
#54731=EDGE_CURVE ( 'NONE', #42828, #26776, #20190, .T. ) ;
#54735=VECTOR ( 'NONE', #96495, 1000.000000000000114 ) ;
#54737=ORIENTED_EDGE ( 'NONE', *, *, #30255, .T. ) ;
#54738=VERTEX_POINT ( 'NONE', #31584 ) ;
#54748=VECTOR ( 'NONE', #35716, 999.9999999999998863 ) ;
#54749=EDGE_CURVE ( 'NONE', #7251, #71473, #56080, .T. ) ;
#54750=EDGE_CURVE ( 'NONE', #93052, #15452, #1024, .T. ) ;
#54757=PLANE ( 'NONE',  #19467 ) ;
#54763=DIRECTION ( 'NONE',  ( 0.000000000000000000, 0.000000000000000000, 1.000000000000000000 ) ) ;
#54766=DIRECTION ( 'NONE',  ( 0.000000000000000000, 1.000000000000000000, 0.000000000000000000 ) ) ;
#54771=ADVANCED_FACE ( 'NONE', ( #5044 ), #87212, .T. ) ;
#54780=FACE_OUTER_BOUND ( 'NONE', #64165, .T. ) ;
#54801=DIRECTION ( 'NONE',  ( -0.000000000000000000, -1.000000000000000000, -0.000000000000000000 ) ) ;
#54802=AXIS2_PLACEMENT_3D ( 'NONE', #92942, #83980, #31452 ) ;
#54804=CARTESIAN_POINT ( 'NONE',  ( 9.876730923139255935, 0.3639310091266618197, 11.28938378619071337 ) ) ;
#54809=DIRECTION ( 'NONE',  ( 0.000000000000000000, 0.000000000000000000, 1.000000000000000000 ) ) ;
#54810=B_SPLINE_CURVE_WITH_KNOTS ( 'NONE', 3,
 ( #19062, #11068, #49540, #64537, #35027, #48067 ),
 .UNSPECIFIED., .F., .F.,
 ( 4, 2, 4 ),
 ( 3.409110551496214716E-05, 0.0004400426677368003410, 0.0008459942299586385890 ),
 .UNSPECIFIED. ) ;
#54814=DIRECTION ( 'NONE',  ( 0.8433914458128921599, 0.000000000000000000, -0.5372996083468137840 ) ) ;
#54828=CARTESIAN_POINT ( 'NONE',  ( 14.29484424893241901, 0.2301500622783320127, 4.345072767107231115 ) ) ;
#54832=CARTESIAN_POINT ( 'NONE',  ( 5.147851794460816421, 14.99999999999795364, -13.68970903997665545 ) ) ;
#54836=EDGE_CURVE ( 'NONE', #6306, #11368, #47301, .T. ) ;
#54861=VERTEX_POINT ( 'NONE', #96545 ) ;
#54863=EDGE_CURVE ( 'NONE', #67942, #33221, #80042, .T. ) ;
#54865=CARTESIAN_POINT ( 'NONE',  ( 5.419894505350487002, 15.00000000000000000, 13.98659156302462314 ) ) ;
#54870=ADVANCED_FACE ( 'NONE', ( #79563 ), #60078, .T. ) ;
#54874=ORIENTED_EDGE ( 'NONE', *, *, #46641, .F. ) ;
#54887=EDGE_CURVE ( 'NONE', #52573, #86532, #94869, .T. ) ;
#54895=DIRECTION ( 'NONE',  ( -0.8141155183563226760, 0.000000000000000000, 0.5807029557109348872 ) ) ;
#54903=VERTEX_POINT ( 'NONE', #10397 ) ;
#54904=DIRECTION ( 'NONE',  ( 0.8141155183563185682, 0.000000000000000000, -0.5807029557109406603 ) ) ;
#54907=EDGE_CURVE ( 'NONE', #57773, #98073, #70319, .T. ) ;
#54920=VERTEX_POINT ( 'NONE', #70909 ) ;
#54922=DIRECTION ( 'NONE',  ( 0.000000000000000000, 1.000000000000000000, 0.000000000000000000 ) ) ;
#54923=CARTESIAN_POINT ( 'NONE',  ( 11.75249112337023760, 14.95037104118845583, -8.918310463591724968 ) ) ;
#54926=CARTESIAN_POINT ( 'NONE',  ( -10.36894250292378317, -2.571251165086037460, 10.36894250292379560 ) ) ;
#54929=ORIENTED_EDGE ( 'NONE', *, *, #31726, .T. ) ;
#54931=CARTESIAN_POINT ( 'NONE',  ( -14.43100913236851568, 15.00000000000000000, 1.412789942453067216 ) ) ;
#54932=CARTESIAN_POINT ( 'NONE',  ( 1.847237859018745487, 0.04962896072147187504, -14.63711110085117717 ) ) ;
#54933=PLANE ( 'NONE',  #28090 ) ;
#54940=EDGE_CURVE ( 'NONE', #1302, #42327, #55304, .T. ) ;
#54941=LINE ( 'NONE', #85456, #27920 ) ;
#54943=DIRECTION ( 'NONE',  ( 0.000000000000000000, 1.000000000000000000, 0.000000000000000000 ) ) ;
#54951=EDGE_CURVE ( 'NONE', #81651, #38851, #82435, .T. ) ;
#54954=DIRECTION ( 'NONE',  ( 0.02617694830788287394, 0.000000000000000000, -0.9996573249755570378 ) ) ;
#54961=EDGE_LOOP ( 'NONE', ( #21622, #5328, #5585, #60665 ) ) ;
#54990=CARTESIAN_POINT ( 'NONE',  ( 0.000000000000000000, 0.000000000000000000, 0.000000000000000000 ) ) ;
#54994=CARTESIAN_POINT ( 'NONE',  ( 7.208316651077764980, 22.88393115100078745, 7.208316651077762316 ) ) ;
#55005=EDGE_CURVE ( 'NONE', #16073, #40514, #32391, .T. ) ;
#55015=CARTESIAN_POINT ( 'NONE',  ( -14.04391541078767958, 4.832815575535569023E-16, 3.608107528142744602 ) ) ;
#55019=AXIS2_PLACEMENT_3D ( 'NONE', #76647, #40137, #24155 ) ;
#55020=( NAMED_UNIT ( * ) SI_UNIT ( $, .STERADIAN. ) SOLID_ANGLE_UNIT ( ) );
#55023=ORIENTED_EDGE ( 'NONE', *, *, #34646, .F. ) ;
#55025=ORIENTED_EDGE ( 'NONE', *, *, #389, .T. ) ;
#55027=CARTESIAN_POINT ( 'NONE',  ( -12.25993886608612371, 14.63595249122789177, 8.642563219313544209 ) ) ;
#55038=AXIS2_PLACEMENT_3D ( 'NONE', #19804, #26814, #58788 ) ;
#55042=LINE ( 'NONE', #77547, #68157 ) ;
#55044=CARTESIAN_POINT ( 'NONE',  ( -5.991992585808714189, 4.061121054423934144E-16, 13.20401548210291054 ) ) ;
#55047=ORIENTED_EDGE ( 'NONE', *, *, #24417, .F. ) ;
#55048=ORIENTED_EDGE ( 'NONE', *, *, #83069, .T. ) ;
#55049=ORIENTED_EDGE ( 'NONE', *, *, #42814, .T. ) ;
#55061=CARTESIAN_POINT ( 'NONE',  ( -10.88017736071110164, 2.855352010821508024, -2.915334737309917212 ) ) ;
#55067=CARTESIAN_POINT ( 'NONE',  ( -13.61464873478161941, 0.3639308181217350557, -6.296136897218030271 ) ) ;
#55071=LINE ( 'NONE', #71578, #15367 ) ;
#55079=VERTEX_POINT ( 'NONE', #61702 ) ;
#55088=CARTESIAN_POINT ( 'NONE',  ( 0.8653096853333108740, 15.00000000000000533, 14.59999144042652475 ) ) ;
#55093=ORIENTED_EDGE ( 'NONE', *, *, #11560, .T. ) ;
#55096=ADVANCED_FACE ( 'NONE', ( #30219 ), #52731, .F. ) ;
#55107=CARTESIAN_POINT ( 'NONE',  ( -4.923371831947292776, -13.15773551566587507, 8.527530157486181039 ) ) ;
#55109=TOROIDAL_SURFACE ( 'NONE', #98262, 14.49999999999999822, 0.5000000000000000000 ) ;
#55112=ORIENTED_EDGE ( 'NONE', *, *, #14696, .F. ) ;
#55118=CARTESIAN_POINT ( 'NONE',  ( -13.07751017357372447, 15.00000000000000000, -6.263284095430686094 ) ) ;
#55119=DIRECTION ( 'NONE',  ( -0.000000000000000000, -1.000000000000000000, -0.000000000000000000 ) ) ;
#55121=AXIS2_PLACEMENT_3D ( 'NONE', #7835, #53816, #69812 ) ;
#55123=ORIENTED_EDGE ( 'NONE', *, *, #41553, .F. ) ;
#55125=ORIENTED_EDGE ( 'NONE', *, *, #71373, .F. ) ;
#55129=LINE ( 'NONE', #47136, #77719 ) ;
#55130=EDGE_CURVE ( 'NONE', #28596, #24676, #45683, .T. ) ;
#55141=ORIENTED_EDGE ( 'NONE', *, *, #49332, .T. ) ;
#55144=CARTESIAN_POINT ( 'NONE',  ( 7.551349515323100725, 15.00000000000000000, 12.08468537022911349 ) ) ;
#55147=CARTESIAN_POINT ( 'NONE',  ( 1.514341385896460501, 15.00000000000000000, 15.92432625271834112 ) ) ;
#55149=LINE ( 'NONE', #83700, #36444 ) ;
#55161=CARTESIAN_POINT ( 'NONE',  ( -5.963430220938278126, 8.495456701841138880, 10.32896413005680358 ) ) ;
#55163=ORIENTED_EDGE ( 'NONE', *, *, #23510, .T. ) ;
#55170=CARTESIAN_POINT ( 'NONE',  ( -11.35178980618966804, 14.49999999999999112, -9.804941009312102551 ) ) ;
#55171=CARTESIAN_POINT ( 'NONE',  ( -14.97687855664610979, 14.63606903414041227, -0.8325315005902708121 ) ) ;
#55176=CARTESIAN_POINT ( 'NONE',  ( 12.26659068614894466, 29.72041550158063927, -7.082119434687053960 ) ) ;
#55188=AXIS2_PLACEMENT_3D ( 'NONE', #82466, #89964, #67967 ) ;
#55194=CARTESIAN_POINT ( 'NONE',  ( -11.22915323889568562, 15.00000000000000000, -8.773176023390764300 ) ) ;
#55195=CARTESIAN_POINT ( 'NONE',  ( -2.962741594153171842, 15.00000000000000000, 13.93860331045670975 ) ) ;
#55204=CARTESIAN_POINT ( 'NONE',  ( 14.22792531055121579, 15.00000000000000711, -3.387425595041105630 ) ) ;
#55210=CARTESIAN_POINT ( 'NONE',  ( -7.684764310694712997, 14.63606916355955434, -12.88194075009949557 ) ) ;
#55215=ORIENTED_EDGE ( 'NONE', *, *, #64209, .T. ) ;
#55216=DIRECTION ( 'NONE',  ( 0.000000000000000000, 1.000000000000000000, 0.000000000000000000 ) ) ;
#55217=AXIS2_PLACEMENT_3D ( 'NONE', #27133, #35124, #80645 ) ;
#55218=LINE ( 'NONE', #48210, #33 ) ;
#55227=CARTESIAN_POINT ( 'NONE',  ( 14.29541133317241730, 14.76930270348881180, 4.345028136609633052 ) ) ;
#55233=EDGE_CURVE ( 'NONE', #74265, #37243, #35157, .T. ) ;
#55237=DIRECTION ( 'NONE',  ( 0.000000000000000000, 0.000000000000000000, 1.000000000000000000 ) ) ;
#55241=CIRCLE ( 'NONE', #32890, 15.00000000000000000 ) ;
#55246=ORIENTED_EDGE ( 'NONE', *, *, #76004, .T. ) ;
#55248=CARTESIAN_POINT ( 'NONE',  ( -2.962741594153171842, 0.000000000000000000, 13.93860331045670975 ) ) ;
#55249=CARTESIAN_POINT ( 'NONE',  ( 11.09922568453595026, 1.206968003263759970, 6.408140936763232709 ) ) ;
#55250=VERTEX_POINT ( 'NONE', #11688 ) ;
#55253=ORIENTED_EDGE ( 'NONE', *, *, #43319, .F. ) ;
#55258=CARTESIAN_POINT ( 'NONE',  ( 13.14228782657339956, 15.00000000000000000, -7.230509711182238064 ) ) ;
#55263=AXIS2_PLACEMENT_3D ( 'NONE', #35922, #34432, #80450 ) ;
#55264=AXIS2_PLACEMENT_3D ( 'NONE', #3856, #47857, #95333 ) ;
#55265=VERTEX_POINT ( 'NONE', #66659 ) ;
#55272=CYLINDRICAL_SURFACE ( 'NONE', #5196, 15.00000000000000000 ) ;
#55288=( NAMED_UNIT ( * ) PLANE_ANGLE_UNIT ( ) SI_UNIT ( $, .RADIAN. ) );
#55291=ORIENTED_EDGE ( 'NONE', *, *, #3089, .T. ) ;
#55296=DIRECTION ( 'NONE',  ( 0.000000000000000000, 1.000000000000000000, 0.000000000000000000 ) ) ;
#55299=CARTESIAN_POINT ( 'NONE',  ( -4.431036607602660382, 0.5000000000000004441, 14.33059365769907956 ) ) ;
#55301=B_SPLINE_CURVE_WITH_KNOTS ( 'NONE', 3,
 ( #62925, #93426, #55930, #47915, #78916, #79417 ),
 .UNSPECIFIED., .F., .F.,
 ( 4, 2, 4 ),
 ( 3.409110551494653465E-05, 0.0004400426677367929684, 0.0008459942299586394564 ),
 .UNSPECIFIED. ) ;
#55303=CARTESIAN_POINT ( 'NONE',  ( -5.817157072110618721, 0.5000000000000004441, -13.82608706751094552 ) ) ;
#55304=CIRCLE ( 'NONE', #71246, 14.49999999999999822 ) ;
#55309=B_SPLINE_CURVE_WITH_KNOTS ( 'NONE', 3,
 ( #26631, #33628, #11634, #65608, #56648, #19630 ),
 .UNSPECIFIED., .F., .F.,
 ( 4, 2, 4 ),
 ( 3.409110551494649399E-05, 0.0004400426677367923721, 0.0008459942299586382638 ),
 .UNSPECIFIED. ) ;
#55312=DIRECTION ( 'NONE',  ( 0.07845909572785238206, 0.000000000000000000, -0.9969173337331274087 ) ) ;
#55313=ORIENTED_EDGE ( 'NONE', *, *, #71254, .F. ) ;
#55317=DIRECTION ( 'NONE',  ( 0.000000000000000000, 1.000000000000000000, 0.000000000000000000 ) ) ;
#55319=B_SPLINE_CURVE_WITH_KNOTS ( 'NONE', 3,
 ( #79111, #77625, #93621, #48608, #94603, #49105 ),
 .UNSPECIFIED., .F., .F.,
 ( 4, 2, 4 ),
 ( 0.0002800289709862447871, 0.0006862344838250761161, 0.001092439996663907391 ),
 .UNSPECIFIED. ) ;
#55326=CARTESIAN_POINT ( 'NONE',  ( -2.815433093577211832, 14.49999999999999112, 14.73340885523754551 ) ) ;
#55337=CARTESIAN_POINT ( 'NONE',  ( 5.056330833731659702, 4.503963689120695453E-16, 13.58983143750703348 ) ) ;
#55341=EDGE_CURVE ( 'NONE', #45656, #28421, #90479, .T. ) ;
#55365=VERTEX_POINT ( 'NONE', #57667 ) ;
#55368=CARTESIAN_POINT ( 'NONE',  ( 6.869455772997054233, 15.00000000000000000, 14.44603661281844431 ) ) ;
#55369=ORIENTED_EDGE ( 'NONE', *, *, #74509, .F. ) ;
#55373=VECTOR ( 'NONE', #88609, 1000.000000000000114 ) ;
#55375=CARTESIAN_POINT ( 'NONE',  ( -1.114591949024829054, 4.106534489568945963E-16, -14.45709807627966015 ) ) ;
#55391=EDGE_CURVE ( 'NONE', #31701, #84883, #12197, .T. ) ;
#55392=AXIS2_PLACEMENT_3D ( 'NONE', #81090, #5605, #28085 ) ;
#55395=ORIENTED_EDGE ( 'NONE', *, *, #57228, .T. ) ;
#55398=ORIENTED_EDGE ( 'NONE', *, *, #90328, .T. ) ;
#55399=ORIENTED_EDGE ( 'NONE', *, *, #82293, .T. ) ;
#55400=DIRECTION ( 'NONE',  ( 0.000000000000000000, 0.000000000000000000, 1.000000000000000000 ) ) ;
#55407=CARTESIAN_POINT ( 'NONE',  ( 2.518025504887150934, 0.000000000000000000, -4.837081990145593480 ) ) ;
#55411=ORIENTED_EDGE ( 'NONE', *, *, #65959, .T. ) ;
#55415=AXIS2_PLACEMENT_3D ( 'NONE', #90694, #76680, #31665 ) ;
#55427=CARTESIAN_POINT ( 'NONE',  ( -3.115783986955657170, 4.161706264368254368E-16, 14.16128137375395468 ) ) ;
#55429=VECTOR ( 'NONE', #18919, 1000.000000000000114 ) ;
#55432=CARTESIAN_POINT ( 'NONE',  ( -14.71525861348291819, 14.49999999999999112, -2.908807992686814003 ) ) ;
#55433=CARTESIAN_POINT ( 'NONE',  ( 14.88232117145530786, 14.49999999999999822, -1.875237731503139438 ) ) ;
#55435=AXIS2_PLACEMENT_3D ( 'NONE', #45068, #30059, #75576 ) ;
#55437=CARTESIAN_POINT ( 'NONE',  ( 12.26659068614894821, -6.112917831752690212, 7.082119434687044190 ) ) ;
#55438=CIRCLE ( 'NONE', #76133, 14.49999999999999822 ) ;
#55444=EDGE_CURVE ( 'NONE', #72583, #88979, #12664, .T. ) ;
#55445=EDGE_CURVE ( 'NONE', #43424, #72059, #65656, .T. ) ;
#55472=VECTOR ( 'NONE', #89886, 1000.000000000000227 ) ;
#55480=DIRECTION ( 'NONE',  ( 0.000000000000000000, 1.000000000000000000, 0.000000000000000000 ) ) ;
#55489=ORIENTED_EDGE ( 'NONE', *, *, #86497, .F. ) ;
#55492=CARTESIAN_POINT ( 'NONE',  ( 14.40939250469966026, 4.578996266948430760E-16, -1.618458416365756714 ) ) ;
#55493=( BOUNDED_CURVE ( )  B_SPLINE_CURVE ( 2, ( #10713, #50678, #26207, #20174, #34673, #56221, #12178, #11196, #73163, #57182, #71708, #88171, #94702 ),
 .UNSPECIFIED., .F., .F. ) 
 B_SPLINE_CURVE_WITH_KNOTS ( ( 3, 2, 2, 2, 2, 2, 3 ),
 ( 0.6333333333333333037, 0.6388888888888888395, 0.6444444444444444864, 0.6500000000000000222, 0.6555555555555555580, 0.6611111111111110938, 0.6666666666666666297 ),
 .UNSPECIFIED. ) 
 CURVE ( )  GEOMETRIC_REPRESENTATION_ITEM ( )  RATIONAL_B_SPLINE_CURVE ( ( 1.000000000000000000, 0.9659258262890683122, 1.000000000000000000, 0.9659258262890683122, 1.000000000000000000, 0.9659258262890683122, 1.000000000000000000, 0.9659258262890683122, 1.000000000000000000, 0.9659258262890683122, 1.000000000000000000, 0.9659258262890683122, 1.000000000000000000 ) ) 
 REPRESENTATION_ITEM ( '' )  );
#55494=ORIENTED_EDGE ( 'NONE', *, *, #67989, .F. ) ;
#55500=CARTESIAN_POINT ( 'NONE',  ( -13.61464873478171889, 0.3640475087720990710, 6.296136897217741613 ) ) ;
#55509=CARTESIAN_POINT ( 'NONE',  ( 2.638427012816829897, 24.55059781766745530, -9.846743663894592657 ) ) ;
#55511=ORIENTED_EDGE ( 'NONE', *, *, #14233, .T. ) ;
#55512=CARTESIAN_POINT ( 'NONE',  ( -6.767445849361073407, 14.49999999999999112, -13.38662304974512729 ) ) ;
#55520=CIRCLE ( 'NONE', #12387, 15.00000000000000000 ) ;
#55525=ORIENTED_EDGE ( 'NONE', *, *, #16662, .T. ) ;
#55528=DIRECTION ( 'NONE',  ( 0.000000000000000000, 0.000000000000000000, 1.000000000000000000 ) ) ;
#55535=CARTESIAN_POINT ( 'NONE',  ( -5.419894505350392855, 0.5000000000000004441, -13.98659156302466045 ) ) ;
#55538=ORIENTED_EDGE ( 'NONE', *, *, #26548, .T. ) ;
#55547=CARTESIAN_POINT ( 'NONE',  ( 14.03351048042397231, 15.00000000000000000, -2.474486531753715024 ) ) ;
#55562=ORIENTED_EDGE ( 'NONE', *, *, #82839, .T. ) ;
#55564=EDGE_CURVE ( 'NONE', #74650, #67193, #9150, .T. ) ;
#55576=CARTESIAN_POINT ( 'NONE',  ( -5.440088680355547268, -1.102981322511818796, 9.422509992056143702 ) ) ;
#55578=CARTESIAN_POINT ( 'NONE',  ( 4.841283923550437684, 14.76930270348882068, -14.13506365971146117 ) ) ;
#55583=FACE_OUTER_BOUND ( 'NONE', #20706, .T. ) ;
#55584=AXIS2_PLACEMENT_3D ( 'NONE', #92258, #77244, #8751 ) ;
#55588=CARTESIAN_POINT ( 'NONE',  ( 5.963430220938287007, 11.35497603579418247, 10.32896413005679825 ) ) ;
#55589=EDGE_CURVE ( 'NONE', #44200, #95213, #55129, .T. ) ;
#55600=EDGE_CURVE ( 'NONE', #25279, #87966, #25005, .T. ) ;
#55606=LINE ( 'NONE', #95565, #13908 ) ;
#55608=CARTESIAN_POINT ( 'NONE',  ( 0.000000000000000000, 14.49999999999999822, 0.000000000000000000 ) ) ;
#55610=ORIENTED_EDGE ( 'NONE', *, *, #1199, .T. ) ;
#55623=CARTESIAN_POINT ( 'NONE',  ( -2.638427012816824124, -12.94940218233254470, 9.846743663894596210 ) ) ;
#55632=CARTESIAN_POINT ( 'NONE',  ( -6.869455772996959197, -0.03417435944610275333, -14.44603661281848517 ) ) ;
#55635=CARTESIAN_POINT ( 'NONE',  ( -3.434112377981047626, 30.16530133659709989, 12.81628187352647963 ) ) ;
#55636=ORIENTED_EDGE ( 'NONE', *, *, #22255, .T. ) ;
#55647=B_SPLINE_CURVE_WITH_KNOTS ( 'NONE', 3,
 ( #75911, #23911, #16403, #83417, #7436, #76889 ),
 .UNSPECIFIED., .F., .F.,
 ( 4, 2, 4 ),
 ( 0.0002800154274984825720, 0.0006862208078247651697, 0.001092426188151047767 ),
 .UNSPECIFIED. ) ;
#55648=EDGE_CURVE ( 'NONE', #86906, #25488, #95485, .T. ) ;
#55650=VECTOR ( 'NONE', #67927, 1000.000000000000114 ) ;
#55651=DIRECTION ( 'NONE',  ( 0.8703556959398941473, 0.000000000000000000, 0.4924235601034769316 ) ) ;
#55655=VERTEX_POINT ( 'NONE', #3509 ) ;
#55658=CARTESIAN_POINT ( 'NONE',  ( 0.000000000000000000, 14.49999999999999822, 0.000000000000000000 ) ) ;
#55661=LINE ( 'NONE', #18156, #89097 ) ;
#55681=CARTESIAN_POINT ( 'NONE',  ( 11.06939482307794620, 12.70153705180264758, -3.010239261523810939 ) ) ;
#55682=CARTESIAN_POINT ( 'NONE',  ( 10.70613742633258170, 4.237152514796235822E-16, -9.778988772285240216 ) ) ;
#55683=LINE ( 'NONE', #4538, #31579 ) ;
#55685=CARTESIAN_POINT ( 'NONE',  ( 0.000000000000000000, 14.49999999999999822, 0.000000000000000000 ) ) ;
#55690=CARTESIAN_POINT ( 'NONE',  ( 14.16423886937410259, 29.30374883491396076, -2.602085213965210642E-15 ) ) ;
#55694=EDGE_CURVE ( 'NONE', #1780, #54920, #57960, .T. ) ;
#55712=DIRECTION ( 'NONE',  ( 0.000000000000000000, 1.000000000000000000, 0.000000000000000000 ) ) ;
#55724=VECTOR ( 'NONE', #63111, 1000.000000000000227 ) ;
#55731=DIRECTION ( 'NONE',  ( 0.1132032137679171296, 0.000000000000000000, -0.9935718556765862353 ) ) ;
#55748=FACE_OUTER_BOUND ( 'NONE', #15896, .T. ) ;
#55749=ORIENTED_EDGE ( 'NONE', *, *, #18341, .F. ) ;
#55758=CARTESIAN_POINT ( 'NONE',  ( 6.408140936763243367, -9.209698663402903662, 11.09922568453594494 ) ) ;
#55763=ORIENTED_EDGE ( 'NONE', *, *, #38608, .F. ) ;
#55770=EDGE_CURVE ( 'NONE', #41488, #11366, #74504, .T. ) ;
#55772=DIRECTION ( 'NONE',  ( -0.000000000000000000, 1.000000000000000000, 0.000000000000000000 ) ) ;
#55778=B_SPLINE_CURVE_WITH_KNOTS ( 'NONE', 3,
 ( #14489, #8934, #92431, #39451, #6980, #62416 ),
 .UNSPECIFIED., .F., .F.,
 ( 4, 2, 4 ),
 ( 0.0002800015744458462423, 0.0006862068192651793203, 0.001092412064084512290 ),
 .UNSPECIFIED. ) ;
#55779=AXIS2_PLACEMENT_3D ( 'NONE', #58794, #34303, #12313 ) ;
#55786=CARTESIAN_POINT ( 'NONE',  ( 14.16722289976685012, 15.00000000000000000, -4.928467845925517565 ) ) ;
#55798=ORIENTED_EDGE ( 'NONE', *, *, #79610, .F. ) ;
#55799=( BOUNDED_CURVE ( )  B_SPLINE_CURVE ( 2, ( #4640, #35612, #37600, #82591, #44084, #29088, #30564, #52583, #117, #28603, #7098, #98110, #21613 ),
 .UNSPECIFIED., .F., .F. ) 
 B_SPLINE_CURVE_WITH_KNOTS ( ( 3, 2, 2, 2, 2, 2, 3 ),
 ( 0.5999999999999999778, 0.6055555555555555136, 0.6111111111111111605, 0.6166666666666666963, 0.6222222222222223431, 0.6277777777777778789, 0.6333333333333334147 ),
 .UNSPECIFIED. ) 
 CURVE ( )  GEOMETRIC_REPRESENTATION_ITEM ( )  RATIONAL_B_SPLINE_CURVE ( ( 1.000000000000000000, 0.9659258262890683122, 1.000000000000000000, 0.9659258262890683122, 1.000000000000000000, 0.9659258262890683122, 1.000000000000000000, 0.9659258262890683122, 1.000000000000000000, 0.9659258262890683122, 1.000000000000000000, 0.9659258262890676461, 1.000000000000000666 ) ) 
 REPRESENTATION_ITEM ( '' )  );
#55802=EDGE_CURVE ( 'NONE', #36587, #339, #31049, .T. ) ;
#55806=AXIS2_PLACEMENT_3D ( 'NONE', #27197, #4725, #44172 ) ;
#55811=CARTESIAN_POINT ( 'NONE',  ( -0.1034006766821533585, 15.00000000000000000, -14.49963131600461175 ) ) ;
#55813=CIRCLE ( 'NONE', #36697, 15.00000000000000000 ) ;
#55820=DIRECTION ( 'NONE',  ( 0.000000000000000000, 1.000000000000000000, -0.000000000000000000 ) ) ;
#55828=ORIENTED_EDGE ( 'NONE', *, *, #50125, .T. ) ;
#55829=CARTESIAN_POINT ( 'NONE',  ( 13.75801628063881488, 4.740223025775510804E-16, -4.578972376164461622 ) ) ;
#55835=EDGE_CURVE ( 'NONE', #23568, #41037, #37589, .T. ) ;
#55861=EDGE_LOOP ( 'NONE', ( #57396, #71838, #28196, #58092 ) ) ;
#55869=CARTESIAN_POINT ( 'NONE',  ( 14.82269085861172719, 14.63606914777062151, -2.299529454046953081 ) ) ;
#55876=VERTEX_POINT ( 'NONE', #92058 ) ;
#55884=DIRECTION ( 'NONE',  ( 0.000000000000000000, 1.000000000000000000, 0.000000000000000000 ) ) ;
#55888=AXIS2_PLACEMENT_3D ( 'NONE', #85511, #83661, #14688 ) ;
#55891=CARTESIAN_POINT ( 'NONE',  ( -1.354709868695410657, 0.5000000000000004441, -14.93870011653153362 ) ) ;
#55892=ADVANCED_FACE ( 'NONE', ( #61057 ), #23583, .T. ) ;
#55893=ORIENTED_EDGE ( 'NONE', *, *, #1810, .T. ) ;
#55902=DIRECTION ( 'NONE',  ( 0.000000000000000000, 1.000000000000000000, 0.000000000000000000 ) ) ;
#55919=EDGE_CURVE ( 'NONE', #80716, #34672, #56990, .T. ) ;
#55930=CARTESIAN_POINT ( 'NONE',  ( 10.91061041304828727, 14.76930270348881002, -10.20767530377049148 ) ) ;
#55934=CARTESIAN_POINT ( 'NONE',  ( -10.36894250292379205, 6.178748834913974086, -10.36894250292378672 ) ) ;
#55947=VECTOR ( 'NONE', #43394, 1000.000000000000227 ) ;
#55948=AXIS2_PLACEMENT_3D ( 'NONE', #95293, #26796, #57292 ) ;
#55952=CARTESIAN_POINT ( 'NONE',  ( 0.000000000000000000, 0.5000000000000004441, 0.000000000000000000 ) ) ;
#55960=ORIENTED_EDGE ( 'NONE', *, *, #97888, .T. ) ;
#55962=ADVANCED_FACE ( 'NONE', ( #46071 ), #15096, .F. ) ;
#55979=CIRCLE ( 'NONE', #79942, 15.00000000000000000 ) ;
#55986=ORIENTED_EDGE ( 'NONE', *, *, #48650, .T. ) ;
#55987=EDGE_LOOP ( 'NONE', ( #45236, #61515, #12486, #2424, #17768, #79682 ) ) ;
#55992=CARTESIAN_POINT ( 'NONE',  ( 13.59943737456455715, 0.04922511925147255579, 5.718514076972947002 ) ) ;
#55993=DIRECTION ( 'NONE',  ( 0.000000000000000000, 0.000000000000000000, 1.000000000000000000 ) ) ;
#56001=CARTESIAN_POINT ( 'NONE',  ( -9.382169495545422677, -36.50136533006957507, -9.382169495545417348 ) ) ;
#56002=VERTEX_POINT ( 'NONE', #98611 ) ;
#56006=ADVANCED_FACE ( 'NONE', ( #60571 ), #24566, .T. ) ;
#56013=AXIS2_PLACEMENT_3D ( 'NONE', #24602, #3085, #26068 ) ;
#56017=ORIENTED_EDGE ( 'NONE', *, *, #205, .T. ) ;
#56028=CARTESIAN_POINT ( 'NONE',  ( -5.419894505350420388, 0.3639313574487524350, -13.98659156302468887 ) ) ;
#56031=ORIENTED_EDGE ( 'NONE', *, *, #74382, .F. ) ;
#56035=ORIENTED_EDGE ( 'NONE', *, *, #39203, .T. ) ;
#56036=ORIENTED_EDGE ( 'NONE', *, *, #91354, .F. ) ;
#56050=AXIS2_PLACEMENT_3D ( 'NONE', #67114, #6611, #20633 ) ;
#56055=CARTESIAN_POINT ( 'NONE',  ( -7.082119434687044190, -27.36291783175269643, 12.26659068614894998 ) ) ;
#56059=ORIENTED_EDGE ( 'NONE', *, *, #28453, .T. ) ;
#56067=DIRECTION ( 'NONE',  ( 0.000000000000000000, 1.000000000000000000, 0.000000000000000000 ) ) ;
#56071=CARTESIAN_POINT ( 'NONE',  ( -2.915334737309934532, 2.022018677488174099, -10.88017736071109987 ) ) ;
#56072=CARTESIAN_POINT ( 'NONE',  ( 14.69266224296342571, 0.04962895675140013840, 1.335284760096239864 ) ) ;
#56076=DIRECTION ( 'NONE',  ( 0.000000000000000000, 0.000000000000000000, -1.000000000000000000 ) ) ;
#56080=LINE ( 'NONE', #11548, #56871 ) ;
#56081=CARTESIAN_POINT ( 'NONE',  ( 3.840373378095567336, 13.17686044187654559, -11.29165764256138260 ) ) ;
#56102=DIRECTION ( 'NONE',  ( -0.000000000000000000, -1.000000000000000000, -0.000000000000000000 ) ) ;
#56115=CARTESIAN_POINT ( 'NONE',  ( 9.846743663894590881, -16.28273551566588040, -2.638427012816833894 ) ) ;
#56117=ORIENTED_EDGE ( 'NONE', *, *, #10931, .F. ) ;
#56119=ORIENTED_EDGE ( 'NONE', *, *, #47320, .F. ) ;
#56131=EDGE_CURVE ( 'NONE', #33705, #61749, #86040, .T. ) ;
#56133=ADVANCED_FACE ( 'NONE', ( #3529 ), #79017, .T. ) ;
#56134=ORIENTED_EDGE ( 'NONE', *, *, #28563, .F. ) ;
#56138=EDGE_LOOP ( 'NONE', ( #97789, #83439, #96863, #52546, #82164, #85044 ) ) ;
#56144=CARTESIAN_POINT ( 'NONE',  ( 0.2850016562179803481, 0.2303298976893956851, -14.93805486374024838 ) ) ;
#56148=DIRECTION ( 'NONE',  ( 0.000000000000000000, 1.000000000000000000, 0.000000000000000000 ) ) ;
#56152=CARTESIAN_POINT ( 'NONE',  ( 0.000000000000000000, 0.5000000000000004441, 0.000000000000000000 ) ) ;
#56153=AXIS2_PLACEMENT_3D ( 'NONE', #16498, #93961, #17488 ) ;
#56154=EDGE_CURVE ( 'NONE', #17335, #27398, #56552, .T. ) ;
#56161=CARTESIAN_POINT ( 'NONE',  ( -13.14228782657351680, 14.49999999999999112, 7.230509711182154575 ) ) ;
#56162=ORIENTED_EDGE ( 'NONE', *, *, #92818, .F. ) ;
#56166=CARTESIAN_POINT ( 'NONE',  ( -14.16722289976688565, 0.5000000000000004441, 4.928467845925418089 ) ) ;
#56174=CARTESIAN_POINT ( 'NONE',  ( 0.000000000000000000, 0.5000000000000004441, 0.000000000000000000 ) ) ;
#56178=CARTESIAN_POINT ( 'NONE',  ( -8.502721643904161297, 0.04962896249296521595, 12.05657636697095825 ) ) ;
#56179=CARTESIAN_POINT ( 'NONE',  ( -14.73551000134585820, 14.95037106540114991, -0.7225335126799745655 ) ) ;
#56183=CARTESIAN_POINT ( 'NONE',  ( 3.795296366450314540, 28.26208216824730712, 14.16423886937410082 ) ) ;
#56201=CARTESIAN_POINT ( 'NONE',  ( 0.000000000000000000, 15.00000000000000000, 0.000000000000000000 ) ) ;
#56202=CARTESIAN_POINT ( 'NONE',  ( -13.59972906620759936, 14.95037118612066784, -5.718800721552383060 ) ) ;
#56206=ORIENTED_EDGE ( 'NONE', *, *, #66771, .F. ) ;
#56215=ORIENTED_EDGE ( 'NONE', *, *, #68560, .T. ) ;
#56216=VECTOR ( 'NONE', #22212, 1000.000000000000000 ) ;
#56221=CARTESIAN_POINT ( 'NONE',  ( 11.25000000000000178, 10.21346884451820181, 3.014428414850127691 ) ) ;
#56234=CIRCLE ( 'NONE', #13096, 15.00000000000000000 ) ;
#56235=FACE_OUTER_BOUND ( 'NONE', #36028, .T. ) ;
#56241=PLANE ( 'NONE',  #93748 ) ;
#56243=VERTEX_POINT ( 'NONE', #25545 ) ;
#56250=EDGE_CURVE ( 'NONE', #66530, #95512, #39561, .T. ) ;
#56252=CARTESIAN_POINT ( 'NONE',  ( -3.434112377981047626, 0.1653013365970882609, 12.81628187352647963 ) ) ;
#56254=ORIENTED_EDGE ( 'NONE', *, *, #20227, .F. ) ;
#56256=ORIENTED_EDGE ( 'NONE', *, *, #18349, .F. ) ;
#56267=CARTESIAN_POINT ( 'NONE',  ( 2.258648100792191471, 14.95077488074853456, 14.57890972981274125 ) ) ;
#56274=CARTESIAN_POINT ( 'NONE',  ( 8.564643372776615138, 15.00000000000000000, -12.31449893000740836 ) ) ;
#56292=AXIS2_PLACEMENT_3D ( 'NONE', #44082, #36611, #75086 ) ;
#56301=CARTESIAN_POINT ( 'NONE',  ( -15.81765804549835330, 15.00000000000000000, -2.383084218347030880 ) ) ;
#56311=CARTESIAN_POINT ( 'NONE',  ( -6.761389522993972001, 14.76930270348881180, 13.32372569557295527 ) ) ;
#56314=CARTESIAN_POINT ( 'NONE',  ( 14.17193700899790265, 0.000000000000000000, -1.489530601564018175 ) ) ;
#56319=VERTEX_POINT ( 'NONE', #32023 ) ;
#56321=DIRECTION ( 'NONE',  ( -0.9981347984218673641, 0.000000000000000000, 0.06104853953484969120 ) ) ;
#56328=DIRECTION ( 'NONE',  ( 0.6755902076156493630, 0.000000000000000000, 0.7372773368101340763 ) ) ;
#56332=CARTESIAN_POINT ( 'NONE',  ( -14.88232117145538069, 14.49999999999999112, 1.875237731503072158 ) ) ;
#56351=ORIENTED_EDGE ( 'NONE', *, *, #11446, .F. ) ;
#56355=CARTESIAN_POINT ( 'NONE',  ( 0.000000000000000000, 15.00000000000000000, 0.000000000000000000 ) ) ;
#56358=VERTEX_POINT ( 'NONE', #94022 ) ;
#56360=LINE ( 'NONE', #34313, #84911 ) ;
#56363=CARTESIAN_POINT ( 'NONE',  ( 14.29730467489533652, 15.00000000000000000, -2.416004766803220072 ) ) ;
#56375=CARTESIAN_POINT ( 'NONE',  ( 0.000000000000000000, 0.5000000000000004441, 0.000000000000000000 ) ) ;
#56376=AXIS2_PLACEMENT_3D ( 'NONE', #20551, #29504, #74524 ) ;
#56385=ORIENTED_EDGE ( 'NONE', *, *, #57768, .T. ) ;
#56396=CARTESIAN_POINT ( 'NONE',  ( -14.26139399674453578, 15.00000000000000000, -2.619664342929994838 ) ) ;
#56397=CARTESIAN_POINT ( 'NONE',  ( 0.000000000000000000, 14.49999999999999822, 0.000000000000000000 ) ) ;
#56398=CIRCLE ( 'NONE', #83525, 15.00000000000000000 ) ;
#56399=ADVANCED_FACE ( 'NONE', ( #49493 ), #4348, .T. ) ;
#56402=VERTEX_POINT ( 'NONE', #73971 ) ;
#56403=VECTOR ( 'NONE', #25898, 1000.000000000000114 ) ;
#56407=CARTESIAN_POINT ( 'NONE',  ( -1.796787675079083879, 14.76984984742152385, -14.83218748772994466 ) ) ;
#56421=VERTEX_POINT ( 'NONE', #57001 ) ;
#56423=CARTESIAN_POINT ( 'NONE',  ( -12.34597252984326765, 0.04962896562384137150, -8.076773567935994436 ) ) ;
#56427=CARTESIAN_POINT ( 'NONE',  ( -14.16423886937410082, 1.803748834913972088, 4.336808689942017736E-15 ) ) ;
#56430=ORIENTED_EDGE ( 'NONE', *, *, #87605, .T. ) ;
#56432=CARTESIAN_POINT ( 'NONE',  ( 2.815433093577024426, 0.5000000000000004441, 14.73340885523751709 ) ) ;
#56436=CARTESIAN_POINT ( 'NONE',  ( -11.92686044187655980, 9.896642702460841434, 3.195792623639539087 ) ) ;
#56443=CARTESIAN_POINT ( 'NONE',  ( -1.354709868695741282, 14.63606900606166228, 14.93870011653154251 ) ) ;
#56461=DIRECTION ( 'NONE',  ( 0.04361938736533305799, 0.000000000000000000, 0.9990482215818579093 ) ) ;
#56469=ORIENTED_EDGE ( 'NONE', *, *, #34646, .T. ) ;
#56484=CARTESIAN_POINT ( 'NONE',  ( 0.000000000000000000, 15.00000000000000000, 0.000000000000000000 ) ) ;
#56486=EDGE_CURVE ( 'NONE', #65885, #47390, #38960, .T. ) ;
#56488=CARTESIAN_POINT ( 'NONE',  ( -12.81628187352647252, -35.66803199673624647, 3.434112377981066722 ) ) ;
#56489=ORIENTED_EDGE ( 'NONE', *, *, #42248, .T. ) ;
#56500=ORIENTED_EDGE ( 'NONE', *, *, #23303, .T. ) ;
#56504=ORIENTED_EDGE ( 'NONE', *, *, #44715, .T. ) ;
#56520=ORIENTED_EDGE ( 'NONE', *, *, #66707, .T. ) ;
#56521=CARTESIAN_POINT ( 'NONE',  ( 9.159723438033203990, -0.03417435944610275333, -10.91613331444542645 ) ) ;
#56524=DIRECTION ( 'NONE',  ( -0.9832549075639550606, 0.000000000000000000, 0.1822355254921448342 ) ) ;
#56535=CARTESIAN_POINT ( 'NONE',  ( 11.62112565934149089, -4.031876828930466656E-16, -8.881879596174739433 ) ) ;
#56538=CARTESIAN_POINT ( 'NONE',  ( -10.36894250292379205, -33.82125116508603213, -10.36894250292378672 ) ) ;
#56552=B_SPLINE_CURVE_WITH_KNOTS ( 'NONE', 3,
 ( #3045, #55027, #49011, #72002, #26503, #78038 ),
 .UNSPECIFIED., .F., .F.,
 ( 4, 2, 4 ),
 ( 3.409110551494646011E-05, 0.0004400426677367931852, 0.0008459942299586398901 ),
 .UNSPECIFIED. ) ;
#56553=CARTESIAN_POINT ( 'NONE',  ( -9.422509992056136596, 8.480352010821514241, 5.440088680355559703 ) ) ;
#56563=CARTESIAN_POINT ( 'NONE',  ( -14.82269085861170232, 15.00000000000000000, 2.299529454046861154 ) ) ;
#56564=VECTOR ( 'NONE', #54904, 1000.000000000000000 ) ;
#56567=EDGE_CURVE ( 'NONE', #47699, #98676, #71368, .T. ) ;
#56573=CARTESIAN_POINT ( 'NONE',  ( 5.795997163830076460, 15.00000000000000000, 13.01802277140709663 ) ) ;
#56575=VERTEX_POINT ( 'NONE', #55432 ) ;
#56586=DIRECTION ( 'NONE',  ( -0.000000000000000000, -1.000000000000000000, -0.000000000000000000 ) ) ;
#56594=EDGE_CURVE ( 'NONE', #61056, #79877, #32632, .T. ) ;
#56595=CARTESIAN_POINT ( 'NONE',  ( 5.795997163830076460, 0.000000000000000000, 13.01802277140709663 ) ) ;
#56600=CARTESIAN_POINT ( 'NONE',  ( 4.096035146093531587, 4.098443466602401877E-16, -13.90943910019259278 ) ) ;
#56602=ADVANCED_FACE ( 'NONE', ( #85436 ), #28229, .T. ) ;
#56603=CARTESIAN_POINT ( 'NONE',  ( -9.846743663894596210, 5.800597817667454414, -2.638427012816824124 ) ) ;
#56605=PLANE ( 'NONE',  #53998 ) ;
#56607=ORIENTED_EDGE ( 'NONE', *, *, #50672, .F. ) ;
#56618=EDGE_LOOP ( 'NONE', ( #90667, #72424, #70840, #77038 ) ) ;
#56626=DIRECTION ( 'NONE',  ( 0.9999619230641714207, 0.000000000000000000, -0.008726535498360278933 ) ) ;
#56627=( GEOMETRIC_REPRESENTATION_CONTEXT ( 3 ) GLOBAL_UNCERTAINTY_ASSIGNED_CONTEXT ( ( #42504 ) ) GLOBAL_UNIT_ASSIGNED_CONTEXT ( ( #86783, #94266, #47288 ) ) REPRESENTATION_CONTEXT ( 'NONE', 'WORKASPACE' ) );
#56632=VECTOR ( 'NONE', #78431, 1000.000000000000000 ) ;
#56638=CARTESIAN_POINT ( 'NONE',  ( 2.962741594152983993, 0.000000000000000000, 13.93860331045674883 ) ) ;
#56641=FACE_OUTER_BOUND ( 'NONE', #78475, .T. ) ;
#56648=CARTESIAN_POINT ( 'NONE',  ( -10.27191093752546891, 15.00000000000000888, -10.41278984915639683 ) ) ;
#56650=FACE_OUTER_BOUND ( 'NONE', #91947, .T. ) ;
#56651=AXIS2_PLACEMENT_3D ( 'NONE', #75859, #7379, #84838 ) ;
#56652=ORIENTED_EDGE ( 'NONE', *, *, #21816, .T. ) ;
#56657=CARTESIAN_POINT ( 'NONE',  ( 7.545084738058070783, 12.99794841920399691, -9.011045663943741957 ) ) ;
#56658=CARTESIAN_POINT ( 'NONE',  ( 13.55157833323629646, 14.76930270348882068, 6.292279346205477353 ) ) ;
#56660=CARTESIAN_POINT ( 'NONE',  ( -12.26659068614894110, 27.22041550158063572, 7.082119434687058401 ) ) ;
#56678=CARTESIAN_POINT ( 'NONE',  ( -13.78891971893203028, 14.63606857305640574, -5.904717858191753876 ) ) ;
#56679=EDGE_CURVE ( 'NONE', #65284, #52058, #55301, .T. ) ;
#56691=DIRECTION ( 'NONE',  ( 0.7604059656000385914, 0.000000000000000000, -0.6494480483301746654 ) ) ;
#56694=ADVANCED_FACE ( 'NONE', ( #9937 ), #13976, .T. ) ;
#56698=ORIENTED_EDGE ( 'NONE', *, *, #83671, .F. ) ;
#56699=CARTESIAN_POINT ( 'NONE',  ( 6.189940676892025984, 0.04962882325992712396, 13.39186120659007351 ) ) ;
#56714=EDGE_CURVE ( 'NONE', #44083, #59040, #14783, .T. ) ;
#56716=FACE_OUTER_BOUND ( 'NONE', #23796, .T. ) ;
#56718=ORIENTED_EDGE ( 'NONE', *, *, #96197, .F. ) ;
#56720=ORIENTED_EDGE ( 'NONE', *, *, #77588, .T. ) ;
#56724=CARTESIAN_POINT ( 'NONE',  ( -9.876730923139145801, 0.5000000000000004441, -11.28938378619076843 ) ) ;
#56729=CARTESIAN_POINT ( 'NONE',  ( -3.434112377981067610, -1.918031996736249356, -12.81628187352647252 ) ) ;
#56733=ORIENTED_EDGE ( 'NONE', *, *, #70277, .F. ) ;
#56747=DIRECTION ( 'NONE',  ( 0.000000000000000000, 0.000000000000000000, -1.000000000000000000 ) ) ;
#56757=CARTESIAN_POINT ( 'NONE',  ( 4.856092091438229730, 15.00000000000000178, 13.79590085420556811 ) ) ;
#56767=ORIENTED_EDGE ( 'NONE', *, *, #40571, .T. ) ;
#56775=DIRECTION ( 'NONE',  ( 0.000000000000000000, 1.000000000000000000, -0.000000000000000000 ) ) ;
#56782=EDGE_CURVE ( 'NONE', #1372, #67800, #12385, .T. ) ;
#56787=CARTESIAN_POINT ( 'NONE',  ( -6.767445849361341637, 14.49999999999999112, 13.38662304974498873 ) ) ;
#56803=CYLINDRICAL_SURFACE ( 'NONE', #36747, 15.00000000000000000 ) ;
#56814=AXIS2_PLACEMENT_3D ( 'NONE', #83274, #36793, #21295 ) ;
#56823=DIRECTION ( 'NONE',  ( 0.5519369853120559277, 0.000000000000000000, 0.8338858220671695465 ) ) ;
#56826=EDGE_CURVE ( 'NONE', #50486, #5813, #21973, .T. ) ;
#56835=VECTOR ( 'NONE', #70923, 1000.000000000000114 ) ;
#56837=VECTOR ( 'NONE', #57326, 1000.000000000000000 ) ;
#56840=CARTESIAN_POINT ( 'NONE',  ( 14.35840480524204210, 14.49999999999999112, 4.340070442838943165 ) ) ;
#56851=DIRECTION ( 'NONE',  ( 0.000000000000000000, 1.000000000000000000, 0.000000000000000000 ) ) ;
#56855=CARTESIAN_POINT ( 'NONE',  ( -9.288883250831421634, 2.385537343846901415, -6.626163283838958584 ) ) ;
#56860=DIRECTION ( 'NONE',  ( -0.000000000000000000, -1.000000000000000000, -0.000000000000000000 ) ) ;
#56870=CARTESIAN_POINT ( 'NONE',  ( 14.09356342482598379, 0.04922511925147127210, -4.360913911515380548 ) ) ;
#56871=VECTOR ( 'NONE', #12040, 1000.000000000000114 ) ;
#56872=CARTESIAN_POINT ( 'NONE',  ( 5.279540384298785582, 0.000000000000000000, -1.365381980696706687 ) ) ;
#56873=ADVANCED_FACE ( 'NONE', ( #39914 ), #39538, .T. ) ;
#56877=VERTEX_POINT ( 'NONE', #86883 ) ;
#56881=CARTESIAN_POINT ( 'NONE',  ( 5.625000000000006217, 6.784700295649323643, 9.742785792574933268 ) ) ;
#56892=DIRECTION ( 'NONE',  ( 0.000000000000000000, 1.000000000000000000, 0.000000000000000000 ) ) ;
#56905=CARTESIAN_POINT ( 'NONE',  ( -14.97687855664615064, 14.49999999999999112, 0.8325315005899805998 ) ) ;
#56907=CARTESIAN_POINT ( 'NONE',  ( -10.91036564011027465, 14.76984962000593704, -10.20716212663452360 ) ) ;
#56910=EDGE_CURVE ( 'NONE', #42104, #65885, #26373, .T. ) ;
#56911=CARTESIAN_POINT ( 'NONE',  ( -13.95806775979391823, 15.00000000000000888, -4.371577651620918381 ) ) ;
#56918=CARTESIAN_POINT ( 'NONE',  ( -1.175037534397337380, 15.00000000000000178, 14.57833316477036334 ) ) ;
#56922=CARTESIAN_POINT ( 'NONE',  ( 13.61464873478162652, 15.00000000000000000, 6.296136897217931683 ) ) ;
#56929=AXIS2_PLACEMENT_3D ( 'NONE', #20623, #5627, #68100 ) ;
#56937=CARTESIAN_POINT ( 'NONE',  ( 13.55255535720595184, 15.00000000000000000, -4.403492169842965431 ) ) ;
#56944=ORIENTED_EDGE ( 'NONE', *, *, #45088, .F. ) ;
#56947=EDGE_CURVE ( 'NONE', #77856, #56575, #79220, .T. ) ;
#56949=DIRECTION ( 'NONE',  ( 0.000000000000000000, -1.000000000000000000, 0.000000000000000000 ) ) ;
#56950=ORIENTED_EDGE ( 'NONE', *, *, #12002, .T. ) ;
#56965=CARTESIAN_POINT ( 'NONE',  ( 9.382169495545419124, -34.00136533006956796, 9.382169495545417348 ) ) ;
#56976=ORIENTED_EDGE ( 'NONE', *, *, #51816, .F. ) ;
#56981=ORIENTED_EDGE ( 'NONE', *, *, #18789, .T. ) ;
#56986=TOROIDAL_SURFACE ( 'NONE', #92119, 14.49999999999999822, 0.5000000000000000000 ) ;
#56988=EDGE_CURVE ( 'NONE', #3803, #48202, #38674, .T. ) ;
#56990=CIRCLE ( 'NONE', #82564, 14.49999999999999822 ) ;
#56996=CARTESIAN_POINT ( 'NONE',  ( 14.62617646268089011, 0.3639308321805998503, 3.327906561566976951 ) ) ;
#56997=TOROIDAL_SURFACE ( 'NONE', #76138, 14.49999999999999822, 0.5000000000000000000 ) ;
#56999=ORIENTED_EDGE ( 'NONE', *, *, #4609, .F. ) ;
#57000=ORIENTED_EDGE ( 'NONE', *, *, #13850, .T. ) ;
#57001=CARTESIAN_POINT ( 'NONE',  ( -9.159723438033054776, 0.000000000000000000, -10.91613331444555079 ) ) ;
#57016=DIRECTION ( 'NONE',  ( 0.000000000000000000, 0.000000000000000000, 1.000000000000000000 ) ) ;
#57018=CARTESIAN_POINT ( 'NONE',  ( 3.795296366450314540, -31.73791783175269288, 14.16423886937410082 ) ) ;
#57022=VERTEX_POINT ( 'NONE', #72356 ) ;
#57035=CARTESIAN_POINT ( 'NONE',  ( -10.88017736071110342, 18.06368534415484106, 3.903127820947815962E-15 ) ) ;
#57039=DIRECTION ( 'NONE',  ( -0.000000000000000000, -1.000000000000000000, -0.000000000000000000 ) ) ;
#57041=AXIS2_PLACEMENT_3D ( 'NONE', #16732, #62702, #47209 ) ;
#57049=DIRECTION ( 'NONE',  ( -0.000000000000000000, -1.000000000000000000, -0.000000000000000000 ) ) ;
#57052=EDGE_LOOP ( 'NONE', ( #3853, #61173, #55215, #25663, #93879, #39573 ) ) ;
#57058=AXIS2_PLACEMENT_3D ( 'NONE', #8783, #39302, #52803 ) ;
#57062=CARTESIAN_POINT ( 'NONE',  ( -4.838527690343426002, 14.49999999999999112, -14.19819177887740302 ) ) ;
#57064=B_SPLINE_CURVE_WITH_KNOTS ( 'NONE', 3,
 ( #1293, #78738, #16272, #84764, #86239, #93731 ),
 .UNSPECIFIED., .F., .F.,
 ( 4, 2, 4 ),
 ( 3.409110551494646011E-05, 0.0004400426677367923179, 0.0008459942299586381553 ),
 .UNSPECIFIED. ) ;
#57065=CIRCLE ( 'NONE', #79414, 15.00000000000000000 ) ;
#57066=EDGE_CURVE ( 'NONE', #94701, #88316, #62898, .T. ) ;
#57067=TOROIDAL_SURFACE ( 'NONE', #69867, 14.49999999999999822, 0.5000000000000000000 ) ;
#57068=CARTESIAN_POINT ( 'NONE',  ( -9.323033696085090583, 0.04962895454604727974, 11.43408728005506880 ) ) ;
#57077=DIRECTION ( 'NONE',  ( 0.000000000000000000, 0.000000000000000000, 1.000000000000000000 ) ) ;
#57084=CARTESIAN_POINT ( 'NONE',  ( 7.208316651077764980, -2.116068848999217877, 7.208316651077762316 ) ) ;
#57085=ORIENTED_EDGE ( 'NONE', *, *, #62588, .F. ) ;
#57094=LINE ( 'NONE', #64088, #61522 ) ;
#57103=VECTOR ( 'NONE', #38223, 1000.000000000000000 ) ;
#57106=EDGE_CURVE ( 'NONE', #44178, #41402, #82621, .T. ) ;
#57109=VERTEX_POINT ( 'NONE', #50349 ) ;
#57112=ADVANCED_FACE ( 'NONE', ( #91186 ), #53682, .T. ) ;
#57117=CARTESIAN_POINT ( 'NONE',  ( -1.780824192092292924, 0.5000000000000004441, -14.89391369643515795 ) ) ;
#57121=CARTESIAN_POINT ( 'NONE',  ( 0.3093388210927633941, 15.00000000000000000, 14.99680997725065978 ) ) ;
#57123=CARTESIAN_POINT ( 'NONE',  ( 14.47650479471825058, 14.49999999999999112, 3.928206833722148517 ) ) ;
#57134=FACE_OUTER_BOUND ( 'NONE', #4903, .T. ) ;
#57141=CARTESIAN_POINT ( 'NONE',  ( 11.12471383767606525, 12.50000000000035527, 1.674288514511126591 ) ) ;
#57142=EDGE_CURVE ( 'NONE', #54254, #55655, #96373, .T. ) ;
#57143=CARTESIAN_POINT ( 'NONE',  ( 13.21236992757673789, 15.00000000000000000, -5.338143956176714333 ) ) ;
#57146=CARTESIAN_POINT ( 'NONE',  ( -2.915334737309917656, -25.89464798917849109, 10.88017736071110164 ) ) ;
#57148=CARTESIAN_POINT ( 'NONE',  ( 14.93928340878672323, 0.2306972965111900864, -0.2363597353049662619 ) ) ;
#57150=CARTESIAN_POINT ( 'NONE',  ( 12.74305857943750730, 15.00000000000000178, -7.177950183686862218 ) ) ;
#57151=CARTESIAN_POINT ( 'NONE',  ( -7.684764310694707667, 15.00000000000000000, -12.88194075009945472 ) ) ;
#57161=CARTESIAN_POINT ( 'NONE',  ( -14.56195259121200714, 15.00000000000000888, -1.374002722866895176 ) ) ;
#57170=CARTESIAN_POINT ( 'NONE',  ( 12.34086200392821908, -0.03417435944610275333, 7.125000000000058620 ) ) ;
#57174=CARTESIAN_POINT ( 'NONE',  ( 5.803070148808231465, 3.918713670743053586E-16, 13.28812917035392260 ) ) ;
#57177=ORIENTED_EDGE ( 'NONE', *, *, #4488, .F. ) ;
#57179=CARTESIAN_POINT ( 'NONE',  ( 8.157990163924704774, 14.76930270348882068, 12.51739793958118874 ) ) ;
#57181=ORIENTED_EDGE ( 'NONE', *, *, #89345, .T. ) ;
#57182=CARTESIAN_POINT ( 'NONE',  ( 8.235571585149870089, 11.04680217785154106, -8.235571585149873641 ) ) ;
#57193=DIRECTION ( 'NONE',  ( 0.000000000000000000, 0.000000000000000000, 1.000000000000000000 ) ) ;
#57196=CARTESIAN_POINT ( 'NONE',  ( -7.208316651077756099, -33.36606884899921255, 7.208316651077766757 ) ) ;
#57197=ORIENTED_EDGE ( 'NONE', *, *, #94928, .T. ) ;
#57201=VERTEX_POINT ( 'NONE', #80860 ) ;
#57205=TOROIDAL_SURFACE ( 'NONE', #14112, 14.49999999999999822, 0.5000000000000000000 ) ;
#57207=VECTOR ( 'NONE', #72448, 1000.000000000000000 ) ;
#57211=CARTESIAN_POINT ( 'NONE',  ( -12.81628187352647252, 14.33196800326375175, 3.434112377981066722 ) ) ;
#57212=ORIENTED_EDGE ( 'NONE', *, *, #20916, .F. ) ;
#57214=VERTEX_POINT ( 'NONE', #53195 ) ;
#57223=( BOUNDED_CURVE ( )  B_SPLINE_CURVE ( 2, ( #77191, #741, #84706, #31194, #54192, #7234, #82725, #16210, #46694, #69701, #68240, #1231, #90220 ),
 .UNSPECIFIED., .F., .F. ) 
 B_SPLINE_CURVE_WITH_KNOTS ( ( 3, 2, 2, 2, 2, 2, 3 ),
 ( 0.5666666666666667629, 0.5722222222222222987, 0.5777777777777778345, 0.5833333333333334814, 0.5888888888888889062, 0.5944444444444444420, 0.5999999999999999778 ),
 .UNSPECIFIED. ) 
 CURVE ( )  GEOMETRIC_REPRESENTATION_ITEM ( )  RATIONAL_B_SPLINE_CURVE ( ( 0.9999999999999993339, 0.9659258262890688673, 1.000000000000000000, 0.9659258262890682012, 1.000000000000000000, 0.9659258262890682012, 1.000000000000000000, 0.9659258262890682012, 1.000000000000000000, 0.9659258262890682012, 1.000000000000000000, 0.9659258262890682012, 1.000000000000000000 ) ) 
 REPRESENTATION_ITEM ( '' )  );
#57224=CARTESIAN_POINT ( 'NONE',  ( -14.88232117145538069, 14.49999999999999112, 1.875237731503072158 ) ) ;
#57227=FACE_OUTER_BOUND ( 'NONE', #18610, .T. ) ;
#57228=EDGE_CURVE ( 'NONE', #25245, #75142, #95868, .T. ) ;
#57229=CARTESIAN_POINT ( 'NONE',  ( 7.551349515323100725, -0.03417435944610275333, 12.08468537022911349 ) ) ;
#57231=EDGE_CURVE ( 'NONE', #78202, #65662, #58334, .T. ) ;
#57233=DIRECTION ( 'NONE',  ( -0.000000000000000000, -1.000000000000000000, -0.000000000000000000 ) ) ;
#57243=EDGE_CURVE ( 'NONE', #50673, #81593, #9989, .T. ) ;
#57244=CARTESIAN_POINT ( 'NONE',  ( 14.02068044289385718, 14.49999999999999112, -5.331089937175661930 ) ) ;
#57250=CARTESIAN_POINT ( 'NONE',  ( -13.14228782657351680, 14.49999999999999112, 7.230509711182154575 ) ) ;
#57272=B_SPLINE_CURVE_WITH_KNOTS ( 'NONE', 3,
 ( #65039, #79581, #40603, #86101, #79077, #10590 ),
 .UNSPECIFIED., .F., .F.,
 ( 4, 2, 4 ),
 ( 3.409110551493610598E-05, 0.0004400426677367820722, 0.0008459942299586279638 ),
 .UNSPECIFIED. ) ;
#57280=CARTESIAN_POINT ( 'NONE',  ( -8.502626202121188470, 0.04922511925147058515, -12.05617882333549851 ) ) ;
#57287=CARTESIAN_POINT ( 'NONE',  ( -10.97221242068696512, -3.876446283109303924E-15, -9.670525607392942646 ) ) ;
#57292=DIRECTION ( 'NONE',  ( -0.2503800040544323924, 0.000000000000000000, -0.9681476403781101858 ) ) ;
#57297=LINE ( 'NONE', #20294, #502 ) ;
#57307=CARTESIAN_POINT ( 'NONE',  ( 0.000000000000000000, 14.49999999999999822, 0.000000000000000000 ) ) ;
#57319=EDGE_CURVE ( 'NONE', #70448, #89913, #45757, .T. ) ;
#57320=DIRECTION ( 'NONE',  ( -0.8870108331782246003, 0.000000000000000000, 0.4617486132350285266 ) ) ;
#57322=ORIENTED_EDGE ( 'NONE', *, *, #81181, .F. ) ;
#57326=DIRECTION ( 'NONE',  ( 0.000000000000000000, -1.000000000000000000, 0.000000000000000000 ) ) ;
#57342=DIRECTION ( 'NONE',  ( 3.552713678800500929E-15, 0.000000000000000000, 1.000000000000000000 ) ) ;
#57347=ADVANCED_FACE ( 'NONE', ( #61661 ), #46194, .F. ) ;
#57350=DIRECTION ( 'NONE',  ( 0.000000000000000000, 0.000000000000000000, 1.000000000000000000 ) ) ;
#57351=ORIENTED_EDGE ( 'NONE', *, *, #97512, .T. ) ;
#57362=CARTESIAN_POINT ( 'NONE',  ( 9.876730923139286134, 14.49999999999999112, 11.28938378619072935 ) ) ;
#57368=ORIENTED_EDGE ( 'NONE', *, *, #2016, .F. ) ;
#57369=CARTESIAN_POINT ( 'NONE',  ( 13.50249619331275674, 15.00000000000000888, -5.623250243473474796 ) ) ;
#57372=CARTESIAN_POINT ( 'NONE',  ( 6.689969769698956625, -0.03417435944610275333, -12.58200319823970226 ) ) ;
#57375=CARTESIAN_POINT ( 'NONE',  ( 0.000000000000000000, 0.5000000000000004441, 0.000000000000000000 ) ) ;
#57385=B_SPLINE_CURVE_WITH_KNOTS ( 'NONE', 3,
 ( #12973, #28955, #50975, #67467, #97987, #35477 ),
 .UNSPECIFIED., .F., .F.,
 ( 4, 2, 4 ),
 ( 0.0002800187770242821444, 0.0006862241901199757875, 0.001092429603215669268 ),
 .UNSPECIFIED. ) ;
#57387=CARTESIAN_POINT ( 'NONE',  ( -8.209432707284690878, 0.5000000000000004441, -12.55409154915497183 ) ) ;
#57390=CARTESIAN_POINT ( 'NONE',  ( 0.000000000000000000, 15.00000000000000000, 0.000000000000000000 ) ) ;
#57395=CARTESIAN_POINT ( 'NONE',  ( -0.1034006766821534140, 4.816303916663454299E-16, 14.49963131600461175 ) ) ;
#57396=ORIENTED_EDGE ( 'NONE', *, *, #18651, .F. ) ;
#57400=CARTESIAN_POINT ( 'NONE',  ( -6.382347221874250742, 14.63595249122788999, -13.57444820018236875 ) ) ;
#57406=ORIENTED_EDGE ( 'NONE', *, *, #59050, .F. ) ;
#57412=FACE_OUTER_BOUND ( 'NONE', #96914, .T. ) ;
#57413=DIRECTION ( 'NONE',  ( 0.000000000000000000, 1.000000000000000000, 0.000000000000000000 ) ) ;
#57424=B_SPLINE_CURVE_WITH_KNOTS ( 'NONE', 3,
 ( #94664, #26173, #95144, #87153, #3680, #64634 ),
 .UNSPECIFIED., .F., .F.,
 ( 4, 2, 4 ),
 ( 3.409110551496107651E-05, 0.0004400426677367867885, 0.0008459942299586125682 ),
 .UNSPECIFIED. ) ;
#57430=VERTEX_POINT ( 'NONE', #70668 ) ;
#57432=FACE_OUTER_BOUND ( 'NONE', #66604, .T. ) ;
#57440=ORIENTED_EDGE ( 'NONE', *, *, #5923, .T. ) ;
#57441=VECTOR ( 'NONE', #40886, 1000.000000000000114 ) ;
#57445=CYLINDRICAL_SURFACE ( 'NONE', #90371, 11.92686044187656513 ) ;
#57461=CARTESIAN_POINT ( 'NONE',  ( -3.434112377981067610, -31.91803199673623936, -12.81628187352647252 ) ) ;
#57469=DIRECTION ( 'NONE',  ( 0.000000000000000000, 0.000000000000000000, 1.000000000000000000 ) ) ;
#57478=ORIENTED_EDGE ( 'NONE', *, *, #7373, .F. ) ;
#57480=CARTESIAN_POINT ( 'NONE',  ( 11.92686044187656336, 7.188309369127517279, -2.602085213965210642E-15 ) ) ;
#57493=DIRECTION ( 'NONE',  ( 0.000000000000000000, 0.000000000000000000, 1.000000000000000000 ) ) ;
#57496=CARTESIAN_POINT ( 'NONE',  ( 2.189108318723648861, -3.258959264560919371E-15, 14.46085460646900245 ) ) ;
#57499=LINE ( 'NONE', #73978, #7108 ) ;
#57513=CARTESIAN_POINT ( 'NONE',  ( 14.16423886937410082, -35.48791783175269643, -3.795296366450314096 ) ) ;
#57516=VERTEX_POINT ( 'NONE', #32146 ) ;
#57528=CARTESIAN_POINT ( 'NONE',  ( 3.469446951953614189E-15, 19.31368534415484106, 10.88017736071110342 ) ) ;
#57530=CARTESIAN_POINT ( 'NONE',  ( -12.00809552683950088, 0.3639308727178954261, -8.989195838243722037 ) ) ;
#57532=DIRECTION ( 'NONE',  ( 1.953992523340275511E-14, 0.000000000000000000, 1.000000000000000000 ) ) ;
#57542=VERTEX_POINT ( 'NONE', #92180 ) ;
#57545=FACE_OUTER_BOUND ( 'NONE', #81647, .T. ) ;
#57554=ADVANCED_FACE ( 'NONE', ( #71156 ), #62648, .T. ) ;
#57555=DIRECTION ( 'NONE',  ( -4.174438572590588592E-14, 0.000000000000000000, 1.000000000000000000 ) ) ;
#57556=CARTESIAN_POINT ( 'NONE',  ( 13.75503023589411633, 0.04922511925147142475, -5.333408231410735389 ) ) ;
#57557=CIRCLE ( 'NONE', #78261, 14.49999999999999822 ) ;
#57562=B_SPLINE_CURVE_WITH_KNOTS ( 'NONE', 3,
 ( #12628, #73620, #95136, #12139, #18671, #5142 ),
 .UNSPECIFIED., .F., .F.,
 ( 4, 2, 4 ),
 ( 3.409110551496119849E-05, 0.0004400426677367863006, 0.0008459942299586114840 ),
 .UNSPECIFIED. ) ;
#57571=CARTESIAN_POINT ( 'NONE',  ( -4.923371831947292776, -3.157735515665872850, 8.527530157486181039 ) ) ;
#57572=ORIENTED_EDGE ( 'NONE', *, *, #62588, .T. ) ;
#57574=ORIENTED_EDGE ( 'NONE', *, *, #19398, .T. ) ;
#57576=AXIS2_PLACEMENT_3D ( 'NONE', #54140, #39159, #26122 ) ;
#57584=EDGE_CURVE ( 'NONE', #84722, #91634, #85172, .T. ) ;
#57589=ORIENTED_EDGE ( 'NONE', *, *, #25272, .T. ) ;
#57595=CARTESIAN_POINT ( 'NONE',  ( -3.115783986955657170, 4.161706264368254368E-16, 14.16128137375395468 ) ) ;
#57597=CIRCLE ( 'NONE', #84744, 15.00000000000000000 ) ;
#57607=EDGE_CURVE ( 'NONE', #26148, #50878, #24675, .T. ) ;
#57614=ORIENTED_EDGE ( 'NONE', *, *, #67640, .T. ) ;
#57615=CARTESIAN_POINT ( 'NONE',  ( -7.313705784284687539, 0.3640475087720989045, 13.09617149020739113 ) ) ;
#57624=CARTESIAN_POINT ( 'NONE',  ( 0.000000000000000000, 35.00000000000000000, 0.000000000000000000 ) ) ;
#57640=CARTESIAN_POINT ( 'NONE',  ( -10.88017736071110342, -21.93631465584515894, 3.903127820947815962E-15 ) ) ;
#57654=CARTESIAN_POINT ( 'NONE',  ( -14.43100913236846061, 15.00000000000000000, -1.412789942453363423 ) ) ;
#57667=CARTESIAN_POINT ( 'NONE',  ( 2.913501739333757889, 3.989000423594319145E-16, -14.20427779279535230 ) ) ;
#57669=VECTOR ( 'NONE', #75847, 1000.000000000000000 ) ;
#57670=EDGE_CURVE ( 'NONE', #2401, #22706, #94134, .T. ) ;
#57671=ORIENTED_EDGE ( 'NONE', *, *, #37323, .T. ) ;
#57686=EDGE_CURVE ( 'NONE', #57201, #97596, #86158, .T. ) ;
#57689=CARTESIAN_POINT ( 'NONE',  ( 6.382347221874423937, 0.5000000000000004441, -13.57444820018227638 ) ) ;
#57690=DIRECTION ( 'NONE',  ( 0.000000000000000000, 0.000000000000000000, 1.000000000000000000 ) ) ;
#57691=CARTESIAN_POINT ( 'NONE',  ( -4.923371831947302546, -34.82440218233254114, -8.527530157486173934 ) ) ;
#57692=EDGE_LOOP ( 'NONE', ( #95198, #80568, #57742, #96501 ) ) ;
#57693=ORIENTED_EDGE ( 'NONE', *, *, #13609, .T. ) ;
#57699=FACE_OUTER_BOUND ( 'NONE', #84625, .T. ) ;
#57703=CARTESIAN_POINT ( 'NONE',  ( 3.434112377981060948, 10.58196800326375353, 12.81628187352647430 ) ) ;
#57704=ORIENTED_EDGE ( 'NONE', *, *, #89986, .F. ) ;
#57707=VERTEX_POINT ( 'NONE', #95110 ) ;
#57715=CARTESIAN_POINT ( 'NONE',  ( -12.83294900548073336, 14.49999999999999112, 7.766300266068329350 ) ) ;
#57716=DIRECTION ( 'NONE',  ( 0.000000000000000000, 1.000000000000000000, 0.000000000000000000 ) ) ;
#57722=CARTESIAN_POINT ( 'NONE',  ( 3.420591144908545100, 0.5000000000000004441, -14.60477854057955938 ) ) ;
#57724=CARTESIAN_POINT ( 'NONE',  ( -14.99847009497944583, 0.5000000000000004441, 0.2142307401079343032 ) ) ;
#57729=CARTESIAN_POINT ( 'NONE',  ( -14.02068044289371684, 0.5000000000000004441, -5.331089937175857330 ) ) ;
#57740=CARTESIAN_POINT ( 'NONE',  ( -5.204170427930421283E-15, 6.671802177851543725, -11.25000000000000178 ) ) ;
#57742=ORIENTED_EDGE ( 'NONE', *, *, #85590, .T. ) ;
#57743=CARTESIAN_POINT ( 'NONE',  ( -11.25000000000000000, 5.326366962315977283, 3.014428414850140570 ) ) ;
#57757=DIRECTION ( 'NONE',  ( -0.000000000000000000, -1.000000000000000000, -0.000000000000000000 ) ) ;
#57768=EDGE_CURVE ( 'NONE', #25488, #30081, #64602, .T. ) ;
#57773=VERTEX_POINT ( 'NONE', #94631 ) ;
#57780=CARTESIAN_POINT ( 'NONE',  ( -0.7375392941515958034, 14.49999999999999112, -14.98185688723478215 ) ) ;
#57781=CARTESIAN_POINT ( 'NONE',  ( 12.00809552683952752, 0.5000000000000004441, 8.989195838243626113 ) ) ;
#57785=CARTESIAN_POINT ( 'NONE',  ( 0.9082943533636183009, 15.00000000000000000, 14.47152380945585648 ) ) ;
#57789=ADVANCED_FACE ( 'NONE', ( #80114 ), #57067, .T. ) ;
#57790=ORIENTED_EDGE ( 'NONE', *, *, #24810, .T. ) ;
#57799=EDGE_CURVE ( 'NONE', #41402, #4498, #72603, .T. ) ;
#57806=ORIENTED_EDGE ( 'NONE', *, *, #94151, .F. ) ;
#57816=TOROIDAL_SURFACE ( 'NONE', #62592, 14.49999999999999822, 0.5000000000000000000 ) ;
#57824=ORIENTED_EDGE ( 'NONE', *, *, #90094, .T. ) ;
#57829=LINE ( 'NONE', #51321, #86558 ) ;
#57834=AXIS2_PLACEMENT_3D ( 'NONE', #44695, #6213, #60189 ) ;
#57843=FACE_OUTER_BOUND ( 'NONE', #62978, .T. ) ;
#57860=FACE_OUTER_BOUND ( 'NONE', #11400, .T. ) ;
#57863=LINE ( 'NONE', #86896, #63179 ) ;
#57865=CARTESIAN_POINT ( 'NONE',  ( 12.58848565468357883, 15.00000000000000888, -7.447709424579856297 ) ) ;
#57870=LINE ( 'NONE', #96393, #35097 ) ;
#57877=LINE ( 'NONE', #58363, #58703 ) ;
#57887=CARTESIAN_POINT ( 'NONE',  ( -7.108715748588991801, 14.95077488074853456, -12.92719074505376575 ) ) ;
#57889=DIRECTION ( 'NONE',  ( -0.000000000000000000, -1.000000000000000000, -0.000000000000000000 ) ) ;
#57890=ORIENTED_EDGE ( 'NONE', *, *, #51700, .F. ) ;
#57895=CARTESIAN_POINT ( 'NONE',  ( 0.000000000000000000, 0.5000000000000004441, 0.000000000000000000 ) ) ;
#57896=CARTESIAN_POINT ( 'NONE',  ( 12.50534872682732690, 4.484280952698287085E-16, -7.339363270777523596 ) ) ;
#57917=CARTESIAN_POINT ( 'NONE',  ( -14.88232117145532385, 0.5000000000000004441, 1.875237731503040628 ) ) ;
#57924=ORIENTED_EDGE ( 'NONE', *, *, #84904, .F. ) ;
#57925=AXIS2_PLACEMENT_3D ( 'NONE', #33767, #26779, #10317 ) ;
#57928=CARTESIAN_POINT ( 'NONE',  ( -5.148594389986093312, 15.00000000000000711, -13.69051944078651317 ) ) ;
#57930=ORIENTED_EDGE ( 'NONE', *, *, #71994, .T. ) ;
#57934=CARTESIAN_POINT ( 'NONE',  ( 12.50534872682727716, 15.00000000000000000, 7.339363270777608861 ) ) ;
#57941=LINE ( 'NONE', #65938, #41320 ) ;
#57946=CARTESIAN_POINT ( 'NONE',  ( -3.434112377981047626, -29.83469866340290721, 12.81628187352647963 ) ) ;
#57954=CIRCLE ( 'NONE', #29266, 15.00000000000000000 ) ;
#57956=AXIS2_PLACEMENT_3D ( 'NONE', #83312, #31279, #46781 ) ;
#57960=LINE ( 'NONE', #87483, #58515 ) ;
#57963=ORIENTED_EDGE ( 'NONE', *, *, #73178, .F. ) ;
#57968=CARTESIAN_POINT ( 'NONE',  ( -4.181050312905175481, -2.964615315390050201E-16, 14.01631781289601442 ) ) ;
#57974=ORIENTED_EDGE ( 'NONE', *, *, #29023, .T. ) ;
#57978=ORIENTED_EDGE ( 'NONE', *, *, #57997, .T. ) ;
#57980=DIRECTION ( 'NONE',  ( 0.9981347984218670311, 0.000000000000000000, -0.06104853953485662316 ) ) ;
#57984=EDGE_CURVE ( 'NONE', #56421, #75686, #15240, .T. ) ;
#57993=ORIENTED_EDGE ( 'NONE', *, *, #78931, .T. ) ;
#57997=EDGE_CURVE ( 'NONE', #81607, #9509, #37249, .T. ) ;
#57999=CARTESIAN_POINT ( 'NONE',  ( -5.204170427930421283E-15, -29.44625116508602858, -14.16423886937410082 ) ) ;
#58007=CARTESIAN_POINT ( 'NONE',  ( 14.09394518620607428, 15.00000000000000000, 3.407449058785458451 ) ) ;
#58009=CARTESIAN_POINT ( 'NONE',  ( -6.761335002693183327, 0.2301500669213601691, 13.32315948060032973 ) ) ;
#58011=CARTESIAN_POINT ( 'NONE',  ( -2.915334737309917656, 9.105352010821512465, 10.88017736071110164 ) ) ;
#58015=AXIS2_PLACEMENT_3D ( 'NONE', #39716, #25213, #94665 ) ;
#58022=EDGE_CURVE ( 'NONE', #89795, #9875, #80267, .T. ) ;
#58031=ORIENTED_EDGE ( 'NONE', *, *, #11000, .T. ) ;
#58034=CARTESIAN_POINT ( 'NONE',  ( -13.21236992757665973, 0.000000000000000000, -5.338143956176898186 ) ) ;
#58041=CARTESIAN_POINT ( 'NONE',  ( -12.00809552683965187, 15.00000000000000000, 8.989195838243462688 ) ) ;
#58043=CARTESIAN_POINT ( 'NONE',  ( 12.34086200392826882, 15.00000000000000000, -7.124999999999971578 ) ) ;
#58046=EDGE_LOOP ( 'NONE', ( #26240, #56385, #62973, #69389, #12921, #94720 ) ) ;
#58057=B_SPLINE_CURVE_WITH_KNOTS ( 'NONE', 3,
 ( #64647, #65147, #95667, #27152, #57161, #57654 ),
 .UNSPECIFIED., .F., .F.,
 ( 4, 2, 4 ),
 ( 3.409110551333730758E-05, 0.0004400426677351795672, 0.0008459942299570218267 ),
 .UNSPECIFIED. ) ;
#58058=EDGE_CURVE ( 'NONE', #77859, #587, #2861, .T. ) ;
#58059=B_SPLINE_CURVE_WITH_KNOTS ( 'NONE', 3,
 ( #56787, #47807, #56311, #94786, #78308, #49773 ),
 .UNSPECIFIED., .F., .F.,
 ( 4, 2, 4 ),
 ( 3.409110551494646011E-05, 0.0004400426677367911795, 0.0008459942299586358785 ),
 .UNSPECIFIED. ) ;
#58060=CYLINDRICAL_SURFACE ( 'NONE', #3525, 15.00000000000000000 ) ;
#58061=CARTESIAN_POINT ( 'NONE',  ( -9.846743663894590881, 6.217264484334116936, 2.638427012816840111 ) ) ;
#58062=ORIENTED_EDGE ( 'NONE', *, *, #43226, .F. ) ;
#58063=EDGE_LOOP ( 'NONE', ( #39134, #70918, #58958, #40637 ) ) ;
#58073=ORIENTED_EDGE ( 'NONE', *, *, #84035, .T. ) ;
#58078=ORIENTED_EDGE ( 'NONE', *, *, #4848, .T. ) ;
#58086=ORIENTED_EDGE ( 'NONE', *, *, #61373, .F. ) ;
#58092=ORIENTED_EDGE ( 'NONE', *, *, #34526, .F. ) ;
#58097=CYLINDRICAL_SURFACE ( 'NONE', #60750, 15.00000000000000000 ) ;
#58102=EDGE_CURVE ( 'NONE', #40543, #26337, #58704, .T. ) ;
#58113=FACE_OUTER_BOUND ( 'NONE', #9186, .T. ) ;
#58116=CARTESIAN_POINT ( 'NONE',  ( 0.000000000000000000, 15.00000000000000000, 0.000000000000000000 ) ) ;
#58120=CARTESIAN_POINT ( 'NONE',  ( -9.422509992056136596, -26.51964798917849109, 5.440088680355559703 ) ) ;
#58124=DIRECTION ( 'NONE',  ( -0.000000000000000000, -1.000000000000000000, -0.000000000000000000 ) ) ;
#58126=CARTESIAN_POINT ( 'NONE',  ( 1.881645754503766366, 15.00000000000000533, 14.50406564081098182 ) ) ;
#58128=B_SPLINE_CURVE_WITH_KNOTS ( 'NONE', 3,
 ( #2645, #80578, #65553, #33099, #42579, #35055 ),
 .UNSPECIFIED., .F., .F.,
 ( 4, 2, 4 ),
 ( 0.0002800170536516742212, 0.0006862224498868413260, 0.001092427846122008593 ),
 .UNSPECIFIED. ) ;
#58133=CARTESIAN_POINT ( 'NONE',  ( -8.209432707284749497, 14.49999999999999112, -12.55409154915501269 ) ) ;
#58151=ORIENTED_EDGE ( 'NONE', *, *, #96432, .T. ) ;
#58152=CARTESIAN_POINT ( 'NONE',  ( 7.993154516100952733, 14.95077488074853811, 12.39982181464619160 ) ) ;
#58154=VERTEX_POINT ( 'NONE', #55170 ) ;
#58170=CARTESIAN_POINT ( 'NONE',  ( 12.34086200392821908, -0.03417435944610275333, 7.125000000000058620 ) ) ;
#58171=CARTESIAN_POINT ( 'NONE',  ( 9.846743663894590881, -31.69940218233254825, 2.638427012816828565 ) ) ;
#58173=CYLINDRICAL_SURFACE ( 'NONE', #44346, 15.00000000000000000 ) ;
#58175=ORIENTED_EDGE ( 'NONE', *, *, #70147, .T. ) ;
#58179=EDGE_CURVE ( 'NONE', #91322, #83574, #48141, .T. ) ;
#58180=DIRECTION ( 'NONE',  ( 3.907985046680551022E-14, 0.000000000000000000, 1.000000000000000000 ) ) ;
#58182=VECTOR ( 'NONE', #42987, 1000.000000000000227 ) ;
#58183=CARTESIAN_POINT ( 'NONE',  ( -12.81628187352647608, 9.123634669930428487, 3.903127820947815962E-15 ) ) ;
#58184=ORIENTED_EDGE ( 'NONE', *, *, #54750, .F. ) ;
#58188=ORIENTED_EDGE ( 'NONE', *, *, #17199, .T. ) ;
#58196=CARTESIAN_POINT ( 'NONE',  ( 0.9082943533637206635, 15.00000000000000000, -14.47152380945584760 ) ) ;
#58199=CARTESIAN_POINT ( 'NONE',  ( 1.780824192092498315, 14.63595249122789177, -14.89391369643514373 ) ) ;
#58202=EDGE_LOOP ( 'NONE', ( #12435, #94337, #35692, #29907, #66489, #79934 ) ) ;
#58204=CARTESIAN_POINT ( 'NONE',  ( -14.99847009497945294, 0.3640475087720990155, 0.2142307401079311391 ) ) ;
#58219=CARTESIAN_POINT ( 'NONE',  ( -13.07907619356937268, 14.76984992095085758, 7.222187741820579099 ) ) ;
#58221=CARTESIAN_POINT ( 'NONE',  ( 14.49440716394873618, 4.800686736885023475E-16, -0.4026921475166205244 ) ) ;
#58233=CARTESIAN_POINT ( 'NONE',  ( 7.082119434687054849, 3.470415501580635720, 12.26659068614894288 ) ) ;
#58242=VERTEX_POINT ( 'NONE', #96528 ) ;
#58254=EDGE_CURVE ( 'NONE', #19349, #3216, #58499, .T. ) ;
#58255=EDGE_LOOP ( 'NONE', ( #69729, #18622, #61899, #77251, #31218, #87524, #22966, #23136, #78499, #30741, #75128, #38189, #34172, #30676, #88927, #65780, #46534, #34015, #67511, #50432, #93404, #25500, #28162, #45590, #54033, #35457, #95351, #31658, #96720, #88484, #84747, #83142, #68856, #63125, #91236, #28564, #95998, #51319, #4584, #28391, #79378, #89698, #5749, #15794, #19753, #95403, #88577, #27688, #11788, #17709, #25411, #21201, #33087, #44534, #89956, #12849, #59149, #33714, #29650, #38093, #49586, #70530, #22210, #68837, #77328, #71536, #57963, #79514, #44486, #20561, #82875, #82490, #23800, #33588, #8386, #18915, #89311, #5402, #22355, #31383, #89163, #26603, #63823, #18953, #90655, #22793, #48359, #55369, #81680, #67661, #8571, #42034, #33288, #3218, #35205, #84645, #42232, #57806, #37934, #82070, #27770, #49330, #18843, #47438, #73313, #12499, #6580, #76653, #17447, #50513, #43188, #27598, #38902, #91579, #28805, #21103, #30493, #47263, #34691, #91522, #5092, #87987, #61916, #78754, #25394, #19635, #51236, #98691, #53042, #38649, #39628, #1294, #9906, #18800, #8046, #1744, #67072, #37574, #65062, #58464, #82601, #45538, #56718, #55538, #15941, #46707, #10144, #34174, #14823, #69418, #30220, #37765, #30616, #20251, #22639, #70610, #88698, #46755, #11689, #33220, #89865, #75990, #72825, #5484, #95571, #9263, #44840, #98283, #72484, #33700, #61411, #57890, #40641, #47147, #55047, #61765, #27430, #16789, #21039, #29919, #59332, #69411, #56500, #58615, #21791, #73200, #96054, #5375, #90134, #94638, #57085, #7088, #80941, #23791, #3639, #15769, #94944, #60617, #12722, #67099, #67215, #36158, #75096, #12928, #28061, #9492, #16189, #20824, #52558, #74164, #83804, #33911, #66086, #68598, #97825, #53029, #48832, #23638, #38110, #18014, #42311, #54036, #572, #36951, #89689, #90517, #18895, #70773, #23037, #83195, #91492, #907, #49940, #68658, #36327, #74284, #6919, #9236, #92388, #7802, #86815, #95939, #43575, #1400, #73909, #13603, #50096, #22994, #78036, #25632, #28188, #87815, #4739, #71051, #40027, #21946, #25994, #60290, #43594, #52862, #17858, #44142, #44976, #32258, #27307, #56254, #68176, #68345, #19498, #32357 ) ) ;
#58257=LINE ( 'NONE', #35272, #38077 ) ;
#58263=CARTESIAN_POINT ( 'NONE',  ( -0.8217048220028323469, 14.95037104780827342, -14.73031263976448457 ) ) ;
#58268=DIRECTION ( 'NONE',  ( 0.000000000000000000, 0.000000000000000000, 1.000000000000000000 ) ) ;
#58275=LINE ( 'NONE', #88793, #74772 ) ;
#58280=DIRECTION ( 'NONE',  ( 0.000000000000000000, 0.000000000000000000, 1.000000000000000000 ) ) ;
#58288=ORIENTED_EDGE ( 'NONE', *, *, #48173, .F. ) ;
#58290=ORIENTED_EDGE ( 'NONE', *, *, #73141, .F. ) ;
#58297=DIRECTION ( 'NONE',  ( 0.000000000000000000, 0.000000000000000000, 1.000000000000000000 ) ) ;
#58298=ORIENTED_EDGE ( 'NONE', *, *, #84241, .F. ) ;
#58306=ADVANCED_FACE ( 'NONE', ( #12023 ), #43013, .T. ) ;
#58310=CARTESIAN_POINT ( 'NONE',  ( 0.000000000000000000, 0.5000000000000004441, 0.000000000000000000 ) ) ;
#58313=FACE_OUTER_BOUND ( 'NONE', #7059, .T. ) ;
#58316=B_SPLINE_CURVE_WITH_KNOTS ( 'NONE', 3,
 ( #79711, #33696, #88682, #88186, #64195, #11210 ),
 .UNSPECIFIED., .F., .F.,
 ( 4, 2, 4 ),
 ( 3.409110551496207940E-05, 0.0004400426677367885232, 0.0008459942299586149534 ),
 .UNSPECIFIED. ) ;
#58330=DIRECTION ( 'NONE',  ( -0.000000000000000000, -1.000000000000000000, -0.000000000000000000 ) ) ;
#58334=LINE ( 'NONE', #11869, #85850 ) ;
#58336=EDGE_CURVE ( 'NONE', #79224, #18387, #10188, .T. ) ;
#58338=ORIENTED_EDGE ( 'NONE', *, *, #38681, .F. ) ;
#58344=EDGE_CURVE ( 'NONE', #58154, #42121, #55683, .T. ) ;
#58352=CARTESIAN_POINT ( 'NONE',  ( 4.862001128006775197, 15.00000000000000000, -13.66056166602457367 ) ) ;
#58358=ORIENTED_EDGE ( 'NONE', *, *, #23608, .T. ) ;
#58363=CARTESIAN_POINT ( 'NONE',  ( -1.983216688680738082, 15.00000000000000000, -14.11131997956740491 ) ) ;
#58366=AXIS2_PLACEMENT_3D ( 'NONE', #11811, #66282, #58280 ) ;
#58368=CARTESIAN_POINT ( 'NONE',  ( -14.36343418943208761, 14.95077488074853456, -3.367173657400845510 ) ) ;
#58370=CARTESIAN_POINT ( 'NONE',  ( -2.120353041430445895, 3.806229657360874111E-16, -14.34413130794948543 ) ) ;
#58373=CARTESIAN_POINT ( 'NONE',  ( -11.92686044187656691, 9.479976035794177136, -3.195792623639521324 ) ) ;
#58382=CARTESIAN_POINT ( 'NONE',  ( 9.876730923139298568, 15.00000000000000000, -11.28938378619063165 ) ) ;
#58384=CARTESIAN_POINT ( 'NONE',  ( 11.35178980618974087, 0.5000000000000004441, -9.804941009311923139 ) ) ;
#58385=CARTESIAN_POINT ( 'NONE',  ( -13.64884605730320644, -0.03417435944610275333, 8.341846182955681144 ) ) ;
#58389=CARTESIAN_POINT ( 'NONE',  ( -2.815433093577223378, 0.5000000000000004441, 14.73340885523747978 ) ) ;
#58395=AXIS2_PLACEMENT_3D ( 'NONE', #58803, #89310, #52298 ) ;
#58402=VERTEX_POINT ( 'NONE', #75482 ) ;
#58415=CARTESIAN_POINT ( 'NONE',  ( -12.11353679309427278, 14.95037110518055989, -8.421373815019801867 ) ) ;
#58417=ORIENTED_EDGE ( 'NONE', *, *, #94697, .F. ) ;
#58422=DIRECTION ( 'NONE',  ( -0.000000000000000000, -1.000000000000000000, -0.000000000000000000 ) ) ;
#58432=VERTEX_POINT ( 'NONE', #75974 ) ;
#58434=CARTESIAN_POINT ( 'NONE',  ( 9.382169495545419124, -19.00136533006957507, 9.382169495545417348 ) ) ;
#58445=DIRECTION ( 'NONE',  ( 0.000000000000000000, 0.000000000000000000, -1.000000000000000000 ) ) ;
#58455=EDGE_CURVE ( 'NONE', #79695, #78202, #14506, .T. ) ;
#58457=CARTESIAN_POINT ( 'NONE',  ( -4.096035146093626622, 4.358906096699807873E-16, 13.90943910019256258 ) ) ;
#58464=ORIENTED_EDGE ( 'NONE', *, *, #73127, .F. ) ;
#58466=EDGE_CURVE ( 'NONE', #16129, #85150, #23129, .T. ) ;
#58472=AXIS2_PLACEMENT_3D ( 'NONE', #10153, #55651, #63620 ) ;
#58481=CARTESIAN_POINT ( 'NONE',  ( 11.12471383767373467, 2.500000000000004885, 1.674288514525068328 ) ) ;
#58486=EDGE_CURVE ( 'NONE', #29308, #62057, #85059, .T. ) ;
#58493=CARTESIAN_POINT ( 'NONE',  ( -12.26659068614894110, -22.77958449841936073, 7.082119434687058401 ) ) ;
#58498=ORIENTED_EDGE ( 'NONE', *, *, #4609, .T. ) ;
#58499=LINE ( 'NONE', #50514, #65110 ) ;
#58509=CARTESIAN_POINT ( 'NONE',  ( 2.915334737309928315, 14.52201867748817499, 10.88017736071109987 ) ) ;
#58514=B_SPLINE_CURVE_WITH_KNOTS ( 'NONE', 3,
 ( #42146, #57615, #88113, #50117, #12121, #42623 ),
 .UNSPECIFIED., .F., .F.,
 ( 4, 2, 4 ),
 ( 3.409110551495909784E-05, 0.0004400426677367837527, 0.0008459942299586083398 ),
 .UNSPECIFIED. ) ;
#58515=VECTOR ( 'NONE', #10998, 999.9999999999998863 ) ;
#58516=CARTESIAN_POINT ( 'NONE',  ( 0.000000000000000000, 0.5000000000000004441, 0.000000000000000000 ) ) ;
#58529=CARTESIAN_POINT ( 'NONE',  ( 9.402796353261051010, 0.5000000000000004441, 11.68706210897763320 ) ) ;
#58532=LINE ( 'NONE', #22041, #59575 ) ;
#58539=VECTOR ( 'NONE', #47300, 1000.000000000000114 ) ;
#58541=CARTESIAN_POINT ( 'NONE',  ( -15.08495336817617982, 15.00000000000000000, 5.321802168063332950 ) ) ;
#58543=ORIENTED_EDGE ( 'NONE', *, *, #45261, .T. ) ;
#58548=FACE_OUTER_BOUND ( 'NONE', #80773, .T. ) ;
#58556=CARTESIAN_POINT ( 'NONE',  ( 8.527530157486175710, 3.925597817667457523, -4.923371831947298993 ) ) ;
#58557=ORIENTED_EDGE ( 'NONE', *, *, #46970, .F. ) ;
#58569=LINE ( 'NONE', #88080, #20752 ) ;
#58571=AXIS2_PLACEMENT_3D ( 'NONE', #6530, #44025, #20050 ) ;
#58585=LINE ( 'NONE', #43583, #1207 ) ;
#58586=CARTESIAN_POINT ( 'NONE',  ( 10.17177286909463341, 14.76984972048479783, 10.94336654633689321 ) ) ;
#58587=ORIENTED_EDGE ( 'NONE', *, *, #79124, .T. ) ;
#58590=ORIENTED_EDGE ( 'NONE', *, *, #93242, .F. ) ;
#58593=EDGE_CURVE ( 'NONE', #37579, #15233, #9093, .T. ) ;
#58597=ORIENTED_EDGE ( 'NONE', *, *, #33525, .F. ) ;
#58601=FACE_OUTER_BOUND ( 'NONE', #1057, .T. ) ;
#58604=DIRECTION ( 'NONE',  ( 0.000000000000000000, 0.000000000000000000, 1.000000000000000000 ) ) ;
#58606=CARTESIAN_POINT ( 'NONE',  ( -13.16740645155975464, 14.95077488074853811, 6.653232860246455438 ) ) ;
#58613=B_SPLINE_CURVE_WITH_KNOTS ( 'NONE', 3,
 ( #67623, #29593, #13622, #44103, #74613, #44611 ),
 .UNSPECIFIED., .F., .F.,
 ( 4, 2, 4 ),
 ( 0.0002800760588436753545, 0.0006862820326555788431, 0.001092488006467482332 ),
 .UNSPECIFIED. ) ;
#58615=ORIENTED_EDGE ( 'NONE', *, *, #42360, .F. ) ;
#58623=ADVANCED_FACE ( 'NONE', ( #77578 ), #79565, .T. ) ;
#58630=CARTESIAN_POINT ( 'NONE',  ( -7.964842623401179544, -27.56131465584515894, -7.964842623401174215 ) ) ;
#58634=CARTESIAN_POINT ( 'NONE',  ( 11.10136736363526744, 14.95077488074853811, 9.716261771424980154 ) ) ;
#58637=CARTESIAN_POINT ( 'NONE',  ( 1.796787675079194013, 14.76984984742152385, 14.83218748772992690 ) ) ;
#58638=AXIS2_PLACEMENT_3D ( 'NONE', #26326, #42323, #4336 ) ;
#58643=LINE ( 'NONE', #88151, #13636 ) ;
#58647=ORIENTED_EDGE ( 'NONE', *, *, #1082, .T. ) ;
#58657=ORIENTED_EDGE ( 'NONE', *, *, #51744, .T. ) ;
#58680=CARTESIAN_POINT ( 'NONE',  ( 9.846743663894590881, -31.28273551566587685, -2.638427012816833894 ) ) ;
#58682=VERTEX_POINT ( 'NONE', #18081 ) ;
#58688=CARTESIAN_POINT ( 'NONE',  ( -9.159723438033054776, -0.03417435944610275333, -10.91613331444555079 ) ) ;
#58691=CARTESIAN_POINT ( 'NONE',  ( 9.382169495545415572, 2.248634669930418273, -9.382169495545422677 ) ) ;
#58695=ORIENTED_EDGE ( 'NONE', *, *, #69650, .T. ) ;
#58703=VECTOR ( 'NONE', #88882, 1000.000000000000114 ) ;
#58704=CIRCLE ( 'NONE', #7701, 14.49999999999999822 ) ;
#58706=CARTESIAN_POINT ( 'NONE',  ( -12.83294900548069961, 14.63595249122789177, 7.766300266068285829 ) ) ;
#58709=CARTESIAN_POINT ( 'NONE',  ( 10.14667048435135577, 15.00000000000000000, 10.35833375027046976 ) ) ;
#58713=EDGE_CURVE ( 'NONE', #189, #77019, #78082, .T. ) ;
#58715=CARTESIAN_POINT ( 'NONE',  ( 8.606322355891288467, 3.856550154308941175E-16, 11.66967075398812703 ) ) ;
#58716=ORIENTED_EDGE ( 'NONE', *, *, #9371, .F. ) ;
#58717=CARTESIAN_POINT ( 'NONE',  ( -14.74963345907815793, 0.04922511925147218109, 0.3072669459659669866 ) ) ;
#58724=CARTESIAN_POINT ( 'NONE',  ( -13.21236992757665973, 15.00000000000000000, -5.338143956176898186 ) ) ;
#58732=ORIENTED_EDGE ( 'NONE', *, *, #37027, .F. ) ;
#58740=CARTESIAN_POINT ( 'NONE',  ( 0.000000000000000000, 0.5000000000000004441, 0.000000000000000000 ) ) ;
#58744=CARTESIAN_POINT ( 'NONE',  ( 12.26659068614894466, 4.720415501580636608, -7.082119434687053960 ) ) ;
#58753=EDGE_LOOP ( 'NONE', ( #22933, #79842, #22688, #86863, #69169, #96072, #20674, #91355, #59857, #7077, #16147, #45289 ) ) ;
#58758=CARTESIAN_POINT ( 'NONE',  ( 11.12471383767373467, 2.500000000000004885, 1.674288514525068328 ) ) ;
#58759=CARTESIAN_POINT ( 'NONE',  ( 2.888614318722341867, 6.013933925505530435E-16, 14.33855829812825888 ) ) ;
#58762=ORIENTED_EDGE ( 'NONE', *, *, #61114, .T. ) ;
#58764=DIRECTION ( 'NONE',  ( -0.7716245833877148907, 0.000000000000000000, -0.6360782202777701677 ) ) ;
#58771=CARTESIAN_POINT ( 'NONE',  ( 11.81378540890930751, -0.03417435944610275333, 7.968498874458199488 ) ) ;
#58788=DIRECTION ( 'NONE',  ( 0.000000000000000000, 0.000000000000000000, -1.000000000000000000 ) ) ;
#58791=LINE ( 'NONE', #95822, #33086 ) ;
#58794=CARTESIAN_POINT ( 'NONE',  ( 0.000000000000000000, 15.00000000000000000, 0.000000000000000000 ) ) ;
#58795=ORIENTED_EDGE ( 'NONE', *, *, #85590, .F. ) ;
#58802=EDGE_CURVE ( 'NONE', #55250, #36305, #66200, .T. ) ;
#58803=CARTESIAN_POINT ( 'NONE',  ( 0.000000000000000000, 0.5000000000000004441, 0.000000000000000000 ) ) ;
#58804=ORIENTED_EDGE ( 'NONE', *, *, #19990, .T. ) ;
#58808=EDGE_LOOP ( 'NONE', ( #50778, #70708, #45714, #80 ) ) ;
#58820=ORIENTED_EDGE ( 'NONE', *, *, #64585, .T. ) ;
#58824=LINE ( 'NONE', #67323, #77029 ) ;
#58828=ORIENTED_EDGE ( 'NONE', *, *, #58455, .F. ) ;
#58829=LINE ( 'NONE', #68324, #91055 ) ;
#58833=DIRECTION ( 'NONE',  ( -0.000000000000000000, -1.000000000000000000, -0.000000000000000000 ) ) ;
#58837=CARTESIAN_POINT ( 'NONE',  ( -10.27090289957542169, 15.00000000000000711, 10.41235154178098199 ) ) ;
#58845=CARTESIAN_POINT ( 'NONE',  ( 7.003840667633619788, 15.00000000000000888, 12.84073839985658161 ) ) ;
#58857=CARTESIAN_POINT ( 'NONE',  ( -10.91036564011048426, 0.2301503799940542716, 10.20716212663429801 ) ) ;
#58860=CIRCLE ( 'NONE', #8001, 14.49999999999999822 ) ;
#58863=VERTEX_POINT ( 'NONE', #14965 ) ;
#58870=CARTESIAN_POINT ( 'NONE',  ( 13.34343830728404079, 0.5000000000000004441, -6.852200678592596184 ) ) ;
#58874=ORIENTED_EDGE ( 'NONE', *, *, #33056, .F. ) ;
#58883=FACE_OUTER_BOUND ( 'NONE', #12511, .T. ) ;
#58885=CARTESIAN_POINT ( 'NONE',  ( -2.962741594152892510, 15.00000000000000000, -13.93860331045676837 ) ) ;
#58886=EDGE_CURVE ( 'NONE', #38526, #3732, #2843, .T. ) ;
#58893=VECTOR ( 'NONE', #79188, 1000.000000000000114 ) ;
#58894=CARTESIAN_POINT ( 'NONE',  ( 2.815433093577122126, 15.00000000000000000, -14.73340885523749932 ) ) ;
#58910=DIRECTION ( 'NONE',  ( 0.000000000000000000, 1.000000000000000000, 0.000000000000000000 ) ) ;
#58914=CIRCLE ( 'NONE', #39795, 14.49999999999999822 ) ;
#58922=CARTESIAN_POINT ( 'NONE',  ( -13.78891971893199830, 0.5000000000000004441, -5.904717858191724567 ) ) ;
#58924=ORIENTED_EDGE ( 'NONE', *, *, #76910, .F. ) ;
#58939=VERTEX_POINT ( 'NONE', #90929 ) ;
#58941=CARTESIAN_POINT ( 'NONE',  ( 12.81628187352647608, -13.37636533006957684, -2.602085213965210642E-15 ) ) ;
#58958=ORIENTED_EDGE ( 'NONE', *, *, #15600, .T. ) ;
#58961=CARTESIAN_POINT ( 'NONE',  ( 11.92686044187656336, 6.979976035794169142, 3.195792623639526653 ) ) ;
#58972=LINE ( 'NONE', #73968, #88530 ) ;
#58976=CARTESIAN_POINT ( 'NONE',  ( 11.59608414876342408, 0.2306972965111887541, 9.421724210956368140 ) ) ;
#58983=EDGE_LOOP ( 'NONE', ( #2839, #69135, #756, #64094 ) ) ;
#58991=EDGE_CURVE ( 'NONE', #73794, #25822, #36453, .T. ) ;
#58994=CARTESIAN_POINT ( 'NONE',  ( 14.16423886937410082, -20.48791783175269643, -3.795296366450314096 ) ) ;
#58998=VERTEX_POINT ( 'NONE', #29931 ) ;
#59009=CARTESIAN_POINT ( 'NONE',  ( -10.88017736071110164, 27.85535201082149470, -2.915334737309917212 ) ) ;
#59012=VERTEX_POINT ( 'NONE', #53929 ) ;
#59022=CARTESIAN_POINT ( 'NONE',  ( -13.82192141328803991, 15.00000000000000000, -4.382292601468865456 ) ) ;
#59024=ORIENTED_EDGE ( 'NONE', *, *, #13155, .T. ) ;
#59035=DIRECTION ( 'NONE',  ( -0.9996573249755572599, 0.000000000000000000, -0.02617694830787627158 ) ) ;
#59037=CARTESIAN_POINT ( 'NONE',  ( 12.11353679309438824, 0.04962889481942911463, -8.421373815019629561 ) ) ;
#59040=VERTEX_POINT ( 'NONE', #7947 ) ;
#59046=DIRECTION ( 'NONE',  ( -0.4617486132350285266, 0.000000000000000000, -0.8870108331782246003 ) ) ;
#59050=EDGE_CURVE ( 'NONE', #21240, #15967, #1355, .T. ) ;
#59055=CARTESIAN_POINT ( 'NONE',  ( 4.923371831947301658, 22.67559781766745175, 8.527530157486175710 ) ) ;
#59056=VERTEX_POINT ( 'NONE', #20799 ) ;
#59057=ORIENTED_EDGE ( 'NONE', *, *, #18789, .F. ) ;
#59058=DIRECTION ( 'NONE',  ( 0.000000000000000000, 1.000000000000000000, 0.000000000000000000 ) ) ;
#59079=VERTEX_POINT ( 'NONE', #65782 ) ;
#59083=CARTESIAN_POINT ( 'NONE',  ( 14.26295192185811445, 14.95077488074852035, -3.770186020345025479 ) ) ;
#59090=DIRECTION ( 'NONE',  ( 0.000000000000000000, 1.000000000000000000, 0.000000000000000000 ) ) ;
#59091=ORIENTED_EDGE ( 'NONE', *, *, #13652, .F. ) ;
#59101=ORIENTED_EDGE ( 'NONE', *, *, #89741, .T. ) ;
#59108=DIRECTION ( 'NONE',  ( 0.000000000000000000, 0.000000000000000000, 1.000000000000000000 ) ) ;
#59113=CARTESIAN_POINT ( 'NONE',  ( 3.469446951953614189E-15, -5.686314655845153609, 10.88017736071110342 ) ) ;
#59117=CARTESIAN_POINT ( 'NONE',  ( 14.94699059465107105, 14.49999999999999112, 1.259949270174897329 ) ) ;
#59132=CARTESIAN_POINT ( 'NONE',  ( 0.000000000000000000, 0.5000000000000004441, 0.000000000000000000 ) ) ;
#59133=VECTOR ( 'NONE', #8009, 1000.000000000000114 ) ;
#59140=CARTESIAN_POINT ( 'NONE',  ( 9.010802615329073006, 14.76984942314351734, -11.91753657575854675 ) ) ;
#59142=ADVANCED_FACE ( 'NONE', ( #64787 ), #73781, .F. ) ;
#59147=ADVANCED_FACE ( 'NONE', ( #41834 ), #57205, .T. ) ;
#59148=VERTEX_POINT ( 'NONE', #73291 ) ;
#59149=ORIENTED_EDGE ( 'NONE', *, *, #65020, .T. ) ;
#59150=DIRECTION ( 'NONE',  ( 0.000000000000000000, 1.000000000000000000, 0.000000000000000000 ) ) ;
#59162=EDGE_CURVE ( 'NONE', #32363, #7251, #65286, .T. ) ;
#59164=CARTESIAN_POINT ( 'NONE',  ( 9.997910040112605756, 4.102332422533249404E-16, -10.50199004140717562 ) ) ;
#59166=CIRCLE ( 'NONE', #19271, 14.49999999999999822 ) ;
#59167=CARTESIAN_POINT ( 'NONE',  ( -2.638427012816824124, -17.94940218233254825, 9.846743663894596210 ) ) ;
#59170=VERTEX_POINT ( 'NONE', #87794 ) ;
#59172=AXIS2_PLACEMENT_3D ( 'NONE', #23113, #31076, #92085 ) ;
#59176=DIRECTION ( 'NONE',  ( 0.000000000000000000, 0.000000000000000000, -1.000000000000000000 ) ) ;
#59180=CARTESIAN_POINT ( 'NONE',  ( 12.81628187352647608, 11.62363466993042493, -2.602085213965210642E-15 ) ) ;
#59194=CARTESIAN_POINT ( 'NONE',  ( 10.19513985507825637, 0.5000000000000004441, 11.00268709613223983 ) ) ;
#59197=DIRECTION ( 'NONE',  ( 0.000000000000000000, 1.000000000000000000, 0.000000000000000000 ) ) ;
#59203=ORIENTED_EDGE ( 'NONE', *, *, #52387, .F. ) ;
#59205=LINE ( 'NONE', #51222, #45858 ) ;
#59216=CARTESIAN_POINT ( 'NONE',  ( 0.7375392941518293943, 0.5000000000000004441, -14.98185688723470932 ) ) ;
#59217=B_SPLINE_CURVE_WITH_KNOTS ( 'NONE', 3,
 ( #18774, #27234, #63752, #72243, #25299, #19250 ),
 .UNSPECIFIED., .F., .F.,
 ( 4, 2, 4 ),
 ( 3.409110551496116460E-05, 0.0004400426677367864632, 0.0008459942299586117008 ),
 .UNSPECIFIED. ) ;
#59220=CARTESIAN_POINT ( 'NONE',  ( -5.624999999999996447, 5.951366962315985276, 9.742785792574938597 ) ) ;
#59227=DIRECTION ( 'NONE',  ( 0.000000000000000000, 1.000000000000000000, 0.000000000000000000 ) ) ;
#59232=CARTESIAN_POINT ( 'NONE',  ( 14.16423886937410437, 9.095415501580637496, 3.795296366450304770 ) ) ;
#59235=VECTOR ( 'NONE', #10312, 1000.000000000000114 ) ;
#59236=CARTESIAN_POINT ( 'NONE',  ( 14.97687855664614531, 14.49999999999999112, -0.8325315005900779664 ) ) ;
#59238=EDGE_CURVE ( 'NONE', #9538, #54489, #58275, .T. ) ;
#59247=DIRECTION ( 'NONE',  ( 0.000000000000000000, 1.000000000000000000, 0.000000000000000000 ) ) ;
#59270=VECTOR ( 'NONE', #53982, 1000.000000000000114 ) ;
#59272=EDGE_LOOP ( 'NONE', ( #18319, #30144, #2285, #15687, #92626, #37219 ) ) ;
#59287=B_SPLINE_CURVE_WITH_KNOTS ( 'NONE', 3,
 ( #28481, #51979, #58976, #51476, #83948, #13986 ),
 .UNSPECIFIED., .F., .F.,
 ( 4, 2, 4 ),
 ( 3.409110551496083934E-05, 0.0004400426677367859753, 0.0008459942299586110503 ),
 .UNSPECIFIED. ) ;
#59290=EDGE_LOOP ( 'NONE', ( #9872, #39355, #42486, #15384 ) ) ;
#59294=ORIENTED_EDGE ( 'NONE', *, *, #73617, .T. ) ;
#59300=EDGE_CURVE ( 'NONE', #84680, #70377, #51783, .T. ) ;
#59317=CARTESIAN_POINT ( 'NONE',  ( 14.49154782523117291, 14.95037109980596135, 2.766288502469715471 ) ) ;
#59332=ORIENTED_EDGE ( 'NONE', *, *, #53785, .F. ) ;
#59334=CARTESIAN_POINT ( 'NONE',  ( 9.240973841163533820, 15.00000000000000000, 11.17382667070378943 ) ) ;
#59335=DIRECTION ( 'NONE',  ( 0.000000000000000000, 0.000000000000000000, 1.000000000000000000 ) ) ;
#59338=DIRECTION ( 'NONE',  ( -0.000000000000000000, -1.000000000000000000, -0.000000000000000000 ) ) ;
#59341=TOROIDAL_SURFACE ( 'NONE', #97714, 14.49999999999999822, 0.5000000000000000000 ) ;
#59342=CARTESIAN_POINT ( 'NONE',  ( 11.81378540890936080, -0.03417435944610275333, -7.968498874458115999 ) ) ;
#59348=CARTESIAN_POINT ( 'NONE',  ( -1.354709868695410657, 15.00000000000000000, -14.93870011653153362 ) ) ;
#59349=AXIS2_PLACEMENT_3D ( 'NONE', #76069, #7598, #38094 ) ;
#59352=B_SPLINE_CURVE_WITH_KNOTS ( 'NONE', 3,
 ( #89182, #36182, #51687, #7170, #43676, #82666 ),
 .UNSPECIFIED., .F., .F.,
 ( 4, 2, 4 ),
 ( 0.0002800005319459029376, 0.0006862057665691747351, 0.001092411001192446695 ),
 .UNSPECIFIED. ) ;
#59359=CARTESIAN_POINT ( 'NONE',  ( 14.61046065509106029, 15.00000000000000533, 0.6655452423543793961 ) ) ;
#59361=CARTESIAN_POINT ( 'NONE',  ( 0.000000000000000000, 14.49999999999999822, 0.000000000000000000 ) ) ;
#59372=ORIENTED_EDGE ( 'NONE', *, *, #65266, .F. ) ;
#59382=CARTESIAN_POINT ( 'NONE',  ( 0.000000000000000000, 0.000000000000000000, 14.25000000000000000 ) ) ;
#59383=CARTESIAN_POINT ( 'NONE',  ( -7.860426697680325425, -0.03417435944610275333, -13.93165778241942832 ) ) ;
#59386=B_SPLINE_CURVE_WITH_KNOTS ( 'NONE', 3,
 ( #86960, #48959, #79469, #10967, #71958, #11926 ),
 .UNSPECIFIED., .F., .F.,
 ( 4, 2, 4 ),
 ( 0.0002800020636817269993, 0.0006862073132860365288, 0.001092412562890346167 ),
 .UNSPECIFIED. ) ;
#59388=EDGE_CURVE ( 'NONE', #28267, #4086, #76745, .T. ) ;
#59394=EDGE_CURVE ( 'NONE', #19380, #56358, #44764, .T. ) ;
#59403=VERTEX_POINT ( 'NONE', #83269 ) ;
#59413=FACE_OUTER_BOUND ( 'NONE', #47045, .T. ) ;
#59417=DIRECTION ( 'NONE',  ( 0.000000000000000000, 0.000000000000000000, 1.000000000000000000 ) ) ;
#59420=DIRECTION ( 'NONE',  ( 0.000000000000000000, 1.000000000000000000, 0.000000000000000000 ) ) ;
#59422=ORIENTED_EDGE ( 'NONE', *, *, #7131, .F. ) ;
#59425=CARTESIAN_POINT ( 'NONE',  ( 3.469446951953614189E-15, -19.62636533006957507, 12.81628187352647608 ) ) ;
#59437=ORIENTED_EDGE ( 'NONE', *, *, #46885, .T. ) ;
#59448=CARTESIAN_POINT ( 'NONE',  ( 9.075906804202286793, 15.00000000000000000, -13.17214151599837990 ) ) ;
#59451=DIRECTION ( 'NONE',  ( -0.9636304532086211738, 0.000000000000000000, -0.2672383760782636175 ) ) ;
#59452=B_SPLINE_CURVE_WITH_KNOTS ( 'NONE', 3,
 ( #75586, #36098, #21110, #82093, #97625, #13604 ),
 .UNSPECIFIED., .F., .F.,
 ( 4, 2, 4 ),
 ( 3.409110551415738455E-05, 0.0004400426677360065966, 0.0008459942299578557950 ),
 .UNSPECIFIED. ) ;
#59457=VECTOR ( 'NONE', #33358, 1000.000000000000000 ) ;
#59478=EDGE_CURVE ( 'NONE', #49035, #43285, #87039, .T. ) ;
#59481=CARTESIAN_POINT ( 'NONE',  ( 12.26659068614894821, -16.11291783175269643, 7.082119434687044190 ) ) ;
#59482=CIRCLE ( 'NONE', #16390, 14.49999999999999822 ) ;
#59492=VECTOR ( 'NONE', #78268, 1000.000000000000000 ) ;
#59494=AXIS2_PLACEMENT_3D ( 'NONE', #28846, #13365, #36364 ) ;
#59497=AXIS2_PLACEMENT_3D ( 'NONE', #9003, #17013, #47491 ) ;
#59499=CARTESIAN_POINT ( 'NONE',  ( -9.422509992056136596, 23.48035201082151957, 5.440088680355559703 ) ) ;
#59505=DIRECTION ( 'NONE',  ( -0.000000000000000000, -1.000000000000000000, -0.000000000000000000 ) ) ;
#59506=ORIENTED_EDGE ( 'NONE', *, *, #84593, .T. ) ;
#59518=FACE_OUTER_BOUND ( 'NONE', #41867, .T. ) ;
#59521=CARTESIAN_POINT ( 'NONE',  ( 5.419894505350532299, 14.49999999999999112, 13.98659156302467466 ) ) ;
#59522=ADVANCED_FACE ( 'NONE', ( #44270 ), #30743, .F. ) ;
#59526=DIRECTION ( 'NONE',  ( 0.000000000000000000, 0.000000000000000000, 1.000000000000000000 ) ) ;
#59533=DIRECTION ( 'NONE',  ( -0.3826834323650877834, 0.000000000000000000, 0.9238795325112876267 ) ) ;
#59535=VERTEX_POINT ( 'NONE', #98801 ) ;
#59549=DIRECTION ( 'NONE',  ( 0.000000000000000000, 0.000000000000000000, -1.000000000000000000 ) ) ;
#59550=CARTESIAN_POINT ( 'NONE',  ( 3.469446951953614189E-15, 12.25893115100078923, 9.846743663894594434 ) ) ;
#59552=VERTEX_POINT ( 'NONE', #37783 ) ;
#59553=CARTESIAN_POINT ( 'NONE',  ( 1.114591949025028450, 15.00000000000000000, -14.45709807627964416 ) ) ;
#59564=ORIENTED_EDGE ( 'NONE', *, *, #86071, .T. ) ;
#59565=AXIS2_PLACEMENT_3D ( 'NONE', #61182, #90691, #82205 ) ;
#59567=AXIS2_PLACEMENT_3D ( 'NONE', #85826, #63785, #93315 ) ;
#59571=EDGE_LOOP ( 'NONE', ( #1594, #7618, #79497, #30540 ) ) ;
#59575=VECTOR ( 'NONE', #60510, 1000.000000000000000 ) ;
#59578=CARTESIAN_POINT ( 'NONE',  ( -15.61289147378506748, -0.03417435944610275333, -3.480663193108890496 ) ) ;
#59582=DIRECTION ( 'NONE',  ( 0.000000000000000000, 1.000000000000000000, 0.000000000000000000 ) ) ;
#59584=CARTESIAN_POINT ( 'NONE',  ( 12.00809552683959325, 14.49999999999999112, 8.989195838243645653 ) ) ;
#59589=CARTESIAN_POINT ( 'NONE',  ( -3.927832320392065313, -0.03417435944610275333, -13.69797916712109398 ) ) ;
#59594=ADVANCED_FACE ( 'NONE', ( #90763 ), #2924, .T. ) ;
#59596=DIRECTION ( 'NONE',  ( 0.000000000000000000, 1.000000000000000000, 0.000000000000000000 ) ) ;
#59597=TOROIDAL_SURFACE ( 'NONE', #81940, 14.49999999999999822, 0.5000000000000000000 ) ;
#59600=VERTEX_POINT ( 'NONE', #27316 ) ;
#59613=CARTESIAN_POINT ( 'NONE',  ( 2.915334737309928315, -10.47798132251182857, 10.88017736071109987 ) ) ;
#59617=CARTESIAN_POINT ( 'NONE',  ( 14.97687855664607781, 0.5000000000000004441, 0.8325315005901553489 ) ) ;
#59621=CARTESIAN_POINT ( 'NONE',  ( 0.000000000000000000, 14.49999999999999822, 0.000000000000000000 ) ) ;
#59625=VECTOR ( 'NONE', #48629, 1000.000000000000000 ) ;
#59641=DIRECTION ( 'NONE',  ( -0.000000000000000000, -1.000000000000000000, -0.000000000000000000 ) ) ;
#59644=B_SPLINE_CURVE_WITH_KNOTS ( 'NONE', 3,
 ( #16314, #357, #39804, #38822, #31295, #46798 ),
 .UNSPECIFIED., .F., .F.,
 ( 4, 2, 4 ),
 ( 0.0002800047503720844394, 0.0006862100262544157739, 0.001092415302136747271 ),
 .UNSPECIFIED. ) ;
#59645=CARTESIAN_POINT ( 'NONE',  ( 11.62719953690064933, 15.00000000000000000, -9.476720473301794456 ) ) ;
#59647=ORIENTED_EDGE ( 'NONE', *, *, #14741, .F. ) ;
#59648=ORIENTED_EDGE ( 'NONE', *, *, #94363, .F. ) ;
#59655=CARTESIAN_POINT ( 'NONE',  ( -3.836325488036279818, 14.49999999999999822, 14.50112432709419963 ) ) ;
#59663=CARTESIAN_POINT ( 'NONE',  ( 8.527530157486179263, -26.90773551566588040, 4.923371831947292776 ) ) ;
#59664=VERTEX_POINT ( 'NONE', #92144 ) ;
#59665=CARTESIAN_POINT ( 'NONE',  ( 9.240973841163606650, 4.560084876699663581E-16, -11.17382667070372726 ) ) ;
#59677=CARTESIAN_POINT ( 'NONE',  ( -5.204170427930421283E-15, 22.87363466993042138, -12.81628187352647608 ) ) ;
#59678=VERTEX_POINT ( 'NONE', #15672 ) ;
#59690=VERTEX_POINT ( 'NONE', #187 ) ;
#59692=DIRECTION ( 'NONE',  ( 0.000000000000000000, 0.000000000000000000, -1.000000000000000000 ) ) ;
#59701=CARTESIAN_POINT ( 'NONE',  ( -12.98685442714190508, 4.246409518909109890E-16, -6.449155920601135072 ) ) ;
#59707=CARTESIAN_POINT ( 'NONE',  ( 9.010802615327829557, 0.2301505768537819852, 11.91753657575788772 ) ) ;
#59714=DIRECTION ( 'NONE',  ( 0.9762960071199331402, 0.000000000000000000, 0.2164396139381037087 ) ) ;
#59718=ORIENTED_EDGE ( 'NONE', *, *, #31602, .F. ) ;
#59731=CARTESIAN_POINT ( 'NONE',  ( 3.795296366450314540, 18.26208216824730712, 14.16423886937410082 ) ) ;
#59743=LINE ( 'NONE', #13261, #64262 ) ;
#59752=DIRECTION ( 'NONE',  ( 0.6883545756937599069, 0.000000000000000000, -0.7253743710122820820 ) ) ;
#59756=FACE_OUTER_BOUND ( 'NONE', #74551, .T. ) ;
#59760=CARTESIAN_POINT ( 'NONE',  ( 4.856092091438321212, -3.602007608198911403E-15, -13.79590085420553081 ) ) ;
#59763=ORIENTED_EDGE ( 'NONE', *, *, #82293, .F. ) ;
#59778=AXIS2_PLACEMENT_3D ( 'NONE', #16093, #74612, #38118 ) ;
#59787=CARTESIAN_POINT ( 'NONE',  ( 15.33206046421389601, 15.00000000000000000, 4.561284726668865197 ) ) ;
#59788=ORIENTED_EDGE ( 'NONE', *, *, #31761, .F. ) ;
#59794=ORIENTED_EDGE ( 'NONE', *, *, #18281, .F. ) ;
#59795=VERTEX_POINT ( 'NONE', #22179 ) ;
#59819=FACE_OUTER_BOUND ( 'NONE', #78598, .T. ) ;
#59824=B_SPLINE_CURVE_WITH_KNOTS ( 'NONE', 3,
 ( #8396, #77369, #91395, #92380, #83411, #8880 ),
 .UNSPECIFIED., .F., .F.,
 ( 4, 2, 4 ),
 ( 0.0002800553958269931185, 0.0006862611673083514937, 0.001092466938789709869 ),
 .UNSPECIFIED. ) ;
#59829=STYLED_ITEM ( 'NONE', ( #2815 ), #72777 ) ;
#59832=AXIS2_PLACEMENT_3D ( 'NONE', #73379, #28384, #11410 ) ;
#59833=ADVANCED_FACE ( 'NONE', ( #10615 ), #86616, .T. ) ;
#59835=LINE ( 'NONE', #66852, #96759 ) ;
#59857=ORIENTED_EDGE ( 'NONE', *, *, #97438, .F. ) ;
#59860=FACE_OUTER_BOUND ( 'NONE', #51516, .T. ) ;
#59861=CARTESIAN_POINT ( 'NONE',  ( -2.189108318723541391, -3.647747387350642832E-15, -14.46085460646901666 ) ) ;
#59868=EDGE_CURVE ( 'NONE', #28932, #15789, #79623, .T. ) ;
#59879=CARTESIAN_POINT ( 'NONE',  ( -5.963430220938290560, 1.828790035174478135, -10.32896413005679648 ) ) ;
#59881=AXIS2_PLACEMENT_3D ( 'NONE', #72577, #64579, #27081 ) ;
#59889=CARTESIAN_POINT ( 'NONE',  ( -8.375939845167600595, -0.03417435944610275333, -11.52849216984310310 ) ) ;
#59896=ORIENTED_EDGE ( 'NONE', *, *, #56714, .F. ) ;
#59902=B_SPLINE_CURVE_WITH_KNOTS ( 'NONE', 3,
 ( #77309, #8823, #33761, #10799, #2337, #55811 ),
 .UNSPECIFIED., .F., .F.,
 ( 4, 2, 4 ),
 ( 0.000000000000000000, 0.0004056965545342633298, 0.0008113931090685266596 ),
 .UNSPECIFIED. ) ;
#59903=EDGE_LOOP ( 'NONE', ( #66210, #7189, #91590, #75779, #11456, #72609 ) ) ;
#59907=DIRECTION ( 'NONE',  ( 0.000000000000000000, 0.000000000000000000, 1.000000000000000000 ) ) ;
#59912=LINE ( 'NONE', #42955, #25403 ) ;
#59918=CARTESIAN_POINT ( 'NONE',  ( 12.81628187352647252, -23.16803199673623936, -3.434112377981059172 ) ) ;
#59922=DIRECTION ( 'NONE',  ( 0.000000000000000000, 1.000000000000000000, 0.000000000000000000 ) ) ;
#59930=EDGE_LOOP ( 'NONE', ( #78986, #62714, #78943, #43693 ) ) ;
#59934=EDGE_LOOP ( 'NONE', ( #45427, #71106, #36320, #64840 ) ) ;
#59939=VECTOR ( 'NONE', #61809, 1000.000000000000114 ) ;
#59949=ADVANCED_FACE ( 'NONE', ( #1166 ), #17636, .F. ) ;
#59954=EDGE_CURVE ( 'NONE', #1208, #70377, #95608, .T. ) ;
#59962=CARTESIAN_POINT ( 'NONE',  ( 14.82679024690670566, 0.2306972965111901697, 1.845086899513388001 ) ) ;
#59971=CARTESIAN_POINT ( 'NONE',  ( -10.36894250292379205, -13.82125116508603035, -10.36894250292378672 ) ) ;
#59975=AXIS2_PLACEMENT_3D ( 'NONE', #57375, #18905, #18407 ) ;
#59985=CARTESIAN_POINT ( 'NONE',  ( 1.236172813752255406, 14.95077488074853456, 14.70095156538448755 ) ) ;
#59987=CARTESIAN_POINT ( 'NONE',  ( 9.422509992056141925, 25.14701867748816966, 5.440088680355547268 ) ) ;
#59994=EDGE_CURVE ( 'NONE', #60175, #56402, #77618, .T. ) ;
#59997=CARTESIAN_POINT ( 'NONE',  ( -14.04391541078760675, 4.104531544909319036E-16, -3.608107528143027043 ) ) ;
#59999=VECTOR ( 'NONE', #61948, 1000.000000000000114 ) ;
#60018=VECTOR ( 'NONE', #18175, 1000.000000000000114 ) ;
#60019=CARTESIAN_POINT ( 'NONE',  ( 12.22474924877146307, 0.2301506569030462857, -8.589397507024894907 ) ) ;
#60028=DIRECTION ( 'NONE',  ( -0.000000000000000000, -1.000000000000000000, -0.000000000000000000 ) ) ;
#60035=B_SPLINE_CURVE_WITH_KNOTS ( 'NONE', 3,
 ( #95735, #33726, #19237, #71270, #27218, #19726 ),
 .UNSPECIFIED., .F., .F.,
 ( 4, 2, 4 ),
 ( 3.409110551494650755E-05, 0.0004400426677367923721, 0.0008459942299586381553 ),
 .UNSPECIFIED. ) ;
#60037=CARTESIAN_POINT ( 'NONE',  ( -9.846743663894594434, 11.00893115100079456, 3.469446951953614189E-15 ) ) ;
#60040=DIRECTION ( 'NONE',  ( -0.3173046564050833740, 0.000000000000000000, -0.9483236552062022096 ) ) ;
#60050=ORIENTED_EDGE ( 'NONE', *, *, #40681, .T. ) ;
#60053=ORIENTED_EDGE ( 'NONE', *, *, #31485, .F. ) ;
#60059=B_SPLINE_CURVE_WITH_KNOTS ( 'NONE', 3,
 ( #48165, #78678, #56179, #18177, #55171, #79159 ),
 .UNSPECIFIED., .F., .F.,
 ( 4, 2, 4 ),
 ( 0.0002800225282680484967, 0.0006862279780657134631, 0.001092433427863378484 ),
 .UNSPECIFIED. ) ;
#60062=DIRECTION ( 'NONE',  ( -0.000000000000000000, -1.000000000000000000, -0.000000000000000000 ) ) ;
#60063=ORIENTED_EDGE ( 'NONE', *, *, #46970, .T. ) ;
#60066=EDGE_LOOP ( 'NONE', ( #62996, #37118, #2974, #58695, #33040, #12162 ) ) ;
#60070=ORIENTED_EDGE ( 'NONE', *, *, #70682, .T. ) ;
#60075=CARTESIAN_POINT ( 'NONE',  ( 11.49658347684022708, 0.04962891477616669655, -9.245857368719784475 ) ) ;
#60077=CARTESIAN_POINT ( 'NONE',  ( 6.741983435833523330, 14.95077488074853456, -13.12218577464087232 ) ) ;
#60078=TOROIDAL_SURFACE ( 'NONE', #29752, 14.49999999999999822, 0.5000000000000000000 ) ;
#60085=ORIENTED_EDGE ( 'NONE', *, *, #60523, .F. ) ;
#60093=CARTESIAN_POINT ( 'NONE',  ( 7.264509831664694772, 14.76984904925306274, -13.05561747642790138 ) ) ;
#60099=CARTESIAN_POINT ( 'NONE',  ( 7.964842623401177768, -13.81131465584516071, -7.964842623401181321 ) ) ;
#60103=CARTESIAN_POINT ( 'NONE',  ( -11.22915323889586858, 0.000000000000000000, 8.773176023390528044 ) ) ;
#60112=CARTESIAN_POINT ( 'NONE',  ( -7.313705784284448619, 0.3639312656126391099, -13.09617149020755633 ) ) ;
#60113=VECTOR ( 'NONE', #25780, 1000.000000000000000 ) ;
#60127=LINE ( 'NONE', #67146, #31439 ) ;
#60129=CIRCLE ( 'NONE', #80842, 15.00000000000000000 ) ;
#60134=ORIENTED_EDGE ( 'NONE', *, *, #52040, .T. ) ;
#60135=ORIENTED_EDGE ( 'NONE', *, *, #21453, .T. ) ;
#60152=CARTESIAN_POINT ( 'NONE',  ( -9.846743663894594434, -23.99106884899920900, 3.469446951953614189E-15 ) ) ;
#60154=LINE ( 'NONE', #14182, #77891 ) ;
#60160=FACE_OUTER_BOUND ( 'NONE', #23306, .T. ) ;
#60169=ADVANCED_FACE ( 'NONE', ( #1660 ), #6192, .T. ) ;
#60170=CARTESIAN_POINT ( 'NONE',  ( -6.408140936763246032, 18.29030133659709279, -11.09922568453594316 ) ) ;
#60175=VERTEX_POINT ( 'NONE', #19584 ) ;
#60181=EDGE_CURVE ( 'NONE', #85753, #22949, #50082, .T. ) ;
#60182=CARTESIAN_POINT ( 'NONE',  ( 14.04867373755350890, -0.03417435944610275333, 7.649324326489743697 ) ) ;
#60185=CARTESIAN_POINT ( 'NONE',  ( -3.881785064875369784, 15.00000000000000711, 14.10213074188650140 ) ) ;
#60187=EDGE_CURVE ( 'NONE', #33570, #73111, #22253, .T. ) ;
#60188=CARTESIAN_POINT ( 'NONE',  ( 0.000000000000000000, 15.00000000000000000, 0.000000000000000000 ) ) ;
#60189=DIRECTION ( 'NONE',  ( -0.3826834323650877279, 0.000000000000000000, 0.9238795325112876267 ) ) ;
#60196=CARTESIAN_POINT ( 'NONE',  ( -4.862001128006591344, 4.779775600002961917E-16, -13.66056166602466604 ) ) ;
#60205=CARTESIAN_POINT ( 'NONE',  ( 9.065164099344453774, 0.5000000000000004441, 11.95084933600773169 ) ) ;
#60210=VECTOR ( 'NONE', #33022, 1000.000000000000000 ) ;
#60216=VERTEX_POINT ( 'NONE', #27570 ) ;
#60222=DIRECTION ( 'NONE',  ( 0.000000000000000000, 0.000000000000000000, 1.000000000000000000 ) ) ;
#60228=CARTESIAN_POINT ( 'NONE',  ( -14.16423886937409726, 22.01208216824731778, 3.795296366450320757 ) ) ;
#60242=CARTESIAN_POINT ( 'NONE',  ( 0.000000000000000000, 15.00000000000000000, 0.000000000000000000 ) ) ;
#60243=FACE_OUTER_BOUND ( 'NONE', #89336, .T. ) ;
#60245=CARTESIAN_POINT ( 'NONE',  ( 2.815433093577024426, 0.5000000000000004441, 14.73340885523751709 ) ) ;
#60251=DIRECTION ( 'NONE',  ( -0.7253743710122820820, 0.000000000000000000, -0.6883545756937599069 ) ) ;
#60255=DIRECTION ( 'NONE',  ( 0.000000000000000000, 0.000000000000000000, 1.000000000000000000 ) ) ;
#60270=CARTESIAN_POINT ( 'NONE',  ( -6.138934250732154041, 15.00000000000000000, 14.77128574976603481 ) ) ;
#60281=VERTEX_POINT ( 'NONE', #46044 ) ;
#60282=AXIS2_PLACEMENT_3D ( 'NONE', #50379, #96399, #82354 ) ;
#60290=ORIENTED_EDGE ( 'NONE', *, *, #6279, .T. ) ;
#60291=CIRCLE ( 'NONE', #93832, 15.00000000000000000 ) ;
#60292=EDGE_CURVE ( 'NONE', #96379, #21109, #1497, .T. ) ;
#60294=EDGE_CURVE ( 'NONE', #47390, #3873, #21571, .T. ) ;
#60295=EDGE_CURVE ( 'NONE', #12471, #83600, #23831, .T. ) ;
#60299=ORIENTED_EDGE ( 'NONE', *, *, #11611, .T. ) ;
#60300=ORIENTED_EDGE ( 'NONE', *, *, #88430, .T. ) ;
#60303=DIRECTION ( 'NONE',  ( 0.000000000000000000, 1.000000000000000000, 0.000000000000000000 ) ) ;
#60308=ORIENTED_EDGE ( 'NONE', *, *, #6234, .T. ) ;
#60311=DIRECTION ( 'NONE',  ( 0.000000000000000000, 0.000000000000000000, 1.000000000000000000 ) ) ;
#60315=EDGE_CURVE ( 'NONE', #43044, #57022, #90536, .T. ) ;
#60316=CARTESIAN_POINT ( 'NONE',  ( -14.62617646268082972, 15.00000000000000000, -3.327906561567078647 ) ) ;
#60322=CARTESIAN_POINT ( 'NONE',  ( 14.69227023463712456, 0.04922511925149390677, -1.335400878252530843 ) ) ;
#60330=EDGE_LOOP ( 'NONE', ( #5507, #64913, #58804, #33682, #20090, #72688 ) ) ;
#60336=CARTESIAN_POINT ( 'NONE',  ( -9.876730923139437124, 14.49999999999999112, 11.28938378619059613 ) ) ;
#60338=DIRECTION ( 'NONE',  ( 0.5519369853120676961, 0.000000000000000000, -0.8338858220671618859 ) ) ;
#60347=CIRCLE ( 'NONE', #17273, 15.00000000000000000 ) ;
#60355=CARTESIAN_POINT ( 'NONE',  ( 0.000000000000000000, 0.5000000000000004441, 0.000000000000000000 ) ) ;
#60360=B_SPLINE_CURVE_WITH_KNOTS ( 'NONE', 3,
 ( #40702, #92708, #56202, #10697, #56678, #93195 ),
 .UNSPECIFIED., .F., .F.,
 ( 4, 2, 4 ),
 ( 0.0002800912045253039183, 0.0006862973266949682705, 0.001092503448864632623 ),
 .UNSPECIFIED. ) ;
#60361=CARTESIAN_POINT ( 'NONE',  ( 11.48952521350015488, 15.00000000000000000, 8.845383562533813304 ) ) ;
#60366=CARTESIAN_POINT ( 'NONE',  ( 10.17198128013144043, 14.76930270348881180, -10.94389562857665688 ) ) ;
#60367=LINE ( 'NONE', #66890, #46377 ) ;
#60372=DIRECTION ( 'NONE',  ( -0.000000000000000000, -1.000000000000000000, -0.000000000000000000 ) ) ;
#60374=EDGE_CURVE ( 'NONE', #30081, #49327, #370, .T. ) ;
#60377=LINE ( 'NONE', #82891, #1140 ) ;
#60383=CARTESIAN_POINT ( 'NONE',  ( 0.000000000000000000, 0.000000000000000000, 0.000000000000000000 ) ) ;
#60389=VECTOR ( 'NONE', #73274, 1000.000000000000000 ) ;
#60392=EDGE_CURVE ( 'NONE', #98676, #38633, #22070, .T. ) ;
#60413=ORIENTED_EDGE ( 'NONE', *, *, #7373, .T. ) ;
#60415=CARTESIAN_POINT ( 'NONE',  ( -3.434112377981047626, -19.83469866340291077, 12.81628187352647963 ) ) ;
#60418=LINE ( 'NONE', #92393, #16406 ) ;
#60423=AXIS2_PLACEMENT_3D ( 'NONE', #56484, #27448, #47984 ) ;
#60424=DIRECTION ( 'NONE',  ( 0.000000000000000000, 0.000000000000000000, -1.000000000000000000 ) ) ;
#60425=ORIENTED_EDGE ( 'NONE', *, *, #6143, .T. ) ;
#60431=ORIENTED_EDGE ( 'NONE', *, *, #45890, .T. ) ;
#60440=CARTESIAN_POINT ( 'NONE',  ( 12.25993886608599581, 0.5000000000000004441, 8.642563219313704082 ) ) ;
#60444=EDGE_CURVE ( 'NONE', #74987, #35164, #51567, .T. ) ;
#60446=CARTESIAN_POINT ( 'NONE',  ( -11.62719953690055164, 14.49999999999999112, -9.476720473302012948 ) ) ;
#60459=CARTESIAN_POINT ( 'NONE',  ( -5.624999999999996447, 10.95136696231598883, 9.742785792574938597 ) ) ;
#60460=CIRCLE ( 'NONE', #73218, 15.00000000000000000 ) ;
#60470=CARTESIAN_POINT ( 'NONE',  ( -12.26659068614894110, -17.77958449841936073, 7.082119434687058401 ) ) ;
#60474=ORIENTED_EDGE ( 'NONE', *, *, #57319, .F. ) ;
#60480=FACE_OUTER_BOUND ( 'NONE', #72597, .T. ) ;
#60482=CARTESIAN_POINT ( 'NONE',  ( -9.159723438033276821, -0.03417435944610275333, 10.91613331444536250 ) ) ;
#60483=LINE ( 'NONE', #88139, #35616 ) ;
#60486=CARTESIAN_POINT ( 'NONE',  ( 5.440088680355549045, 26.39701867748816966, -9.422509992056141925 ) ) ;
#60492=EDGE_LOOP ( 'NONE', ( #58657, #32642, #41657, #24420 ) ) ;
#60493=EDGE_CURVE ( 'NONE', #44552, #88245, #26532, .T. ) ;
#60497=DIRECTION ( 'NONE',  ( -0.9099612708765398850, 0.000000000000000000, -0.4146932426562461860 ) ) ;
#60504=DIRECTION ( 'NONE',  ( -0.000000000000000000, -1.000000000000000000, -0.000000000000000000 ) ) ;
#60506=ORIENTED_EDGE ( 'NONE', *, *, #90514, .F. ) ;
#60510=DIRECTION ( 'NONE',  ( -0.000000000000000000, -1.000000000000000000, -0.000000000000000000 ) ) ;
#60516=DIRECTION ( 'NONE',  ( -0.9588197348681947174, 0.000000000000000000, 0.2840153447039170387 ) ) ;
#60523=EDGE_CURVE ( 'NONE', #28000, #68696, #32499, .T. ) ;
#60532=EDGE_CURVE ( 'NONE', #63992, #60570, #78987, .T. ) ;
#60533=CARTESIAN_POINT ( 'NONE',  ( 12.22506292814020945, 14.76930270348882068, -8.589871424854703008 ) ) ;
#60536=CARTESIAN_POINT ( 'NONE',  ( -8.527530157486173934, 21.42559781766745175, 4.923371831947302546 ) ) ;
#60537=ORIENTED_EDGE ( 'NONE', *, *, #70589, .T. ) ;
#60538=VECTOR ( 'NONE', #31103, 1000.000000000000000 ) ;
#60550=B_SPLINE_CURVE_WITH_KNOTS ( 'NONE', 3,
 ( #39982, #24500, #39499, #1516, #62964, #69988 ),
 .UNSPECIFIED., .F., .F.,
 ( 4, 2, 4 ),
 ( 3.409110551496101553E-05, 0.0004400426677367863006, 0.0008459942299586115924 ),
 .UNSPECIFIED. ) ;
#60557=B_SPLINE_CURVE_WITH_KNOTS ( 'NONE', 3,
 ( #35981, #20499, #66483, #50498, #27984, #6476 ),
 .UNSPECIFIED., .F., .F.,
 ( 4, 2, 4 ),
 ( 3.409110551494651432E-05, 0.0004400426677367942152, 0.0008459942299586418416 ),
 .UNSPECIFIED. ) ;
#60558=ORIENTED_EDGE ( 'NONE', *, *, #86246, .F. ) ;
#60565=VECTOR ( 'NONE', #76529, 1000.000000000000114 ) ;
#60568=ORIENTED_EDGE ( 'NONE', *, *, #40605, .T. ) ;
#60570=VERTEX_POINT ( 'NONE', #32988 ) ;
#60571=FACE_OUTER_BOUND ( 'NONE', #64488, .T. ) ;
#60572=CARTESIAN_POINT ( 'NONE',  ( 14.99847009497944583, 0.5000000000000004441, -0.2142307401080305596 ) ) ;
#60573=CIRCLE ( 'NONE', #87913, 15.00000000000000000 ) ;
#60575=DIRECTION ( 'NONE',  ( -0.000000000000000000, -1.000000000000000000, -0.000000000000000000 ) ) ;
#60576=DIRECTION ( 'NONE',  ( 0.000000000000000000, 0.000000000000000000, 1.000000000000000000 ) ) ;
#60580=CARTESIAN_POINT ( 'NONE',  ( 11.36220558718863138, 4.417444789370043464E-16, -9.008345252845243678 ) ) ;
#60587=LINE ( 'NONE', #45089, #50701 ) ;
#60588=VERTEX_POINT ( 'NONE', #17025 ) ;
#60589=ORIENTED_EDGE ( 'NONE', *, *, #75438, .T. ) ;
#60601=CARTESIAN_POINT ( 'NONE',  ( 7.964842623401177768, -8.811314655845162491, -7.964842623401181321 ) ) ;
#60603=CARTESIAN_POINT ( 'NONE',  ( 13.74344568549456902, 0.2301512731879840901, -5.860030649989653284 ) ) ;
#60605=CARTESIAN_POINT ( 'NONE',  ( 14.56195259121195207, 15.00000000000000888, 1.374002722866818793 ) ) ;
#60607=CARTESIAN_POINT ( 'NONE',  ( 14.16722289976688032, 0.3639312946971514084, -4.928467845925542434 ) ) ;
#60608=CARTESIAN_POINT ( 'NONE',  ( -0.3093388210927896509, 14.49999999999999112, 14.99680997725072373 ) ) ;
#60615=CARTESIAN_POINT ( 'NONE',  ( 8.549759589250252034, 0.2301501389895041494, -12.25250350990697612 ) ) ;
#60617=ORIENTED_EDGE ( 'NONE', *, *, #55600, .T. ) ;
#60619=CARTESIAN_POINT ( 'NONE',  ( 3.469446951953614189E-15, 6.368033628982654903, 11.25000000000000178 ) ) ;
#60625=DIRECTION ( 'NONE',  ( 0.000000000000000000, 0.000000000000000000, 1.000000000000000000 ) ) ;
#60647=CARTESIAN_POINT ( 'NONE',  ( -7.208316651077764980, -29.61606884899920900, -7.208316651077759651 ) ) ;
#60650=EDGE_LOOP ( 'NONE', ( #74358, #80667, #28257, #85134 ) ) ;
#60652=VECTOR ( 'NONE', #71263, 1000.000000000000000 ) ;
#60654=LINE ( 'NONE', #38654, #7320 ) ;
#60660=CARTESIAN_POINT ( 'NONE',  ( -6.408140936763232709, 24.95696800326376064, 11.09922568453595026 ) ) ;
#60661=VERTEX_POINT ( 'NONE', #17165 ) ;
#60663=VERTEX_POINT ( 'NONE', #93633 ) ;
#60665=ORIENTED_EDGE ( 'NONE', *, *, #15044, .F. ) ;
#60671=CARTESIAN_POINT ( 'NONE',  ( 13.30156849913881878, 0.2306972965111892537, 6.804875469488154138 ) ) ;
#60675=EDGE_CURVE ( 'NONE', #67193, #65046, #4004, .T. ) ;
#60677=VERTEX_POINT ( 'NONE', #42483 ) ;
#60678=CARTESIAN_POINT ( 'NONE',  ( -0.1034006766821533585, 0.000000000000000000, -14.49963131600461175 ) ) ;
#60688=LINE ( 'NONE', #84202, #92102 ) ;
#60692=CARTESIAN_POINT ( 'NONE',  ( -9.240973841163672375, 15.00000000000000000, 11.17382667070363667 ) ) ;
#60697=B_SPLINE_CURVE_WITH_KNOTS ( 'NONE', 3,
 ( #60580, #67603, #60075, #90577, #98622, #91072 ),
 .UNSPECIFIED., .F., .F.,
 ( 4, 2, 4 ),
 ( 0.0002800338592536525577, 0.0006862394199285712457, 0.001092444980603490042 ),
 .UNSPECIFIED. ) ;
#60700=CARTESIAN_POINT ( 'NONE',  ( 0.000000000000000000, 0.5000000000000004441, 0.000000000000000000 ) ) ;
#60710=LINE ( 'NONE', #61209, #10262 ) ;
#60712=CYLINDRICAL_SURFACE ( 'NONE', #77551, 15.00000000000000000 ) ;
#60716=CARTESIAN_POINT ( 'NONE',  ( -3.795296366450300773, 22.84541550158063927, 14.16423886937410437 ) ) ;
#60720=CARTESIAN_POINT ( 'NONE',  ( -10.19513985507840736, 0.5000000000000004441, 11.00268709613209950 ) ) ;
#60724=VERTEX_POINT ( 'NONE', #45425 ) ;
#60730=DIRECTION ( 'NONE',  ( 0.5372996083468138950, 0.000000000000000000, 0.8433914458128921599 ) ) ;
#60734=ORIENTED_EDGE ( 'NONE', *, *, #53750, .T. ) ;
#60737=DIRECTION ( 'NONE',  ( 0.000000000000000000, 0.000000000000000000, 1.000000000000000000 ) ) ;
#60748=ORIENTED_EDGE ( 'NONE', *, *, #16837, .T. ) ;
#60750=AXIS2_PLACEMENT_3D ( 'NONE', #80122, #34118, #96627 ) ;
#60752=CARTESIAN_POINT ( 'NONE',  ( 11.35178980618974087, 15.00000000000000000, -9.804941009311923139 ) ) ;
#60763=FACE_OUTER_BOUND ( 'NONE', #65152, .T. ) ;
#60765=EDGE_CURVE ( 'NONE', #50106, #65696, #69713, .T. ) ;
#60768=ORIENTED_EDGE ( 'NONE', *, *, #37027, .T. ) ;
#60779=( BOUNDED_CURVE ( )  B_SPLINE_CURVE ( 2, ( #94883, #26382, #56881, #18902, #26879, #28836, #42384, #35855, #88371, #72861, #5860, #96882, #36353 ),
 .UNSPECIFIED., .F., .F. ) 
 B_SPLINE_CURVE_WITH_KNOTS ( ( 3, 2, 2, 2, 2, 2, 3 ),
 ( 0.6333333333333333037, 0.6388888888888888395, 0.6444444444444444864, 0.6500000000000000222, 0.6555555555555555580, 0.6611111111111110938, 0.6666666666666666297 ),
 .UNSPECIFIED. ) 
 CURVE ( )  GEOMETRIC_REPRESENTATION_ITEM ( )  RATIONAL_B_SPLINE_CURVE ( ( 1.000000000000000000, 0.9659258262890684232, 1.000000000000000000, 0.9659258262890684232, 1.000000000000000000, 0.9659258262890684232, 1.000000000000000000, 0.9659258262890684232, 1.000000000000000000, 0.9659258262890684232, 1.000000000000000000, 0.9659258262890684232, 1.000000000000000000 ) ) 
 REPRESENTATION_ITEM ( '' )  );
#60793=EDGE_LOOP ( 'NONE', ( #8610, #56733, #26445, #37390 ) ) ;
#60794=DIRECTION ( 'NONE',  ( -0.6883545756937501370, 0.000000000000000000, -0.7253743710122912969 ) ) ;
#60796=CARTESIAN_POINT ( 'NONE',  ( 12.34086200392826882, -0.03417435944610275333, -7.124999999999971578 ) ) ;
#60803=DIRECTION ( 'NONE',  ( 0.000000000000000000, 0.000000000000000000, 1.000000000000000000 ) ) ;
#60817=B_SPLINE_CURVE_WITH_KNOTS ( 'NONE', 3,
 ( #8620, #55088, #69129, #92116, #77594, #53618 ),
 .UNSPECIFIED., .F., .F.,
 ( 4, 2, 4 ),
 ( 0.0002800124554126355017, 0.0006862178066638149887, 0.001092423157914994367 ),
 .UNSPECIFIED. ) ;
#60825=PLANE ( 'NONE',  #95059 ) ;
#60833=VECTOR ( 'NONE', #93773, 1000.000000000000000 ) ;
#60835=CARTESIAN_POINT ( 'NONE',  ( 13.55255535720595184, -0.03417435944610275333, -4.403492169842965431 ) ) ;
#60838=EDGE_CURVE ( 'NONE', #16656, #48202, #67452, .T. ) ;
#60841=AXIS2_PLACEMENT_3D ( 'NONE', #82818, #23329, #60803 ) ;
#60843=DIRECTION ( 'NONE',  ( 0.4924235601034769316, 0.000000000000000000, -0.8703556959398940363 ) ) ;
#60848=CARTESIAN_POINT ( 'NONE',  ( 12.87890026492933515, 14.95077488074853456, 7.195834080858436899 ) ) ;
#60857=CARTESIAN_POINT ( 'NONE',  ( -14.99847009497948136, 0.3639309181704115104, -0.2142307401082224061 ) ) ;
#60863=DIRECTION ( 'NONE',  ( 4.440892098500626162E-14, 0.000000000000000000, 1.000000000000000000 ) ) ;
#60868=CARTESIAN_POINT ( 'NONE',  ( -9.722841580490317881, -0.03417435944610275333, -12.70211588817950066 ) ) ;
#60885=ORIENTED_EDGE ( 'NONE', *, *, #45642, .T. ) ;
#60892=VERTEX_POINT ( 'NONE', #74217 ) ;
#60894=DIRECTION ( 'NONE',  ( 0.000000000000000000, 1.000000000000000000, 0.000000000000000000 ) ) ;
#60902=CARTESIAN_POINT ( 'NONE',  ( -14.11917416961162353, 0.2306972965111909191, -4.887430353539129690 ) ) ;
#60904=ORIENTED_EDGE ( 'NONE', *, *, #8210, .T. ) ;
#60906=CARTESIAN_POINT ( 'NONE',  ( 12.81628187352647608, -8.376365330069578619, -2.602085213965210642E-15 ) ) ;
#60909=AXIS2_PLACEMENT_3D ( 'NONE', #12137, #42640, #78676 ) ;
#60911=DIRECTION ( 'NONE',  ( 0.000000000000000000, 0.000000000000000000, 1.000000000000000000 ) ) ;
#60931=CARTESIAN_POINT ( 'NONE',  ( -8.157990163924628391, 14.76930270348881002, -12.51739793958124380 ) ) ;
#60943=CARTESIAN_POINT ( 'NONE',  ( -2.863771337576333842, 14.95037103301162418, -14.47259902956233013 ) ) ;
#60945=CARTESIAN_POINT ( 'NONE',  ( -11.25000000000000178, 9.909700295649315649, -3.014428414850122806 ) ) ;
#60950=DIRECTION ( 'NONE',  ( -0.000000000000000000, -1.000000000000000000, -0.000000000000000000 ) ) ;
#60955=CARTESIAN_POINT ( 'NONE',  ( -10.36894250292378317, -7.571251165086024137, 10.36894250292379560 ) ) ;
#60967=DIRECTION ( 'NONE',  ( -0.3665012267243009103, 0.000000000000000000, 0.9304175679820231304 ) ) ;
#60972=CARTESIAN_POINT ( 'NONE',  ( -10.88017736071109987, 33.27201867748819097, 2.915334737309934532 ) ) ;
#60982=CARTESIAN_POINT ( 'NONE',  ( -15.94536257719939698, -0.03417435944610275333, -1.273895096820171657 ) ) ;
#60983=CIRCLE ( 'NONE', #21094, 14.49999999999999822 ) ;
#60988=CARTESIAN_POINT ( 'NONE',  ( 0.000000000000000000, 15.00000000000000000, 0.000000000000000000 ) ) ;
#60992=VERTEX_POINT ( 'NONE', #58221 ) ;
#60997=EDGE_CURVE ( 'NONE', #24087, #3541, #8497, .T. ) ;
#61001=FACE_OUTER_BOUND ( 'NONE', #90059, .T. ) ;
#61004=LINE ( 'NONE', #55, #63501 ) ;
#61007=CARTESIAN_POINT ( 'NONE',  ( 6.382347221874455023, 14.63606860869882986, -13.57444820018230480 ) ) ;
#61010=B_SPLINE_CURVE_WITH_KNOTS ( 'NONE', 3,
 ( #66829, #81340, #80361, #28340, #95867, #27350 ),
 .UNSPECIFIED., .F., .F.,
 ( 4, 2, 4 ),
 ( 3.409110551496214039E-05, 0.0004400426677368013710, 0.0008459942299586405406 ),
 .UNSPECIFIED. ) ;
#61012=ORIENTED_EDGE ( 'NONE', *, *, #28997, .T. ) ;
#61024=DIRECTION ( 'NONE',  ( -0.000000000000000000, 1.000000000000000000, -0.000000000000000000 ) ) ;
#61025=CARTESIAN_POINT ( 'NONE',  ( 7.208316651077762316, 14.13393115100078923, -7.208316651077764980 ) ) ;
#61027=CARTESIAN_POINT ( 'NONE',  ( 1.326261724323017699, 14.76984959128329677, -14.88164196614431845 ) ) ;
#61050=EDGE_CURVE ( 'NONE', #77207, #51781, #81437, .T. ) ;
#61053=VECTOR ( 'NONE', #97733, 1000.000000000000000 ) ;
#61056=VERTEX_POINT ( 'NONE', #5750 ) ;
#61057=FACE_OUTER_BOUND ( 'NONE', #21824, .T. ) ;
#61059=VECTOR ( 'NONE', #11137, 1000.000000000000000 ) ;
#61061=AXIS2_PLACEMENT_3D ( 'NONE', #97961, #30901, #91413 ) ;
#61063=EDGE_LOOP ( 'NONE', ( #32468, #39869, #37796, #84470, #87886, #88553 ) ) ;
#61064=CARTESIAN_POINT ( 'NONE',  ( 0.000000000000000000, 15.00000000000000000, 0.000000000000000000 ) ) ;
#61065=CARTESIAN_POINT ( 'NONE',  ( 0.000000000000000000, 0.5000000000000004441, 0.000000000000000000 ) ) ;
#61075=AXIS2_PLACEMENT_3D ( 'NONE', #2, #83959, #15485 ) ;
#61077=EDGE_CURVE ( 'NONE', #47253, #17634, #80257, .T. ) ;
#61081=EDGE_CURVE ( 'NONE', #13218, #49035, #22523, .T. ) ;
#61089=CARTESIAN_POINT ( 'NONE',  ( -13.82192141328807011, 3.982798640990670655E-16, -4.382292601468863680 ) ) ;
#61093=CARTESIAN_POINT ( 'NONE',  ( -10.88017736071109987, -6.727981322511824125, 2.915334737309934532 ) ) ;
#61099=CARTESIAN_POINT ( 'NONE',  ( -0.3093388210927806581, 14.63606905933214364, 14.99680997725070242 ) ) ;
#61101=AXIS2_PLACEMENT_3D ( 'NONE', #39790, #48254, #77769 ) ;
#61108=DIRECTION ( 'NONE',  ( -0.1478094111296046620, 0.000000000000000000, -0.9890158633619178241 ) ) ;
#61113=FACE_OUTER_BOUND ( 'NONE', #16768, .T. ) ;
#61114=EDGE_CURVE ( 'NONE', #32515, #16129, #52227, .T. ) ;
#61124=VERTEX_POINT ( 'NONE', #69695 ) ;
#61125=ORIENTED_EDGE ( 'NONE', *, *, #37057, .T. ) ;
#61138=PLANE ( 'NONE',  #9264 ) ;
#61141=CARTESIAN_POINT ( 'NONE',  ( 8.527530157486175710, -21.07440218233254470, -4.923371831947298993 ) ) ;
#61144=VECTOR ( 'NONE', #88560, 1000.000000000000000 ) ;
#61146=DIRECTION ( 'NONE',  ( 0.000000000000000000, 0.000000000000000000, 1.000000000000000000 ) ) ;
#61154=B_SPLINE_CURVE_WITH_KNOTS ( 'NONE', 3,
 ( #40057, #30570, #53572, #1590, #1094, #38585 ),
 .UNSPECIFIED., .F., .F.,
 ( 4, 2, 4 ),
 ( 3.409110551494641945E-05, 0.0004400426677367909084, 0.0008459942299586353364 ),
 .UNSPECIFIED. ) ;
#61156=CARTESIAN_POINT ( 'NONE',  ( 6.408140936763243367, 25.79030133659709989, 11.09922568453594494 ) ) ;
#61167=CARTESIAN_POINT ( 'NONE',  ( 10.58223187591001135, 14.76930270348881002, 10.54772123337538048 ) ) ;
#61172=CARTESIAN_POINT ( 'NONE',  ( -3.836325488036278042, 14.63595249122790598, 14.50112432709420318 ) ) ;
#61173=ORIENTED_EDGE ( 'NONE', *, *, #64354, .T. ) ;
#61174=AXIS2_PLACEMENT_3D ( 'NONE', #72714, #59197, #36212 ) ;
#61175=CARTESIAN_POINT ( 'NONE',  ( -14.42956166533734041, -3.121739927105722716E-15, -2.386684097925192205 ) ) ;
#61182=CARTESIAN_POINT ( 'NONE',  ( 0.000000000000000000, 0.5000000000000004441, 0.000000000000000000 ) ) ;
#61184=EDGE_LOOP ( 'NONE', ( #94598, #25406, #95989, #13811, #77249, #24347 ) ) ;
#61185=DIRECTION ( 'NONE',  ( -0.02617694830786282401, 0.000000000000000000, -0.9996573249755575929 ) ) ;
#61186=FACE_OUTER_BOUND ( 'NONE', #80680, .T. ) ;
#61190=DIRECTION ( 'NONE',  ( -0.000000000000000000, 1.000000000000000000, 0.000000000000000000 ) ) ;
#61197=EDGE_CURVE ( 'NONE', #69916, #92653, #9040, .T. ) ;
#61207=VECTOR ( 'NONE', #5033, 1000.000000000000114 ) ;
#61208=CARTESIAN_POINT ( 'NONE',  ( -7.640985187756333730, 0.04962896822202291641, 12.62032702733647049 ) ) ;
#61209=CARTESIAN_POINT ( 'NONE',  ( -11.81378540890942119, 15.00000000000000000, 7.968498874458034287 ) ) ;
#61211=CARTESIAN_POINT ( 'NONE',  ( -5.056330833731569108, 4.047076681631624764E-16, -13.58983143750706724 ) ) ;
#61216=CARTESIAN_POINT ( 'NONE',  ( 3.795296366450314540, 13.26208216824729647, 14.16423886937410082 ) ) ;
#61223=VERTEX_POINT ( 'NONE', #16204 ) ;
#61233=ORIENTED_EDGE ( 'NONE', *, *, #73229, .F. ) ;
#61239=DIRECTION ( 'NONE',  ( 0.000000000000000000, 1.000000000000000000, 0.000000000000000000 ) ) ;
#61245=ADVANCED_FACE ( 'NONE', ( #8692 ), #92049, .T. ) ;
#61270=CARTESIAN_POINT ( 'NONE',  ( 3.866399090317279796, 14.95077488074853456, -14.23717170745771909 ) ) ;
#61273=AXIS2_PLACEMENT_3D ( 'NONE', #66155, #59150, #43170 ) ;
#61274=ORIENTED_EDGE ( 'NONE', *, *, #69435, .T. ) ;
#61277=ORIENTED_EDGE ( 'NONE', *, *, #50275, .F. ) ;
#61282=CARTESIAN_POINT ( 'NONE',  ( 14.11917416961165195, 0.2306972965111870610, 4.887430353539040873 ) ) ;
#61286=EDGE_CURVE ( 'NONE', #7312, #22776, #92199, .T. ) ;
#61295=FACE_OUTER_BOUND ( 'NONE', #23168, .T. ) ;
#61301=CYLINDRICAL_SURFACE ( 'NONE', #40228, 15.00000000000000000 ) ;
#61311=EDGE_CURVE ( 'NONE', #83674, #10324, #44719, .T. ) ;
#61317=EDGE_CURVE ( 'NONE', #79877, #91116, #60129, .T. ) ;
#61328=CARTESIAN_POINT ( 'NONE',  ( -11.81378540890942119, -0.03417435944610275333, 7.968498874458034287 ) ) ;
#61335=ORIENTED_EDGE ( 'NONE', *, *, #43887, .F. ) ;
#61339=CARTESIAN_POINT ( 'NONE',  ( 14.88232117145535760, 14.49999999999999112, 1.875237731503272887 ) ) ;
#61348=AXIS2_PLACEMENT_3D ( 'NONE', #18670, #94160, #77681 ) ;
#61354=CARTESIAN_POINT ( 'NONE',  ( 9.399392868737814766, 15.00000000000000000, -11.04089732309474314 ) ) ;
#61355=CARTESIAN_POINT ( 'NONE',  ( 0.000000000000000000, 0.000000000000000000, 0.000000000000000000 ) ) ;
#61360=CARTESIAN_POINT ( 'NONE',  ( -11.92686044187656336, 2.870456701841150871, 3.195792623639540864 ) ) ;
#61362=EDGE_CURVE ( 'NONE', #97076, #47923, #37752, .T. ) ;
#61373=EDGE_CURVE ( 'NONE', #17685, #93052, #45217, .T. ) ;
#61376=VERTEX_POINT ( 'NONE', #735 ) ;
#61378=VECTOR ( 'NONE', #8745, 1000.000000000000227 ) ;
#61385=CARTESIAN_POINT ( 'NONE',  ( 4.180366052176762715, -2.683400376901622685E-15, 14.01545757926331071 ) ) ;
#61388=CARTESIAN_POINT ( 'NONE',  ( -13.82192141328815715, 15.00000000000000000, 4.382292601468586568 ) ) ;
#61389=CARTESIAN_POINT ( 'NONE',  ( -14.56311970191030625, 14.76984991344722253, 3.337330457605781397 ) ) ;
#61404=EDGE_CURVE ( 'NONE', #18352, #51389, #33598, .T. ) ;
#61411=ORIENTED_EDGE ( 'NONE', *, *, #22160, .T. ) ;
#61421=CARTESIAN_POINT ( 'NONE',  ( 8.813102413620015341, -0.03417435944610275333, 13.34940531570970457 ) ) ;
#61427=CIRCLE ( 'NONE', #16775, 14.49999999999999822 ) ;
#61437=CARTESIAN_POINT ( 'NONE',  ( -9.159723438033054776, 15.00000000000000000, -10.91613331444555079 ) ) ;
#61445=AXIS2_PLACEMENT_3D ( 'NONE', #23178, #36695, #28681 ) ;
#61446=CARTESIAN_POINT ( 'NONE',  ( 11.62006642628028175, 14.99999999999807088, -8.881585844848984834 ) ) ;
#61449=CARTESIAN_POINT ( 'NONE',  ( -7.082119434687044190, -12.36291783175269643, 12.26659068614894998 ) ) ;
#61465=CARTESIAN_POINT ( 'NONE',  ( -14.56089864659467814, -3.220842781934475856E-15, -1.374314915485489896 ) ) ;
#61471=LINE ( 'NONE', #45996, #8885 ) ;
#61474=EDGE_CURVE ( 'NONE', #15967, #44777, #77184, .T. ) ;
#61476=DIRECTION ( 'NONE',  ( 0.2672383760782571227, 0.000000000000000000, 0.9636304532086229502 ) ) ;
#61479=AXIS2_PLACEMENT_3D ( 'NONE', #22838, #68826, #45323 ) ;
#61492=CARTESIAN_POINT ( 'NONE',  ( 0.000000000000000000, 14.49999999999999822, 0.000000000000000000 ) ) ;
#61496=DIRECTION ( 'NONE',  ( -0.6755902076156641289, 0.000000000000000000, 0.7372773368101205316 ) ) ;
#61513=CARTESIAN_POINT ( 'NONE',  ( 11.09922568453595026, -38.79303199673623936, 6.408140936763232709 ) ) ;
#61514=ORIENTED_EDGE ( 'NONE', *, *, #4197, .T. ) ;
#61515=ORIENTED_EDGE ( 'NONE', *, *, #70529, .T. ) ;
#61522=VECTOR ( 'NONE', #81078, 1000.000000000000114 ) ;
#61524=VECTOR ( 'NONE', #19663, 1000.000000000000000 ) ;
#61525=ADVANCED_FACE ( 'NONE', ( #3666 ), #96854, .T. ) ;
#61527=ADVANCED_FACE ( 'NONE', ( #94651 ), #86177, .F. ) ;
#61528=ORIENTED_EDGE ( 'NONE', *, *, #10862, .T. ) ;
#61531=VERTEX_POINT ( 'NONE', #48159 ) ;
#61543=EDGE_LOOP ( 'NONE', ( #6583, #67526, #46896, #94476, #93385, #30897 ) ) ;
#61548=CARTESIAN_POINT ( 'NONE',  ( 6.767445849361247490, 15.00000000000000000, -13.38662304974496564 ) ) ;
#61551=EDGE_CURVE ( 'NONE', #80599, #31483, #66495, .T. ) ;
#61566=AXIS2_PLACEMENT_3D ( 'NONE', #986, #15973, #29107 ) ;
#61579=CARTESIAN_POINT ( 'NONE',  ( 7.964842623401181321, -0.06131465584516315737, 7.964842623401174215 ) ) ;
#61581=DIRECTION ( 'NONE',  ( -0.7132504491541847846, 0.000000000000000000, 0.7009092642998475675 ) ) ;
#61584=AXIS2_PLACEMENT_3D ( 'NONE', #66739, #36243, #34246 ) ;
#61588=DIRECTION ( 'NONE',  ( -0.000000000000000000, -1.000000000000000000, -0.000000000000000000 ) ) ;
#61594=ORIENTED_EDGE ( 'NONE', *, *, #74873, .T. ) ;
#61602=LINE ( 'NONE', #85109, #63350 ) ;
#61607=AXIS2_PLACEMENT_3D ( 'NONE', #71847, #26832, #85876 ) ;
#61608=ORIENTED_EDGE ( 'NONE', *, *, #3663, .F. ) ;
#61621=CARTESIAN_POINT ( 'NONE',  ( -0.7375392941519317569, 15.00000000000000000, 14.98185688723470044 ) ) ;
#61623=CARTESIAN_POINT ( 'NONE',  ( 7.208316651077764980, -17.11606884899921255, 7.208316651077762316 ) ) ;
#61624=ORIENTED_EDGE ( 'NONE', *, *, #66318, .T. ) ;
#61635=CARTESIAN_POINT ( 'NONE',  ( 9.382169495545419124, 20.99863466993042493, 9.382169495545417348 ) ) ;
#61636=ADVANCED_FACE ( 'NONE', ( #85190 ), #79153, .F. ) ;
#61637=ORIENTED_EDGE ( 'NONE', *, *, #28003, .F. ) ;
#61649=LINE ( 'NONE', #6210, #77612 ) ;
#61651=DIRECTION ( 'NONE',  ( 0.000000000000000000, 0.000000000000000000, 1.000000000000000000 ) ) ;
#61654=DIRECTION ( 'NONE',  ( 0.8616291604415267091, 0.000000000000000000, 0.5075383629607025382 ) ) ;
#61661=FACE_OUTER_BOUND ( 'NONE', #47971, .T. ) ;
#61668=B_SPLINE_CURVE_WITH_KNOTS ( 'NONE', 3,
 ( #51464, #44939, #13467, #75445, #89949, #43949 ),
 .UNSPECIFIED., .F., .F.,
 ( 4, 2, 4 ),
 ( 3.409110551496204552E-05, 0.0004400426677368010999, 0.0008459942299586402153 ),
 .UNSPECIFIED. ) ;
#61682=CARTESIAN_POINT ( 'NONE',  ( 6.728956594450720807, 1.228197773518735097E-15, 12.98689685418147555 ) ) ;
#61686=LINE ( 'NONE', #44723, #83933 ) ;
#61689=FACE_OUTER_BOUND ( 'NONE', #29939, .T. ) ;
#61691=CARTESIAN_POINT ( 'NONE',  ( 1.780824192092403058, 0.5000000000000004441, 14.89391369643514729 ) ) ;
#61692=CARTESIAN_POINT ( 'NONE',  ( -7.082119434687058401, 20.97041550158063217, -12.26659068614894110 ) ) ;
#61702=CARTESIAN_POINT ( 'NONE',  ( -13.82192141328815715, 15.00000000000000000, 4.382292601468586568 ) ) ;
#61703=VERTEX_POINT ( 'NONE', #2702 ) ;
#61708=DIRECTION ( 'NONE',  ( 0.000000000000000000, 1.000000000000000000, 0.000000000000000000 ) ) ;
#61713=VERTEX_POINT ( 'NONE', #3172 ) ;
#61724=EDGE_CURVE ( 'NONE', #26974, #77529, #83190, .T. ) ;
#61728=EDGE_LOOP ( 'NONE', ( #95082, #17719, #88886, #82066 ) ) ;
#61730=CARTESIAN_POINT ( 'NONE',  ( 5.625000000000005329, 4.588468844518209799, 9.742785792574933268 ) ) ;
#61737=AXIS2_PLACEMENT_3D ( 'NONE', #1526, #38522, #93479 ) ;
#61744=ORIENTED_EDGE ( 'NONE', *, *, #89951, .T. ) ;
#61745=DIRECTION ( 'NONE',  ( -0.02617694830787627158, 0.000000000000000000, 0.9996573249755572599 ) ) ;
#61749=VERTEX_POINT ( 'NONE', #71176 ) ;
#61755=ORIENTED_EDGE ( 'NONE', *, *, #38637, .F. ) ;
#61758=DIRECTION ( 'NONE',  ( -0.000000000000000000, -1.000000000000000000, -0.000000000000000000 ) ) ;
#61765=ORIENTED_EDGE ( 'NONE', *, *, #2386, .F. ) ;
#61768=DIRECTION ( 'NONE',  ( 0.000000000000000000, 0.000000000000000000, 1.000000000000000000 ) ) ;
#61772=AXIS2_PLACEMENT_3D ( 'NONE', #89891, #29382, #37903 ) ;
#61774=TOROIDAL_SURFACE ( 'NONE', #77765, 14.49999999999999822, 0.5000000000000000000 ) ;
#61781=B_SPLINE_CURVE_WITH_KNOTS ( 'NONE', 3,
 ( #43483, #97014, #20998, #51486, #81981, #47425 ),
 .UNSPECIFIED., .F., .F.,
 ( 4, 2, 4 ),
 ( 3.409110551467034092E-05, 0.0004400426677364971981, 0.0008459942299583240620 ),
 .UNSPECIFIED. ) ;
#61787=CARTESIAN_POINT ( 'NONE',  ( 7.860426697680415131, 15.00000000000000000, 13.93165778241937680 ) ) ;
#61792=AXIS2_PLACEMENT_3D ( 'NONE', #43385, #65390, #27397 ) ;
#61809=DIRECTION ( 'NONE',  ( -0.1132032137678971873, 0.000000000000000000, -0.9935718556765885667 ) ) ;
#61812=CARTESIAN_POINT ( 'NONE',  ( -13.78891971893204804, 14.49999999999999112, -5.904717858191772528 ) ) ;
#61817=CARTESIAN_POINT ( 'NONE',  ( -5.815502996284770632, 0.2306972965111892260, -13.76292046016129866 ) ) ;
#61818=DIRECTION ( 'NONE',  ( -0.9981347984218673641, 0.000000000000000000, 0.06104853953484969120 ) ) ;
#61819=PLANE ( 'NONE',  #34791 ) ;
#61824=ORIENTED_EDGE ( 'NONE', *, *, #30600, .F. ) ;
#61835=VERTEX_POINT ( 'NONE', #84112 ) ;
#61841=VECTOR ( 'NONE', #93519, 1000.000000000000114 ) ;
#61852=EDGE_CURVE ( 'NONE', #11368, #60663, #30061, .T. ) ;
#61855=VECTOR ( 'NONE', #14302, 1000.000000000000000 ) ;
#61866=ORIENTED_EDGE ( 'NONE', *, *, #96714, .T. ) ;
#61869=ORIENTED_EDGE ( 'NONE', *, *, #67877, .T. ) ;
#61878=LINE ( 'NONE', #98446, #92956 ) ;
#61889=CARTESIAN_POINT ( 'NONE',  ( 0.000000000000000000, 15.00000000000000000, 0.000000000000000000 ) ) ;
#61899=ORIENTED_EDGE ( 'NONE', *, *, #78556, .T. ) ;
#61906=CARTESIAN_POINT ( 'NONE',  ( 0.000000000000000000, 14.49999999999999822, 0.000000000000000000 ) ) ;
#61908=CARTESIAN_POINT ( 'NONE',  ( 14.94699059465105684, 14.63606911935685595, -1.259949270174804736 ) ) ;
#61913=CARTESIAN_POINT ( 'NONE',  ( 12.03829478939421982, 8.656676720938946507E-16, 8.307695547791484003 ) ) ;
#61916=ORIENTED_EDGE ( 'NONE', *, *, #72024, .T. ) ;
#61918=CARTESIAN_POINT ( 'NONE',  ( 2.815433093577122126, 0.5000000000000004441, -14.73340885523749932 ) ) ;
#61922=DIRECTION ( 'NONE',  ( -0.000000000000000000, 1.000000000000000000, 0.000000000000000000 ) ) ;
#61939=B_SPLINE_CURVE_WITH_KNOTS ( 'NONE', 3,
 ( #34021, #96031, #74001, #20521, #27515, #58007 ),
 .UNSPECIFIED., .F., .F.,
 ( 4, 2, 4 ),
 ( 3.409110551494655498E-05, 0.0004400426677367920468, 0.0008459942299586376132 ),
 .UNSPECIFIED. ) ;
#61940=CARTESIAN_POINT ( 'NONE',  ( -14.16423886937409726, -7.987917831752695541, 3.795296366450320757 ) ) ;
#61946=DIRECTION ( 'NONE',  ( 0.000000000000000000, 1.000000000000000000, 0.000000000000000000 ) ) ;
#61948=DIRECTION ( 'NONE',  ( -0.2334453638558956767, 0.000000000000000000, -0.9723699203976788885 ) ) ;
#61955=CARTESIAN_POINT ( 'NONE',  ( 0.000000000000000000, 0.5000000000000004441, 0.000000000000000000 ) ) ;
#61963=DIRECTION ( 'NONE',  ( 0.000000000000000000, 1.000000000000000000, 0.000000000000000000 ) ) ;
#61964=ORIENTED_EDGE ( 'NONE', *, *, #93389, .T. ) ;
#61983=CYLINDRICAL_SURFACE ( 'NONE', #51352, 15.00000000000000000 ) ;
#61987=EDGE_LOOP ( 'NONE', ( #85527, #46735, #25969, #71259 ) ) ;
#61991=DIRECTION ( 'NONE',  ( -0.000000000000000000, -1.000000000000000000, -0.000000000000000000 ) ) ;
#61996=ADVANCED_FACE ( 'NONE', ( #17099 ), #47582, .F. ) ;
#62003=LINE ( 'NONE', #77015, #97141 ) ;
#62005=ADVANCED_FACE ( 'NONE', ( #34032 ), #2605, .F. ) ;
#62007=CARTESIAN_POINT ( 'NONE',  ( 12.81628187352647608, -38.58469866340291077, 3.434112377981052511 ) ) ;
#62019=ORIENTED_EDGE ( 'NONE', *, *, #90552, .F. ) ;
#62026=CARTESIAN_POINT ( 'NONE',  ( 5.963430220938287007, 6.354976035794178024, 10.32896413005679825 ) ) ;
#62034=ORIENTED_EDGE ( 'NONE', *, *, #45259, .T. ) ;
#62051=AXIS2_PLACEMENT_3D ( 'NONE', #49098, #41622, #26586 ) ;
#62054=AXIS2_PLACEMENT_3D ( 'NONE', #88220, #28213, #41279 ) ;
#62057=VERTEX_POINT ( 'NONE', #9582 ) ;
#62061=ADVANCED_FACE ( 'NONE', ( #48553 ), #40083, .F. ) ;
#62068=CARTESIAN_POINT ( 'NONE',  ( 9.422509992056141925, -4.852981322511822349, 5.440088680355547268 ) ) ;
#62070=CARTESIAN_POINT ( 'NONE',  ( 14.94699059465104440, 0.3639308806417268505, 1.259949270174905767 ) ) ;
#62079=EDGE_CURVE ( 'NONE', #34327, #3454, #28855, .T. ) ;
#62080=ADVANCED_FACE ( 'NONE', ( #94551 ), #79054, .T. ) ;
#62084=FACE_OUTER_BOUND ( 'NONE', #89944, .T. ) ;
#62099=VERTEX_POINT ( 'NONE', #10569 ) ;
#62114=CARTESIAN_POINT ( 'NONE',  ( -8.527530157486182816, -4.407735515665881287, -4.923371831947288335 ) ) ;
#62115=ORIENTED_EDGE ( 'NONE', *, *, #70361, .F. ) ;
#62117=ORIENTED_EDGE ( 'NONE', *, *, #79376, .F. ) ;
#62125=VECTOR ( 'NONE', #93002, 1000.000000000000000 ) ;
#62132=ORIENTED_EDGE ( 'NONE', *, *, #44189, .T. ) ;
#62142=DIRECTION ( 'NONE',  ( -0.000000000000000000, -1.000000000000000000, -0.000000000000000000 ) ) ;
#62144=CARTESIAN_POINT ( 'NONE',  ( -8.606322355891443010, 15.00000000000000000, 11.66967075398801335 ) ) ;
#62152=ORIENTED_EDGE ( 'NONE', *, *, #96311, .F. ) ;
#62169=ORIENTED_EDGE ( 'NONE', *, *, #84063, .T. ) ;
#62174=DIRECTION ( 'NONE',  ( -0.000000000000000000, -1.000000000000000000, -0.000000000000000000 ) ) ;
#62181=CARTESIAN_POINT ( 'NONE',  ( 9.422509992056141925, -34.01964798917848753, -5.440088680355554374 ) ) ;
#62183=ADVANCED_FACE ( 'NONE', ( #55583 ), #49056, .F. ) ;
#62193=ORIENTED_EDGE ( 'NONE', *, *, #49448, .T. ) ;
#62201=EDGE_CURVE ( 'NONE', #54738, #87096, #40582, .T. ) ;
#62210=AXIS2_PLACEMENT_3D ( 'NONE', #27895, #11918, #21399 ) ;
#62219=CIRCLE ( 'NONE', #68661, 14.49999999999999822 ) ;
#62222=PLANE ( 'NONE',  #34667 ) ;
#62224=VERTEX_POINT ( 'NONE', #33058 ) ;
#62225=LINE ( 'NONE', #17246, #43705 ) ;
#62232=DIRECTION ( 'NONE',  ( 0.000000000000000000, 0.000000000000000000, 1.000000000000000000 ) ) ;
#62236=FACE_OUTER_BOUND ( 'NONE', #7936, .T. ) ;
#62241=VERTEX_POINT ( 'NONE', #65016 ) ;
#62249=CARTESIAN_POINT ( 'NONE',  ( 6.898461952320343649, 4.875757609050324087E-16, 12.75387089053313971 ) ) ;
#62250=EDGE_LOOP ( 'NONE', ( #16764, #69639, #66366, #16695 ) ) ;
#62259=LINE ( 'NONE', #53791, #92891 ) ;
#62268=EDGE_LOOP ( 'NONE', ( #72400, #42839, #50527, #58073 ) ) ;
#62269=CARTESIAN_POINT ( 'NONE',  ( 11.12471383767606525, 12.50000000000035527, 1.674288514511126591 ) ) ;
#62282=FACE_OUTER_BOUND ( 'NONE', #13015, .T. ) ;
#62296=CARTESIAN_POINT ( 'NONE',  ( -5.803070148808410877, 15.00000000000000000, 13.28812917035381780 ) ) ;
#62303=LINE ( 'NONE', #61328, #57669 ) ;
#62313=FACE_OUTER_BOUND ( 'NONE', #61184, .T. ) ;
#62314=CARTESIAN_POINT ( 'NONE',  ( 4.181050312904970312, 15.00000000000000888, 14.01631781289605705 ) ) ;
#62317=EDGE_CURVE ( 'NONE', #22095, #42454, #17684, .T. ) ;
#62322=ORIENTED_EDGE ( 'NONE', *, *, #13914, .T. ) ;
#62323=DIRECTION ( 'NONE',  ( 0.3826834323650877834, -0.000000000000000000, -0.9238795325112876267 ) ) ;
#62329=CARTESIAN_POINT ( 'NONE',  ( 13.95697193428308758, -2.801561473043597583E-15, 4.371663894958916607 ) ) ;
#62334=CARTESIAN_POINT ( 'NONE',  ( 7.860426697680415131, -0.03417435944610275333, 13.93165778241937680 ) ) ;
#62335=DIRECTION ( 'NONE',  ( -0.000000000000000000, -1.000000000000000000, -0.000000000000000000 ) ) ;
#62339=CIRCLE ( 'NONE', #19236, 13.75000000000001776 ) ;
#62343=CARTESIAN_POINT ( 'NONE',  ( -11.22915323889568562, -0.03417435944610275333, -8.773176023390764300 ) ) ;
#62351=EDGE_CURVE ( 'NONE', #13980, #65168, #78334, .T. ) ;
#62356=ORIENTED_EDGE ( 'NONE', *, *, #86246, .T. ) ;
#62359=ORIENTED_EDGE ( 'NONE', *, *, #13989, .F. ) ;
#62381=DIRECTION ( 'NONE',  ( 0.000000000000000000, 0.000000000000000000, 1.000000000000000000 ) ) ;
#62382=ORIENTED_EDGE ( 'NONE', *, *, #85831, .T. ) ;
#62383=B_SPLINE_CURVE_WITH_KNOTS ( 'NONE', 3,
 ( #61354, #882, #84853, #46841, #98903, #53866 ),
 .UNSPECIFIED., .F., .F.,
 ( 4, 2, 4 ),
 ( 0.0002800289709862387156, 0.0006862344838250689603, 0.001092439996663899368 ),
 .UNSPECIFIED. ) ;
#62386=EDGE_LOOP ( 'NONE', ( #80217, #87365, #43942, #43150 ) ) ;
#62392=CARTESIAN_POINT ( 'NONE',  ( -14.24131928502210975, 15.00000000000000000, -0.4973178280107823923 ) ) ;
#62395=ADVANCED_FACE ( 'NONE', ( #11544 ), #51212, .T. ) ;
#62399=ORIENTED_EDGE ( 'NONE', *, *, #51375, .F. ) ;
#62401=AXIS2_PLACEMENT_3D ( 'NONE', #25584, #33542, #78078 ) ;
#62403=CARTESIAN_POINT ( 'NONE',  ( 0.000000000000000000, 0.000000000000000000, 0.000000000000000000 ) ) ;
#62409=CARTESIAN_POINT ( 'NONE',  ( -11.35178980618960409, 0.5000000000000004441, -9.804941009312079458 ) ) ;
#62416=CARTESIAN_POINT ( 'NONE',  ( -3.836325488035982278, 14.49999999999999112, -14.50112432709434351 ) ) ;
#62419=ORIENTED_EDGE ( 'NONE', *, *, #9639, .F. ) ;
#62421=CARTESIAN_POINT ( 'NONE',  ( -12.60589901313213979, 0.3639308464568737911, -8.129656208642234816 ) ) ;
#62422=DIRECTION ( 'NONE',  ( -0.000000000000000000, -1.000000000000000000, -0.000000000000000000 ) ) ;
#62425=CARTESIAN_POINT ( 'NONE',  ( 14.16423886937410437, -10.90458449841935717, 3.795296366450304770 ) ) ;
#62428=EDGE_CURVE ( 'NONE', #85153, #88314, #73540, .T. ) ;
#62431=CARTESIAN_POINT ( 'NONE',  ( -9.240973841163453883, 4.157471065789850032E-16, -11.17382667070385160 ) ) ;
#62432=CARTESIAN_POINT ( 'NONE',  ( 0.000000000000000000, 15.00000000000000000, 0.000000000000000000 ) ) ;
#62442=CARTESIAN_POINT ( 'NONE',  ( 0.000000000000000000, 14.49999999999999822, 0.000000000000000000 ) ) ;
#62448=ORIENTED_EDGE ( 'NONE', *, *, #2058, .F. ) ;
#62449=TOROIDAL_SURFACE ( 'NONE', #32111, 14.49999999999999822, 0.5000000000000000000 ) ;
#62453=FACE_OUTER_BOUND ( 'NONE', #33601, .T. ) ;
#62460=CARTESIAN_POINT ( 'NONE',  ( 12.98685442714199390, 3.839196892837649736E-16, -6.449155920600954772 ) ) ;
#62461=CARTESIAN_POINT ( 'NONE',  ( 0.000000000000000000, 14.49999999999999822, 0.000000000000000000 ) ) ;
#62475=DIRECTION ( 'NONE',  ( -0.6225146366376129725, 0.000000000000000000, -0.7826081568524191345 ) ) ;
#62476=ADVANCED_FACE ( 'NONE', ( #90490 ), #81604, .F. ) ;
#62480=VERTEX_POINT ( 'NONE', #8004 ) ;
#62492=LINE ( 'NONE', #24032, #9318 ) ;
#62496=CARTESIAN_POINT ( 'NONE',  ( -2.638427012816840111, 24.96726448433411960, -9.846743663894590881 ) ) ;
#62515=CARTESIAN_POINT ( 'NONE',  ( 5.795997163830076460, 15.00000000000000000, 13.01802277140709663 ) ) ;
#62518=DIRECTION ( 'NONE',  ( 0.000000000000000000, 1.000000000000000000, 0.000000000000000000 ) ) ;
#62519=EDGE_CURVE ( 'NONE', #19933, #92892, #25756, .T. ) ;
#62525=VERTEX_POINT ( 'NONE', #52019 ) ;
#62526=ORIENTED_EDGE ( 'NONE', *, *, #72467, .T. ) ;
#62527=CARTESIAN_POINT ( 'NONE',  ( 0.000000000000000000, 15.00000000000000000, 0.000000000000000000 ) ) ;
#62532=PLANE ( 'NONE',  #49062 ) ;
#62533=FACE_OUTER_BOUND ( 'NONE', #47989, .T. ) ;
#62537=ORIENTED_EDGE ( 'NONE', *, *, #7939, .T. ) ;
#62543=CARTESIAN_POINT ( 'NONE',  ( 0.2076750170234817061, 14.95077488074853811, 14.75137184266415247 ) ) ;
#62547=ORIENTED_EDGE ( 'NONE', *, *, #97728, .T. ) ;
#62557=EDGE_CURVE ( 'NONE', #22303, #24915, #98538, .T. ) ;
#62558=CARTESIAN_POINT ( 'NONE',  ( -0.9940297508535884674, 0.000000000000000000, -14.21528771620250886 ) ) ;
#62561=CARTESIAN_POINT ( 'NONE',  ( -10.88017736071110342, 3.063685344154846835, 3.903127820947815962E-15 ) ) ;
#62564=TOROIDAL_SURFACE ( 'NONE', #48150, 14.49999999999999822, 0.5000000000000000000 ) ;
#62567=DIRECTION ( 'NONE',  ( -0.000000000000000000, -1.000000000000000000, -0.000000000000000000 ) ) ;
#62576=CARTESIAN_POINT ( 'NONE',  ( -10.39655283154092125, 0.04922511925147211170, 10.46698568711257771 ) ) ;
#62578=ORIENTED_EDGE ( 'NONE', *, *, #71722, .F. ) ;
#62588=EDGE_CURVE ( 'NONE', #14583, #84680, #44995, .T. ) ;
#62589=DIRECTION ( 'NONE',  ( 0.000000000000000000, 1.000000000000000000, 0.000000000000000000 ) ) ;
#62591=ORIENTED_EDGE ( 'NONE', *, *, #10058, .F. ) ;
#62592=AXIS2_PLACEMENT_3D ( 'NONE', #45032, #67559, #43070 ) ;
#62602=CARTESIAN_POINT ( 'NONE',  ( 0.000000000000000000, 15.00000000000000000, 0.000000000000000000 ) ) ;
#62604=CARTESIAN_POINT ( 'NONE',  ( -9.846743663894594434, -13.99106884899921432, 3.469446951953614189E-15 ) ) ;
#62608=CARTESIAN_POINT ( 'NONE',  ( 0.000000000000000000, 0.5000000000000004441, 0.000000000000000000 ) ) ;
#62609=ORIENTED_EDGE ( 'NONE', *, *, #51144, .F. ) ;
#62616=CARTESIAN_POINT ( 'NONE',  ( -14.16722289976683946, 14.49999999999999112, -4.928467845925748492 ) ) ;
#62618=CARTESIAN_POINT ( 'NONE',  ( -12.81628187352647252, 29.33196800326377840, 3.434112377981066722 ) ) ;
#62621=AXIS2_PLACEMENT_3D ( 'NONE', #74592, #7095, #20111 ) ;
#62628=DIRECTION ( 'NONE',  ( 0.000000000000000000, 1.000000000000000000, 0.000000000000000000 ) ) ;
#62635=ADVANCED_FACE ( 'NONE', ( #14526 ), #7014, .F. ) ;
#62637=CARTESIAN_POINT ( 'NONE',  ( 0.000000000000000000, 15.00000000000000000, 0.000000000000000000 ) ) ;
#62639=DIRECTION ( 'NONE',  ( 0.000000000000000000, 0.000000000000000000, 1.000000000000000000 ) ) ;
#62648=CYLINDRICAL_SURFACE ( 'NONE', #90606, 15.00000000000000000 ) ;
#62649=EDGE_LOOP ( 'NONE', ( #44, #81161, #52907, #89516 ) ) ;
#62655=VERTEX_POINT ( 'NONE', #59997 ) ;
#62658=ADVANCED_FACE ( 'NONE', ( #23016 ), #75993, .F. ) ;
#62663=AXIS2_PLACEMENT_3D ( 'NONE', #85894, #3378, #57350 ) ;
#62665=EDGE_LOOP ( 'NONE', ( #56489, #12829, #91384, #85468 ) ) ;
#62671=LINE ( 'NONE', #40183, #60018 ) ;
#62672=EDGE_CURVE ( 'NONE', #2288, #1302, #92508, .T. ) ;
#62674=FACE_OUTER_BOUND ( 'NONE', #70631, .T. ) ;
#62679=CARTESIAN_POINT ( 'NONE',  ( 10.88017736071109987, -34.22798132251183034, -2.915334737309928315 ) ) ;
#62695=CARTESIAN_POINT ( 'NONE',  ( -2.393480905992949381, 14.63595249122789177, -14.80781041047755409 ) ) ;
#62699=ORIENTED_EDGE ( 'NONE', *, *, #37137, .T. ) ;
#62702=DIRECTION ( 'NONE',  ( 0.000000000000000000, 1.000000000000000000, 0.000000000000000000 ) ) ;
#62709=CARTESIAN_POINT ( 'NONE',  ( -7.595945211628163385, 15.00000000000000000, -12.35117874301652030 ) ) ;
#62714=ORIENTED_EDGE ( 'NONE', *, *, #55391, .F. ) ;
#62715=CARTESIAN_POINT ( 'NONE',  ( 14.47650479471825058, 14.49999999999999112, 3.928206833722148517 ) ) ;
#62716=CARTESIAN_POINT ( 'NONE',  ( -9.159723438033054776, -0.03417435944610275333, -10.91613331444555079 ) ) ;
#62724=DIRECTION ( 'NONE',  ( 0.000000000000000000, 1.000000000000000000, 0.000000000000000000 ) ) ;
#62735=EDGE_LOOP ( 'NONE', ( #98217, #62743, #7662, #40391 ) ) ;
#62737=ORIENTED_EDGE ( 'NONE', *, *, #55835, .T. ) ;
#62743=ORIENTED_EDGE ( 'NONE', *, *, #53761, .T. ) ;
#62745=VECTOR ( 'NONE', #33248, 1000.000000000000000 ) ;
#62746=CARTESIAN_POINT ( 'NONE',  ( 14.99847009497944406, 0.5000000000000004441, 0.2142307401081381124 ) ) ;
#62747=CARTESIAN_POINT ( 'NONE',  ( 12.81628187352647608, -3.584698663402908991, 3.434112377981052511 ) ) ;
#62748=VERTEX_POINT ( 'NONE', #47947 ) ;
#62751=ORIENTED_EDGE ( 'NONE', *, *, #18023, .T. ) ;
#62756=CARTESIAN_POINT ( 'NONE',  ( 9.402796353261127393, 15.00000000000000000, -11.68706210897757103 ) ) ;
#62761=EDGE_LOOP ( 'NONE', ( #25645, #39644, #41715, #37471 ) ) ;
#62762=EDGE_CURVE ( 'NONE', #50542, #23491, #48447, .T. ) ;
#62766=FACE_OUTER_BOUND ( 'NONE', #79995, .T. ) ;
#62770=ADVANCED_FACE ( 'NONE', ( #70472 ), #48060, .T. ) ;
#62776=CARTESIAN_POINT ( 'NONE',  ( 1.683889348827610062E-15, 0.000000000000000000, 13.74999999999999467 ) ) ;
#62789=CARTESIAN_POINT ( 'NONE',  ( 0.000000000000000000, 14.49999999999999822, 0.000000000000000000 ) ) ;
#62791=ORIENTED_EDGE ( 'NONE', *, *, #70485, .T. ) ;
#62801=CARTESIAN_POINT ( 'NONE',  ( 5.378451019861598681, 0.000000000000000000, -0.9000440264802418433 ) ) ;
#62806=ADVANCED_FACE ( 'NONE', ( #62453 ), #12951, .T. ) ;
#62810=CARTESIAN_POINT ( 'NONE',  ( 12.35505582470273644, -0.03417435944610275333, -10.16021613965630443 ) ) ;
#62811=ORIENTED_EDGE ( 'NONE', *, *, #36603, .T. ) ;
#62814=LINE ( 'NONE', #9827, #13184 ) ;
#62822=ORIENTED_EDGE ( 'NONE', *, *, #88225, .F. ) ;
#62830=CARTESIAN_POINT ( 'NONE',  ( 8.209432707284774366, 15.00000000000000000, 12.55409154915492032 ) ) ;
#62832=DIRECTION ( 'NONE',  ( 0.000000000000000000, 0.000000000000000000, -1.000000000000000000 ) ) ;
#62840=VECTOR ( 'NONE', #36888, 1000.000000000000114 ) ;
#62860=VERTEX_POINT ( 'NONE', #39971 ) ;
#62864=ORIENTED_EDGE ( 'NONE', *, *, #10436, .F. ) ;
#62866=LINE ( 'NONE', #54865, #96298 ) ;
#62880=CARTESIAN_POINT ( 'NONE',  ( -14.02068044289383586, 0.3640475087720986269, 5.331089937175563342 ) ) ;
#62886=LINE ( 'NONE', #10877, #59457 ) ;
#62887=ORIENTED_EDGE ( 'NONE', *, *, #71461, .F. ) ;
#62890=ADVANCED_FACE ( 'NONE', ( #54284 ), #68853, .T. ) ;
#62898=LINE ( 'NONE', #70912, #29935 ) ;
#62899=CARTESIAN_POINT ( 'NONE',  ( 9.159723438033203990, -0.03417435944610275333, -10.91613331444542645 ) ) ;
#62901=CARTESIAN_POINT ( 'NONE',  ( -5.888281321711915872, 1.823139558123406223, -10.37198838585826266 ) ) ;
#62902=DIRECTION ( 'NONE',  ( 0.000000000000000000, 1.000000000000000000, 0.000000000000000000 ) ) ;
#62907=VECTOR ( 'NONE', #90139, 1000.000000000000000 ) ;
#62912=CARTESIAN_POINT ( 'NONE',  ( 10.58981376305282041, -0.03417435944610275333, 9.535111140613782510 ) ) ;
#62925=CARTESIAN_POINT ( 'NONE',  ( 10.93781366033349833, 14.49999999999999112, -10.26470809774071569 ) ) ;
#62929=CARTESIAN_POINT ( 'NONE',  ( 3.469446951953614189E-15, -1.946251165086031243, 14.16423886937410259 ) ) ;
#62931=CARTESIAN_POINT ( 'NONE',  ( 15.99538290524656503, -0.03417435944610275333, 0.1584996864329874799 ) ) ;
#62934=FACE_OUTER_BOUND ( 'NONE', #95091, .T. ) ;
#62936=DIRECTION ( 'NONE',  ( 0.000000000000000000, 0.000000000000000000, -1.000000000000000000 ) ) ;
#62954=DIRECTION ( 'NONE',  ( 0.000000000000000000, 0.000000000000000000, 1.000000000000000000 ) ) ;
#62960=CYLINDRICAL_SURFACE ( 'NONE', #28806, 15.00000000000000000 ) ;
#62963=EDGE_LOOP ( 'NONE', ( #11228, #69054, #98750, #78034, #36303, #26840 ) ) ;
#62964=CARTESIAN_POINT ( 'NONE',  ( 3.881785064875176605, 2.337810934421868936E-16, 14.10213074188657778 ) ) ;
#62973=ORIENTED_EDGE ( 'NONE', *, *, #60374, .T. ) ;
#62978=EDGE_LOOP ( 'NONE', ( #44666, #37291, #70875, #70049 ) ) ;
#62983=AXIS2_PLACEMENT_3D ( 'NONE', #80498, #3042, #64485 ) ;
#62989=VECTOR ( 'NONE', #61946, 1000.000000000000000 ) ;
#62990=CARTESIAN_POINT ( 'NONE',  ( -14.02068044289371684, 14.49999999999999822, -5.331089937175857330 ) ) ;
#62992=CIRCLE ( 'NONE', #37459, 15.00000000000000000 ) ;
#62995=CARTESIAN_POINT ( 'NONE',  ( 3.469446951953614189E-15, 32.25893115100078745, 9.846743663894594434 ) ) ;
#62996=ORIENTED_EDGE ( 'NONE', *, *, #95536, .T. ) ;
#63005=EDGE_CURVE ( 'NONE', #9752, #63527, #4976, .T. ) ;
#63012=ORIENTED_EDGE ( 'NONE', *, *, #24182, .T. ) ;
#63018=CARTESIAN_POINT ( 'NONE',  ( -5.795997163829992083, 15.00000000000000000, -13.01802277140713926 ) ) ;
#63024=ORIENTED_EDGE ( 'NONE', *, *, #24016, .T. ) ;
#63025=CARTESIAN_POINT ( 'NONE',  ( -2.602060718268784267, 0.000000000000000000, -4.792399674598892823 ) ) ;
#63029=DIRECTION ( 'NONE',  ( 0.000000000000000000, 0.000000000000000000, -1.000000000000000000 ) ) ;
#63034=DIRECTION ( 'NONE',  ( 0.9099612708765483227, 0.000000000000000000, -0.4146932426562279228 ) ) ;
#63038=ORIENTED_EDGE ( 'NONE', *, *, #59238, .F. ) ;
#63040=VECTOR ( 'NONE', #79434, 1000.000000000000000 ) ;
#63044=ADVANCED_FACE ( 'NONE', ( #98352 ), #84832, .T. ) ;
#63047=CARTESIAN_POINT ( 'NONE',  ( 0.3093388210927670023, 14.63595249122790598, 14.99680997725066867 ) ) ;
#63051=TOROIDAL_SURFACE ( 'NONE', #55121, 14.49999999999999822, 0.5000000000000000000 ) ;
#63061=CARTESIAN_POINT ( 'NONE',  ( 2.915334737309928315, 4.522018677488174099, 10.88017736071109987 ) ) ;
#63077=ORIENTED_EDGE ( 'NONE', *, *, #27881, .T. ) ;
#63089=AXIS2_PLACEMENT_3D ( 'NONE', #21363, #43846, #13864 ) ;
#63090=EDGE_CURVE ( 'NONE', #26110, #65168, #22830, .T. ) ;
#63091=DIRECTION ( 'NONE',  ( -0.000000000000000000, -1.000000000000000000, -0.000000000000000000 ) ) ;
#63104=CARTESIAN_POINT ( 'NONE',  ( 12.07856007377828078, 4.686601975994315497E-16, -8.022367888854837759 ) ) ;
#63106=CARTESIAN_POINT ( 'NONE',  ( -4.923371831947302546, -14.82440218233254470, -8.527530157486173934 ) ) ;
#63107=EDGE_LOOP ( 'NONE', ( #84311, #87117, #31132, #96334 ) ) ;
#63111=DIRECTION ( 'NONE',  ( 0.000000000000000000, -0.7071067811865492381, -0.7071067811865457964 ) ) ;
#63119=LINE ( 'NONE', #41135, #81417 ) ;
#63123=VERTEX_POINT ( 'NONE', #66638 ) ;
#63125=ORIENTED_EDGE ( 'NONE', *, *, #87724, .F. ) ;
#63126=EDGE_CURVE ( 'NONE', #74503, #84500, #82622, .T. ) ;
#63128=ORIENTED_EDGE ( 'NONE', *, *, #13914, .F. ) ;
#63135=CARTESIAN_POINT ( 'NONE',  ( 0.3093388210927642268, 0.5000000000000004441, -14.99680997725065978 ) ) ;
#63145=EDGE_CURVE ( 'NONE', #78251, #34327, #23292, .T. ) ;
#63146=CARTESIAN_POINT ( 'NONE',  ( -1.780824192092290481, 0.3640475087720979608, -14.89391369643516860 ) ) ;
#63155=EDGE_CURVE ( 'NONE', #71998, #26702, #88030, .T. ) ;
#63162=CARTESIAN_POINT ( 'NONE',  ( 14.16722289976690163, 14.49999999999999112, -4.928467845925561974 ) ) ;
#63163=EDGE_CURVE ( 'NONE', #25279, #48910, #35642, .T. ) ;
#63165=FACE_OUTER_BOUND ( 'NONE', #45075, .T. ) ;
#63168=CARTESIAN_POINT ( 'NONE',  ( -3.795296366450300773, 32.84541550158063217, 14.16423886937410437 ) ) ;
#63179=VECTOR ( 'NONE', #88375, 1000.000000000000227 ) ;
#63186=DIRECTION ( 'NONE',  ( 0.8526401643540917341, 0.000000000000000000, -0.5224985647159496871 ) ) ;
#63193=CARTESIAN_POINT ( 'NONE',  ( 0.000000000000000000, 0.5000000000000004441, 0.000000000000000000 ) ) ;
#63206=VERTEX_POINT ( 'NONE', #65635 ) ;
#63209=CARTESIAN_POINT ( 'NONE',  ( 5.810202895580461657, 14.95077488074853456, -13.56051778013764242 ) ) ;
#63213=CARTESIAN_POINT ( 'NONE',  ( 3.836325488036175457, 14.49999999999999112, -14.50112432709429378 ) ) ;
#63216=DIRECTION ( 'NONE',  ( 0.000000000000000000, 1.000000000000000000, 0.000000000000000000 ) ) ;
#63225=ORIENTED_EDGE ( 'NONE', *, *, #29842, .F. ) ;
#63227=ORIENTED_EDGE ( 'NONE', *, *, #64993, .F. ) ;
#63231=VECTOR ( 'NONE', #41582, 1000.000000000000000 ) ;
#63235=CARTESIAN_POINT ( 'NONE',  ( 14.26139399674455710, 4.125707382711286748E-16, 2.619664342929903356 ) ) ;
#63236=VERTEX_POINT ( 'NONE', #80656 ) ;
#63239=CARTESIAN_POINT ( 'NONE',  ( 3.434112377981054287, -2.334698663402912100, -12.81628187352647608 ) ) ;
#63242=EDGE_CURVE ( 'NONE', #22706, #52000, #31573, .T. ) ;
#63246=LINE ( 'NONE', #16784, #25631 ) ;
#63249=CIRCLE ( 'NONE', #75971, 15.00000000000000000 ) ;
#63252=CARTESIAN_POINT ( 'NONE',  ( 2.393480905993088381, 14.49999999999999112, 14.80781041047758784 ) ) ;
#63253=AXIS2_PLACEMENT_3D ( 'NONE', #38199, #62142, #94622 ) ;
#63257=CARTESIAN_POINT ( 'NONE',  ( -6.138934250732154041, -0.03417435944610275333, 14.77128574976603481 ) ) ;
#63272=AXIS2_PLACEMENT_3D ( 'NONE', #56174, #78673, #93168 ) ;
#63274=VECTOR ( 'NONE', #30430, 999.9999999999998863 ) ;
#63275=FILL_AREA_STYLE ('',( #86290 ) ) ;
#63280=DIRECTION ( 'NONE',  ( -0.5075383629607084224, 0.000000000000000000, 0.8616291604415231564 ) ) ;
#63292=FACE_OUTER_BOUND ( 'NONE', #97027, .T. ) ;
#63296=CARTESIAN_POINT ( 'NONE',  ( 0.000000000000000000, 0.5000000000000004441, 0.000000000000000000 ) ) ;
#63299=CARTESIAN_POINT ( 'NONE',  ( 5.240416992896709480, 14.95077488074852390, 13.79072622793305136 ) ) ;
#63306=CARTESIAN_POINT ( 'NONE',  ( -13.78891971893217239, 14.49999999999999112, 5.904717858191482094 ) ) ;
#63315=CARTESIAN_POINT ( 'NONE',  ( 0.000000000000000000, 15.00000000000000000, 0.000000000000000000 ) ) ;
#63323=AXIS2_PLACEMENT_3D ( 'NONE', #12748, #50247, #13748 ) ;
#63331=ADVANCED_FACE ( 'NONE', ( #8113 ), #92581, .F. ) ;
#63333=EDGE_CURVE ( 'NONE', #29027, #53769, #76912, .T. ) ;
#63349=ORIENTED_EDGE ( 'NONE', *, *, #17550, .T. ) ;
#63350=VECTOR ( 'NONE', #8135, 1000.000000000000000 ) ;
#63352=AXIS2_PLACEMENT_3D ( 'NONE', #10057, #10542, #64013 ) ;
#63354=LINE ( 'NONE', #25386, #40866 ) ;
#63357=ADVANCED_FACE ( 'NONE', ( #44622 ), #75117, .F. ) ;
#63363=ADVANCED_FACE ( 'NONE', ( #15627 ), #48133, .F. ) ;
#63365=ORIENTED_EDGE ( 'NONE', *, *, #29563, .F. ) ;
#63369=CARTESIAN_POINT ( 'NONE',  ( -13.61912076658552095, 7.098136097991034869E-16, 5.334594295380809648 ) ) ;
#63377=VECTOR ( 'NONE', #60516, 1000.000000000000000 ) ;
#63380=CARTESIAN_POINT ( 'NONE',  ( 3.192513988408024694, -3.228466078459764559E-15, 14.27292421863752914 ) ) ;
#63386=CARTESIAN_POINT ( 'NONE',  ( -13.75543905097459429, 0.04962897369418823451, -5.333404663735767492 ) ) ;
#63394=ORIENTED_EDGE ( 'NONE', *, *, #80326, .F. ) ;
#63395=CARTESIAN_POINT ( 'NONE',  ( 13.40508947812165097, 15.00000000000000000, -5.527528931046084004 ) ) ;
#63413=CIRCLE ( 'NONE', #45885, 14.49999999999999822 ) ;
#63422=CARTESIAN_POINT ( 'NONE',  ( 14.16423886937410259, 4.303748834913974086, -2.602085213965210642E-15 ) ) ;
#63428=CARTESIAN_POINT ( 'NONE',  ( -10.82361996477964361, 14.95037106895822809, -10.02529603627149690 ) ) ;
#63434=DIRECTION ( 'NONE',  ( -0.000000000000000000, -1.000000000000000000, -0.000000000000000000 ) ) ;
#63450=B_SPLINE_CURVE_WITH_KNOTS ( 'NONE', 3,
 ( #26654, #57150, #87647, #19161, #13629, #91100 ),
 .UNSPECIFIED., .F., .F.,
 ( 4, 2, 4 ),
 ( 0.0002800020636817285172, 0.0006862073132860471540, 0.001092412562890365899 ),
 .UNSPECIFIED. ) ;
#63469=ORIENTED_EDGE ( 'NONE', *, *, #72914, .T. ) ;
#63474=AXIS2_PLACEMENT_3D ( 'NONE', #22272, #89269, #60737 ) ;
#63476=ORIENTED_EDGE ( 'NONE', *, *, #32507, .T. ) ;
#63479=CARTESIAN_POINT ( 'NONE',  ( 13.78891971893204271, 0.5000000000000004441, 5.904717858191622426 ) ) ;
#63487=EDGE_CURVE ( 'NONE', #96588, #30635, #82944, .T. ) ;
#63489=CARTESIAN_POINT ( 'NONE',  ( -7.208316651077756099, 26.63393115100079811, 7.208316651077766757 ) ) ;
#63490=ORIENTED_EDGE ( 'NONE', *, *, #36022, .T. ) ;
#63500=CARTESIAN_POINT ( 'NONE',  ( 0.000000000000000000, 0.5000000000000004441, 0.000000000000000000 ) ) ;
#63501=VECTOR ( 'NONE', #1523, 1000.000000000000114 ) ;
#63514=ORIENTED_EDGE ( 'NONE', *, *, #9622, .T. ) ;
#63515=CARTESIAN_POINT ( 'NONE',  ( 12.60589901313228189, 14.49999999999999112, -8.129656208642064286 ) ) ;
#63524=CARTESIAN_POINT ( 'NONE',  ( -14.24131928502211863, -0.03417435944610275333, 0.4973178280104966764 ) ) ;
#63527=VERTEX_POINT ( 'NONE', #52614 ) ;
#63531=EDGE_CURVE ( 'NONE', #55250, #55876, #83114, .T. ) ;
#63542=CARTESIAN_POINT ( 'NONE',  ( 9.065164099344530158, 0.5000000000000004441, -11.95084933600767307 ) ) ;
#63545=AXIS2_PLACEMENT_3D ( 'NONE', #73096, #88596, #29082 ) ;
#63548=CARTESIAN_POINT ( 'NONE',  ( -5.204170427930421283E-15, 6.813685344154843726, -10.88017736071110342 ) ) ;
#63553=DIRECTION ( 'NONE',  ( -0.000000000000000000, -1.000000000000000000, -0.000000000000000000 ) ) ;
#63557=DIRECTION ( 'NONE',  ( -0.000000000000000000, 1.000000000000000000, -0.000000000000000000 ) ) ;
#63558=ADVANCED_FACE ( 'NONE', ( #45106 ), #30593, .F. ) ;
#63561=EDGE_CURVE ( 'NONE', #72221, #13031, #76597, .T. ) ;
#63565=FACE_OUTER_BOUND ( 'NONE', #86063, .T. ) ;
#63577=DIRECTION ( 'NONE',  ( -0.000000000000000000, -1.000000000000000000, -0.000000000000000000 ) ) ;
#63579=CARTESIAN_POINT ( 'NONE',  ( -9.240973841163681257, 4.382479893023984083E-16, 11.17382667070366331 ) ) ;
#63580=FACE_OUTER_BOUND ( 'NONE', #21624, .T. ) ;
#63586=CARTESIAN_POINT ( 'NONE',  ( -14.82269085861176983, 14.49999999999999112, 2.299529454046846499 ) ) ;
#63595=CARTESIAN_POINT ( 'NONE',  ( 8.527530157486175710, -16.07440218233254470, -4.923371831947298993 ) ) ;
#63596=VERTEX_POINT ( 'NONE', #85089 ) ;
#63605=PLANE ( 'NONE',  #96596 ) ;
#63608=ORIENTED_EDGE ( 'NONE', *, *, #52821, .T. ) ;
#63619=AXIS2_PLACEMENT_3D ( 'NONE', #48592, #4593, #4100 ) ;
#63620=DIRECTION ( 'NONE',  ( 0.4924235601034769316, 0.000000000000000000, -0.8703556959398941473 ) ) ;
#63622=CARTESIAN_POINT ( 'NONE',  ( 0.000000000000000000, 14.49999999999999822, 0.000000000000000000 ) ) ;
#63623=ORIENTED_EDGE ( 'NONE', *, *, #22411, .F. ) ;
#63626=DIRECTION ( 'NONE',  ( -0.000000000000000000, -1.000000000000000000, -0.000000000000000000 ) ) ;
#63630=CARTESIAN_POINT ( 'NONE',  ( 8.209432707284774366, 0.5000000000000004441, 12.55409154915492032 ) ) ;
#63633=CARTESIAN_POINT ( 'NONE',  ( 12.03768810259479594, 15.00000000000000533, 8.306778944023417210 ) ) ;
#63635=CARTESIAN_POINT ( 'NONE',  ( 14.26328062697241705, 14.95037112300443560, 3.770429249334884325 ) ) ;
#63640=EDGE_CURVE ( 'NONE', #46092, #54024, #36365, .T. ) ;
#63651=CARTESIAN_POINT ( 'NONE',  ( -8.470640952597646489, -3.255147616298275020E-15, 11.92295067084760696 ) ) ;
#63654=AXIS2_PLACEMENT_3D ( 'NONE', #59132, #52139, #98666 ) ;
#63657=CARTESIAN_POINT ( 'NONE',  ( -5.204170427930421283E-15, -38.18631465584515183, -10.88017736071110342 ) ) ;
#63680=PLANE ( 'NONE',  #39781 ) ;
#63688=PLANE ( 'NONE',  #38384 ) ;
#63693=CARTESIAN_POINT ( 'NONE',  ( 8.209432707284781472, 14.63595249122790598, 12.55409154915492387 ) ) ;
#63696=FACE_OUTER_BOUND ( 'NONE', #47849, .T. ) ;
#63705=CARTESIAN_POINT ( 'NONE',  ( 10.97324858046202323, 2.151463686025922861E-16, -9.670892530813203436 ) ) ;
#63713=EDGE_CURVE ( 'NONE', #27622, #25275, #33541, .T. ) ;
#63714=ORIENTED_EDGE ( 'NONE', *, *, #60997, .T. ) ;
#63718=EDGE_LOOP ( 'NONE', ( #20427, #53401, #49847, #42522 ) ) ;
#63722=ADVANCED_FACE ( 'NONE', ( #40081 ), #94549, .T. ) ;
#63723=CIRCLE ( 'NONE', #54156, 14.49999999999999822 ) ;
#63726=CARTESIAN_POINT ( 'NONE',  ( 3.434112377981054287, -7.334698663402913432, -12.81628187352647608 ) ) ;
#63727=ORIENTED_EDGE ( 'NONE', *, *, #29511, .F. ) ;
#63731=VERTEX_POINT ( 'NONE', #9088 ) ;
#63741=CARTESIAN_POINT ( 'NONE',  ( -14.94699059465108881, 14.49999999999999112, 1.259949270174695268 ) ) ;
#63752=CARTESIAN_POINT ( 'NONE',  ( 7.674335239599196612, 0.2306972965111885598, 12.81961907869222372 ) ) ;
#63758=EDGE_CURVE ( 'NONE', #72571, #40524, #41801, .T. ) ;
#63761=CARTESIAN_POINT ( 'NONE',  ( -6.382347221874291598, 14.49999999999999112, -13.57444820018240783 ) ) ;
#63772=CARTESIAN_POINT ( 'NONE',  ( -5.817157072110619609, 0.3640475087720984049, -13.82608706751095085 ) ) ;
#63773=DIRECTION ( 'NONE',  ( 0.000000000000000000, 1.000000000000000000, 0.000000000000000000 ) ) ;
#63775=CIRCLE ( 'NONE', #68593, 14.49999999999999822 ) ;
#63778=DIRECTION ( 'NONE',  ( 0.3338068592337714025, 0.000000000000000000, 0.9426414910921783186 ) ) ;
#63783=FACE_OUTER_BOUND ( 'NONE', #66381, .T. ) ;
#63785=DIRECTION ( 'NONE',  ( 0.4771587602596153999, 0.000000000000000000, -0.8788171126619616080 ) ) ;
#63793=CARTESIAN_POINT ( 'NONE',  ( -3.927832320392065313, 15.00000000000000000, -13.69797916712109398 ) ) ;
#63799=VECTOR ( 'NONE', #56775, 1000.000000000000000 ) ;
#63823=ORIENTED_EDGE ( 'NONE', *, *, #33865, .F. ) ;
#63830=ORIENTED_EDGE ( 'NONE', *, *, #45259, .F. ) ;
#63853=CYLINDRICAL_SURFACE ( 'NONE', #27553, 15.00000000000000000 ) ;
#63857=ADVANCED_FACE ( 'NONE', ( #61001 ), #61983, .T. ) ;
#63858=VERTEX_POINT ( 'NONE', #22534 ) ;
#63869=CARTESIAN_POINT ( 'NONE',  ( 0.000000000000000000, 14.49999999999999822, 0.000000000000000000 ) ) ;
#63881=LINE ( 'NONE', #8928, #2992 ) ;
#63882=CARTESIAN_POINT ( 'NONE',  ( 8.470897558477602729, 15.00000000000000711, -11.92401951126078963 ) ) ;
#63891=ORIENTED_EDGE ( 'NONE', *, *, #14836, .T. ) ;
#63893=DIRECTION ( 'NONE',  ( 0.000000000000000000, 0.000000000000000000, 1.000000000000000000 ) ) ;
#63897=CARTESIAN_POINT ( 'NONE',  ( -14.16423886937410437, 6.595415501580630391, -3.795296366450299885 ) ) ;
#63911=EDGE_CURVE ( 'NONE', #37674, #32127, #13019, .T. ) ;
#63915=DIRECTION ( 'NONE',  ( -0.1993679344171901680, 0.000000000000000000, -0.9799247046208311440 ) ) ;
#63920=CARTESIAN_POINT ( 'NONE',  ( -0.7375392941516176748, 0.5000000000000004441, -14.98185688723471820 ) ) ;
#63931=ORIENTED_EDGE ( 'NONE', *, *, #25409, .T. ) ;
#63946=ORIENTED_EDGE ( 'NONE', *, *, #47541, .F. ) ;
#63952=DIRECTION ( 'NONE',  ( -0.000000000000000000, -1.000000000000000000, -0.000000000000000000 ) ) ;
#63960=CARTESIAN_POINT ( 'NONE',  ( 5.378451019861591575, 0.000000000000000000, 0.9000440264802798129 ) ) ;
#63962=CARTESIAN_POINT ( 'NONE',  ( -3.434112377981067610, -36.91803199673623936, -12.81628187352647252 ) ) ;
#63963=ORIENTED_EDGE ( 'NONE', *, *, #2981, .T. ) ;
#63980=CARTESIAN_POINT ( 'NONE',  ( 14.48718990079890112, 15.00000000000000000, -0.6093675230840328583 ) ) ;
#63992=VERTEX_POINT ( 'NONE', #87949 ) ;
#63993=ADVANCED_FACE ( 'NONE', ( #34942 ), #44418, .F. ) ;
#63999=ADVANCED_FACE ( 'NONE', ( #5461 ), #42954, .F. ) ;
#64010=AXIS2_PLACEMENT_3D ( 'NONE', #19045, #25087, #3075 ) ;
#64013=DIRECTION ( 'NONE',  ( 0.000000000000000000, 0.000000000000000000, 1.000000000000000000 ) ) ;
#64016=CARTESIAN_POINT ( 'NONE',  ( -14.16423886937410082, -38.19625116508603213, 4.336808689942017736E-15 ) ) ;
#64028=EDGE_CURVE ( 'NONE', #14809, #97109, #78549, .T. ) ;
#64032=CARTESIAN_POINT ( 'NONE',  ( 10.88017736071110519, 10.56368534415484639, -2.602085213965210642E-15 ) ) ;
#64034=CARTESIAN_POINT ( 'NONE',  ( -13.48255862861931043, 15.00000000000000000, 5.335786055104065895 ) ) ;
#64035=CARTESIAN_POINT ( 'NONE',  ( 14.99847009497944406, 15.00000000000000000, 0.2142307401081381124 ) ) ;
#64037=EDGE_CURVE ( 'NONE', #98896, #16073, #91315, .T. ) ;
#64042=DIRECTION ( 'NONE',  ( -0.000000000000000000, -1.000000000000000000, -0.000000000000000000 ) ) ;
#64049=CIRCLE ( 'NONE', #28936, 15.00000000000000000 ) ;
#64051=ORIENTED_EDGE ( 'NONE', *, *, #90552, .T. ) ;
#64060=CARTESIAN_POINT ( 'NONE',  ( -8.564643372776465924, 14.49999999999999112, -12.31449893000758955 ) ) ;
#64063=ORIENTED_EDGE ( 'NONE', *, *, #98651, .T. ) ;
#64069=CARTESIAN_POINT ( 'NONE',  ( 7.771322705631394712, 15.00000000000000000, 12.24159072199921283 ) ) ;
#64070=CARTESIAN_POINT ( 'NONE',  ( 0.9940297508536876103, 0.000000000000000000, 14.21528771620250353 ) ) ;
#64076=CARTESIAN_POINT ( 'NONE',  ( 7.208316651077762316, -0.8660688489992137695, -7.208316651077764980 ) ) ;
#64088=CARTESIAN_POINT ( 'NONE',  ( -3.166711953933234014, 0.000000000000000000, 4.439566422914446697 ) ) ;
#64089=VECTOR ( 'NONE', #91839, 1000.000000000000000 ) ;
#64091=CARTESIAN_POINT ( 'NONE',  ( -14.09394518620605297, 15.00000000000000000, -3.407449058785551710 ) ) ;
#64094=ORIENTED_EDGE ( 'NONE', *, *, #19983, .F. ) ;
#64096=ORIENTED_EDGE ( 'NONE', *, *, #46564, .T. ) ;
#64103=CARTESIAN_POINT ( 'NONE',  ( -13.21236992757665973, 15.00000000000000000, -5.338143956176898186 ) ) ;
#64104=AXIS2_PLACEMENT_3D ( 'NONE', #37929, #37435, #76402 ) ;
#64105=ADVANCED_FACE ( 'NONE', ( #20947 ), #30573, .T. ) ;
#64116=DIRECTION ( 'NONE',  ( 0.9799247046208269252, 0.000000000000000000, 0.1993679344172108736 ) ) ;
#64121=VERTEX_POINT ( 'NONE', #42465 ) ;
#64122=DIRECTION ( 'NONE',  ( 0.000000000000000000, 0.000000000000000000, 1.000000000000000000 ) ) ;
#64130=ADVANCED_FACE ( 'NONE', ( #72946 ), #25809, .T. ) ;
#64131=EDGE_LOOP ( 'NONE', ( #27919, #52293, #59101, #94532 ) ) ;
#64133=DIRECTION ( 'NONE',  ( 0.000000000000000000, 1.000000000000000000, 0.000000000000000000 ) ) ;
#64136=LINE ( 'NONE', #5638, #52912 ) ;
#64137=CARTESIAN_POINT ( 'NONE',  ( 10.82361996477978217, 0.04962893104176950565, -10.02529603627134236 ) ) ;
#64138=EDGE_CURVE ( 'NONE', #46976, #1757, #30395, .T. ) ;
#64142=B_SPLINE_CURVE_WITH_KNOTS ( 'NONE', 3,
 ( #11241, #70784, #9282, #24303, #94742, #63741 ),
 .UNSPECIFIED., .F., .F.,
 ( 4, 2, 4 ),
 ( 0.0002800098398967154449, 0.0006862151655623427004, 0.001092420491227969956 ),
 .UNSPECIFIED. ) ;
#64143=CARTESIAN_POINT ( 'NONE',  ( -3.795296366450322534, 30.76208216824731423, -14.16423886937409904 ) ) ;
#64165=EDGE_LOOP ( 'NONE', ( #66660, #35479, #87209, #18216 ) ) ;
#64175=ORIENTED_EDGE ( 'NONE', *, *, #31140, .T. ) ;
#64177=VECTOR ( 'NONE', #75689, 999.9999999999998863 ) ;
#64178=CARTESIAN_POINT ( 'NONE',  ( -4.856044144387521300, 2.253107639696438902E-16, -13.79699902221167918 ) ) ;
#64180=VERTEX_POINT ( 'NONE', #91398 ) ;
#64184=B_SPLINE_CURVE_WITH_KNOTS ( 'NONE', 3,
 ( #87355, #56855, #42356, #4369, #96356, #18869, #34834, #72831 ),
 .UNSPECIFIED., .F., .F.,
 ( 4, 2, 2, 4 ),
 ( 2.665285624635612776E-17, 0.003056699928650253879, 0.004585049892975365422, 0.006113399857300476532 ),
 .UNSPECIFIED. ) ;
#64195=CARTESIAN_POINT ( 'NONE',  ( 0.8649609010933267950, 15.00000000000000178, -14.60103384664011195 ) ) ;
#64197=CIRCLE ( 'NONE', #21101, 11.25000000000000178 ) ;
#64200=ORIENTED_EDGE ( 'NONE', *, *, #73608, .T. ) ;
#64202=AXIS2_PLACEMENT_3D ( 'NONE', #27882, #37383, #66876 ) ;
#64209=EDGE_CURVE ( 'NONE', #55079, #10597, #37204, .T. ) ;
#64212=CARTESIAN_POINT ( 'NONE',  ( -3.434112377981067610, -6.918031996736242917, -12.81628187352647252 ) ) ;
#64215=ORIENTED_EDGE ( 'NONE', *, *, #62079, .T. ) ;
#64216=ORIENTED_EDGE ( 'NONE', *, *, #11405, .T. ) ;
#64229=CYLINDRICAL_SURFACE ( 'NONE', #62054, 11.92686044187656513 ) ;
#64238=FACE_OUTER_BOUND ( 'NONE', #51439, .T. ) ;
#64242=LINE ( 'NONE', #18279, #8813 ) ;
#64262=VECTOR ( 'NONE', #5286, 999.9999999999998863 ) ;
#64274=CARTESIAN_POINT ( 'NONE',  ( 13.55255535720591986, 0.000000000000000000, 4.403492169843056914 ) ) ;
#64290=FACE_OUTER_BOUND ( 'NONE', #3750, .T. ) ;
#64292=CARTESIAN_POINT ( 'NONE',  ( -14.09394518620614711, 4.304378373471060795E-16, 3.407449058785263940 ) ) ;
#64294=CARTESIAN_POINT ( 'NONE',  ( -14.52941021839284907, 15.00000000000000888, 1.683622718072942170 ) ) ;
#64300=CIRCLE ( 'NONE', #48395, 15.00000000000000000 ) ;
#64318=ORIENTED_EDGE ( 'NONE', *, *, #85385, .T. ) ;
#64319=CARTESIAN_POINT ( 'NONE',  ( 13.34989199099680413, 14.95037102702803544, -6.279943681065447869 ) ) ;
#64322=EDGE_LOOP ( 'NONE', ( #12571, #20545, #30290, #53554 ) ) ;
#64325=CARTESIAN_POINT ( 'NONE',  ( 14.43063482171895373, -2.066760391300490855E-16, -2.386446184883025179 ) ) ;
#64326=DIRECTION ( 'NONE',  ( -0.000000000000000000, -1.000000000000000000, -0.000000000000000000 ) ) ;
#64332=VECTOR ( 'NONE', #95899, 1000.000000000000000 ) ;
#64337=ORIENTED_EDGE ( 'NONE', *, *, #73815, .T. ) ;
#64354=EDGE_CURVE ( 'NONE', #92170, #55079, #61878, .T. ) ;
#64362=CARTESIAN_POINT ( 'NONE',  ( -4.326345305608602310, 0.000000000000000000, -3.319721512309643074 ) ) ;
#64369=ORIENTED_EDGE ( 'NONE', *, *, #34526, .T. ) ;
#64370=AXIS2_PLACEMENT_3D ( 'NONE', #9161, #32641, #19977 ) ;
#64371=LINE ( 'NONE', #17429, #66108 ) ;
#64374=LINE ( 'NONE', #2443, #88813 ) ;
#64384=LINE ( 'NONE', #87396, #16612 ) ;
#64388=EDGE_CURVE ( 'NONE', #50974, #8774, #73750, .T. ) ;
#64391=CARTESIAN_POINT ( 'NONE',  ( 3.469446951953614189E-15, 8.053748834913978527, 14.16423886937410259 ) ) ;
#64394=ORIENTED_EDGE ( 'NONE', *, *, #27801, .T. ) ;
#64397=CARTESIAN_POINT ( 'NONE',  ( -14.48718990079890290, 15.00000000000000000, 0.6093675230839377122 ) ) ;
#64399=CARTESIAN_POINT ( 'NONE',  ( -10.76445796112971109, 15.00000000000000711, -9.901260316209995693 ) ) ;
#64401=AXIS2_PLACEMENT_3D ( 'NONE', #9404, #70903, #74707 ) ;
#64412=DIRECTION ( 'NONE',  ( -3.286260152890462729E-14, 0.000000000000000000, 1.000000000000000000 ) ) ;
#64427=ORIENTED_EDGE ( 'NONE', *, *, #96753, .T. ) ;
#64428=B_SPLINE_CURVE_WITH_KNOTS ( 'NONE', 3,
 ( #50792, #10829, #81283, #35781, #86826, #94311 ),
 .UNSPECIFIED., .F., .F.,
 ( 4, 2, 4 ),
 ( 0.0002800086601589242097, 0.0006862139742844824888, 0.001092419288410040931 ),
 .UNSPECIFIED. ) ;
#64453=CARTESIAN_POINT ( 'NONE',  ( -3.927832320392065313, 15.00000000000000000, -13.69797916712109398 ) ) ;
#64456=CARTESIAN_POINT ( 'NONE',  ( 11.09922568453595026, -28.79303199673624292, 6.408140936763232709 ) ) ;
#64457=ORIENTED_EDGE ( 'NONE', *, *, #2547, .T. ) ;
#64458=B_SPLINE_CURVE_WITH_KNOTS ( 'NONE', 3,
 ( #32898, #78402, #9921, #85919, #57369, #63395 ),
 .UNSPECIFIED., .F., .F.,
 ( 4, 2, 4 ),
 ( 3.409110551475976050E-05, 0.0004400426677365986252, 0.0008459942299584374695 ),
 .UNSPECIFIED. ) ;
#64467=CARTESIAN_POINT ( 'NONE',  ( -14.97687855664607781, 0.3640475087720984604, -0.8325315005902566012 ) ) ;
#64481=( NAMED_UNIT ( * ) PLANE_ANGLE_UNIT ( ) SI_UNIT ( $, .RADIAN. ) );
#64485=DIRECTION ( 'NONE',  ( 0.000000000000000000, 0.000000000000000000, 1.000000000000000000 ) ) ;
#64488=EDGE_LOOP ( 'NONE', ( #51306, #24487, #38543, #35287 ) ) ;
#64505=CARTESIAN_POINT ( 'NONE',  ( 11.48952521350024192, 4.570664323179305100E-16, -8.845383562533745803 ) ) ;
#64509=CARTESIAN_POINT ( 'NONE',  ( -12.26659068614895354, -38.61291783175269643, -7.082119434687038861 ) ) ;
#64512=EDGE_LOOP ( 'NONE', ( #2280, #66813, #12889, #57478 ) ) ;
#64518=DIRECTION ( 'NONE',  ( -0.04361938736532633420, 0.000000000000000000, -0.9990482215818581313 ) ) ;
#64519=DIRECTION ( 'NONE',  ( 0.000000000000000000, 0.000000000000000000, -1.000000000000000000 ) ) ;
#64525=CARTESIAN_POINT ( 'NONE',  ( 7.964842623401181321, 14.93868534415484106, 7.964842623401174215 ) ) ;
#64528=CARTESIAN_POINT ( 'NONE',  ( 0.000000000000000000, 14.49999999999999822, 0.000000000000000000 ) ) ;
#64537=CARTESIAN_POINT ( 'NONE',  ( -8.838651438279397254, 14.95077488074853456, -11.81204219878349804 ) ) ;
#64552=CARTESIAN_POINT ( 'NONE',  ( -14.47650479471822393, 14.49999999999999112, -3.928206833722243108 ) ) ;
#64560=PLANE ( 'NONE',  #31559 ) ;
#64564=EDGE_CURVE ( 'NONE', #41967, #23012, #17887, .T. ) ;
#64565=EDGE_CURVE ( 'NONE', #77740, #43585, #96236, .T. ) ;
#64566=CARTESIAN_POINT ( 'NONE',  ( -13.21236992757677164, -0.03417435944610275333, 5.338143956176621074 ) ) ;
#64568=CARTESIAN_POINT ( 'NONE',  ( -9.846743663894594434, 6.008931151000790116, 3.469446951953614189E-15 ) ) ;
#64572=ORIENTED_EDGE ( 'NONE', *, *, #24511, .T. ) ;
#64579=DIRECTION ( 'NONE',  ( -0.000000000000000000, -1.000000000000000000, -0.000000000000000000 ) ) ;
#64582=ORIENTED_EDGE ( 'NONE', *, *, #94836, .T. ) ;
#64585=EDGE_CURVE ( 'NONE', #33221, #90159, #50214, .T. ) ;
#64591=CARTESIAN_POINT ( 'NONE',  ( 13.64884605730314426, 15.00000000000000000, -8.341846182955777067 ) ) ;
#64598=CIRCLE ( 'NONE', #59832, 14.49999999999999822 ) ;
#64601=CIRCLE ( 'NONE', #21536, 15.00000000000000000 ) ;
#64602=LINE ( 'NONE', #87613, #1219 ) ;
#64603=ORIENTED_EDGE ( 'NONE', *, *, #84233, .T. ) ;
#64608=DIRECTION ( 'NONE',  ( 0.000000000000000000, 1.000000000000000000, 0.000000000000000000 ) ) ;
#64609=EDGE_LOOP ( 'NONE', ( #50309, #39455, #62811, #62864, #58358, #23581 ) ) ;
#64610=DIRECTION ( 'NONE',  ( -0.000000000000000000, -1.000000000000000000, -0.000000000000000000 ) ) ;
#64625=CARTESIAN_POINT ( 'NONE',  ( -14.82269085861172364, 14.49999999999999112, -2.299529454047143595 ) ) ;
#64626=PLANE ( 'NONE',  #42163 ) ;
#64630=CARTESIAN_POINT ( 'NONE',  ( 2.915334737309921209, -18.39464798917849109, -10.88017736071110164 ) ) ;
#64634=CARTESIAN_POINT ( 'NONE',  ( 8.439016546559821919, 3.791394052158136007E-16, 11.79122553964979048 ) ) ;
#64635=CARTESIAN_POINT ( 'NONE',  ( -6.767445849361066301, 0.5000000000000004441, -13.38662304974505801 ) ) ;
#64647=CARTESIAN_POINT ( 'NONE',  ( -14.94699059465099822, 14.49999999999999822, -1.259949270175015013 ) ) ;
#64661=ADVANCED_FACE ( 'NONE', ( #79744 ), #88166, .T. ) ;
#64663=CARTESIAN_POINT ( 'NONE',  ( -4.850115630859501259, 0.04922511925147174394, -13.93278430610814844 ) ) ;
#64665=VERTEX_POINT ( 'NONE', #58709 ) ;
#64685=CARTESIAN_POINT ( 'NONE',  ( -8.527530157486173934, -33.57440218233254114, 4.923371831947302546 ) ) ;
#64686=ORIENTED_EDGE ( 'NONE', *, *, #16941, .F. ) ;
#64690=ORIENTED_EDGE ( 'NONE', *, *, #73384, .T. ) ;
#64697=CARTESIAN_POINT ( 'NONE',  ( -9.382169495545413795, 14.74863466993041961, 9.382169495545428006 ) ) ;
#64698=ORIENTED_EDGE ( 'NONE', *, *, #54443, .F. ) ;
#64702=EDGE_CURVE ( 'NONE', #86853, #27481, #81216, .T. ) ;
#64703=VERTEX_POINT ( 'NONE', #28704 ) ;
#64711=ADVANCED_FACE ( 'NONE', ( #97236 ), #81699, .F. ) ;
#64714=LINE ( 'NONE', #41276, #47874 ) ;
#64717=FACE_OUTER_BOUND ( 'NONE', #24187, .T. ) ;
#64720=CYLINDRICAL_SURFACE ( 'NONE', #83485, 15.00000000000000000 ) ;
#64730=CARTESIAN_POINT ( 'NONE',  ( 9.159723438033129383, -0.03417435944610275333, 10.91613331444548507 ) ) ;
#64741=ORIENTED_EDGE ( 'NONE', *, *, #13305, .T. ) ;
#64755=CARTESIAN_POINT ( 'NONE',  ( 12.58848565468353797, 2.439454888092384977E-16, 7.447709424579961990 ) ) ;
#64760=ORIENTED_EDGE ( 'NONE', *, *, #68889, .F. ) ;
#64761=CIRCLE ( 'NONE', #85565, 15.00000000000000000 ) ;
#64764=DIRECTION ( 'NONE',  ( -0.000000000000000000, -1.000000000000000000, -0.000000000000000000 ) ) ;
#64778=DIRECTION ( 'NONE',  ( -0.7372773368101340763, -0.000000000000000000, 0.6755902076156493630 ) ) ;
#64784=AXIS2_PLACEMENT_3D ( 'NONE', #96767, #65240, #95765 ) ;
#64785=EDGE_CURVE ( 'NONE', #81069, #77887, #90189, .T. ) ;
#64787=FACE_OUTER_BOUND ( 'NONE', #2158, .T. ) ;
#64806=CYLINDRICAL_SURFACE ( 'NONE', #80917, 15.00000000000000000 ) ;
#64814=CARTESIAN_POINT ( 'NONE',  ( 14.76044511231853207, 14.76984987354014400, -2.313329003772379266 ) ) ;
#64825=CARTESIAN_POINT ( 'NONE',  ( -10.58171042697161646, 0.2301503269722709466, -10.54749450092416296 ) ) ;
#64830=CARTESIAN_POINT ( 'NONE',  ( -14.02068044289371684, 14.49999999999999822, -5.331089937175857330 ) ) ;
#64840=ORIENTED_EDGE ( 'NONE', *, *, #15283, .F. ) ;
#64886=VERTEX_POINT ( 'NONE', #52689 ) ;
#64892=FACE_OUTER_BOUND ( 'NONE', #64609, .T. ) ;
#64900=VECTOR ( 'NONE', #10363, 1000.000000000000000 ) ;
#64906=EDGE_CURVE ( 'NONE', #79719, #46092, #96182, .T. ) ;
#64913=ORIENTED_EDGE ( 'NONE', *, *, #2248, .T. ) ;
#64914=CARTESIAN_POINT ( 'NONE',  ( -12.25993886608611660, 15.00000000000000000, 8.642563219313529999 ) ) ;
#64929=CARTESIAN_POINT ( 'NONE',  ( 0.000000000000000000, 0.5000000000000004441, 0.000000000000000000 ) ) ;
#64933=CARTESIAN_POINT ( 'NONE',  ( -14.40939250469963895, 4.354406223596783273E-16, -1.618458416365949226 ) ) ;
#64939=CARTESIAN_POINT ( 'NONE',  ( -11.22915323889568562, 0.000000000000000000, -8.773176023390764300 ) ) ;
#64943=CARTESIAN_POINT ( 'NONE',  ( 11.09922568453594671, -27.95969866340291077, -6.408140936763241591 ) ) ;
#64944=ADVANCED_FACE ( 'NONE', ( #89700 ), #9969, .T. ) ;
#64952=EDGE_CURVE ( 'NONE', #39344, #94453, #48272, .T. ) ;
#64956=ORIENTED_EDGE ( 'NONE', *, *, #51299, .T. ) ;
#64960=DIRECTION ( 'NONE',  ( -0.8141155183563226760, 0.000000000000000000, 0.5807029557109348872 ) ) ;
#64961=EDGE_CURVE ( 'NONE', #1475, #20937, #37222, .T. ) ;
#64975=CARTESIAN_POINT ( 'NONE',  ( -8.838651438279651273, 0.04922511925147145251, 11.81204219878332751 ) ) ;
#64977=ORIENTED_EDGE ( 'NONE', *, *, #17906, .T. ) ;
#64981=DIRECTION ( 'NONE',  ( 0.000000000000000000, 0.000000000000000000, 1.000000000000000000 ) ) ;
#64993=EDGE_CURVE ( 'NONE', #20387, #42602, #29680, .T. ) ;
#64995=CARTESIAN_POINT ( 'NONE',  ( 3.469446951953614189E-15, -31.94625116508602858, 14.16423886937410259 ) ) ;
#65000=EDGE_CURVE ( 'NONE', #29785, #25526, #14716, .T. ) ;
#65011=CARTESIAN_POINT ( 'NONE',  ( -2.915334737309917656, 19.10535201082151247, 10.88017736071110164 ) ) ;
#65016=CARTESIAN_POINT ( 'NONE',  ( 14.88232117145529720, 0.5000000000000004441, 1.875237731503240024 ) ) ;
#65019=DIRECTION ( 'NONE',  ( 0.000000000000000000, 0.000000000000000000, 1.000000000000000000 ) ) ;
#65020=EDGE_CURVE ( 'NONE', #88318, #7347, #60983, .T. ) ;
#65032=CARTESIAN_POINT ( 'NONE',  ( 0.000000000000000000, 0.000000000000000000, 0.000000000000000000 ) ) ;
#65035=VECTOR ( 'NONE', #62518, 1000.000000000000000 ) ;
#65039=CARTESIAN_POINT ( 'NONE',  ( 13.34343830728408697, 14.49999999999999112, -6.852200678592647698 ) ) ;
#65041=AXIS2_PLACEMENT_3D ( 'NONE', #83844, #38356, #382 ) ;
#65043=CARTESIAN_POINT ( 'NONE',  ( -9.281709892946549800, -3.133174871893655771E-15, 11.30302492080699928 ) ) ;
#65046=VERTEX_POINT ( 'NONE', #87130 ) ;
#65051=DIRECTION ( 'NONE',  ( 0.3665012267242946375, 0.000000000000000000, 0.9304175679820254619 ) ) ;
#65058=CARTESIAN_POINT ( 'NONE',  ( -8.527530157486173934, -3.574402182332542033, 4.923371831947302546 ) ) ;
#65059=VERTEX_POINT ( 'NONE', #86658 ) ;
#65062=ORIENTED_EDGE ( 'NONE', *, *, #36054, .F. ) ;
#65076=VERTEX_POINT ( 'NONE', #56166 ) ;
#65081=AXIS2_PLACEMENT_3D ( 'NONE', #60700, #52710, #21235 ) ;
#65085=CARTESIAN_POINT ( 'NONE',  ( 1.354709868695515684, 0.5000000000000004441, 14.93870011653152652 ) ) ;
#65088=ORIENTED_EDGE ( 'NONE', *, *, #52392, .T. ) ;
#65100=CARTESIAN_POINT ( 'NONE',  ( -1.354709868695410657, 14.49999999999999822, -14.93870011653153718 ) ) ;
#65101=LINE ( 'NONE', #97621, #78568 ) ;
#65110=VECTOR ( 'NONE', #4045, 1000.000000000000000 ) ;
#65117=EDGE_CURVE ( 'NONE', #1561, #22307, #88350, .T. ) ;
#65118=EDGE_CURVE ( 'NONE', #23568, #88606, #7262, .T. ) ;
#65119=ORIENTED_EDGE ( 'NONE', *, *, #29798, .T. ) ;
#65131=CARTESIAN_POINT ( 'NONE',  ( 10.88017736071109987, -24.22798132251182324, -2.915334737309928315 ) ) ;
#65136=LINE ( 'NONE', #66126, #67607 ) ;
#65143=ADVANCED_FACE ( 'NONE', ( #97135 ), #51109, .F. ) ;
#65147=CARTESIAN_POINT ( 'NONE',  ( -14.94699059465100355, 14.63595249122795394, -1.259949270175012570 ) ) ;
#65152=EDGE_LOOP ( 'NONE', ( #45328, #69090, #66950, #59294 ) ) ;
#65153=EDGE_CURVE ( 'NONE', #33705, #18498, #28605, .T. ) ;
#65158=LINE ( 'NONE', #95676, #44569 ) ;
#65165=AXIS2_PLACEMENT_3D ( 'NONE', #3007, #19460, #2522 ) ;
#65168=VERTEX_POINT ( 'NONE', #20115 ) ;
#65183=CARTESIAN_POINT ( 'NONE',  ( 2.638427012816835227, -37.53273551566588395, 9.846743663894590881 ) ) ;
#65185=DIRECTION ( 'NONE',  ( 0.000000000000000000, 0.000000000000000000, -1.000000000000000000 ) ) ;
#65193=CARTESIAN_POINT ( 'NONE',  ( 9.399392868737814766, 4.153235915537064750E-16, -11.04089732309474314 ) ) ;
#65196=CARTESIAN_POINT ( 'NONE',  ( -5.204170427930421283E-15, 12.87363466993042493, -12.81628187352647608 ) ) ;
#65200=ORIENTED_EDGE ( 'NONE', *, *, #1567, .F. ) ;
#65210=EDGE_CURVE ( 'NONE', #43044, #94701, #13108, .T. ) ;
#65211=DIRECTION ( 'NONE',  ( 0.3007057995042701770, 0.000000000000000000, 0.9537169507482278208 ) ) ;
#65213=CARTESIAN_POINT ( 'NONE',  ( -9.383795276901610194, 0.2306972965111761253, -11.62679839395705272 ) ) ;
#65214=FACE_OUTER_BOUND ( 'NONE', #42887, .T. ) ;
#65225=ADVANCED_FACE ( 'NONE', ( #36615 ), #48348, .T. ) ;
#65227=CARTESIAN_POINT ( 'NONE',  ( -10.76493118081678091, 2.303929616531696922E-16, -9.902252441915882386 ) ) ;
#65235=ADVANCED_FACE ( 'NONE', ( #6596 ), #89107, .F. ) ;
#65236=CARTESIAN_POINT ( 'NONE',  ( -9.742785792574931492, 3.338468844518207579, 5.625000000000008882 ) ) ;
#65240=DIRECTION ( 'NONE',  ( 0.000000000000000000, 1.000000000000000000, 0.000000000000000000 ) ) ;
#65249=LINE ( 'NONE', #95777, #36984 ) ;
#65251=CIRCLE ( 'NONE', #70071, 14.49999999999999822 ) ;
#65254=DIRECTION ( 'NONE',  ( 0.8038568606172245001, 0.000000000000000000, -0.5948227867513318223 ) ) ;
#65266=EDGE_CURVE ( 'NONE', #24761, #62099, #35577, .T. ) ;
#65273=LINE ( 'NONE', #88287, #17631 ) ;
#65274=CARTESIAN_POINT ( 'NONE',  ( -4.873787042390612001, -0.03417435944610275333, -13.39061984619925916 ) ) ;
#65284=VERTEX_POINT ( 'NONE', #83088 ) ;
#65286=LINE ( 'NONE', #26808, #49219 ) ;
#65298=CIRCLE ( 'NONE', #81223, 15.00000000000000000 ) ;
#65305=LINE ( 'NONE', #94831, #30646 ) ;
#65317=ORIENTED_EDGE ( 'NONE', *, *, #73608, .F. ) ;
#65324=CARTESIAN_POINT ( 'NONE',  ( 0.000000000000000000, 0.000000000000000000, 0.000000000000000000 ) ) ;
#65327=DIRECTION ( 'NONE',  ( -0.000000000000000000, -1.000000000000000000, -0.000000000000000000 ) ) ;
#65334=CARTESIAN_POINT ( 'NONE',  ( -7.993154516101138363, 0.04922511925147102924, 12.39982181464608679 ) ) ;
#65339=VERTEX_POINT ( 'NONE', #63920 ) ;
#65346=CARTESIAN_POINT ( 'NONE',  ( 11.29168986245492157, 0.2301502372707088795, 9.783658503027474751 ) ) ;
#65347=CARTESIAN_POINT ( 'NONE',  ( -12.74414838903266123, 15.00000000000000888, -7.178093659842149421 ) ) ;
#65364=CARTESIAN_POINT ( 'NONE',  ( 12.83294900548068007, 14.49999999999999112, -7.766300266068417280 ) ) ;
#65369=CARTESIAN_POINT ( 'NONE',  ( 7.640985187756951014, 14.95037103177511284, 12.62032702734131995 ) ) ;
#65382=EDGE_CURVE ( 'NONE', #7455, #61223, #28404, .T. ) ;
#65390=DIRECTION ( 'NONE',  ( 0.000000000000000000, 1.000000000000000000, 0.000000000000000000 ) ) ;
#65391=ORIENTED_EDGE ( 'NONE', *, *, #26557, .T. ) ;
#65396=CARTESIAN_POINT ( 'NONE',  ( -8.375939845167600595, 15.00000000000000000, -11.52849216984310310 ) ) ;
#65398=DIRECTION ( 'NONE',  ( -0.000000000000000000, -1.000000000000000000, -0.000000000000000000 ) ) ;
#65406=B_SPLINE_CURVE_WITH_KNOTS ( 'NONE', 3,
 ( #95686, #63693, #57179, #58152, #33198, #34670 ),
 .UNSPECIFIED., .F., .F.,
 ( 4, 2, 4 ),
 ( 3.409110551496207262E-05, 0.0004400426677368006120, 0.0008459942299586391311 ),
 .UNSPECIFIED. ) ;
#65414=ORIENTED_EDGE ( 'NONE', *, *, #84910, .T. ) ;
#65416=DIRECTION ( 'NONE',  ( 0.9799247046208295897, 0.000000000000000000, -0.1993679344171971901 ) ) ;
#65421=AXIS2_PLACEMENT_3D ( 'NONE', #97912, #31342, #84376 ) ;
#65424=EDGE_LOOP ( 'NONE', ( #70513, #36827, #64318, #66059, #97433, #50355 ) ) ;
#65440=DIRECTION ( 'NONE',  ( 0.9762960071199360268, 0.000000000000000000, -0.2164396139380906636 ) ) ;
#65445=CARTESIAN_POINT ( 'NONE',  ( 9.382169495545415572, -37.75136533006957507, -9.382169495545422677 ) ) ;
#65446=VECTOR ( 'NONE', #38348, 1000.000000000000000 ) ;
#65453=ADVANCED_FACE ( 'NONE', ( #73398 ), #27901, .F. ) ;
#65454=DIRECTION ( 'NONE',  ( 0.000000000000000000, 1.000000000000000000, 0.000000000000000000 ) ) ;
#65456=ORIENTED_EDGE ( 'NONE', *, *, #62079, .F. ) ;
#65470=B_SPLINE_CURVE_WITH_KNOTS ( 'NONE', 3,
 ( #73501, #95024, #42528, #27023, #4052, #73012 ),
 .UNSPECIFIED., .F., .F.,
 ( 4, 2, 4 ),
 ( 0.0002800313526871184180, 0.0006862368888281838043, 0.001092442424969249353 ),
 .UNSPECIFIED. ) ;
#65488=CARTESIAN_POINT ( 'NONE',  ( -14.24131928502211863, -0.03417435944610275333, 0.4973178280104966764 ) ) ;
#65494=CIRCLE ( 'NONE', #6480, 14.49999999999999822 ) ;
#65495=ORIENTED_EDGE ( 'NONE', *, *, #66158, .T. ) ;
#65500=CARTESIAN_POINT ( 'NONE',  ( -12.26659068614895354, -33.61291783175269643, -7.082119434687038861 ) ) ;
#65504=B_SPLINE_CURVE_WITH_KNOTS ( 'NONE', 3,
 ( #13627, #84107, #141, #60603, #91098, #8110 ),
 .UNSPECIFIED., .F., .F.,
 ( 4, 2, 4 ),
 ( 0.0002800912045164337893, 0.0006862973266905198974, 0.001092503448864605951 ),
 .UNSPECIFIED. ) ;
#65514=CARTESIAN_POINT ( 'NONE',  ( 2.915334737309921209, 21.60535201082150536, -10.88017736071110164 ) ) ;
#65531=ORIENTED_EDGE ( 'NONE', *, *, #95205, .F. ) ;
#65541=CARTESIAN_POINT ( 'NONE',  ( -8.439016546561676435, 15.00000000000000000, -11.79122553965791553 ) ) ;
#65544=AXIS2_PLACEMENT_3D ( 'NONE', #32064, #70092, #56076 ) ;
#65545=ORIENTED_EDGE ( 'NONE', *, *, #29591, .T. ) ;
#65551=CARTESIAN_POINT ( 'NONE',  ( 3.822225673302274362, 0.000000000000000000, -3.889525102760237552 ) ) ;
#65553=CARTESIAN_POINT ( 'NONE',  ( 10.09792486685190482, 0.04962894416274275106, -10.75589247084411859 ) ) ;
#65558=CARTESIAN_POINT ( 'NONE',  ( -4.923371831947302546, 0.1755978176674541369, -8.527530157486173934 ) ) ;
#65560=FACE_OUTER_BOUND ( 'NONE', #17890, .T. ) ;
#65562=VERTEX_POINT ( 'NONE', #80915 ) ;
#65569=EDGE_CURVE ( 'NONE', #40063, #53280, #42428, .T. ) ;
#65577=EDGE_LOOP ( 'NONE', ( #2650, #87554, #65849, #70103, #24517, #73779 ) ) ;
#65584=CARTESIAN_POINT ( 'NONE',  ( 1.354709868695618935, 0.5000000000000004441, -14.93870011653151586 ) ) ;
#65587=VECTOR ( 'NONE', #28987, 1000.000000000000227 ) ;
#65590=ORIENTED_EDGE ( 'NONE', *, *, #71517, .F. ) ;
#65592=CARTESIAN_POINT ( 'NONE',  ( 4.841283923550342649, 0.2306972965111894203, 14.13506365971150025 ) ) ;
#65593=ADVANCED_FACE ( 'NONE', ( #12902 ), #43399, .T. ) ;
#65601=( BOUNDED_CURVE ( )  B_SPLINE_CURVE ( 2, ( #73381, #5408, #52364, #42899, #96909, #43379, #13885, #27392, #20400, #66877, #89869, #65879, #74868 ),
 .UNSPECIFIED., .F., .T. ) 
 B_SPLINE_CURVE_WITH_KNOTS ( ( 3, 2, 2, 2, 2, 2, 3 ),
 ( 0.5999999999999999778, 0.6055555555555555136, 0.6111111111111111605, 0.6166666666666666963, 0.6222222222222222321, 0.6277777777777777679, 0.6333333333333333037 ),
 .UNSPECIFIED. ) 
 CURVE ( )  GEOMETRIC_REPRESENTATION_ITEM ( )  RATIONAL_B_SPLINE_CURVE ( ( 1.000000000000000000, 0.9659258262890683122, 1.000000000000000000, 0.9659258262890683122, 1.000000000000000000, 0.9659258262890683122, 1.000000000000000000, 0.9659258262890683122, 1.000000000000000000, 0.9659258262890683122, 1.000000000000000000, 0.9659258262890683122, 1.000000000000000000 ) ) 
 REPRESENTATION_ITEM ( '' )  );
#65608=CARTESIAN_POINT ( 'NONE',  ( -10.39655283154069743, 14.95077488074853456, -10.46698568711278732 ) ) ;
#65618=AXIS2_PLACEMENT_3D ( 'NONE', #50789, #28767, #96801 ) ;
#65627=CARTESIAN_POINT ( 'NONE',  ( -2.915334737309934532, -27.97798132251182679, -10.88017736071109987 ) ) ;
#65632=CARTESIAN_POINT ( 'NONE',  ( 14.82269085861175384, 14.49999999999999112, -2.299529454046946864 ) ) ;
#65635=CARTESIAN_POINT ( 'NONE',  ( -6.898461952320517732, 15.00000000000000000, 12.75387089053304557 ) ) ;
#65641=LINE ( 'NONE', #96665, #91874 ) ;
#65655=LINE ( 'NONE', #33676, #81468 ) ;
#65656=LINE ( 'NONE', #27663, #44166 ) ;
#65658=VECTOR ( 'NONE', #38961, 999.9999999999998863 ) ;
#65662=VERTEX_POINT ( 'NONE', #13903 ) ;
#65665=LINE ( 'NONE', #3220, #10177 ) ;
#65678=CARTESIAN_POINT ( 'NONE',  ( 2.815433093577024426, 15.00000000000000000, 14.73340885523751709 ) ) ;
#65680=CARTESIAN_POINT ( 'NONE',  ( -9.846743663894596210, -34.19940218233254825, -2.638427012816824124 ) ) ;
#65691=AXIS2_PLACEMENT_3D ( 'NONE', #84972, #78454, #9968 ) ;
#65694=EDGE_CURVE ( 'NONE', #9024, #87326, #25742, .T. ) ;
#65695=CARTESIAN_POINT ( 'NONE',  ( 11.09922568453594671, 2.040301336597091897, -6.408140936763241591 ) ) ;
#65696=VERTEX_POINT ( 'NONE', #21906 ) ;
#65699=VERTEX_POINT ( 'NONE', #98414 ) ;
#65705=EDGE_CURVE ( 'NONE', #93129, #81651, #29870, .T. ) ;
#65709=CARTESIAN_POINT ( 'NONE',  ( -1.915564264621230972, 4.378229052359348391E-16, -14.37291249357993372 ) ) ;
#65711=CARTESIAN_POINT ( 'NONE',  ( -9.282040431732539787, 1.863472483959460746E-16, -11.30407325590354439 ) ) ;
#65715=EDGE_CURVE ( 'NONE', #89674, #61056, #83476, .T. ) ;
#65716=DIRECTION ( 'NONE',  ( 0.000000000000000000, 1.000000000000000000, -0.000000000000000000 ) ) ;
#65718=CARTESIAN_POINT ( 'NONE',  ( -13.48255862861917009, 15.00000000000000000, -5.335786055104346559 ) ) ;
#65740=FACE_OUTER_BOUND ( 'NONE', #35598, .T. ) ;
#65753=AXIS2_PLACEMENT_3D ( 'NONE', #4960, #89433, #95964 ) ;
#65776=AXIS2_PLACEMENT_3D ( 'NONE', #33998, #86537, #19022 ) ;
#65777=DIRECTION ( 'NONE',  ( -0.9981347984218665870, 0.000000000000000000, -0.06104853953486361756 ) ) ;
#65780=ORIENTED_EDGE ( 'NONE', *, *, #213, .F. ) ;
#65782=CARTESIAN_POINT ( 'NONE',  ( 5.803070148808322948, 4.011383936018713867E-16, -13.28812917035388175 ) ) ;
#65798=EDGE_CURVE ( 'NONE', #15328, #46342, #91368, .T. ) ;
#65800=EDGE_LOOP ( 'NONE', ( #10525, #12248, #89855, #49692, #40143, #34345 ) ) ;
#65803=CARTESIAN_POINT ( 'NONE',  ( 0.000000000000000000, 0.000000000000000000, -14.25000000000000000 ) ) ;
#65804=EDGE_LOOP ( 'NONE', ( #38437, #8422, #50977, #79715 ) ) ;
#65805=ADVANCED_FACE ( 'NONE', ( #76373 ), #68881, .F. ) ;
#65811=EDGE_CURVE ( 'NONE', #1475, #4350, #69242, .T. ) ;
#65812=EDGE_CURVE ( 'NONE', #56002, #18731, #53366, .T. ) ;
#65825=ADVANCED_FACE ( 'NONE', ( #37897 ), #68389, .F. ) ;
#65830=CARTESIAN_POINT ( 'NONE',  ( 14.26139399675174957, 15.00000000000000000, 2.619664342934486356 ) ) ;
#65833=VECTOR ( 'NONE', #89103, 1000.000000000000114 ) ;
#65835=EDGE_CURVE ( 'NONE', #5117, #44051, #59482, .T. ) ;
#65843=CARTESIAN_POINT ( 'NONE',  ( -14.26328062697247212, 0.04962887699556481347, 3.770429249334694255 ) ) ;
#65844=DIRECTION ( 'NONE',  ( 0.000000000000000000, 1.000000000000000000, 0.000000000000000000 ) ) ;
#65849=ORIENTED_EDGE ( 'NONE', *, *, #1437, .T. ) ;
#65851=VECTOR ( 'NONE', #25725, 1000.000000000000000 ) ;
#65860=CARTESIAN_POINT ( 'NONE',  ( 7.618303901328586036, -2.732951804315999255E-15, -12.48478900416261617 ) ) ;
#65862=CIRCLE ( 'NONE', #86648, 14.49999999999999822 ) ;
#65865=LINE ( 'NONE', #73366, #3107 ) ;
#65874=CARTESIAN_POINT ( 'NONE',  ( 14.73551000134586531, 14.95037106540114991, 0.7225335126798774210 ) ) ;
#65876=ORIENTED_EDGE ( 'NONE', *, *, #31618, .F. ) ;
#65879=CARTESIAN_POINT ( 'NONE',  ( -3.014428414850124138, 8.963468844518210688, 11.25000000000000178 ) ) ;
#65881=B_SPLINE_CURVE_WITH_KNOTS ( 'NONE', 3,
 ( #92169, #90683, #45187, #98722, #91174, #36711 ),
 .UNSPECIFIED., .F., .F.,
 ( 4, 2, 4 ),
 ( 3.409110551496115105E-05, 0.0004400426677367861379, 0.0008459942299586110503 ),
 .UNSPECIFIED. ) ;
#65883=CARTESIAN_POINT ( 'NONE',  ( -11.92686044187656513, 9.688309369127519943, 3.903127820947815962E-15 ) ) ;
#65885=VERTEX_POINT ( 'NONE', #9850 ) ;
#65889=LINE ( 'NONE', #96919, #63040 ) ;
#65892=CARTESIAN_POINT ( 'NONE',  ( 5.073789285385966963, 0.000000000000000000, 1.998618750576407699 ) ) ;
#65896=CARTESIAN_POINT ( 'NONE',  ( -5.803070148808410877, 4.629725225344712954E-16, 13.28812917035384267 ) ) ;
#65897=DIRECTION ( 'NONE',  ( 0.04361938736533305799, 0.000000000000000000, 0.9990482215818579093 ) ) ;
#65900=ADVANCED_FACE ( 'NONE', ( #93335 ), #71338, .T. ) ;
#65908=CIRCLE ( 'NONE', #43570, 15.00000000000000000 ) ;
#65909=ORIENTED_EDGE ( 'NONE', *, *, #80971, .F. ) ;
#65919=VERTEX_POINT ( 'NONE', #24855 ) ;
#65923=CARTESIAN_POINT ( 'NONE',  ( -11.96291822454869802, 15.00000000000000000, -8.193813980849247613 ) ) ;
#65924=VERTEX_POINT ( 'NONE', #39368 ) ;
#65935=DIRECTION ( 'NONE',  ( 0.000000000000000000, 0.000000000000000000, 1.000000000000000000 ) ) ;
#65936=B_SPLINE_CURVE_WITH_KNOTS ( 'NONE', 3,
 ( #77828, #62329, #92837, #54828, #85340, #47328 ),
 .UNSPECIFIED., .F., .F.,
 ( 4, 2, 4 ),
 ( 0.0002800008091676944129, 0.0006862060465022835464, 0.001092411283836872788 ),
 .UNSPECIFIED. ) ;
#65938=CARTESIAN_POINT ( 'NONE',  ( 0.000000000000000000, -0.03417435944610275333, 14.25000000000000000 ) ) ;
#65940=EDGE_LOOP ( 'NONE', ( #55763, #19816, #80620, #13425 ) ) ;
#65941=VECTOR ( 'NONE', #50312, 1000.000000000000000 ) ;
#65943=CARTESIAN_POINT ( 'NONE',  ( 6.408140936763236262, -27.54303199673624292, -11.09922568453595026 ) ) ;
#65951=VECTOR ( 'NONE', #39956, 999.9999999999998863 ) ;
#65959=EDGE_CURVE ( 'NONE', #48237, #935, #67572, .T. ) ;
#65960=EDGE_LOOP ( 'NONE', ( #73511, #58290, #323, #7385 ) ) ;
#65962=CARTESIAN_POINT ( 'NONE',  ( 3.195792623639469809, 8.229976035794180689, -11.92686044187660066 ) ) ;
#65968=PLANE ( 'NONE',  #8423 ) ;
#65971=ORIENTED_EDGE ( 'NONE', *, *, #45437, .F. ) ;
#65975=ORIENTED_EDGE ( 'NONE', *, *, #50608, .F. ) ;
#65978=VECTOR ( 'NONE', #25531, 1000.000000000000000 ) ;
#65979=DIRECTION ( 'NONE',  ( 0.4305110968082926370, -0.000000000000000000, 0.9025852843498617384 ) ) ;
#65986=CARTESIAN_POINT ( 'NONE',  ( 13.40508947812165097, 15.00000000000000000, -5.527528931046084004 ) ) ;
#65987=ORIENTED_EDGE ( 'NONE', *, *, #13337, .F. ) ;
#65996=CARTESIAN_POINT ( 'NONE',  ( 7.082119434687054849, -31.52958449841936073, 12.26659068614894288 ) ) ;
#66007=DIRECTION ( 'NONE',  ( -0.000000000000000000, -1.000000000000000000, -0.000000000000000000 ) ) ;
#66010=CARTESIAN_POINT ( 'NONE',  ( -10.88017736071109987, 18.27201867748817321, 2.915334737309934532 ) ) ;
#66018=DIRECTION ( 'NONE',  ( 0.000000000000000000, 0.000000000000000000, 1.000000000000000000 ) ) ;
#66026=CARTESIAN_POINT ( 'NONE',  ( 10.32896413005680181, 10.57879003517447813, -5.963430220938285231 ) ) ;
#66028=VERTEX_POINT ( 'NONE', #57785 ) ;
#66031=LINE ( 'NONE', #96560, #23876 ) ;
#66040=LINE ( 'NONE', #58541, #3418 ) ;
#66053=ADVANCED_FACE ( 'NONE', ( #19305 ), #75555, .T. ) ;
#66058=CARTESIAN_POINT ( 'NONE',  ( 9.846743663894594434, -1.491068848999209440, -2.168404344971008868E-15 ) ) ;
#66059=ORIENTED_EDGE ( 'NONE', *, *, #23066, .F. ) ;
#66060=ORIENTED_EDGE ( 'NONE', *, *, #31602, .T. ) ;
#66062=ORIENTED_EDGE ( 'NONE', *, *, #57607, .T. ) ;
#66071=ORIENTED_EDGE ( 'NONE', *, *, #15810, .F. ) ;
#66083=EDGE_CURVE ( 'NONE', #1208, #36938, #57297, .T. ) ;
#66084=ORIENTED_EDGE ( 'NONE', *, *, #25425, .T. ) ;
#66086=ORIENTED_EDGE ( 'NONE', *, *, #65835, .T. ) ;
#66092=LINE ( 'NONE', #20108, #93742 ) ;
#66093=CARTESIAN_POINT ( 'NONE',  ( 0.000000000000000000, 0.000000000000000000, 0.000000000000000000 ) ) ;
#66096=DIRECTION ( 'NONE',  ( 0.9799247046208268141, 0.000000000000000000, 0.1993679344172108459 ) ) ;
#66098=DIRECTION ( 'NONE',  ( 0.9969173337331289630, 0.000000000000000000, -0.07845909572783234254 ) ) ;
#66100=CARTESIAN_POINT ( 'NONE',  ( 0.000000000000000000, 14.49999999999999822, 0.000000000000000000 ) ) ;
#66106=CARTESIAN_POINT ( 'NONE',  ( 14.40939250469964961, 15.00000000000000000, 1.618458416365853747 ) ) ;
#66107=B_SPLINE_CURVE_WITH_KNOTS ( 'NONE', 3,
 ( #34931, #19451, #4463, #41972, #95453, #5450 ),
 .UNSPECIFIED., .F., .F.,
 ( 4, 2, 4 ),
 ( 3.409110551496096132E-05, 0.0004400426677367858127, 0.0008459942299586107250 ),
 .UNSPECIFIED. ) ;
#66108=VECTOR ( 'NONE', #10406, 1000.000000000000227 ) ;
#66116=CARTESIAN_POINT ( 'NONE',  ( -12.60589901313227124, 0.5000000000000004441, 8.129656208641961257 ) ) ;
#66117=FACE_OUTER_BOUND ( 'NONE', #50924, .T. ) ;
#66122=CARTESIAN_POINT ( 'NONE',  ( -5.440088680355547268, -21.10298132251182324, 9.422509992056143702 ) ) ;
#66126=CARTESIAN_POINT ( 'NONE',  ( -14.99847009497944406, 15.00000000000000000, -0.2142307401082361173 ) ) ;
#66128=EDGE_CURVE ( 'NONE', #58242, #64886, #64428, .T. ) ;
#66138=ORIENTED_EDGE ( 'NONE', *, *, #8485, .T. ) ;
#66147=CARTESIAN_POINT ( 'NONE',  ( -3.420591144908647241, 0.5000000000000004441, 14.60477854057953451 ) ) ;
#66150=ORIENTED_EDGE ( 'NONE', *, *, #72450, .T. ) ;
#66155=CARTESIAN_POINT ( 'NONE',  ( 0.000000000000000000, 0.5000000000000004441, 0.000000000000000000 ) ) ;
#66158=EDGE_CURVE ( 'NONE', #32127, #29785, #25836, .T. ) ;
#66172=B_SPLINE_CURVE_WITH_KNOTS ( 'NONE', 3,
 ( #54180, #84693, #94150, #54667, #2201, #85184 ),
 .UNSPECIFIED., .F., .F.,
 ( 4, 2, 4 ),
 ( 0.0002800591277523066546, 0.0006862649357714347472, 0.001092470743790562894 ),
 .UNSPECIFIED. ) ;
#66173=CARTESIAN_POINT ( 'NONE',  ( -9.846743663894594434, -38.99106884899920544, 3.469446951953614189E-15 ) ) ;
#66180=FACE_OUTER_BOUND ( 'NONE', #62268, .T. ) ;
#66184=CARTESIAN_POINT ( 'NONE',  ( -3.434112377981047626, 10.16530133659709101, 12.81628187352647963 ) ) ;
#66199=EDGE_CURVE ( 'NONE', #89050, #7752, #95908, .T. ) ;
#66200=( BOUNDED_CURVE ( )  B_SPLINE_CURVE ( 2, ( #32069, #86575, #55588, #49060, #70097, #94067, #9586, #1620, #86084, #40586, #2115, #10087, #56081 ),
 .UNSPECIFIED., .F., .F. ) 
 B_SPLINE_CURVE_WITH_KNOTS ( ( 3, 2, 2, 2, 2, 2, 3 ),
 ( 0.6999999999999999556, 0.7055555555555556024, 0.7111111111111111382, 0.7166666666666666741, 0.7222222222222222099, 0.7277777777777777457, 0.7298586539780400617 ),
 .UNSPECIFIED. ) 
 CURVE ( )  GEOMETRIC_REPRESENTATION_ITEM ( )  RATIONAL_B_SPLINE_CURVE ( ( 1.000000000000000000, 0.9659258262890683122, 1.000000000000000000, 0.9659258262890683122, 1.000000000000000000, 0.9659258262890683122, 1.000000000000000000, 0.9659258262890683122, 1.000000000000000000, 0.9659258262890683122, 1.000000000000000000, 0.9872372553186372635, 0.9840352796339646435 ) ) 
 REPRESENTATION_ITEM ( '' )  );
#66205=DIRECTION ( 'NONE',  ( 0.3826834323650877279, 0.000000000000000000, -0.9238795325112876267 ) ) ;
#66210=ORIENTED_EDGE ( 'NONE', *, *, #77155, .T. ) ;
#66219=CARTESIAN_POINT ( 'NONE',  ( -10.91061041304814694, 0.2306972965111899476, -10.20767530377064247 ) ) ;
#66220=CIRCLE ( 'NONE', #19918, 15.00000000000000000 ) ;
#66225=CARTESIAN_POINT ( 'NONE',  ( 9.898881779040729967, -0.03417435944610275333, -10.25059215482576214 ) ) ;
#66228=CARTESIAN_POINT ( 'NONE',  ( 3.469446951953614189E-15, 6.368033628982654903, 11.25000000000000178 ) ) ;
#66238=CARTESIAN_POINT ( 'NONE',  ( 10.36894250292379027, 3.678748834913966981, 10.36894250292378672 ) ) ;
#66241=CARTESIAN_POINT ( 'NONE',  ( 9.240973841163597768, 15.00000000000000000, -11.17382667070370061 ) ) ;
#66249=EDGE_CURVE ( 'NONE', #5813, #57430, #66776, .T. ) ;
#66251=DIRECTION ( 'NONE',  ( 0.9099612708765425495, 0.000000000000000000, 0.4146932426562403018 ) ) ;
#66259=CARTESIAN_POINT ( 'NONE',  ( -12.58848565468349001, 1.192622389734054483E-15, -7.447709424580051696 ) ) ;
#66277=EDGE_CURVE ( 'NONE', #1146, #28932, #44062, .T. ) ;
#66282=DIRECTION ( 'NONE',  ( 0.000000000000000000, 1.000000000000000000, 0.000000000000000000 ) ) ;
#66287=CARTESIAN_POINT ( 'NONE',  ( -14.88640444357871395, 0.2306972965111902807, 1.277895705730144993 ) ) ;
#66292=ORIENTED_EDGE ( 'NONE', *, *, #80725, .F. ) ;
#66295=ORIENTED_EDGE ( 'NONE', *, *, #7012, .F. ) ;
#66299=CARTESIAN_POINT ( 'NONE',  ( -14.99847009497950978, 14.49999999999999112, 0.2142307401079103502 ) ) ;
#66303=TOROIDAL_SURFACE ( 'NONE', #15231, 14.49999999999999822, 0.5000000000000000000 ) ;
#66308=ORIENTED_EDGE ( 'NONE', *, *, #18765, .F. ) ;
#66310=ORIENTED_EDGE ( 'NONE', *, *, #98402, .T. ) ;
#66311=TOROIDAL_SURFACE ( 'NONE', #50321, 14.49999999999999822, 0.5000000000000000000 ) ;
#66318=EDGE_CURVE ( 'NONE', #15469, #70448, #94241, .T. ) ;
#66328=ORIENTED_EDGE ( 'NONE', *, *, #87058, .F. ) ;
#66331=CARTESIAN_POINT ( 'NONE',  ( 7.313705784284503686, 15.00000000000000000, 13.09617149020748705 ) ) ;
#66332=CARTESIAN_POINT ( 'NONE',  ( -7.264509831664783590, 14.76984904925306097, 13.05561747642785342 ) ) ;
#66340=CARTESIAN_POINT ( 'NONE',  ( -10.93781366033354452, 14.63595249122790598, 10.26470809774058779 ) ) ;
#66341=CARTESIAN_POINT ( 'NONE',  ( 0.000000000000000000, 15.00000000000000000, 0.000000000000000000 ) ) ;
#66359=EDGE_LOOP ( 'NONE', ( #82786, #89570, #83736, #70154 ) ) ;
#66363=DIRECTION ( 'NONE',  ( 0.000000000000000000, 0.000000000000000000, -1.000000000000000000 ) ) ;
#66366=ORIENTED_EDGE ( 'NONE', *, *, #74756, .T. ) ;
#66374=DIRECTION ( 'NONE',  ( -0.1305261922200653402, -0.000000000000000000, 0.9914448613738086058 ) ) ;
#66381=EDGE_LOOP ( 'NONE', ( #92857, #58175, #93291, #81270, #73582, #1790 ) ) ;
#66382=DIRECTION ( 'NONE',  ( 0.000000000000000000, 1.000000000000000000, 0.000000000000000000 ) ) ;
#66383=B_SPLINE_CURVE_WITH_KNOTS ( 'NONE', 3,
 ( #48680, #49176, #79678, #72166, #85221, #47200 ),
 .UNSPECIFIED., .F., .F.,
 ( 4, 2, 4 ),
 ( 0.0002800313526786637011, 0.0006862368888239586684, 0.001092442424969253690 ),
 .UNSPECIFIED. ) ;
#66385=CARTESIAN_POINT ( 'NONE',  ( 8.564643372776616914, 14.49999999999999822, -12.31449893000740836 ) ) ;
#66387=CARTESIAN_POINT ( 'NONE',  ( 0.000000000000000000, 0.5000000000000004441, 0.000000000000000000 ) ) ;
#66400=VECTOR ( 'NONE', #40922, 1000.000000000000000 ) ;
#66411=DIRECTION ( 'NONE',  ( -0.3173046564050834295, 0.000000000000000000, -0.9483236552062023206 ) ) ;
#66413=EDGE_CURVE ( 'NONE', #92402, #74265, #68759, .T. ) ;
#66431=PLANE ( 'NONE',  #20602 ) ;
#66434=ORIENTED_EDGE ( 'NONE', *, *, #19577, .F. ) ;
#66436=CARTESIAN_POINT ( 'NONE',  ( 3.434112377981060948, -24.41803199673624647, 12.81628187352647430 ) ) ;
#66445=CARTESIAN_POINT ( 'NONE',  ( -13.16767742306221400, 0.04962884061926597229, 6.653539137814544979 ) ) ;
#66446=ORIENTED_EDGE ( 'NONE', *, *, #79376, .T. ) ;
#66459=EDGE_CURVE ( 'NONE', #43481, #1023, #57557, .T. ) ;
#66460=LINE ( 'NONE', #59448, #14951 ) ;
#66463=DIRECTION ( 'NONE',  ( 0.000000000000000000, 1.000000000000000000, 0.000000000000000000 ) ) ;
#66468=CIRCLE ( 'NONE', #72884, 15.00000000000000000 ) ;
#66483=CARTESIAN_POINT ( 'NONE',  ( -11.59608414876355198, 14.76930270348881002, 9.421724210956202938 ) ) ;
#66484=ORIENTED_EDGE ( 'NONE', *, *, #33090, .F. ) ;
#66489=ORIENTED_EDGE ( 'NONE', *, *, #93846, .T. ) ;
#66495=CIRCLE ( 'NONE', #63272, 15.00000000000000000 ) ;
#66497=CARTESIAN_POINT ( 'NONE',  ( 3.795296366450314540, -21.73791783175269998, 14.16423886937410082 ) ) ;
#66504=EDGE_CURVE ( 'NONE', #32902, #78512, #53641, .T. ) ;
#66511=CARTESIAN_POINT ( 'NONE',  ( 0.000000000000000000, 14.49999999999999822, 0.000000000000000000 ) ) ;
#66513=CARTESIAN_POINT ( 'NONE',  ( 9.422509992056141925, 25.98035201082152312, -5.440088680355554374 ) ) ;
#66517=ORIENTED_EDGE ( 'NONE', *, *, #58179, .F. ) ;
#66518=AXIS2_PLACEMENT_3D ( 'NONE', #89649, #13154, #80676 ) ;
#66522=B_SPLINE_CURVE_WITH_KNOTS ( 'NONE', 3,
 ( #54453, #24970, #46467, #40461, #25468, #10445 ),
 .UNSPECIFIED., .F., .F.,
 ( 4, 2, 4 ),
 ( 3.409110551378489334E-05, 0.0004400426677356115675, 0.0008459942299574381604 ),
 .UNSPECIFIED. ) ;
#66530=VERTEX_POINT ( 'NONE', #47216 ) ;
#66536=DIRECTION ( 'NONE',  ( 0.000000000000000000, 1.000000000000000000, 0.000000000000000000 ) ) ;
#66544=B_SPLINE_CURVE_WITH_KNOTS ( 'NONE', 3,
 ( #20468, #50955, #66445, #81451, #12952, #5960 ),
 .UNSPECIFIED., .F., .F.,
 ( 4, 2, 4 ),
 ( 0.0002800760588349525144, 0.0006862820326512275061, 0.001092488006467502498 ),
 .UNSPECIFIED. ) ;
#66547=EDGE_LOOP ( 'NONE', ( #85399, #52088, #4813, #21663 ) ) ;
#66553=CARTESIAN_POINT ( 'NONE',  ( 0.000000000000000000, 14.49999999999999822, 0.000000000000000000 ) ) ;
#66556=CIRCLE ( 'NONE', #26637, 14.49999999999999822 ) ;
#66561=CARTESIAN_POINT ( 'NONE',  ( -2.638427012816824124, 22.05059781766745886, 9.846743663894596210 ) ) ;
#66562=ORIENTED_EDGE ( 'NONE', *, *, #26204, .T. ) ;
#66582=ORIENTED_EDGE ( 'NONE', *, *, #57142, .T. ) ;
#66589=EDGE_CURVE ( 'NONE', #5813, #24761, #67997, .T. ) ;
#66593=ORIENTED_EDGE ( 'NONE', *, *, #15246, .T. ) ;
#66595=CARTESIAN_POINT ( 'NONE',  ( 14.97687855664607781, 15.00000000000000000, 0.8325315005901553489 ) ) ;
#66599=CARTESIAN_POINT ( 'NONE',  ( -11.30818108475026129, 12.95584178848497281, 3.038558417133429668 ) ) ;
#66600=CARTESIAN_POINT ( 'NONE',  ( -1.983216688680738082, 0.000000000000000000, -14.11131997956740491 ) ) ;
#66604=EDGE_LOOP ( 'NONE', ( #96313, #73797, #77755, #51843, #69608, #77485 ) ) ;
#66610=DIRECTION ( 'NONE',  ( 0.000000000000000000, 0.000000000000000000, 1.000000000000000000 ) ) ;
#66613=DIRECTION ( 'NONE',  ( 0.000000000000000000, 0.000000000000000000, -1.000000000000000000 ) ) ;
#66616=EDGE_CURVE ( 'NONE', #7648, #54903, #65655, .T. ) ;
#66622=PLANE ( 'NONE',  #56050 ) ;
#66624=LINE ( 'NONE', #97152, #82047 ) ;
#66625=CIRCLE ( 'NONE', #98579, 15.00000000000000000 ) ;
#66629=CARTESIAN_POINT ( 'NONE',  ( -5.440088680355558814, -27.76964798917849109, -9.422509992056136596 ) ) ;
#66635=CARTESIAN_POINT ( 'NONE',  ( 12.87890026492940088, 0.04922511925147125822, -7.195834080858350745 ) ) ;
#66636=CARTESIAN_POINT ( 'NONE',  ( -1.354709868695754826, 14.49999999999999112, 14.93870011653156915 ) ) ;
#66638=CARTESIAN_POINT ( 'NONE',  ( 10.84451454130498149, 15.00000000000000000, 9.625305416630897781 ) ) ;
#66645=DIRECTION ( 'NONE',  ( 0.000000000000000000, 1.000000000000000000, 0.000000000000000000 ) ) ;
#66656=PLANE ( 'NONE',  #94748 ) ;
#66658=CARTESIAN_POINT ( 'NONE',  ( 12.80781515976314822, 0.000000000000000000, -6.246788841744324472 ) ) ;
#66659=CARTESIAN_POINT ( 'NONE',  ( 10.93781366033343083, 14.49999999999999112, 10.26470809774079029 ) ) ;
#66660=ORIENTED_EDGE ( 'NONE', *, *, #22728, .T. ) ;
#66663=VERTEX_POINT ( 'NONE', #18705 ) ;
#66665=CARTESIAN_POINT ( 'NONE',  ( -14.82679024690668967, 0.2306972965111902529, -1.845086899513486367 ) ) ;
#66677=VECTOR ( 'NONE', #67891, 1000.000000000000114 ) ;
#66681=CARTESIAN_POINT ( 'NONE',  ( -9.846743663894590881, -18.78273551566588040, 2.638427012816840111 ) ) ;
#66683=CARTESIAN_POINT ( 'NONE',  ( -14.29730467489527967, 15.00000000000000000, -2.416004766803415471 ) ) ;
#66689=CARTESIAN_POINT ( 'NONE',  ( 0.000000000000000000, 0.000000000000000000, 0.000000000000000000 ) ) ;
#66693=CARTESIAN_POINT ( 'NONE',  ( -9.382169495545422677, 3.498634669930421826, -9.382169495545417348 ) ) ;
#66703=CARTESIAN_POINT ( 'NONE',  ( 14.02068044289378967, 15.00000000000000000, -5.331089937175664595 ) ) ;
#66706=EDGE_CURVE ( 'NONE', #5095, #9889, #4195, .T. ) ;
#66707=EDGE_CURVE ( 'NONE', #4865, #92052, #87885, .T. ) ;
#66708=VECTOR ( 'NONE', #91713, 1000.000000000000000 ) ;
#66710=CARTESIAN_POINT ( 'NONE',  ( 10.04796213703172647, 2.879912020664621153E-16, 10.62905469192473440 ) ) ;
#66713=DIRECTION ( 'NONE',  ( -0.000000000000000000, -1.000000000000000000, -0.000000000000000000 ) ) ;
#66717=CARTESIAN_POINT ( 'NONE',  ( -0.9940297508538862292, 15.00000000000000000, 14.21528771620248932 ) ) ;
#66718=ORIENTED_EDGE ( 'NONE', *, *, #98591, .T. ) ;
#66720=CARTESIAN_POINT ( 'NONE',  ( -9.876730923139385609, 0.3640475087720987935, 11.28938378619056948 ) ) ;
#66721=ADVANCED_FACE ( 'NONE', ( #33195 ), #63688, .F. ) ;
#66732=ADVANCED_FACE ( 'NONE', ( #94695 ), #72179, .T. ) ;
#66739=CARTESIAN_POINT ( 'NONE',  ( 0.000000000000000000, 14.49999999999999822, 0.000000000000000000 ) ) ;
#66742=FACE_OUTER_BOUND ( 'NONE', #36552, .T. ) ;
#66746=CARTESIAN_POINT ( 'NONE',  ( -14.16423886937409726, 12.01208216824730357, 3.795296366450320757 ) ) ;
#66749=CARTESIAN_POINT ( 'NONE',  ( 12.83294900548058415, 0.3640475087720986269, 7.766300266068457248 ) ) ;
#66758=DIRECTION ( 'NONE',  ( 0.000000000000000000, 0.000000000000000000, 1.000000000000000000 ) ) ;
#66759=CARTESIAN_POINT ( 'NONE',  ( 3.193136578976985440, 15.00000000000000888, 14.27383009353652987 ) ) ;
#66760=CARTESIAN_POINT ( 'NONE',  ( 9.898881779040729967, 15.00000000000000000, -10.25059215482576214 ) ) ;
#66763=ORIENTED_EDGE ( 'NONE', *, *, #22160, .F. ) ;
#66766=CARTESIAN_POINT ( 'NONE',  ( 0.000000000000000000, 14.49999999999999822, 0.000000000000000000 ) ) ;
#66771=EDGE_CURVE ( 'NONE', #70993, #64180, #71218, .T. ) ;
#66776=LINE ( 'NONE', #89280, #14471 ) ;
#66782=VECTOR ( 'NONE', #82045, 1000.000000000000000 ) ;
#66801=ORIENTED_EDGE ( 'NONE', *, *, #97677, .F. ) ;
#66807=CARTESIAN_POINT ( 'NONE',  ( -5.376821459230213485, 14.76984886575651501, 13.93958558162633921 ) ) ;
#66811=ORIENTED_EDGE ( 'NONE', *, *, #54184, .F. ) ;
#66813=ORIENTED_EDGE ( 'NONE', *, *, #30362, .F. ) ;
#66822=EDGE_LOOP ( 'NONE', ( #60904, #77744, #60135, #92640, #98015, #30542 ) ) ;
#66829=CARTESIAN_POINT ( 'NONE',  ( -7.684764310694971456, 14.49999999999999822, 12.88194075009929840 ) ) ;
#66833=CARTESIAN_POINT ( 'NONE',  ( 0.000000000000000000, 14.49999999999999822, 0.000000000000000000 ) ) ;
#66840=DIRECTION ( 'NONE',  ( -0.000000000000000000, -1.000000000000000000, -0.000000000000000000 ) ) ;
#66843=VECTOR ( 'NONE', #73706, 1000.000000000000000 ) ;
#66846=EDGE_CURVE ( 'NONE', #38139, #92170, #42196, .T. ) ;
#66852=CARTESIAN_POINT ( 'NONE',  ( 7.551349515323185990, 15.00000000000000000, -12.08468537022906020 ) ) ;
#66863=ORIENTED_EDGE ( 'NONE', *, *, #7382, .F. ) ;
#66876=DIRECTION ( 'NONE',  ( 0.000000000000000000, 0.000000000000000000, 1.000000000000000000 ) ) ;
#66877=CARTESIAN_POINT ( 'NONE',  ( -8.235571585149864760, 8.546802177851539284, 8.235571585149875418 ) ) ;
#66884=LINE ( 'NONE', #58885, #29293 ) ;
#66885=DIRECTION ( 'NONE',  ( 0.000000000000000000, 1.000000000000000000, 0.000000000000000000 ) ) ;
#66890=CARTESIAN_POINT ( 'NONE',  ( 0.7375392941517235901, 15.00000000000000000, 14.98185688723471110 ) ) ;
#66894=DIRECTION ( 'NONE',  ( -0.000000000000000000, -1.000000000000000000, -0.000000000000000000 ) ) ;
#66898=EDGE_CURVE ( 'NONE', #13755, #46052, #25721, .T. ) ;
#66900=CARTESIAN_POINT ( 'NONE',  ( 10.14667048435138064, 4.748928130477084912E-16, 10.35833375027048042 ) ) ;
#66918=DIRECTION ( 'NONE',  ( -0.9862856015372308827, 0.000000000000000000, -0.1650476058606810681 ) ) ;
#66920=ORIENTED_EDGE ( 'NONE', *, *, #11527, .T. ) ;
#66936=CARTESIAN_POINT ( 'NONE',  ( 12.81628187352647608, -18.58469866340291077, 3.434112377981052511 ) ) ;
#66946=EDGE_CURVE ( 'NONE', #65284, #25080, #72660, .T. ) ;
#66950=ORIENTED_EDGE ( 'NONE', *, *, #81754, .T. ) ;
#66955=ORIENTED_EDGE ( 'NONE', *, *, #95849, .T. ) ;
#66964=CARTESIAN_POINT ( 'NONE',  ( 6.689969769698956625, -0.03417435944610275333, -12.58200319823970226 ) ) ;
#66969=DIRECTION ( 'NONE',  ( -0.8038568606172203923, 0.000000000000000000, 0.5948227867513371514 ) ) ;
#66982=ORIENTED_EDGE ( 'NONE', *, *, #6586, .T. ) ;
#66992=CARTESIAN_POINT ( 'NONE',  ( 14.16423886937410437, -25.90458449841936073, 3.795296366450304770 ) ) ;
#67003=CARTESIAN_POINT ( 'NONE',  ( 0.000000000000000000, 0.5000000000000004441, 0.000000000000000000 ) ) ;
#67009=CARTESIAN_POINT ( 'NONE',  ( -10.88017736071109987, 28.27201867748817676, 2.915334737309934532 ) ) ;
#67015=AXIS2_PLACEMENT_3D ( 'NONE', #51413, #80929, #65416 ) ;
#67016=ADVANCED_FACE ( 'NONE', ( #4694 ), #51161, .T. ) ;
#67018=CARTESIAN_POINT ( 'NONE',  ( 0.000000000000000000, 14.49999999999999822, 0.000000000000000000 ) ) ;
#67025=DIRECTION ( 'NONE',  ( 0.000000000000000000, 0.000000000000000000, -1.000000000000000000 ) ) ;
#67033=DIRECTION ( 'NONE',  ( -0.000000000000000000, -1.000000000000000000, -0.000000000000000000 ) ) ;
#67037=CARTESIAN_POINT ( 'NONE',  ( 13.21382278599139859, 7.555533889508357052E-16, -6.271621331965521406 ) ) ;
#67039=CYLINDRICAL_SURFACE ( 'NONE', #48970, 15.00000000000000000 ) ;
#67055=CARTESIAN_POINT ( 'NONE',  ( -2.638427012816840111, 19.96726448433413026, -9.846743663894590881 ) ) ;
#67060=EDGE_LOOP ( 'NONE', ( #64698, #93594, #64051, #98451, #28653 ) ) ;
#67072=ORIENTED_EDGE ( 'NONE', *, *, #24772, .F. ) ;
#67074=EDGE_LOOP ( 'NONE', ( #89813, #58417, #18576, #82570 ) ) ;
#67081=AXIS2_PLACEMENT_3D ( 'NONE', #88829, #50837, #81330 ) ;
#67082=EDGE_CURVE ( 'NONE', #96556, #58998, #36660, .T. ) ;
#67085=FACE_OUTER_BOUND ( 'NONE', #29613, .T. ) ;
#67093=CARTESIAN_POINT ( 'NONE',  ( -11.09639892720896093, 12.99830704344312693, 3.869676107586555336 ) ) ;
#67099=ORIENTED_EDGE ( 'NONE', *, *, #66616, .F. ) ;
#67102=CARTESIAN_POINT ( 'NONE',  ( 6.767445849361248378, 14.63595249122789177, -13.38662304974498340 ) ) ;
#67105=CARTESIAN_POINT ( 'NONE',  ( -14.82269085861170232, 0.5000000000000004441, 2.299529454046861154 ) ) ;
#67114=CARTESIAN_POINT ( 'NONE',  ( -10.58981376305275468, -0.03417435944610275333, -9.535111140613857117 ) ) ;
#67116=FACE_OUTER_BOUND ( 'NONE', #28995, .T. ) ;
#67117=FACE_OUTER_BOUND ( 'NONE', #32656, .T. ) ;
#67121=CARTESIAN_POINT ( 'NONE',  ( -7.964842623401172439, -6.311314655845153609, 7.964842623401183097 ) ) ;
#67124=CARTESIAN_POINT ( 'NONE',  ( 14.73513795193454534, 0.04922511925147087658, 0.7223639599947853096 ) ) ;
#67125=DIRECTION ( 'NONE',  ( 0.000000000000000000, 0.000000000000000000, 1.000000000000000000 ) ) ;
#67143=EDGE_CURVE ( 'NONE', #73111, #33570, #62339, .T. ) ;
#67146=CARTESIAN_POINT ( 'NONE',  ( -12.80781515976305762, -0.03417435944610275333, -6.246788841744501219 ) ) ;
#67147=DIRECTION ( 'NONE',  ( 0.7716245833877193316, 0.000000000000000000, -0.6360782202777648386 ) ) ;
#67148=VECTOR ( 'NONE', #69294, 1000.000000000000000 ) ;
#67149=EDGE_CURVE ( 'NONE', #72566, #72059, #60127, .T. ) ;
#67150=VERTEX_POINT ( 'NONE', #66147 ) ;
#67151=CARTESIAN_POINT ( 'NONE',  ( -14.43063482171890399, 15.00000000000000888, -2.386446184883220578 ) ) ;
#67154=ORIENTED_EDGE ( 'NONE', *, *, #98535, .T. ) ;
#67155=DIRECTION ( 'NONE',  ( 0.09584575252023383451, 0.000000000000000000, -0.9953961983671778535 ) ) ;
#67172=CARTESIAN_POINT ( 'NONE',  ( -9.846743663894596210, -24.19940218233254114, -2.638427012816824124 ) ) ;
#67175=ORIENTED_EDGE ( 'NONE', *, *, #9982, .F. ) ;
#67176=ORIENTED_EDGE ( 'NONE', *, *, #51871, .F. ) ;
#67178=CARTESIAN_POINT ( 'NONE',  ( 11.81378540890930751, 15.00000000000000000, 7.968498874458199488 ) ) ;
#67186=ADVANCED_FACE ( 'NONE', ( #52145 ), #61774, .T. ) ;
#67188=CARTESIAN_POINT ( 'NONE',  ( -3.434112377981067610, 18.08196800326375708, -12.81628187352647252 ) ) ;
#67189=EDGE_CURVE ( 'NONE', #76776, #3849, #6155, .T. ) ;
#67190=ORIENTED_EDGE ( 'NONE', *, *, #35460, .T. ) ;
#67193=VERTEX_POINT ( 'NONE', #5672 ) ;
#67203=VECTOR ( 'NONE', #47076, 999.9999999999998863 ) ;
#67204=EDGE_LOOP ( 'NONE', ( #36704, #10454, #19848, #32478, #98208, #45568 ) ) ;
#67205=DIRECTION ( 'NONE',  ( -0.000000000000000000, -1.000000000000000000, -0.000000000000000000 ) ) ;
#67206=DIRECTION ( 'NONE',  ( 0.000000000000000000, 1.000000000000000000, 0.000000000000000000 ) ) ;
#67208=EDGE_CURVE ( 'NONE', #52058, #57773, #15491, .T. ) ;
#67213=LINE ( 'NONE', #53681, #21239 ) ;
#67214=ADVANCED_FACE ( 'NONE', ( #97670 ), #91126, .F. ) ;
#67215=ORIENTED_EDGE ( 'NONE', *, *, #14696, .T. ) ;
#67217=CARTESIAN_POINT ( 'NONE',  ( -9.399392868737892925, 4.026710370808002065E-16, 11.04089732309467919 ) ) ;
#67222=DIRECTION ( 'NONE',  ( -0.000000000000000000, -1.000000000000000000, -0.000000000000000000 ) ) ;
#67224=CARTESIAN_POINT ( 'NONE',  ( 0.000000000000000000, 15.00000000000000000, 0.000000000000000000 ) ) ;
#67230=ORIENTED_EDGE ( 'NONE', *, *, #88708, .F. ) ;
#67231=CARTESIAN_POINT ( 'NONE',  ( -3.843478602184351889, 0.2306972965111881713, -14.43834224996327897 ) ) ;
#67235=DIRECTION ( 'NONE',  ( -1.154631945610162802E-14, 0.000000000000000000, 1.000000000000000000 ) ) ;
#67242=CARTESIAN_POINT ( 'NONE',  ( -1.796645268984824240, 14.76930270348881002, 14.83273813124057661 ) ) ;
#67243=CARTESIAN_POINT ( 'NONE',  ( -10.36894250292378317, 17.42874883491396787, 10.36894250292379560 ) ) ;
#67252=VECTOR ( 'NONE', #64518, 1000.000000000000114 ) ;
#67257=FACE_OUTER_BOUND ( 'NONE', #44303, .T. ) ;
#67262=VERTEX_POINT ( 'NONE', #66658 ) ;
#67265=CARTESIAN_POINT ( 'NONE',  ( -12.03829478939416120, 2.168404344971008868E-16, -8.307695547791567492 ) ) ;
#67276=EDGE_CURVE ( 'NONE', #31971, #35670, #42947, .T. ) ;
#67277=EDGE_CURVE ( 'NONE', #74063, #60663, #44642, .T. ) ;
#67295=EDGE_LOOP ( 'NONE', ( #69287, #56999, #57181, #58078, #40371, #98516 ) ) ;
#67304=EDGE_CURVE ( 'NONE', #66028, #84144, #60817, .T. ) ;
#67309=ORIENTED_EDGE ( 'NONE', *, *, #48740, .T. ) ;
#67311=ORIENTED_EDGE ( 'NONE', *, *, #94046, .T. ) ;
#67319=VECTOR ( 'NONE', #10920, 1000.000000000000000 ) ;
#67320=VERTEX_POINT ( 'NONE', #39129 ) ;
#67323=CARTESIAN_POINT ( 'NONE',  ( 2.174473938468889589, 0.000000000000000000, 5.000947681547232904 ) ) ;
#67340=CARTESIAN_POINT ( 'NONE',  ( -10.82344394350238304, 14.95077488074853811, 10.02492699998869163 ) ) ;
#67341=CARTESIAN_POINT ( 'NONE',  ( 0.000000000000000000, 0.000000000000000000, 0.000000000000000000 ) ) ;
#67351=FACE_OUTER_BOUND ( 'NONE', #4567, .T. ) ;
#67357=VECTOR ( 'NONE', #39072, 1000.000000000000000 ) ;
#67376=ORIENTED_EDGE ( 'NONE', *, *, #66706, .F. ) ;
#67383=LINE ( 'NONE', #52869, #92540 ) ;
#67388=CARTESIAN_POINT ( 'NONE',  ( -2.815433093577217161, 0.3639308411966859502, 14.73340885523751531 ) ) ;
#67392=EDGE_CURVE ( 'NONE', #75686, #34469, #44215, .T. ) ;
#67394=AXIS2_PLACEMENT_3D ( 'NONE', #21567, #82048, #37061 ) ;
#67408=ORIENTED_EDGE ( 'NONE', *, *, #4755, .T. ) ;
#67413=DIRECTION ( 'NONE',  ( 0.000000000000000000, 1.000000000000000000, 0.000000000000000000 ) ) ;
#67421=CARTESIAN_POINT ( 'NONE',  ( 14.76100041229771342, 0.2306972965111887264, -2.313205896730830879 ) ) ;
#67426=VECTOR ( 'NONE', #65716, 1000.000000000000000 ) ;
#67427=CARTESIAN_POINT ( 'NONE',  ( 4.267749253172103074, 0.000000000000000000, -3.394721039305288457 ) ) ;
#67432=EDGE_CURVE ( 'NONE', #5083, #89199, #61602, .T. ) ;
#67436=CARTESIAN_POINT ( 'NONE',  ( -12.81628187352647252, -20.66803199673624292, 3.434112377981066722 ) ) ;
#67452=LINE ( 'NONE', #44931, #79271 ) ;
#67461=FACE_BOUND ( 'NONE', #94356, .T. ) ;
#67462=LINE ( 'NONE', #38448, #69716 ) ;
#67467=CARTESIAN_POINT ( 'NONE',  ( 0.2849401152835440709, 0.2301503025712808848, 14.93790629078169019 ) ) ;
#67474=EDGE_CURVE ( 'NONE', #5244, #22303, #23647, .T. ) ;
#67481=CARTESIAN_POINT ( 'NONE',  ( -6.689969769699040114, 15.00000000000000000, 12.58200319823965785 ) ) ;
#67486=DIRECTION ( 'NONE',  ( 0.000000000000000000, 0.000000000000000000, 1.000000000000000000 ) ) ;
#67489=CARTESIAN_POINT ( 'NONE',  ( -14.16423886937410082, -23.19625116508602858, 4.336808689942017736E-15 ) ) ;
#67490=AXIS2_PLACEMENT_3D ( 'NONE', #19915, #5428, #11924 ) ;
#67500=CIRCLE ( 'NONE', #83487, 15.00000000000000000 ) ;
#67501=DIRECTION ( 'NONE',  ( 0.000000000000000000, 0.000000000000000000, 1.000000000000000000 ) ) ;
#67503=CARTESIAN_POINT ( 'NONE',  ( -0.7375392941519274270, 14.63595249122789177, 14.98185688723471110 ) ) ;
#67504=CARTESIAN_POINT ( 'NONE',  ( 10.88017736071109987, 30.77201867748818032, -2.915334737309928315 ) ) ;
#67510=CARTESIAN_POINT ( 'NONE',  ( -14.29730467489535428, 3.987535082655999417E-16, 2.416004766803123260 ) ) ;
#67511=ORIENTED_EDGE ( 'NONE', *, *, #39579, .F. ) ;
#67516=AXIS2_PLACEMENT_3D ( 'NONE', #34548, #56102, #57555 ) ;
#67526=ORIENTED_EDGE ( 'NONE', *, *, #96791, .F. ) ;
#67532=CARTESIAN_POINT ( 'NONE',  ( -11.36220558718869711, 4.706058445226104967E-16, 9.008345252845160189 ) ) ;
#67537=LINE ( 'NONE', #97069, #45810 ) ;
#67544=TOROIDAL_SURFACE ( 'NONE', #57956, 14.49999999999999822, 0.5000000000000000000 ) ;
#67548=EDGE_CURVE ( 'NONE', #40259, #29043, #55438, .T. ) ;
#67558=EDGE_CURVE ( 'NONE', #952, #28596, #87076, .T. ) ;
#67559=DIRECTION ( 'NONE',  ( 0.000000000000000000, 1.000000000000000000, 0.000000000000000000 ) ) ;
#67560=CARTESIAN_POINT ( 'NONE',  ( 8.527530157486179263, 18.09226448433412671, 4.923371831947292776 ) ) ;
#67564=ORIENTED_EDGE ( 'NONE', *, *, #85065, .F. ) ;
#67572=CIRCLE ( 'NONE', #6895, 15.00000000000000000 ) ;
#67575=CIRCLE ( 'NONE', #93107, 14.49999999999999822 ) ;
#67596=ORIENTED_EDGE ( 'NONE', *, *, #45451, .F. ) ;
#67597=CARTESIAN_POINT ( 'NONE',  ( -11.05007230724497092, 12.65949770494214377, -2.855270967710901164 ) ) ;
#67599=DIRECTION ( 'NONE',  ( 0.000000000000000000, 0.000000000000000000, 1.000000000000000000 ) ) ;
#67601=LINE ( 'NONE', #50615, #16324 ) ;
#67603=CARTESIAN_POINT ( 'NONE',  ( 11.42891328973224141, -3.217031133671831504E-15, -9.126250717928387601 ) ) ;
#67605=DIRECTION ( 'NONE',  ( -0.000000000000000000, -1.000000000000000000, -0.000000000000000000 ) ) ;
#67607=VECTOR ( 'NONE', #95657, 1000.000000000000000 ) ;
#67612=CARTESIAN_POINT ( 'NONE',  ( 3.420591144908545100, 15.00000000000000000, -14.60477854057955938 ) ) ;
#67622=CARTESIAN_POINT ( 'NONE',  ( 6.898461952320431578, 15.00000000000000000, -12.75387089053309175 ) ) ;
#67623=CARTESIAN_POINT ( 'NONE',  ( 12.98685442714775640, 15.00000000000000000, 6.449155920607609893 ) ) ;
#67627=CARTESIAN_POINT ( 'NONE',  ( -5.440088680355547268, -16.10298132251182324, 9.422509992056143702 ) ) ;
#67631=CARTESIAN_POINT ( 'NONE',  ( 11.81378540890936080, 15.00000000000000000, -7.968498874458115999 ) ) ;
#67632=CARTESIAN_POINT ( 'NONE',  ( 0.000000000000000000, 0.000000000000000000, 0.000000000000000000 ) ) ;
#67635=EDGE_CURVE ( 'NONE', #49672, #68696, #88265, .T. ) ;
#67640=EDGE_CURVE ( 'NONE', #53171, #15924, #36233, .T. ) ;
#67641=EDGE_CURVE ( 'NONE', #47206, #50542, #7577, .T. ) ;
#67648=VECTOR ( 'NONE', #56461, 1000.000000000000000 ) ;
#67657=VERTEX_POINT ( 'NONE', #34544 ) ;
#67661=ORIENTED_EDGE ( 'NONE', *, *, #54940, .T. ) ;
#67677=EDGE_CURVE ( 'NONE', #67800, #35833, #94087, .T. ) ;
#67678=CARTESIAN_POINT ( 'NONE',  ( -4.923371831947292776, -23.15773551566587685, 8.527530157486181039 ) ) ;
#67679=ORIENTED_EDGE ( 'NONE', *, *, #32736, .T. ) ;
#67681=ORIENTED_EDGE ( 'NONE', *, *, #61311, .F. ) ;
#67684=ORIENTED_EDGE ( 'NONE', *, *, #54300, .F. ) ;
#67685=CARTESIAN_POINT ( 'NONE',  ( 0.000000000000000000, 12.49999999999999112, 11.25000000000000178 ) ) ;
#67692=CARTESIAN_POINT ( 'NONE',  ( 3.469446951953614189E-15, 15.37363466993042849, 12.81628187352647608 ) ) ;
#67693=ORIENTED_EDGE ( 'NONE', *, *, #9140, .T. ) ;
#67696=EDGE_LOOP ( 'NONE', ( #8012, #169, #39549, #59422, #18406, #76870 ) ) ;
#67705=DIRECTION ( 'NONE',  ( 0.000000000000000000, 0.000000000000000000, 1.000000000000000000 ) ) ;
#67707=CARTESIAN_POINT ( 'NONE',  ( -3.420591144908350589, 15.00000000000000000, -14.60477854057960556 ) ) ;
#67708=CARTESIAN_POINT ( 'NONE',  ( -8.839000071696917260, 0.04962890530003090384, -11.81225584161653330 ) ) ;
#67709=DIRECTION ( 'NONE',  ( 0.000000000000000000, 1.000000000000000000, 0.000000000000000000 ) ) ;
#67712=AXIS2_PLACEMENT_3D ( 'NONE', #72875, #11398, #41921 ) ;
#67713=CARTESIAN_POINT ( 'NONE',  ( 0.000000000000000000, 14.49999999999999822, 0.000000000000000000 ) ) ;
#67714=ORIENTED_EDGE ( 'NONE', *, *, #58022, .T. ) ;
#67716=DIRECTION ( 'NONE',  ( 0.000000000000000000, 0.000000000000000000, 1.000000000000000000 ) ) ;
#67732=ORIENTED_EDGE ( 'NONE', *, *, #47320, .T. ) ;
#67737=CARTESIAN_POINT ( 'NONE',  ( 0.000000000000000000, 14.49999999999999822, 0.000000000000000000 ) ) ;
#67741=CARTESIAN_POINT ( 'NONE',  ( -7.684764310694971456, 15.00000000000000000, 12.88194075009929840 ) ) ;
#67745=CARTESIAN_POINT ( 'NONE',  ( -7.082119434687044190, 22.63708216824730712, 12.26659068614894998 ) ) ;
#67747=EDGE_CURVE ( 'NONE', #69120, #58939, #57272, .T. ) ;
#67752=EDGE_CURVE ( 'NONE', #74794, #30654, #71100, .T. ) ;
#67760=EDGE_CURVE ( 'NONE', #54280, #71137, #55606, .T. ) ;
#67764=VERTEX_POINT ( 'NONE', #57062 ) ;
#67767=CARTESIAN_POINT ( 'NONE',  ( -14.82269085861176983, 14.49999999999999112, 2.299529454046846499 ) ) ;
#67774=CARTESIAN_POINT ( 'NONE',  ( 4.838527690343618737, 0.5000000000000004441, -14.19819177887726624 ) ) ;
#67777=ORIENTED_EDGE ( 'NONE', *, *, #56679, .T. ) ;
#67780=VECTOR ( 'NONE', #20487, 1000.000000000000000 ) ;
#67790=DIRECTION ( 'NONE',  ( -0.000000000000000000, -1.000000000000000000, -0.000000000000000000 ) ) ;
#67793=EDGE_CURVE ( 'NONE', #88979, #90692, #88051, .T. ) ;
#67798=ORIENTED_EDGE ( 'NONE', *, *, #97234, .F. ) ;
#67800=VERTEX_POINT ( 'NONE', #87563 ) ;
#67806=ORIENTED_EDGE ( 'NONE', *, *, #54217, .F. ) ;
#67810=ORIENTED_EDGE ( 'NONE', *, *, #81770, .T. ) ;
#67818=CARTESIAN_POINT ( 'NONE',  ( -14.35840480524203144, 15.00000000000000000, 4.340070442838751319 ) ) ;
#67824=VERTEX_POINT ( 'NONE', #82031 ) ;
#67836=AXIS2_PLACEMENT_3D ( 'NONE', #44278, #74782, #14799 ) ;
#67837=CARTESIAN_POINT ( 'NONE',  ( 14.94699059465101776, 0.5000000000000004441, -1.259949270174818059 ) ) ;
#67842=EDGE_CURVE ( 'NONE', #20604, #64886, #52036, .T. ) ;
#67845=EDGE_LOOP ( 'NONE', ( #1657, #15019, #54615, #88615, #71882, #19830 ) ) ;
#67864=CARTESIAN_POINT ( 'NONE',  ( 9.820177974736324700, 0.2301504389881812163, 11.25994418464059343 ) ) ;
#67874=CARTESIAN_POINT ( 'NONE',  ( -14.03351048042399007, 15.00000000000000000, 2.474486531753619989 ) ) ;
#67877=EDGE_CURVE ( 'NONE', #70287, #11472, #67537, .T. ) ;
#67886=CARTESIAN_POINT ( 'NONE',  ( 0.000000000000000000, 14.49999999999999822, 0.000000000000000000 ) ) ;
#67887=CARTESIAN_POINT ( 'NONE',  ( -13.61464873478158211, 15.00000000000000000, -6.296136897218027606 ) ) ;
#67891=DIRECTION ( 'NONE',  ( -0.6626200482157408311, 0.000000000000000000, 0.7489557207889990798 ) ) ;
#67917=ORIENTED_EDGE ( 'NONE', *, *, #26548, .F. ) ;
#67925=CARTESIAN_POINT ( 'NONE',  ( -14.35840480524207585, 14.63606918001612200, 4.340070442838747766 ) ) ;
#67926=CIRCLE ( 'NONE', #4046, 15.00000000000000000 ) ;
#67927=DIRECTION ( 'NONE',  ( 0.3007057995042831666, 0.000000000000000000, -0.9537169507482237130 ) ) ;
#67933=CARTESIAN_POINT ( 'NONE',  ( -6.408140936763246032, -21.70969866340290721, -11.09922568453594316 ) ) ;
#67942=VERTEX_POINT ( 'NONE', #22046 ) ;
#67952=DIRECTION ( 'NONE',  ( -0.000000000000000000, -1.000000000000000000, -0.000000000000000000 ) ) ;
#67953=CIRCLE ( 'NONE', #2541, 15.00000000000000000 ) ;
#67959=CARTESIAN_POINT ( 'NONE',  ( -14.17193700899791153, 15.00000000000000000, 1.489530601563921808 ) ) ;
#67961=ORIENTED_EDGE ( 'NONE', *, *, #80971, .T. ) ;
#67962=CARTESIAN_POINT ( 'NONE',  ( -5.428133280998947541, 0.000000000000000000, 0.5226697871167153009 ) ) ;
#67964=AXIS2_PLACEMENT_3D ( 'NONE', #98778, #60730, #91230 ) ;
#67967=DIRECTION ( 'NONE',  ( 0.000000000000000000, 0.000000000000000000, 1.000000000000000000 ) ) ;
#67974=CARTESIAN_POINT ( 'NONE',  ( 14.02068044289378967, 0.5000000000000004441, -5.331089937175664595 ) ) ;
#67981=CARTESIAN_POINT ( 'NONE',  ( 11.94665733272910302, 14.76984983274819996, -8.972157519073995502 ) ) ;
#67983=CARTESIAN_POINT ( 'NONE',  ( -3.795296366450300773, -17.15458449841936073, 14.16423886937410437 ) ) ;
#67984=AXIS2_PLACEMENT_3D ( 'NONE', #71104, #2136, #94089 ) ;
#67989=EDGE_CURVE ( 'NONE', #75294, #43658, #91823, .T. ) ;
#67990=EDGE_LOOP ( 'NONE', ( #55511, #1275, #69173, #87931, #93547, #72346 ) ) ;
#67991=ADVANCED_FACE ( 'NONE', ( #50552 ), #2719, .T. ) ;
#67997=B_SPLINE_CURVE_WITH_KNOTS ( 'NONE', 3,
 ( #38266, #290, #91749, #53745, #84263, #57174 ),
 .UNSPECIFIED., .F., .F.,
 ( 4, 2, 4 ),
 ( 3.409110551496124592E-05, 0.0004400426677367849453, 0.0008459942299586086650 ),
 .UNSPECIFIED. ) ;
#67998=LINE ( 'NONE', #21017, #65587 ) ;
#68000=CARTESIAN_POINT ( 'NONE',  ( -6.741983435833344807, 0.04922511925147134149, -13.12218577464097180 ) ) ;
#68002=CARTESIAN_POINT ( 'NONE',  ( 10.88017736071110164, 25.35535201082151957, 2.915334737309921209 ) ) ;
#68007=LINE ( 'NONE', #82007, #12091 ) ;
#68012=AXIS2_PLACEMENT_3D ( 'NONE', #62432, #54446, #38974 ) ;
#68017=DIRECTION ( 'NONE',  ( 0.000000000000000000, 0.000000000000000000, 1.000000000000000000 ) ) ;
#68026=DIRECTION ( 'NONE',  ( -0.000000000000000000, -1.000000000000000000, -0.000000000000000000 ) ) ;
#68030=DIRECTION ( 'NONE',  ( 0.000000000000000000, 0.000000000000000000, 1.000000000000000000 ) ) ;
#68032=CARTESIAN_POINT ( 'NONE',  ( 12.03768810259485100, -3.163668057994810583E-15, -8.306778944023331945 ) ) ;
#68036=ORIENTED_EDGE ( 'NONE', *, *, #54184, .T. ) ;
#68042=CARTESIAN_POINT ( 'NONE',  ( 2.815433093577111467, 14.49999999999999112, -14.73340885523756683 ) ) ;
#68047=LINE ( 'NONE', #44044, #1357 ) ;
#68050=CARTESIAN_POINT ( 'NONE',  ( -9.846743663894590881, 21.21726448433412315, 2.638427012816840111 ) ) ;
#68054=ORIENTED_EDGE ( 'NONE', *, *, #74548, .F. ) ;
#68061=CIRCLE ( 'NONE', #93588, 15.00000000000000000 ) ;
#68062=AXIS2_PLACEMENT_3D ( 'NONE', #89357, #98372, #90830 ) ;
#68063=VECTOR ( 'NONE', #9877, 1000.000000000000227 ) ;
#68066=ORIENTED_EDGE ( 'NONE', *, *, #5923, .F. ) ;
#68070=VERTEX_POINT ( 'NONE', #96567 ) ;
#68079=LINE ( 'NONE', #69062, #9025 ) ;
#68080=ORIENTED_EDGE ( 'NONE', *, *, #29023, .F. ) ;
#68085=DIRECTION ( 'NONE',  ( 0.000000000000000000, 0.000000000000000000, 1.000000000000000000 ) ) ;
#68089=CARTESIAN_POINT ( 'NONE',  ( -8.439016546559974685, 15.00000000000000000, 11.79122553964965014 ) ) ;
#68091=CARTESIAN_POINT ( 'NONE',  ( -11.81378540890925066, -0.03417435944610275333, -7.968498874458281200 ) ) ;
#68094=DIRECTION ( 'NONE',  ( -0.9999619230641713097, 0.000000000000000000, 0.008726535498367547425 ) ) ;
#68100=DIRECTION ( 'NONE',  ( 0.000000000000000000, 0.000000000000000000, 1.000000000000000000 ) ) ;
#68102=B_SPLINE_CURVE_WITH_KNOTS ( 'NONE', 3,
 ( #85289, #94249, #1324, #9286, #69801, #32265 ),
 .UNSPECIFIED., .F., .F.,
 ( 4, 2, 4 ),
 ( 0.0002800086601590456403, 0.0006862139742846182309, 0.001092419288410190767 ),
 .UNSPECIFIED. ) ;
#68103=DIRECTION ( 'NONE',  ( 0.000000000000000000, -1.000000000000000000, 0.000000000000000000 ) ) ;
#68104=ADVANCED_FACE ( 'NONE', ( #28042 ), #37540, .F. ) ;
#68105=ORIENTED_EDGE ( 'NONE', *, *, #20646, .T. ) ;
#68106=ORIENTED_EDGE ( 'NONE', *, *, #1822, .F. ) ;
#68112=CARTESIAN_POINT ( 'NONE',  ( 0.000000000000000000, 0.000000000000000000, 0.000000000000000000 ) ) ;
#68115=CARTESIAN_POINT ( 'NONE',  ( -13.95697193428306093, -2.793938176518308880E-15, -4.371663894959005425 ) ) ;
#68119=CARTESIAN_POINT ( 'NONE',  ( -10.88017736071110164, -17.14464798917848753, -2.915334737309917212 ) ) ;
#68123=B_SPLINE_CURVE_WITH_KNOTS ( 'NONE', 3,
 ( #95618, #35094, #65592, #29077, #43100, #97122 ),
 .UNSPECIFIED., .F., .F.,
 ( 4, 2, 4 ),
 ( 3.409110551496115105E-05, 0.0004400426677367873306, 0.0008459942299586134355 ),
 .UNSPECIFIED. ) ;
#68124=DIRECTION ( 'NONE',  ( 0.000000000000000000, 0.000000000000000000, 1.000000000000000000 ) ) ;
#68126=DIRECTION ( 'NONE',  ( 0.9304175679820206879, 0.000000000000000000, 0.3665012267243071831 ) ) ;
#68137=AXIS2_PLACEMENT_3D ( 'NONE', #9558, #17570, #70559 ) ;
#68146=DIRECTION ( 'NONE',  ( 0.000000000000000000, 0.000000000000000000, 1.000000000000000000 ) ) ;
#68149=AXIS2_PLACEMENT_3D ( 'NONE', #82442, #28937, #75930 ) ;
#68152=TOROIDAL_SURFACE ( 'NONE', #34576, 14.49999999999999822, 0.5000000000000000000 ) ;
#68153=ORIENTED_EDGE ( 'NONE', *, *, #80948, .T. ) ;
#68154=VERTEX_POINT ( 'NONE', #46020 ) ;
#68157=VECTOR ( 'NONE', #31555, 1000.000000000000114 ) ;
#68171=CARTESIAN_POINT ( 'NONE',  ( -4.923371831947302546, -19.82440218233254114, -8.527530157486173934 ) ) ;
#68176=ORIENTED_EDGE ( 'NONE', *, *, #73953, .T. ) ;
#68177=CARTESIAN_POINT ( 'NONE',  ( -0.8217048220046814233, 0.04962895218885818305, 14.73031263975986249 ) ) ;
#68183=CARTESIAN_POINT ( 'NONE',  ( -2.120353041430744323, 15.00000000000000000, 14.34413130794943925 ) ) ;
#68185=CARTESIAN_POINT ( 'NONE',  ( -12.81628187352647608, 19.12363466993041783, 3.903127820947815962E-15 ) ) ;
#68191=EDGE_LOOP ( 'NONE', ( #7366, #3623, #47035, #71725, #53030, #78637 ) ) ;
#68201=ORIENTED_EDGE ( 'NONE', *, *, #31687, .F. ) ;
#68220=B_SPLINE_CURVE_WITH_KNOTS ( 'NONE', 3,
 ( #42021, #72485, #49489, #49006, #26499, #17548 ),
 .UNSPECIFIED., .F., .F.,
 ( 4, 2, 4 ),
 ( 0.0002800001862106003543, 0.0006862054174524986287, 0.001092410648694397066 ),
 .UNSPECIFIED. ) ;
#68223=AXIS2_PLACEMENT_3D ( 'NONE', #72959, #49969, #33475 ) ;
#68230=PLANE ( 'NONE',  #23588 ) ;
#68231=EDGE_CURVE ( 'NONE', #81191, #51046, #55520, .T. ) ;
#68233=ORIENTED_EDGE ( 'NONE', *, *, #60838, .T. ) ;
#68238=EDGE_CURVE ( 'NONE', #84641, #30081, #9184, .T. ) ;
#68239=CARTESIAN_POINT ( 'NONE',  ( -7.595945211628415628, 4.258289072137175049E-16, 12.35117874301636398 ) ) ;
#68240=CARTESIAN_POINT ( 'NONE',  ( 5.963430220938279902, 5.995456701841144209, -10.32896413005680181 ) ) ;
#68245=CARTESIAN_POINT ( 'NONE',  ( 3.795296366450306547, 20.34541550158063572, -14.16423886937410259 ) ) ;
#68248=CARTESIAN_POINT ( 'NONE',  ( -14.88232117145528655, 0.5000000000000004441, -1.875237731503337946 ) ) ;
#68252=ORIENTED_EDGE ( 'NONE', *, *, #23797, .T. ) ;
#68257=DIRECTION ( 'NONE',  ( -0.000000000000000000, -1.000000000000000000, -0.000000000000000000 ) ) ;
#68280=CARTESIAN_POINT ( 'NONE',  ( -9.159723438033054776, 15.00000000000000000, -10.91613331444555079 ) ) ;
#68290=CYLINDRICAL_SURFACE ( 'NONE', #73049, 15.00000000000000000 ) ;
#68296=ORIENTED_EDGE ( 'NONE', *, *, #98268, .F. ) ;
#68298=EDGE_LOOP ( 'NONE', ( #7596, #79361, #56652, #43336, #88236, #98188 ) ) ;
#68303=ORIENTED_EDGE ( 'NONE', *, *, #13850, .F. ) ;
#68310=DIRECTION ( 'NONE',  ( -0.9935718556765877896, 0.000000000000000000, 0.1132032137679039180 ) ) ;
#68311=EDGE_CURVE ( 'NONE', #95614, #59664, #68524, .T. ) ;
#68312=CARTESIAN_POINT ( 'NONE',  ( 9.898881779040660689, -0.03417435944610275333, 10.25059215482582786 ) ) ;
#68315=ADVANCED_FACE ( 'NONE', ( #18347 ), #4418, .T. ) ;
#68316=VERTEX_POINT ( 'NONE', #30502 ) ;
#68319=LINE ( 'NONE', #60796, #86664 ) ;
#68322=EDGE_CURVE ( 'NONE', #50188, #90286, #60291, .T. ) ;
#68324=CARTESIAN_POINT ( 'NONE',  ( 1.377727649040772586E-15, 12.49999999999999112, -11.25000000000000178 ) ) ;
#68334=LINE ( 'NONE', #38332, #2419 ) ;
#68345=ORIENTED_EDGE ( 'NONE', *, *, #65812, .F. ) ;
#68346=DIRECTION ( 'NONE',  ( -0.000000000000000000, 1.000000000000000000, -0.000000000000000000 ) ) ;
#68350=B_SPLINE_CURVE_WITH_KNOTS ( 'NONE', 3,
 ( #51898, #20912, #52874, #44872, #67388, #58389 ),
 .UNSPECIFIED., .F., .F.,
 ( 4, 2, 4 ),
 ( 0.0002800039672440407979, 0.0006862092354666064070, 0.001092414503689172070 ),
 .UNSPECIFIED. ) ;
#68358=LINE ( 'NONE', #98876, #18653 ) ;
#68362=CARTESIAN_POINT ( 'NONE',  ( -12.87930560075664488, 0.04962897030442339763, -7.195887444332561778 ) ) ;
#68363=EDGE_CURVE ( 'NONE', #55365, #50602, #61004, .T. ) ;
#68370=DIRECTION ( 'NONE',  ( 0.000000000000000000, 1.000000000000000000, 0.000000000000000000 ) ) ;
#68379=CARTESIAN_POINT ( 'NONE',  ( -14.62129639376010637, -3.201784540621254098E-15, -0.3552502084987199105 ) ) ;
#68384=PLANE ( 'NONE',  #16046 ) ;
#68388=CARTESIAN_POINT ( 'NONE',  ( 5.240693273022541732, 14.95037116783232456, -13.79102773478290622 ) ) ;
#68389=PLANE ( 'NONE',  #89812 ) ;
#68405=EDGE_LOOP ( 'NONE', ( #30563, #3247, #45797, #19884, #67693, #47354 ) ) ;
#68407=EDGE_CURVE ( 'NONE', #67262, #43658, #23032, .T. ) ;
#68414=CARTESIAN_POINT ( 'NONE',  ( -5.056330833731841778, 4.586016791640643039E-16, 13.58983143750696421 ) ) ;
#68415=CARTESIAN_POINT ( 'NONE',  ( 14.62617646268094518, 14.49999999999999112, -3.327906561566873478 ) ) ;
#68423=EDGE_LOOP ( 'NONE', ( #90424, #63365, #50467, #70766, #14684, #34059 ) ) ;
#68425=CARTESIAN_POINT ( 'NONE',  ( -5.204170427930421283E-15, -2.126365330069574178, -12.81628187352647608 ) ) ;
#68436=VECTOR ( 'NONE', #39029, 1000.000000000000000 ) ;
#68440=EDGE_LOOP ( 'NONE', ( #81697, #35937, #14099, #50021 ) ) ;
#68446=ORIENTED_EDGE ( 'NONE', *, *, #44284, .F. ) ;
#68454=CARTESIAN_POINT ( 'NONE',  ( -8.209432707284705089, 14.63595249122789177, -12.55409154915497538 ) ) ;
#68457=VERTEX_POINT ( 'NONE', #11325 ) ;
#68460=EDGE_CURVE ( 'NONE', #1436, #37674, #3342, .T. ) ;
#68472=CARTESIAN_POINT ( 'NONE',  ( -4.289191146912808207E-15, 8.868033628982656680, -11.25000000000000178 ) ) ;
#68476=PLANE ( 'NONE',  #61075 ) ;
#68481=CARTESIAN_POINT ( 'NONE',  ( 3.795296366450306547, -14.65458449841936428, -14.16423886937410259 ) ) ;
#68485=EDGE_LOOP ( 'NONE', ( #41251, #65391, #77707, #78191, #4201, #61608 ) ) ;
#68488=DIRECTION ( 'NONE',  ( -0.9914448613738093830, 0.000000000000000000, -0.1305261922200583180 ) ) ;
#68491=LINE ( 'NONE', #44493, #88011 ) ;
#68497=CARTESIAN_POINT ( 'NONE',  ( -10.88017736071110164, 32.85535201082151957, -2.915334737309917212 ) ) ;
#68506=VECTOR ( 'NONE', #80729, 1000.000000000000000 ) ;
#68514=ORIENTED_EDGE ( 'NONE', *, *, #58254, .T. ) ;
#68516=CARTESIAN_POINT ( 'NONE',  ( 0.000000000000000000, 14.49999999999999822, 0.000000000000000000 ) ) ;
#68524=LINE ( 'NONE', #91006, #25196 ) ;
#68526=DIRECTION ( 'NONE',  ( -0.7604059656000257128, 0.000000000000000000, -0.6494480483301898754 ) ) ;
#68527=EDGE_CURVE ( 'NONE', #23491, #87709, #11816, .T. ) ;
#68530=LINE ( 'NONE', #59, #39226 ) ;
#68544=CARTESIAN_POINT ( 'NONE',  ( 8.527530157486175710, 18.92559781766745175, -4.923371831947298993 ) ) ;
#68548=DIRECTION ( 'NONE',  ( -0.000000000000000000, -1.000000000000000000, -0.000000000000000000 ) ) ;
#68560=EDGE_CURVE ( 'NONE', #3454, #48192, #58791, .T. ) ;
#68562=ORIENTED_EDGE ( 'NONE', *, *, #69340, .T. ) ;
#68573=ORIENTED_EDGE ( 'NONE', *, *, #77588, .F. ) ;
#68575=EDGE_LOOP ( 'NONE', ( #28463, #31888, #35807, #44049, #85256, #58732 ) ) ;
#68578=CIRCLE ( 'NONE', #40034, 14.49999999999999822 ) ;
#68593=AXIS2_PLACEMENT_3D ( 'NONE', #71944, #87439, #85485 ) ;
#68598=ORIENTED_EDGE ( 'NONE', *, *, #37160, .F. ) ;
#68607=FACE_OUTER_BOUND ( 'NONE', #67295, .T. ) ;
#68610=CARTESIAN_POINT ( 'NONE',  ( 10.88017736071110164, -9.644647989178485759, 2.915334737309921209 ) ) ;
#68614=DIRECTION ( 'NONE',  ( -0.5519369853120617009, 0.000000000000000000, 0.8338858220671657717 ) ) ;
#68616=CARTESIAN_POINT ( 'NONE',  ( 13.96552416078066550, 0.04962884865031113452, -4.756200848675081971 ) ) ;
#68624=FACE_OUTER_BOUND ( 'NONE', #58983, .T. ) ;
#68639=ORIENTED_EDGE ( 'NONE', *, *, #74061, .T. ) ;
#68654=AXIS2_PLACEMENT_3D ( 'NONE', #83375, #92349, #98408 ) ;
#68655=CARTESIAN_POINT ( 'NONE',  ( -4.923371831947302546, -29.82440218233254470, -8.527530157486173934 ) ) ;
#68656=EDGE_LOOP ( 'NONE', ( #86238, #51876, #73095, #76772 ) ) ;
#68658=ORIENTED_EDGE ( 'NONE', *, *, #49456, .T. ) ;
#68661=AXIS2_PLACEMENT_3D ( 'NONE', #83302, #7316, #13327 ) ;
#68671=CARTESIAN_POINT ( 'NONE',  ( 3.434112377981060948, 25.58196800326376419, 12.81628187352647430 ) ) ;
#68681=DIRECTION ( 'NONE',  ( 0.9996573249755575929, 0.000000000000000000, -0.02617694830786282401 ) ) ;
#68696=VERTEX_POINT ( 'NONE', #50810 ) ;
#68698=DIRECTION ( 'NONE',  ( 0.000000000000000000, 1.000000000000000000, 0.000000000000000000 ) ) ;
#68707=EDGE_CURVE ( 'NONE', #63596, #3959, #39539, .T. ) ;
#68709=CARTESIAN_POINT ( 'NONE',  ( 0.8217048220045788387, 0.04962895218885213927, -14.73031263975987493 ) ) ;
#68714=AXIS2_PLACEMENT_3D ( 'NONE', #55952, #69475, #46955 ) ;
#68717=DIRECTION ( 'NONE',  ( -0.000000000000000000, -1.000000000000000000, -0.000000000000000000 ) ) ;
#68718=ADVANCED_FACE ( 'NONE', ( #89298 ), #3841, .F. ) ;
#68720=CARTESIAN_POINT ( 'NONE',  ( 13.14228782657339956, 0.5000000000000004441, -7.230509711182238064 ) ) ;
#68721=VECTOR ( 'NONE', #15391, 1000.000000000000114 ) ;
#68727=CARTESIAN_POINT ( 'NONE',  ( -3.795296366450322534, 15.76208216824730535, -14.16423886937409904 ) ) ;
#68759=LINE ( 'NONE', #30736, #9607 ) ;
#68762=EDGE_CURVE ( 'NONE', #39241, #92547, #14259, .T. ) ;
#68763=ORIENTED_EDGE ( 'NONE', *, *, #46851, .F. ) ;
#68764=EDGE_LOOP ( 'NONE', ( #1687, #6818, #87427, #38054, #83330, #15304 ) ) ;
#68766=CARTESIAN_POINT ( 'NONE',  ( -14.61046065509106029, -3.236089374985053262E-15, 0.6655452423541795559 ) ) ;
#68774=ADVANCED_FACE ( 'NONE', ( #60763 ), #68290, .T. ) ;
#68794=EDGE_LOOP ( 'NONE', ( #85239, #57322, #97874, #43895 ) ) ;
#68799=CIRCLE ( 'NONE', #87899, 14.49999999999999822 ) ;
#68808=ORIENTED_EDGE ( 'NONE', *, *, #57584, .F. ) ;
#68815=LINE ( 'NONE', #60316, #30721 ) ;
#68826=DIRECTION ( 'NONE',  ( -0.000000000000000000, -1.000000000000000000, -0.000000000000000000 ) ) ;
#68832=CARTESIAN_POINT ( 'NONE',  ( -0.7375392941516148992, 0.3640475087720989045, -14.98185688723471998 ) ) ;
#68837=ORIENTED_EDGE ( 'NONE', *, *, #1199, .F. ) ;
#68853=TOROIDAL_SURFACE ( 'NONE', #22607, 14.49999999999999822, 0.5000000000000000000 ) ;
#68856=ORIENTED_EDGE ( 'NONE', *, *, #42681, .T. ) ;
#68868=VERTEX_POINT ( 'NONE', #98312 ) ;
#68876=CARTESIAN_POINT ( 'NONE',  ( 14.97687855664611689, 0.3639309658595352159, -0.8325315005900656429 ) ) ;
#68881=PLANE ( 'NONE',  #91465 ) ;
#68889=EDGE_CURVE ( 'NONE', #4994, #89266, #23287, .T. ) ;
#68903=AXIS2_PLACEMENT_3D ( 'NONE', #57390, #40935, #10916 ) ;
#68909=CARTESIAN_POINT ( 'NONE',  ( 0.000000000000000000, 0.5000000000000004441, 0.000000000000000000 ) ) ;
#68910=AXIS2_PLACEMENT_3D ( 'NONE', #62931, #93433, #24955 ) ;
#68915=CARTESIAN_POINT ( 'NONE',  ( 10.19513985507833276, 0.5000000000000004441, -11.00268709613217055 ) ) ;
#68918=EDGE_CURVE ( 'NONE', #50302, #72594, #45951, .T. ) ;
#68930=ORIENTED_EDGE ( 'NONE', *, *, #59162, .T. ) ;
#68957=LINE ( 'NONE', #69445, #38211 ) ;
#68960=B_SPLINE_CURVE_WITH_KNOTS ( 'NONE', 3,
 ( #22447, #37452, #1431, #52920, #14953, #933 ),
 .UNSPECIFIED., .F., .F.,
 ( 4, 2, 4 ),
 ( 0.0002800289709865070556, 0.0006862344838253337225, 0.001092439996664160444 ),
 .UNSPECIFIED. ) ;
#68966=EDGE_CURVE ( 'NONE', #71703, #74605, #93900, .T. ) ;
#68967=CARTESIAN_POINT ( 'NONE',  ( -9.820682251645022731, 14.76930270348881002, -11.26020669458372758 ) ) ;
#68970=CARTESIAN_POINT ( 'NONE',  ( -7.082119434687044190, -7.362917831752691100, 12.26659068614894998 ) ) ;
#68975=ORIENTED_EDGE ( 'NONE', *, *, #5973, .T. ) ;
#68983=CARTESIAN_POINT ( 'NONE',  ( -0.7575892234032817196, 14.76930270348881002, 14.92193396517713033 ) ) ;
#68997=AXIS2_PLACEMENT_3D ( 'NONE', #14215, #67206, #13710 ) ;
#68998=ADVANCED_FACE ( 'NONE', ( #62236 ), #76286, .T. ) ;
#69001=EDGE_CURVE ( 'NONE', #15586, #73495, #52315, .T. ) ;
#69008=ORIENTED_EDGE ( 'NONE', *, *, #83306, .T. ) ;
#69013=TOROIDAL_SURFACE ( 'NONE', #25891, 14.49999999999999822, 0.5000000000000000000 ) ;
#69023=ORIENTED_EDGE ( 'NONE', *, *, #75348, .F. ) ;
#69028=CARTESIAN_POINT ( 'NONE',  ( -14.03351048042399007, 15.00000000000000000, 2.474486531753619989 ) ) ;
#69035=EDGE_CURVE ( 'NONE', #85150, #17634, #78525, .T. ) ;
#69037=CARTESIAN_POINT ( 'NONE',  ( 3.469446951953614189E-15, -39.62636533006958217, 12.81628187352647608 ) ) ;
#69038=ORIENTED_EDGE ( 'NONE', *, *, #54183, .F. ) ;
#69040=ORIENTED_EDGE ( 'NONE', *, *, #35822, .F. ) ;
#69052=ORIENTED_EDGE ( 'NONE', *, *, #37290, .F. ) ;
#69054=ORIENTED_EDGE ( 'NONE', *, *, #18993, .T. ) ;
#69060=CARTESIAN_POINT ( 'NONE',  ( -5.056330833731841778, 15.00000000000000000, 13.58983143750696421 ) ) ;
#69062=CARTESIAN_POINT ( 'NONE',  ( 8.134956207566084174, 15.00000000000000000, -13.77315809598639085 ) ) ;
#69063=VECTOR ( 'NONE', #75878, 1000.000000000000000 ) ;
#69069=VECTOR ( 'NONE', #31776, 1000.000000000000114 ) ;
#69074=CARTESIAN_POINT ( 'NONE',  ( -3.420591144908684988, 14.49999999999999112, 14.60477854057959313 ) ) ;
#69084=DIRECTION ( 'NONE',  ( -0.3502073812594621582, 0.000000000000000000, -0.9366721892483996781 ) ) ;
#69087=FACE_OUTER_BOUND ( 'NONE', #14718, .T. ) ;
#69089=ORIENTED_EDGE ( 'NONE', *, *, #59238, .T. ) ;
#69090=ORIENTED_EDGE ( 'NONE', *, *, #47851, .T. ) ;
#69102=CARTESIAN_POINT ( 'NONE',  ( -5.440088680355558814, -12.76964798917849109, -9.422509992056136596 ) ) ;
#69109=VECTOR ( 'NONE', #23321, 1000.000000000000227 ) ;
#69120=VERTEX_POINT ( 'NONE', #25257 ) ;
#69123=CARTESIAN_POINT ( 'NONE',  ( 1.909764518474464046, 0.000000000000000000, -5.107897229450591325 ) ) ;
#69129=CARTESIAN_POINT ( 'NONE',  ( 0.8217048220044697038, 14.95037104781115467, 14.73031263975989269 ) ) ;
#69132=AXIS2_PLACEMENT_3D ( 'NONE', #46847, #62335, #15882 ) ;
#69135=ORIENTED_EDGE ( 'NONE', *, *, #38319, .F. ) ;
#69136=ORIENTED_EDGE ( 'NONE', *, *, #18083, .T. ) ;
#69153=CARTESIAN_POINT ( 'NONE',  ( -7.208316651077756099, -8.366068848999207219, 7.208316651077766757 ) ) ;
#69156=CIRCLE ( 'NONE', #48439, 15.00000000000000000 ) ;
#69168=CARTESIAN_POINT ( 'NONE',  ( -3.434112377981047626, 25.16530133659708213, 12.81628187352647963 ) ) ;
#69169=ORIENTED_EDGE ( 'NONE', *, *, #21116, .T. ) ;
#69171=ORIENTED_EDGE ( 'NONE', *, *, #85151, .T. ) ;
#69173=ORIENTED_EDGE ( 'NONE', *, *, #43710, .T. ) ;
#69182=CARTESIAN_POINT ( 'NONE',  ( -7.551349515323269479, 0.000000000000000000, 12.08468537022900868 ) ) ;
#69184=CARTESIAN_POINT ( 'NONE',  ( 0.000000000000000000, 0.000000000000000000, 0.000000000000000000 ) ) ;
#69187=EDGE_LOOP ( 'NONE', ( #55253, #77392, #10247, #7806 ) ) ;
#69194=DIRECTION ( 'NONE',  ( 0.000000000000000000, 1.000000000000000000, 0.000000000000000000 ) ) ;
#69198=CARTESIAN_POINT ( 'NONE',  ( 13.82192141328812518, 15.00000000000000000, -4.382292601468683380 ) ) ;
#69206=CARTESIAN_POINT ( 'NONE',  ( -10.32896413005679470, 8.078790035174483464, 5.963430220938290560 ) ) ;
#69209=DIRECTION ( 'NONE',  ( -4.529709940470638685E-14, 0.000000000000000000, 1.000000000000000000 ) ) ;
#69217=LINE ( 'NONE', #67741, #20786 ) ;
#69221=CARTESIAN_POINT ( 'NONE',  ( 12.26659068614894821, 23.88708216824731068, 7.082119434687044190 ) ) ;
#69226=B_SPLINE_CURVE_WITH_KNOTS ( 'NONE', 3,
 ( #6230, #29210, #66219, #97251, #65227, #89228 ),
 .UNSPECIFIED., .F., .F.,
 ( 4, 2, 4 ),
 ( 3.409110551496067671E-05, 0.0004400426677367857043, 0.0008459942299586107250 ),
 .UNSPECIFIED. ) ;
#69233=EDGE_CURVE ( 'NONE', #26361, #22285, #50798, .T. ) ;
#69242=B_SPLINE_CURVE_WITH_KNOTS ( 'NONE', 3,
 ( #44873, #29378, #45374, #98909, #82886, #75376 ),
 .UNSPECIFIED., .F., .F.,
 ( 4, 2, 4 ),
 ( 3.409110551494644656E-05, 0.0004400426677367928600, 0.0008459942299586393480 ),
 .UNSPECIFIED. ) ;
#69244=ORIENTED_EDGE ( 'NONE', *, *, #6804, .T. ) ;
#69247=CARTESIAN_POINT ( 'NONE',  ( 14.62617646268092031, 14.63606916781938772, -3.327906561566877919 ) ) ;
#69267=CARTESIAN_POINT ( 'NONE',  ( 11.35178980618974975, 0.3640475087720984604, -9.804941009311923139 ) ) ;
#69271=CARTESIAN_POINT ( 'NONE',  ( -12.00809552683947068, 14.63595249122795394, -8.989195838243713155 ) ) ;
#69276=CARTESIAN_POINT ( 'NONE',  ( 13.82671409943296226, 15.00000000000000000, -3.447387012295225261 ) ) ;
#69282=ADVANCED_FACE ( 'NONE', ( #80195 ), #98721, .T. ) ;
#69286=TOROIDAL_SURFACE ( 'NONE', #48494, 14.49999999999999822, 0.5000000000000000000 ) ;
#69287=ORIENTED_EDGE ( 'NONE', *, *, #11863, .T. ) ;
#69291=EDGE_LOOP ( 'NONE', ( #90923, #74066, #18238, #73237, #10263, #35769 ) ) ;
#69294=DIRECTION ( 'NONE',  ( -0.000000000000000000, -1.000000000000000000, -0.000000000000000000 ) ) ;
#69297=ORIENTED_EDGE ( 'NONE', *, *, #23694, .F. ) ;
#69310=CARTESIAN_POINT ( 'NONE',  ( -2.261421327065682441, 0.000000000000000000, -4.962236210031271355 ) ) ;
#69334=DIRECTION ( 'NONE',  ( 0.000000000000000000, 1.000000000000000000, 0.000000000000000000 ) ) ;
#69340=EDGE_CURVE ( 'NONE', #51116, #59690, #60347, .T. ) ;
#69341=CIRCLE ( 'NONE', #19865, 14.49999999999999822 ) ;
#69344=CARTESIAN_POINT ( 'NONE',  ( 5.451370222425311773, 0.000000000000000000, -0.1427491530890097615 ) ) ;
#69354=AXIS2_PLACEMENT_3D ( 'NONE', #75981, #44983, #74996 ) ;
#69356=CARTESIAN_POINT ( 'NONE',  ( -14.49440716394873085, 4.311470567659570904E-16, -0.4026921475168178111 ) ) ;
#69361=CARTESIAN_POINT ( 'NONE',  ( 10.19513985507833453, 14.63595249122788999, -11.00268709613217943 ) ) ;
#69382=ORIENTED_EDGE ( 'NONE', *, *, #9140, .F. ) ;
#69384=ORIENTED_EDGE ( 'NONE', *, *, #51023, .F. ) ;
#69389=ORIENTED_EDGE ( 'NONE', *, *, #25883, .F. ) ;
#69411=ORIENTED_EDGE ( 'NONE', *, *, #37450, .F. ) ;
#69417=ORIENTED_EDGE ( 'NONE', *, *, #87477, .F. ) ;
#69418=ORIENTED_EDGE ( 'NONE', *, *, #17393, .T. ) ;
#69431=EDGE_LOOP ( 'NONE', ( #37801, #90196, #96948, #33622, #62382, #74077 ) ) ;
#69432=CARTESIAN_POINT ( 'NONE',  ( -4.289191146912808207E-15, 3.868033628982651795, -11.25000000000000178 ) ) ;
#69435=EDGE_CURVE ( 'NONE', #1179, #86906, #58316, .T. ) ;
#69438=ADVANCED_FACE ( 'NONE', ( #56235 ), #41729, .F. ) ;
#69445=CARTESIAN_POINT ( 'NONE',  ( 5.418184704451237899, 0.000000000000000000, 0.6173241701923447566 ) ) ;
#69451=CARTESIAN_POINT ( 'NONE',  ( 0.000000000000000000, 15.00000000000000000, 14.25000000000000000 ) ) ;
#69452=CARTESIAN_POINT ( 'NONE',  ( -12.34086200392831678, -0.03417435944610275333, 7.124999999999885425 ) ) ;
#69454=CARTESIAN_POINT ( 'NONE',  ( 0.000000000000000000, 0.000000000000000000, 0.000000000000000000 ) ) ;
#69457=CARTESIAN_POINT ( 'NONE',  ( 7.082119434687047743, -9.862917831752692877, -12.26659068614894821 ) ) ;
#69473=DIRECTION ( 'NONE',  ( 0.000000000000000000, 0.000000000000000000, -1.000000000000000000 ) ) ;
#69475=DIRECTION ( 'NONE',  ( 0.000000000000000000, 1.000000000000000000, 0.000000000000000000 ) ) ;
#69483=ORIENTED_EDGE ( 'NONE', *, *, #76326, .T. ) ;
#69489=B_SPLINE_CURVE_WITH_KNOTS ( 'NONE', 3,
 ( #91357, #98898, #83862, #44863, #30852, #91858 ),
 .UNSPECIFIED., .F., .F.,
 ( 4, 2, 4 ),
 ( 3.409110551461945796E-05, 0.0004400426677364667862, 0.0008459942299583140873 ),
 .UNSPECIFIED. ) ;
#69491=VECTOR ( 'NONE', #65844, 1000.000000000000000 ) ;
#69499=DIRECTION ( 'NONE',  ( -0.000000000000000000, 1.000000000000000000, 0.000000000000000000 ) ) ;
#69512=VERTEX_POINT ( 'NONE', #81184 ) ;
#69518=CARTESIAN_POINT ( 'NONE',  ( -13.34948392230381309, 0.04922511925147153578, 6.279918722514886475 ) ) ;
#69524=DIRECTION ( 'NONE',  ( 0.2503800040544526539, 0.000000000000000000, -0.9681476403781048568 ) ) ;
#69527=CARTESIAN_POINT ( 'NONE',  ( -9.382169495545413795, -40.25136533006956796, 9.382169495545428006 ) ) ;
#69538=TOROIDAL_SURFACE ( 'NONE', #26403, 14.49999999999999822, 0.5000000000000000000 ) ;
#69540=VERTEX_POINT ( 'NONE', #87203 ) ;
#69548=DIRECTION ( 'NONE',  ( -0.7253743710122820820, 0.000000000000000000, -0.6883545756937599069 ) ) ;
#69549=AXIS2_PLACEMENT_3D ( 'NONE', #42505, #26998, #27978 ) ;
#69553=DIRECTION ( 'NONE',  ( -0.000000000000000000, -1.000000000000000000, -0.000000000000000000 ) ) ;
#69558=VERTEX_POINT ( 'NONE', #89177 ) ;
#69559=ORIENTED_EDGE ( 'NONE', *, *, #10014, .T. ) ;
#69565=CARTESIAN_POINT ( 'NONE',  ( 1.983216688680936812, 15.00000000000000000, -14.11131997956737649 ) ) ;
#69579=VERTEX_POINT ( 'NONE', #59164 ) ;
#69588=CYLINDRICAL_SURFACE ( 'NONE', #96558, 11.25000000000000178 ) ;
#69591=CARTESIAN_POINT ( 'NONE',  ( 9.422509992056141925, 0.9803520108215141304, -5.440088680355554374 ) ) ;
#69593=LINE ( 'NONE', #86567, #38810 ) ;
#69601=CARTESIAN_POINT ( 'NONE',  ( 7.881609424766030436, 15.00000000000000711, -12.32025747423893591 ) ) ;
#69608=ORIENTED_EDGE ( 'NONE', *, *, #69793, .T. ) ;
#69618=VECTOR ( 'NONE', #49867, 1000.000000000000114 ) ;
#69623=ORIENTED_EDGE ( 'NONE', *, *, #36889, .T. ) ;
#69635=CARTESIAN_POINT ( 'NONE',  ( 13.55255535720595184, -0.03417435944610275333, -4.403492169842965431 ) ) ;
#69637=CARTESIAN_POINT ( 'NONE',  ( -2.638427012816840111, -5.032735515665881287, -9.846743663894590881 ) ) ;
#69639=ORIENTED_EDGE ( 'NONE', *, *, #86151, .T. ) ;
#69641=VERTEX_POINT ( 'NONE', #22171 ) ;
#69642=DIRECTION ( 'NONE',  ( 0.000000000000000000, 0.000000000000000000, -1.000000000000000000 ) ) ;
#69643=ORIENTED_EDGE ( 'NONE', *, *, #95980, .F. ) ;
#69650=EDGE_CURVE ( 'NONE', #30382, #93734, #20690, .T. ) ;
#69656=ORIENTED_EDGE ( 'NONE', *, *, #54907, .T. ) ;
#69669=DIRECTION ( 'NONE',  ( -0.000000000000000000, -1.000000000000000000, -0.000000000000000000 ) ) ;
#69679=LINE ( 'NONE', #83204, #48987 ) ;
#69695=CARTESIAN_POINT ( 'NONE',  ( -9.898881779040801021, 0.000000000000000000, 10.25059215482569641 ) ) ;
#69699=DIRECTION ( 'NONE',  ( -0.000000000000000000, -1.000000000000000000, -0.000000000000000000 ) ) ;
#69701=CARTESIAN_POINT ( 'NONE',  ( 8.731067818237038480, 5.787123368507815613, -8.731067818237040257 ) ) ;
#69703=DIRECTION ( 'NONE',  ( -0.000000000000000000, -1.000000000000000000, -0.000000000000000000 ) ) ;
#69706=CARTESIAN_POINT ( 'NONE',  ( -14.16423886937410437, 26.59541550158064283, -3.795296366450299885 ) ) ;
#69710=VECTOR ( 'NONE', #57320, 999.9999999999998863 ) ;
#69713=CIRCLE ( 'NONE', #68149, 11.92686044187656513 ) ;
#69716=VECTOR ( 'NONE', #75942, 1000.000000000000000 ) ;
#69719=ORIENTED_EDGE ( 'NONE', *, *, #67640, .F. ) ;
#69724=CARTESIAN_POINT ( 'NONE',  ( 0.000000000000000000, 0.5000000000000004441, 0.000000000000000000 ) ) ;
#69729=ORIENTED_EDGE ( 'NONE', *, *, #57768, .F. ) ;
#69731=B_SPLINE_CURVE_WITH_KNOTS ( 'NONE', 3,
 ( #86452, #61465, #39479, #45990, #92945, #91972 ),
 .UNSPECIFIED., .F., .F.,
 ( 4, 2, 4 ),
 ( 0.0002800098398849580313, 0.0006862151655504416300, 0.001092420491215925337 ),
 .UNSPECIFIED. ) ;
#69747=ORIENTED_EDGE ( 'NONE', *, *, #42056, .T. ) ;
#69756=AXIS2_PLACEMENT_3D ( 'NONE', #26920, #79440, #41948 ) ;
#69764=CARTESIAN_POINT ( 'NONE',  ( -1.326261724322778557, 0.2301504087166175161, -14.88164196614427226 ) ) ;
#69765=ORIENTED_EDGE ( 'NONE', *, *, #74212, .T. ) ;
#69771=ADVANCED_FACE ( 'NONE', ( #1653 ), #93109, .T. ) ;
#69777=AXIS2_PLACEMENT_3D ( 'NONE', #75201, #45697, #22713 ) ;
#69778=ORIENTED_EDGE ( 'NONE', *, *, #8812, .F. ) ;
#69785=LINE ( 'NONE', #67818, #32227 ) ;
#69791=ORIENTED_EDGE ( 'NONE', *, *, #26636, .F. ) ;
#69792=AXIS2_PLACEMENT_3D ( 'NONE', #20508, #5016, #67486 ) ;
#69793=EDGE_CURVE ( 'NONE', #94935, #4865, #33175, .T. ) ;
#69794=DIRECTION ( 'NONE',  ( 0.000000000000000000, 1.000000000000000000, 0.000000000000000000 ) ) ;
#69796=LINE ( 'NONE', #29802, #69109 ) ;
#69801=CARTESIAN_POINT ( 'NONE',  ( 12.00809552683956305, 0.3639308727179669245, 8.989195838243638548 ) ) ;
#69812=DIRECTION ( 'NONE',  ( 0.000000000000000000, 0.000000000000000000, 1.000000000000000000 ) ) ;
#69820=ORIENTED_EDGE ( 'NONE', *, *, #52075, .F. ) ;
#69821=CARTESIAN_POINT ( 'NONE',  ( 7.771322705631503069, 15.00000000000000000, -12.24159072199917375 ) ) ;
#69829=EDGE_CURVE ( 'NONE', #83990, #26974, #45235, .T. ) ;
#69832=EDGE_CURVE ( 'NONE', #90632, #90778, #181, .T. ) ;
#69834=DIRECTION ( 'NONE',  ( 0.000000000000000000, 0.000000000000000000, 1.000000000000000000 ) ) ;
#69837=CARTESIAN_POINT ( 'NONE',  ( -5.171435456984210255, 0.000000000000000000, -1.730338099014048669 ) ) ;
#69842=CARTESIAN_POINT ( 'NONE',  ( 13.07964015051220485, 14.76930270348881180, 7.222261988160834534 ) ) ;
#69850=CARTESIAN_POINT ( 'NONE',  ( -2.888614318722539487, 15.00000000000000888, 14.33855829812819849 ) ) ;
#69860=DIRECTION ( 'NONE',  ( -0.000000000000000000, -1.000000000000000000, -0.000000000000000000 ) ) ;
#69862=DIRECTION ( 'NONE',  ( -0.9862856015372319929, 0.000000000000000000, 0.1650476058606741014 ) ) ;
#69867=AXIS2_PLACEMENT_3D ( 'NONE', #88595, #34110, #4138 ) ;
#69868=AXIS2_PLACEMENT_3D ( 'NONE', #39011, #8990, #38033 ) ;
#69871=CARTESIAN_POINT ( 'NONE',  ( 9.159723438033203990, 15.00000000000000000, -10.91613331444542645 ) ) ;
#69898=ORIENTED_EDGE ( 'NONE', *, *, #56131, .F. ) ;
#69900=TOROIDAL_SURFACE ( 'NONE', #65081, 14.49999999999999822, 0.5000000000000000000 ) ;
#69908=AXIS2_PLACEMENT_3D ( 'NONE', #12070, #33575, #96077 ) ;
#69911=CARTESIAN_POINT ( 'NONE',  ( 0.000000000000000000, 15.00000000000000000, 0.000000000000000000 ) ) ;
#69915=EDGE_CURVE ( 'NONE', #74674, #97132, #18829, .T. ) ;
#69916=VERTEX_POINT ( 'NONE', #77126 ) ;
#69917=VECTOR ( 'NONE', #47117, 999.9999999999998863 ) ;
#69921=DIRECTION ( 'NONE',  ( -0.5807029557109348872, 0.000000000000000000, -0.8141155183563226760 ) ) ;
#69927=CARTESIAN_POINT ( 'NONE',  ( 0.8218345515128016032, 0.04922511925147077944, 14.72992491912911639 ) ) ;
#69931=AXIS2_PLACEMENT_3D ( 'NONE', #2149, #76634, #84159 ) ;
#69932=CARTESIAN_POINT ( 'NONE',  ( 5.624999999999999112, 3.451366962315989717, -9.742785792574936821 ) ) ;
#69942=CARTESIAN_POINT ( 'NONE',  ( -2.827051895225590972, 14.76984989550149940, -14.67071941139717062 ) ) ;
#69943=CARTESIAN_POINT ( 'NONE',  ( 13.82671409943293739, 15.00000000000000000, 3.447387012295318076 ) ) ;
#69947=CARTESIAN_POINT ( 'NONE',  ( -12.07856007377816887, 4.482427100288500905E-16, -8.022367888855006512 ) ) ;
#69952=CARTESIAN_POINT ( 'NONE',  ( 12.26659068614894466, -5.279584498419365168, -7.082119434687053960 ) ) ;
#69958=CARTESIAN_POINT ( 'NONE',  ( -12.67147417979165525, 14.95037112956503478, -7.555862176155688559 ) ) ;
#69969=DIRECTION ( 'NONE',  ( 0.7604059656000385914, 0.000000000000000000, -0.6494480483301746654 ) ) ;
#69976=ORIENTED_EDGE ( 'NONE', *, *, #67635, .F. ) ;
#69986=DIRECTION ( 'NONE',  ( 0.000000000000000000, 0.000000000000000000, -1.000000000000000000 ) ) ;
#69988=CARTESIAN_POINT ( 'NONE',  ( 3.897244926436124857, 3.990182060915936250E-16, 13.96644127841333294 ) ) ;
#70006=ORIENTED_EDGE ( 'NONE', *, *, #33124, .F. ) ;
#70015=ADVANCED_FACE ( 'NONE', ( #10122 ), #61138, .F. ) ;
#70021=CARTESIAN_POINT ( 'NONE',  ( 2.638427012816829897, 29.55059781766745530, -9.846743663894592657 ) ) ;
#70022=VERTEX_POINT ( 'NONE', #56600 ) ;
#70032=ORIENTED_EDGE ( 'NONE', *, *, #40605, .F. ) ;
#70036=ADVANCED_FACE ( 'NONE', ( #49094 ), #41615, .T. ) ;
#70041=CARTESIAN_POINT ( 'NONE',  ( 0.000000000000000000, 14.49999999999999822, 0.000000000000000000 ) ) ;
#70046=VECTOR ( 'NONE', #98938, 1000.000000000000114 ) ;
#70049=ORIENTED_EDGE ( 'NONE', *, *, #10726, .F. ) ;
#70050=ORIENTED_EDGE ( 'NONE', *, *, #71461, .T. ) ;
#70069=EDGE_CURVE ( 'NONE', #44471, #81942, #72083, .T. ) ;
#70071=AXIS2_PLACEMENT_3D ( 'NONE', #70291, #70785, #39791 ) ;
#70075=ORIENTED_EDGE ( 'NONE', *, *, #2981, .F. ) ;
#70085=CARTESIAN_POINT ( 'NONE',  ( -5.204170427930421283E-15, -3.186314655845158494, -10.88017736071110342 ) ) ;
#70089=CARTESIAN_POINT ( 'NONE',  ( 0.000000000000000000, 0.5000000000000004441, 0.000000000000000000 ) ) ;
#70091=DIRECTION ( 'NONE',  ( 0.000000000000000000, 0.000000000000000000, 1.000000000000000000 ) ) ;
#70092=DIRECTION ( 'NONE',  ( -0.000000000000000000, -1.000000000000000000, -0.000000000000000000 ) ) ;
#70096=CARTESIAN_POINT ( 'NONE',  ( 14.17193700899790265, -0.03417435944610275333, -1.489530601564018175 ) ) ;
#70097=CARTESIAN_POINT ( 'NONE',  ( 10.32896413005680181, 11.77164270246085209, 5.963430220938278126 ) ) ;
#70103=ORIENTED_EDGE ( 'NONE', *, *, #2386, .T. ) ;
#70106=CARTESIAN_POINT ( 'NONE',  ( -12.79413655343702239, 0.2301508429231322317, 7.715718893782787191 ) ) ;
#70114=EDGE_CURVE ( 'NONE', #10914, #89676, #87577, .T. ) ;
#70117=LINE ( 'NONE', #18104, #34414 ) ;
#70118=EDGE_CURVE ( 'NONE', #42348, #24535, #49222, .T. ) ;
#70119=EDGE_LOOP ( 'NONE', ( #74126, #62356, #24547, #55399 ) ) ;
#70128=B_SPLINE_CURVE_WITH_KNOTS ( 'NONE', 3,
 ( #78073, #85581, #55578, #17095, #40078, #1114 ),
 .UNSPECIFIED., .F., .F.,
 ( 4, 2, 4 ),
 ( 3.409110551496212006E-05, 0.0004400426677368009373, 0.0008459942299586397816 ),
 .UNSPECIFIED. ) ;
#70129=EDGE_CURVE ( 'NONE', #243, #67764, #41531, .T. ) ;
#70131=EDGE_CURVE ( 'NONE', #69579, #13031, #58128, .T. ) ;
#70136=CARTESIAN_POINT ( 'NONE',  ( 2.638427012816835227, -12.53273551566588395, 9.846743663894590881 ) ) ;
#70137=ORIENTED_EDGE ( 'NONE', *, *, #8919, .F. ) ;
#70138=CARTESIAN_POINT ( 'NONE',  ( -13.82192141328807011, 3.982798640990670655E-16, -4.382292601468863680 ) ) ;
#70139=VERTEX_POINT ( 'NONE', #73059 ) ;
#70141=ORIENTED_EDGE ( 'NONE', *, *, #9036, .T. ) ;
#70147=EDGE_CURVE ( 'NONE', #79425, #41646, #96081, .T. ) ;
#70154=ORIENTED_EDGE ( 'NONE', *, *, #18708, .F. ) ;
#70166=TOROIDAL_SURFACE ( 'NONE', #19114, 14.49999999999999822, 0.5000000000000000000 ) ;
#70167=CYLINDRICAL_SURFACE ( 'NONE', #74459, 15.00000000000000000 ) ;
#70168=ORIENTED_EDGE ( 'NONE', *, *, #94080, .T. ) ;
#70181=ORIENTED_EDGE ( 'NONE', *, *, #82084, .T. ) ;
#70193=DIRECTION ( 'NONE',  ( -0.000000000000000000, -1.000000000000000000, -0.000000000000000000 ) ) ;
#70198=EDGE_CURVE ( 'NONE', #47627, #51188, #82064, .T. ) ;
#70201=CARTESIAN_POINT ( 'NONE',  ( -2.915334737309917656, -35.89464798917849464, 10.88017736071110164 ) ) ;
#70213=B_SPLINE_CURVE_WITH_KNOTS ( 'NONE', 3,
 ( #36849, #66340, #96878, #67340, #13853, #5856 ),
 .UNSPECIFIED., .F., .F.,
 ( 4, 2, 4 ),
 ( 3.409110551496207940E-05, 0.0004400426677368021299, 0.0008459942299586421669 ),
 .UNSPECIFIED. ) ;
#70220=LINE ( 'NONE', #55195, #32755 ) ;
#70225=ORIENTED_EDGE ( 'NONE', *, *, #87350, .F. ) ;
#70240=ADVANCED_FACE ( 'NONE', ( #14561 ), #6064, .F. ) ;
#70242=EDGE_LOOP ( 'NONE', ( #44165, #44911, #88499, #53283 ) ) ;
#70251=FACE_OUTER_BOUND ( 'NONE', #15180, .T. ) ;
#70256=CARTESIAN_POINT ( 'NONE',  ( -10.97221242069369218, 14.99999999999805844, 9.670525607395029866 ) ) ;
#70264=ORIENTED_EDGE ( 'NONE', *, *, #22055, .F. ) ;
#70268=CARTESIAN_POINT ( 'NONE',  ( 14.37657372141816481, 1.111307226797641650E-15, 2.693041920167452918 ) ) ;
#70271=CARTESIAN_POINT ( 'NONE',  ( 14.62129639376010815, -3.239901023247697614E-15, 0.3552502084986245423 ) ) ;
#70272=CARTESIAN_POINT ( 'NONE',  ( 3.469446951953614189E-15, 0.3736346699304282648, 12.81628187352647608 ) ) ;
#70273=VERTEX_POINT ( 'NONE', #35563 ) ;
#70277=EDGE_CURVE ( 'NONE', #339, #33071, #31653, .T. ) ;
#70287=VERTEX_POINT ( 'NONE', #37557 ) ;
#70288=CARTESIAN_POINT ( 'NONE',  ( 0.000000000000000000, 0.000000000000000000, 0.000000000000000000 ) ) ;
#70290=CARTESIAN_POINT ( 'NONE',  ( 2.393480905993059515, 14.63595249122789177, 14.80781041047753632 ) ) ;
#70291=CARTESIAN_POINT ( 'NONE',  ( 0.000000000000000000, 0.000000000000000000, 0.000000000000000000 ) ) ;
#70294=LINE ( 'NONE', #40281, #78634 ) ;
#70295=AXIS2_PLACEMENT_3D ( 'NONE', #93575, #54095, #92591 ) ;
#70300=( BOUNDED_CURVE ( )  B_SPLINE_CURVE ( 2, ( #28852, #36871, #21877, #14375, #35873, #13875, #44843, #44357, #35381 ),
 .UNSPECIFIED., .F., .F. ) 
 B_SPLINE_CURVE_WITH_KNOTS ( ( 3, 2, 2, 2, 3 ),
 ( 0.5784801414667655184, 0.5833333333333333703, 0.5888888888888889062, 0.5944444444444444420, 0.5999999999999999778 ),
 .UNSPECIFIED. ) 
 CURVE ( )  GEOMETRIC_REPRESENTATION_ITEM ( )  RATIONAL_B_SPLINE_CURVE ( ( 0.9924735557117673190, 0.9702336695114960330, 1.000000000000000000, 0.9659258262890683122, 1.000000000000000000, 0.9659258262890683122, 1.000000000000000000, 0.9659258262890683122, 1.000000000000000000 ) ) 
 REPRESENTATION_ITEM ( '' )  );
#70312=SURFACE_STYLE_FILL_AREA ( #63275 ) ;
#70318=CARTESIAN_POINT ( 'NONE',  ( 10.14667048435145169, 4.379817243679289018E-16, -10.35833375027041292 ) ) ;
#70319=B_SPLINE_CURVE_WITH_KNOTS ( 'NONE', 3,
 ( #39427, #93395, #33368, #78391, #1441, #8910 ),
 .UNSPECIFIED., .F., .F.,
 ( 4, 2, 4 ),
 ( 0.0002800206007755258637, 0.0006862260317143902954, 0.001092431462653254727 ),
 .UNSPECIFIED. ) ;
#70331=DIRECTION ( 'NONE',  ( 0.000000000000000000, 1.000000000000000000, 0.000000000000000000 ) ) ;
#70332=ORIENTED_EDGE ( 'NONE', *, *, #90328, .F. ) ;
#70355=CARTESIAN_POINT ( 'NONE',  ( 0.000000000000000000, 0.5000000000000004441, 0.000000000000000000 ) ) ;
#70361=EDGE_CURVE ( 'NONE', #79695, #69512, #40272, .T. ) ;
#70366=DIRECTION ( 'NONE',  ( 0.000000000000000000, 0.000000000000000000, 1.000000000000000000 ) ) ;
#70369=EDGE_CURVE ( 'NONE', #73524, #68154, #26873, .T. ) ;
#70377=VERTEX_POINT ( 'NONE', #21565 ) ;
#70386=CARTESIAN_POINT ( 'NONE',  ( 13.55255535720595184, 0.000000000000000000, -4.403492169842965431 ) ) ;
#70392=VERTEX_POINT ( 'NONE', #82547 ) ;
#70406=EDGE_LOOP ( 'NONE', ( #35505, #63012, #69656, #6801, #97210, #6405 ) ) ;
#70423=ORIENTED_EDGE ( 'NONE', *, *, #98139, .T. ) ;
#70431=DIRECTION ( 'NONE',  ( -0.000000000000000000, -1.000000000000000000, -0.000000000000000000 ) ) ;
#70437=CARTESIAN_POINT ( 'NONE',  ( 0.000000000000000000, 0.5000000000000004441, 0.000000000000000000 ) ) ;
#70445=CARTESIAN_POINT ( 'NONE',  ( 12.26659068614894466, -10.27958449841935540, -7.082119434687053960 ) ) ;
#70447=FACE_OUTER_BOUND ( 'NONE', #68485, .T. ) ;
#70448=VERTEX_POINT ( 'NONE', #21064 ) ;
#70450=DIRECTION ( 'NONE',  ( 0.000000000000000000, 1.000000000000000000, 0.000000000000000000 ) ) ;
#70468=CIRCLE ( 'NONE', #19357, 15.00000000000000000 ) ;
#70472=FACE_OUTER_BOUND ( 'NONE', #24274, .T. ) ;
#70473=EDGE_CURVE ( 'NONE', #1302, #81942, #14063, .T. ) ;
#70485=EDGE_CURVE ( 'NONE', #34672, #86489, #68047, .T. ) ;
#70493=EDGE_LOOP ( 'NONE', ( #64582, #13658, #79296, #97535 ) ) ;
#70498=VECTOR ( 'NONE', #84799, 1000.000000000000114 ) ;
#70503=CARTESIAN_POINT ( 'NONE',  ( -13.61464873478171533, 0.5000000000000004441, 6.296136897217742501 ) ) ;
#70512=CARTESIAN_POINT ( 'NONE',  ( 7.208316651077762316, 24.13393115100078745, -7.208316651077764980 ) ) ;
#70513=ORIENTED_EDGE ( 'NONE', *, *, #65210, .T. ) ;
#70525=ORIENTED_EDGE ( 'NONE', *, *, #2782, .F. ) ;
#70529=EDGE_CURVE ( 'NONE', #57542, #17879, #62003, .T. ) ;
#70530=ORIENTED_EDGE ( 'NONE', *, *, #89951, .F. ) ;
#70536=CARTESIAN_POINT ( 'NONE',  ( -10.17198128013128589, 0.2306972965111904195, -10.94389562857679898 ) ) ;
#70538=SURFACE_STYLE_USAGE ( .BOTH. , #93024 ) ;
#70549=CARTESIAN_POINT ( 'NONE',  ( 14.62617646268092209, 14.49999999999999112, 3.327906561566971622 ) ) ;
#70551=VERTEX_POINT ( 'NONE', #85015 ) ;
#70557=EDGE_CURVE ( 'NONE', #95164, #48237, #31986, .T. ) ;
#70559=DIRECTION ( 'NONE',  ( -0.04361938736533987893, 0.000000000000000000, 0.9990482215818576872 ) ) ;
#70563=ORIENTED_EDGE ( 'NONE', *, *, #41553, .T. ) ;
#70572=FACE_OUTER_BOUND ( 'NONE', #41546, .T. ) ;
#70577=CARTESIAN_POINT ( 'NONE',  ( 2.915334737309928315, -0.4779813225118263453, 10.88017736071109987 ) ) ;
#70583=CARTESIAN_POINT ( 'NONE',  ( -13.55101055326446513, 0.2301500585724586545, -6.292244619294828922 ) ) ;
#70584=DIRECTION ( 'NONE',  ( -0.4924235601034707144, 0.000000000000000000, 0.8703556959398975890 ) ) ;
#70588=CARTESIAN_POINT ( 'NONE',  ( 0.000000000000000000, 15.00000000000000000, 0.000000000000000000 ) ) ;
#70589=EDGE_CURVE ( 'NONE', #62099, #95614, #568, .T. ) ;
#70594=CARTESIAN_POINT ( 'NONE',  ( 0.000000000000000000, 0.5000000000000004441, 0.000000000000000000 ) ) ;
#70596=EDGE_LOOP ( 'NONE', ( #64572, #20475, #72666, #42777, #78170, #70721 ) ) ;
#70598=EDGE_CURVE ( 'NONE', #65919, #97109, #62492, .T. ) ;
#70610=ORIENTED_EDGE ( 'NONE', *, *, #94697, .T. ) ;
#70611=VERTEX_POINT ( 'NONE', #76523 ) ;
#70612=AXIS2_PLACEMENT_3D ( 'NONE', #24034, #85017, #77498 ) ;
#70625=CARTESIAN_POINT ( 'NONE',  ( -9.846743663894594434, -8.991068848999208996, 3.469446951953614189E-15 ) ) ;
#70627=ORIENTED_EDGE ( 'NONE', *, *, #16954, .F. ) ;
#70628=PLANE ( 'NONE',  #74691 ) ;
#70630=CARTESIAN_POINT ( 'NONE',  ( 0.000000000000000000, 15.00000000000000000, 0.000000000000000000 ) ) ;
#70631=EDGE_LOOP ( 'NONE', ( #78878, #29291, #61824, #79997 ) ) ;
#70638=FACE_OUTER_BOUND ( 'NONE', #25679, .T. ) ;
#70640=VECTOR ( 'NONE', #83193, 1000.000000000000000 ) ;
#70642=ORIENTED_EDGE ( 'NONE', *, *, #63145, .T. ) ;
#70647=VECTOR ( 'NONE', #5191, 999.9999999999998863 ) ;
#70649=VERTEX_POINT ( 'NONE', #62990 ) ;
#70659=DIRECTION ( 'NONE',  ( 0.000000000000000000, 0.000000000000000000, 1.000000000000000000 ) ) ;
#70668=CARTESIAN_POINT ( 'NONE',  ( 5.817157072110708427, 14.49999999999999112, 13.82608706751097749 ) ) ;
#70670=CARTESIAN_POINT ( 'NONE',  ( 7.881609424765942506, -3.117928278843078365E-15, 12.32025747423898920 ) ) ;
#70675=CARTESIAN_POINT ( 'NONE',  ( 0.000000000000000000, 35.00000000000000000, -11.92686044187656513 ) ) ;
#70681=CIRCLE ( 'NONE', #16372, 15.00000000000000000 ) ;
#70682=EDGE_CURVE ( 'NONE', #38225, #55365, #77986, .T. ) ;
#70683=EDGE_CURVE ( 'NONE', #87096, #44552, #77496, .T. ) ;
#70691=CARTESIAN_POINT ( 'NONE',  ( -3.881909499400522989, -2.713893563002777498E-15, 14.10103859407592353 ) ) ;
#70693=CYLINDRICAL_SURFACE ( 'NONE', #79126, 15.00000000000000000 ) ;
#70696=CARTESIAN_POINT ( 'NONE',  ( -5.204170427930421283E-15, 30.55374883491396432, -14.16423886937410082 ) ) ;
#70704=VECTOR ( 'NONE', #82381, 999.9999999999998863 ) ;
#70708=ORIENTED_EDGE ( 'NONE', *, *, #68238, .F. ) ;
#70713=CARTESIAN_POINT ( 'NONE',  ( -5.279540384298767819, 0.000000000000000000, -1.365381980696781294 ) ) ;
#70721=ORIENTED_EDGE ( 'NONE', *, *, #42814, .F. ) ;
#70724=FACE_OUTER_BOUND ( 'NONE', #71935, .T. ) ;
#70735=CARTESIAN_POINT ( 'NONE',  ( -7.881609424771932382, 14.99999999999799982, 12.32025747424302864 ) ) ;
#70736=ORIENTED_EDGE ( 'NONE', *, *, #51539, .F. ) ;
#70739=DIRECTION ( 'NONE',  ( -0.000000000000000000, -1.000000000000000000, -0.000000000000000000 ) ) ;
#70753=CARTESIAN_POINT ( 'NONE',  ( -11.10175276308059722, 14.95037105032149150, 9.716398248526216364 ) ) ;
#70757=EDGE_LOOP ( 'NONE', ( #35182, #65200, #32249, #27310 ) ) ;
#70758=CARTESIAN_POINT ( 'NONE',  ( -1.175037534397030736, -2.805373121306241934E-15, -14.57833316477038110 ) ) ;
#70759=VERTEX_POINT ( 'NONE', #39524 ) ;
#70766=ORIENTED_EDGE ( 'NONE', *, *, #52091, .T. ) ;
#70769=CARTESIAN_POINT ( 'NONE',  ( 3.469446951953614189E-15, -9.626365330069580395, 12.81628187352647608 ) ) ;
#70773=ORIENTED_EDGE ( 'NONE', *, *, #83094, .T. ) ;
#70781=ORIENTED_EDGE ( 'NONE', *, *, #6837, .F. ) ;
#70784=CARTESIAN_POINT ( 'NONE',  ( -14.56089864659471544, 15.00000000000000533, 1.374314915485193245 ) ) ;
#70785=DIRECTION ( 'NONE',  ( -0.000000000000000000, -1.000000000000000000, -0.000000000000000000 ) ) ;
#70787=VECTOR ( 'NONE', #63626, 1000.000000000000000 ) ;
#70790=DIRECTION ( 'NONE',  ( 0.9170600743851238246, 0.000000000000000000, -0.3987490689252466969 ) ) ;
#70824=FACE_OUTER_BOUND ( 'NONE', #54050, .T. ) ;
#70840=ORIENTED_EDGE ( 'NONE', *, *, #15254, .T. ) ;
#70848=CARTESIAN_POINT ( 'NONE',  ( 0.000000000000000000, 14.49999999999999822, 0.000000000000000000 ) ) ;
#70875=ORIENTED_EDGE ( 'NONE', *, *, #29122, .F. ) ;
#70880=CARTESIAN_POINT ( 'NONE',  ( 5.817157072110800797, 15.00000000000000000, -13.82608706751086558 ) ) ;
#70888=VERTEX_POINT ( 'NONE', #41499 ) ;
#70897=EDGE_CURVE ( 'NONE', #40528, #85153, #71968, .T. ) ;
#70902=VERTEX_POINT ( 'NONE', #64939 ) ;
#70903=DIRECTION ( 'NONE',  ( 0.000000000000000000, 1.000000000000000000, 0.000000000000000000 ) ) ;
#70909=CARTESIAN_POINT ( 'NONE',  ( -5.795997163830251431, 15.00000000000000000, 13.01802277140702024 ) ) ;
#70910=CARTESIAN_POINT ( 'NONE',  ( -13.48255862861919852, 3.931018169630358772E-16, -5.335786055104346559 ) ) ;
#70912=CARTESIAN_POINT ( 'NONE',  ( 15.08495336817614607, 15.00000000000000000, -5.321802168063438643 ) ) ;
#70915=CARTESIAN_POINT ( 'NONE',  ( 0.7375392941517235901, 0.5000000000000004441, 14.98185688723471110 ) ) ;
#70916=DIRECTION ( 'NONE',  ( 0.000000000000000000, 0.000000000000000000, 1.000000000000000000 ) ) ;
#70918=ORIENTED_EDGE ( 'NONE', *, *, #47881, .T. ) ;
#70921=EDGE_CURVE ( 'NONE', #30230, #41646, #2929, .T. ) ;
#70923=DIRECTION ( 'NONE',  ( 0.6225146366376183016, 0.000000000000000000, -0.7826081568524148047 ) ) ;
#70926=B_SPLINE_CURVE_WITH_KNOTS ( 'NONE', 3,
 ( #62249, #76766, #15308, #90785, #45288, #75783 ),
 .UNSPECIFIED., .F., .F.,
 ( 4, 2, 4 ),
 ( 0.0002800671705680555569, 0.0006862730573397291499, 0.001092478944111402797 ),
 .UNSPECIFIED. ) ;
#70930=AXIS2_PLACEMENT_3D ( 'NONE', #16703, #2211, #87145 ) ;
#70940=ORIENTED_EDGE ( 'NONE', *, *, #87122, .F. ) ;
#70942=CARTESIAN_POINT ( 'NONE',  ( 0.000000000000000000, 14.49999999999999822, 0.000000000000000000 ) ) ;
#70946=CARTESIAN_POINT ( 'NONE',  ( -10.36894250292378317, 12.42874883491396432, 10.36894250292379560 ) ) ;
#70951=CARTESIAN_POINT ( 'NONE',  ( -5.991992585808451288, 3.888230080364882544E-16, -13.20401548210303311 ) ) ;
#70955=LINE ( 'NONE', #39952, #9801 ) ;
#70966=FACE_OUTER_BOUND ( 'NONE', #97184, .T. ) ;
#70978=CARTESIAN_POINT ( 'NONE',  ( -5.817157072110618721, 14.63606918420059877, -13.82608706751098815 ) ) ;
#70990=VERTEX_POINT ( 'NONE', #64453 ) ;
#70993=VERTEX_POINT ( 'NONE', #26957 ) ;
#70999=CIRCLE ( 'NONE', #8667, 14.49999999999999822 ) ;
#71000=CARTESIAN_POINT ( 'NONE',  ( 10.19513985507825637, 0.5000000000000004441, 11.00268709613223983 ) ) ;
#71010=CARTESIAN_POINT ( 'NONE',  ( -2.638427012816840111, 29.96726448433413381, -9.846743663894590881 ) ) ;
#71022=ORIENTED_EDGE ( 'NONE', *, *, #88542, .F. ) ;
#71034=PRESENTATION_STYLE_ASSIGNMENT (( #70538 ) ) ;
#71037=ORIENTED_EDGE ( 'NONE', *, *, #29663, .F. ) ;
#71038=CARTESIAN_POINT ( 'NONE',  ( 14.22792531055119092, -2.184074454495212635E-15, 3.387425595041200665 ) ) ;
#71051=ORIENTED_EDGE ( 'NONE', *, *, #3851, .F. ) ;
#71070=EDGE_CURVE ( 'NONE', #32615, #94433, #51935, .T. ) ;
#71073=CARTESIAN_POINT ( 'NONE',  ( 10.88017736071109987, 5.772018677488179428, -2.915334737309928315 ) ) ;
#71076=CARTESIAN_POINT ( 'NONE',  ( 13.82192141328809676, 4.465570197798056962E-16, 4.382292601468775750 ) ) ;
#71077=ADVANCED_FACE ( 'NONE', ( #50444 ), #66431, .F. ) ;
#71082=DIRECTION ( 'NONE',  ( -0.000000000000000000, -1.000000000000000000, -0.000000000000000000 ) ) ;
#71094=CARTESIAN_POINT ( 'NONE',  ( -12.83294900548068895, 0.5000000000000004441, 7.766300266068274283 ) ) ;
#71100=LINE ( 'NONE', #50060, #10687 ) ;
#71104=CARTESIAN_POINT ( 'NONE',  ( 0.000000000000000000, 0.5000000000000004441, 0.000000000000000000 ) ) ;
#71106=ORIENTED_EDGE ( 'NONE', *, *, #5216, .F. ) ;
#71118=CARTESIAN_POINT ( 'NONE',  ( 4.547378612396755670, 0.000000000000000000, 3.009844244835539584 ) ) ;
#71120=CARTESIAN_POINT ( 'NONE',  ( 8.527530157486179263, -6.907735515665875958, 4.923371831947292776 ) ) ;
#71123=VECTOR ( 'NONE', #65979, 1000.000000000000114 ) ;
#71131=DIRECTION ( 'NONE',  ( -3.552713678800500929E-14, 0.000000000000000000, 1.000000000000000000 ) ) ;
#71133=AXIS2_PLACEMENT_3D ( 'NONE', #12730, #5253, #95753 ) ;
#71137=VERTEX_POINT ( 'NONE', #36935 ) ;
#71139=VERTEX_POINT ( 'NONE', #96465 ) ;
#71145=LINE ( 'NONE', #93638, #36139 ) ;
#71146=ORIENTED_EDGE ( 'NONE', *, *, #98339, .T. ) ;
#71147=AXIS2_PLACEMENT_3D ( 'NONE', #84955, #77441, #39470 ) ;
#71151=EDGE_LOOP ( 'NONE', ( #56117, #81570, #73075, #37865 ) ) ;
#71154=DIRECTION ( 'NONE',  ( -0.000000000000000000, -1.000000000000000000, -0.000000000000000000 ) ) ;
#71155=ADVANCED_FACE ( 'NONE', ( #21437 ), #20948, .F. ) ;
#71156=FACE_OUTER_BOUND ( 'NONE', #94219, .T. ) ;
#71158=CARTESIAN_POINT ( 'NONE',  ( -1.796645268984514487, 0.2306972965111897533, -14.83273813124061036 ) ) ;
#71164=DIRECTION ( 'NONE',  ( 0.000000000000000000, -1.000000000000000000, 0.000000000000000000 ) ) ;
#71173=CIRCLE ( 'NONE', #35832, 15.00000000000000000 ) ;
#71176=CARTESIAN_POINT ( 'NONE',  ( 9.159723438033203990, 15.00000000000000000, -10.91613331444542645 ) ) ;
#71182=CARTESIAN_POINT ( 'NONE',  ( -15.99538290524656503, -0.03417435944610275333, -0.1584996864330918964 ) ) ;
#71186=CARTESIAN_POINT ( 'NONE',  ( -12.26659068614895354, 31.38708216824731423, -7.082119434687038861 ) ) ;
#71189=LINE ( 'NONE', #94166, #72877 ) ;
#71190=FACE_OUTER_BOUND ( 'NONE', #10731, .T. ) ;
#71198=VECTOR ( 'NONE', #96337, 1000.000000000000000 ) ;
#71199=VERTEX_POINT ( 'NONE', #4961 ) ;
#71204=DIRECTION ( 'NONE',  ( 0.2503800040544526539, 0.000000000000000000, -0.9681476403781048568 ) ) ;
#71205=CARTESIAN_POINT ( 'NONE',  ( -13.78891971893199830, 15.00000000000000000, -5.904717858191724567 ) ) ;
#71212=CARTESIAN_POINT ( 'NONE',  ( -5.419894505350723257, 14.49999999999999112, 13.98659156302460183 ) ) ;
#71218=LINE ( 'NONE', #80175, #84694 ) ;
#71232=CARTESIAN_POINT ( 'NONE',  ( 11.29222593019777499, 0.2306972965111881713, -9.783848334571253247 ) ) ;
#71237=CARTESIAN_POINT ( 'NONE',  ( -11.48952521350009448, 15.00000000000000000, -8.845383562533896793 ) ) ;
#71242=DIRECTION ( 'NONE',  ( -0.000000000000000000, -1.000000000000000000, -0.000000000000000000 ) ) ;
#71246=AXIS2_PLACEMENT_3D ( 'NONE', #46904, #85409, #32886 ) ;
#71250=LINE ( 'NONE', #2279, #79247 ) ;
#71251=EDGE_CURVE ( 'NONE', #53769, #70273, #39744, .T. ) ;
#71254=EDGE_CURVE ( 'NONE', #29582, #46734, #57941, .T. ) ;
#71255=CARTESIAN_POINT ( 'NONE',  ( 12.81628187352647252, -8.168031996736246469, -3.434112377981059172 ) ) ;
#71256=ORIENTED_EDGE ( 'NONE', *, *, #30883, .T. ) ;
#71258=ORIENTED_EDGE ( 'NONE', *, *, #27705, .F. ) ;
#71259=ORIENTED_EDGE ( 'NONE', *, *, #96875, .F. ) ;
#71263=DIRECTION ( 'NONE',  ( -0.000000000000000000, -1.000000000000000000, -0.000000000000000000 ) ) ;
#71267=CIRCLE ( 'NONE', #23394, 15.00000000000000000 ) ;
#71270=CARTESIAN_POINT ( 'NONE',  ( 14.49120296996857959, 14.95077488074853456, -2.766068805437525757 ) ) ;
#71271=CARTESIAN_POINT ( 'NONE',  ( -15.96747533562963994, 15.00000000000000000, 0.9576679184939570488 ) ) ;
#71276=EDGE_CURVE ( 'NONE', #51412, #70611, #89329, .T. ) ;
#71286=CARTESIAN_POINT ( 'NONE',  ( 4.838527690343521925, 14.63606918327236706, 14.19819177887734263 ) ) ;
#71290=AXIS2_PLACEMENT_3D ( 'NONE', #91708, #23227, #69209 ) ;
#71293=( LENGTH_UNIT ( ) NAMED_UNIT ( * ) SI_UNIT ( .MILLI., .METRE. ) );
#71296=B_SPLINE_CURVE_WITH_KNOTS ( 'NONE', 3,
 ( #64830, #95348, #26846, #89326, #87835, #19354 ),
 .UNSPECIFIED., .F., .F.,
 ( 4, 2, 4 ),
 ( 3.409110551496216072E-05, 0.0004400426677368010999, 0.0008459942299586401069 ),
 .UNSPECIFIED. ) ;
#71298=ORIENTED_EDGE ( 'NONE', *, *, #94836, .F. ) ;
#71302=LINE ( 'NONE', #33273, #85437 ) ;
#71314=ORIENTED_EDGE ( 'NONE', *, *, #60187, .F. ) ;
#71326=ORIENTED_EDGE ( 'NONE', *, *, #86042, .F. ) ;
#71338=CYLINDRICAL_SURFACE ( 'NONE', #69132, 15.00000000000000000 ) ;
#71342=B_SPLINE_CURVE_WITH_KNOTS ( 'NONE', 3,
 ( #39526, #7057, #53027, #46516, #16028, #92504 ),
 .UNSPECIFIED., .F., .F.,
 ( 4, 2, 4 ),
 ( 3.409110551494637880E-05, 0.0004400426677367927516, 0.0008459942299586391311 ),
 .UNSPECIFIED. ) ;
#71351=TOROIDAL_SURFACE ( 'NONE', #55415, 14.49999999999999822, 0.5000000000000000000 ) ;
#71359=B_SPLINE_CURVE_WITH_KNOTS ( 'NONE', 3,
 ( #32466, #85977, #31959, #39000, #2500, #92475 ),
 .UNSPECIFIED., .F., .F.,
 ( 4, 2, 4 ),
 ( 3.409110551496104263E-05, 0.0004400426677367857585, 0.0008459942299586103998 ),
 .UNSPECIFIED. ) ;
#71364=EDGE_CURVE ( 'NONE', #11587, #98827, #79624, .T. ) ;
#71366=EDGE_LOOP ( 'NONE', ( #23309, #73956, #73560, #67798, #84431, #11841 ) ) ;
#71367=CARTESIAN_POINT ( 'NONE',  ( 0.000000000000000000, 0.5000000000000004441, 0.000000000000000000 ) ) ;
#71368=CIRCLE ( 'NONE', #79345, 14.49999999999999822 ) ;
#71371=AXIS2_PLACEMENT_3D ( 'NONE', #1138, #24127, #85608 ) ;
#71373=EDGE_CURVE ( 'NONE', #37516, #76346, #19950, .T. ) ;
#71380=EDGE_CURVE ( 'NONE', #18961, #88806, #59912, .T. ) ;
#71393=FACE_OUTER_BOUND ( 'NONE', #25220, .T. ) ;
#71405=DIRECTION ( 'NONE',  ( -0.000000000000000000, -1.000000000000000000, -0.000000000000000000 ) ) ;
#71406=DIRECTION ( 'NONE',  ( -0.9969173337331284079, 0.000000000000000000, 0.07845909572783861530 ) ) ;
#71427=FACE_OUTER_BOUND ( 'NONE', #94343, .T. ) ;
#71428=CARTESIAN_POINT ( 'NONE',  ( 0.000000000000000000, 0.000000000000000000, 0.000000000000000000 ) ) ;
#71432=CARTESIAN_POINT ( 'NONE',  ( 3.897244926436219892, 4.401207273199346175E-16, -13.96644127841330807 ) ) ;
#71433=VECTOR ( 'NONE', #93398, 1000.000000000000000 ) ;
#71435=CARTESIAN_POINT ( 'NONE',  ( -12.26659068614895354, 6.387082168247300018, -7.082119434687038861 ) ) ;
#71443=CARTESIAN_POINT ( 'NONE',  ( -6.091055032734201014, 15.00000000000000888, -13.29802223412764484 ) ) ;
#71449=ADVANCED_FACE ( 'NONE', ( #39885 ), #46881, .T. ) ;
#71456=DIRECTION ( 'NONE',  ( -0.2672383760782501838, 0.000000000000000000, -0.9636304532086248376 ) ) ;
#71459=VERTEX_POINT ( 'NONE', #30396 ) ;
#71461=EDGE_CURVE ( 'NONE', #67657, #95164, #89254, .T. ) ;
#71469=AXIS2_PLACEMENT_3D ( 'NONE', #23449, #69921, #54895 ) ;
#71473=VERTEX_POINT ( 'NONE', #92384 ) ;
#71480=EDGE_LOOP ( 'NONE', ( #45671, #88761, #57000, #58762, #52940, #46135 ) ) ;
#71490=EDGE_CURVE ( 'NONE', #21109, #81310, #72662, .T. ) ;
#71495=B_SPLINE_CURVE_WITH_KNOTS ( 'NONE', 3,
 ( #5049, #21036, #5548, #89527, #35532, #81520 ),
 .UNSPECIFIED., .F., .F.,
 ( 4, 2, 4 ),
 ( 0.0002800715030460590818, 0.0006862774322447821786, 0.001092483361443505330 ),
 .UNSPECIFIED. ) ;
#71501=CARTESIAN_POINT ( 'NONE',  ( 14.49440716394873618, 15.00000000000000000, -0.4026921475166200803 ) ) ;
#71503=CARTESIAN_POINT ( 'NONE',  ( -9.382169495545413795, -25.25136533006957862, 9.382169495545428006 ) ) ;
#71517=EDGE_CURVE ( 'NONE', #91342, #12526, #65251, .T. ) ;
#71519=ORIENTED_EDGE ( 'NONE', *, *, #18082, .F. ) ;
#71530=DIRECTION ( 'NONE',  ( 0.000000000000000000, 1.000000000000000000, 0.000000000000000000 ) ) ;
#71534=FACE_OUTER_BOUND ( 'NONE', #78419, .T. ) ;
#71536=ORIENTED_EDGE ( 'NONE', *, *, #60295, .T. ) ;
#71538=CARTESIAN_POINT ( 'NONE',  ( -4.922013193295457611, 0.000000000000000000, 2.347679864819414153 ) ) ;
#71543=CARTESIAN_POINT ( 'NONE',  ( -14.97687855664608847, 0.5000000000000004441, 0.8325315005899532883 ) ) ;
#71554=CARTESIAN_POINT ( 'NONE',  ( 3.469446951953614189E-15, -26.94625116508602858, 14.16423886937410259 ) ) ;
#71564=AXIS2_PLACEMENT_3D ( 'NONE', #78157, #95112, #2683 ) ;
#71567=CARTESIAN_POINT ( 'NONE',  ( -10.88017736071110342, 8.063685344154844614, 3.903127820947815962E-15 ) ) ;
#71575=AXIS2_PLACEMENT_3D ( 'NONE', #36564, #22555, #30026 ) ;
#71578=CARTESIAN_POINT ( 'NONE',  ( 1.377727649040772586E-15, 15.00000000000000000, 11.25000000000000178 ) ) ;
#71585=DIRECTION ( 'NONE',  ( 0.000000000000000000, 0.000000000000000000, 1.000000000000000000 ) ) ;
#71611=ADVANCED_FACE ( 'NONE', ( #23814 ), #31725, .T. ) ;
#71613=CARTESIAN_POINT ( 'NONE',  ( 7.208316651077762316, 9.133931151000789228, -7.208316651077764980 ) ) ;
#71623=CARTESIAN_POINT ( 'NONE',  ( 14.97687855664614176, 14.49999999999999112, 0.8325315005901842147 ) ) ;
#71636=B_SPLINE_CURVE_WITH_KNOTS ( 'NONE', 3,
 ( #57722, #73710, #87731, #80234, #34223, #28216 ),
 .UNSPECIFIED., .F., .F.,
 ( 4, 2, 4 ),
 ( 3.409110551496141533E-05, 0.0004400426677367868427, 0.0008459942299586122429 ),
 .UNSPECIFIED. ) ;
#71637=CARTESIAN_POINT ( 'NONE',  ( 0.9940297508536876103, -0.03417435944610275333, 14.21528771620250353 ) ) ;
#71639=DIRECTION ( 'NONE',  ( 0.000000000000000000, 1.000000000000000000, 0.000000000000000000 ) ) ;
#71640=ORIENTED_EDGE ( 'NONE', *, *, #85395, .F. ) ;
#71651=CARTESIAN_POINT ( 'NONE',  ( 12.22474924877137070, 14.76984934309701991, 8.589397507024928657 ) ) ;
#71652=EDGE_LOOP ( 'NONE', ( #68080, #54633, #53152, #71326 ) ) ;
#71653=CARTESIAN_POINT ( 'NONE',  ( 14.47650479471822926, 14.63606881343832100, 3.928206833722133862 ) ) ;
#71665=CARTESIAN_POINT ( 'NONE',  ( 7.792922786566074400, 12.98375417942040322, -8.778698621334729779 ) ) ;
#71666=CARTESIAN_POINT ( 'NONE',  ( -7.551349515323020789, 0.000000000000000000, -12.08468537022916323 ) ) ;
#71668=DIRECTION ( 'NONE',  ( 0.000000000000000000, 0.000000000000000000, 1.000000000000000000 ) ) ;
#71671=CARTESIAN_POINT ( 'NONE',  ( -9.422509992056145478, -32.35298132251182324, -5.440088680355541939 ) ) ;
#71683=ORIENTED_EDGE ( 'NONE', *, *, #16385, .T. ) ;
#71688=FACE_OUTER_BOUND ( 'NONE', #89835, .T. ) ;
#71689=PLANE ( 'NONE',  #75948 ) ;
#71700=DIRECTION ( 'NONE',  ( -0.9762960071199346945, 0.000000000000000000, 0.2164396139380971029 ) ) ;
#71703=VERTEX_POINT ( 'NONE', #81218 ) ;
#71705=DIRECTION ( 'NONE',  ( -0.6087614290087242086, 0.000000000000000000, 0.7933533402912323895 ) ) ;
#71708=CARTESIAN_POINT ( 'NONE',  ( 5.624999999999998224, 11.25513551118487676, -9.742785792574936821 ) ) ;
#71711=EDGE_CURVE ( 'NONE', #69641, #26110, #18763, .T. ) ;
#71720=DIRECTION ( 'NONE',  ( 0.000000000000000000, 0.000000000000000000, 1.000000000000000000 ) ) ;
#71722=EDGE_CURVE ( 'NONE', #86936, #97713, #42942, .T. ) ;
#71725=ORIENTED_EDGE ( 'NONE', *, *, #48113, .F. ) ;
#71726=CARTESIAN_POINT ( 'NONE',  ( 15.81765804549837107, 15.00000000000000000, 2.383084218346927408 ) ) ;
#71729=ORIENTED_EDGE ( 'NONE', *, *, #21925, .F. ) ;
#71736=B_SPLINE_CURVE_WITH_KNOTS ( 'NONE', 3,
 ( #44202, #97740, #74712, #98736, #92183, #30678 ),
 .UNSPECIFIED., .F., .F.,
 ( 4, 2, 4 ),
 ( 3.409110551496111717E-05, 0.0004400426677367866800, 0.0008459942299586122429 ),
 .UNSPECIFIED. ) ;
#71737=CARTESIAN_POINT ( 'NONE',  ( 12.81628187352647608, -8.584698663402908991, 3.434112377981052511 ) ) ;
#71738=ORIENTED_EDGE ( 'NONE', *, *, #33841, .F. ) ;
#71751=CARTESIAN_POINT ( 'NONE',  ( -11.81378540890925066, -0.03417435944610275333, -7.968498874458281200 ) ) ;
#71752=CARTESIAN_POINT ( 'NONE',  ( 9.383795276901695459, 0.2306972965111900586, 11.62679839395699943 ) ) ;
#71757=EDGE_CURVE ( 'NONE', #85662, #23769, #23827, .T. ) ;
#71764=CARTESIAN_POINT ( 'NONE',  ( -14.43100913236848371, 4.112960668137814512E-16, -1.412789942453356318 ) ) ;
#71772=( BOUNDED_SURFACE ( )  B_SPLINE_SURFACE ( 1, 2, ( 
 ( #48532, #88009, #33520, #49511, #64509, #19035, #64016, #11036, #88505, #26048, #94528, #96022, #73002, #95013, #80018, #18540, #3067, #11520, #49031, #57513, #42044, #79032, #19521, #3551, #12508, #5018, #34503, #56538, #65500, #79536, #87028, #41558, #35501, #72022, #26522, #27503, #64995, #57018, #65996, #96524, #87520, #86548, #10545, #81007, #4041, #50017, #95521, #27014, #57999, #80521, #12019, #20008, #42519, #4533, #34997, #73491, #50509, #43009, #56055, #41055, #71554, #73991, #89496, #44971, #81491, #66992, #98510, #82981, #75476, #21499, #35994, #14997, #21007, #97515, #89004, #52476, #20511, #5517, #67489, #6991, #58493, #97023, #98011, #50996, #12994, #66497, #6486, #43490, #22001, #37495, #22491, #58994, #6005, #83475, #29964, #51494, #29465, #51996, #28500, #36500, #45467, #7495, #74483, #28978, #60470, #14003, #81988, #67983, #75967, #13500, #43979, #90959, #59481, #37989, #52964, #89982, #82485, #44480, #36993, #68481, #14501, #74982, #27996, #59971, #90466, #78425, #8943, #76948, #16458, #16949, #61449, #8458, #31438, #23964, #47434, #77431, #84465, #62425, #17453, #38964, #70445, #54438, #69457, #31925, #84947, #92928, #46938, #9942, #91464, #46455, #85442, #61940, #53456, #60955, #68970, #30950, #23485, #83963, #501, #91955, #55437, #24953, #9441, #975, #69952, #39462, #92441, #1471, #53958, #77933, #85942, #22990, #38477, #39942, #24460, #47920, #40445, #54926, #1962, #32428, #62929, #93431, #8, #30456, #15490, #45973, #76463, #7978, #15963, #48906, #88753, #89248, #33398, #79421, #3427, #94901, #20758, #50762, #56427, #35751, #89733, #10918, #43741, #26399, #41443, #5274, #58233, #66238, #20263, #51750, #63422, #18423, #58744, #33886, #25451, #32920, #40937, #2950, #94410, #55934, #71435, #63897, #28741, #97270, #81734, #71903, #43248, #81251, #64391, #82234, #25925, #2464, #93925, #59232, #10430, #96773, #86914, #12749, #74227, #73743, #78920, #13250, #28249, #51247, #5761, #21252, #36249, #66746, #13749, #70946, #86434, #17933, #48418, #61216, #97768, #83230, #15739, #255, #91719, #37747, #52239, #31199, #37258, #14754, #6249, #68727, #36753, #21758, #83727, #23240, #74736, #14250, #15250, #67243, #29232, #82731, #22741, #59731, #38237, #53712, #38721, #75228, #22248, #746, #46222, #6741, #45727, #68245, #44731, #52724, #61692, #23734, #90723, #45228, #76707, #60228, #75726, #30704, #67745, #60716, #92208, #44232, #84231, #8227, #69221, #90226, #54197, #76229, #91213, #7241, #7743, #98265, #84712, #29722, #98763, #30213, #53224, #69706, #33647, #85691, #56660, #16214, #54682, #2215, #24705, #56183, #39220, #85204, #79163, #9694, #55690, #17211, #55176, #41191, #86188, #16708, #70696, #64143, #77198, #39712, #71186, #93179, #77685, #47181, #32674, #1236, #9200, #63168, #2711 ),
 ( #63657, #94660, #48169, #33163, #8703, #78681, #92691, #40188, #47688, #78181, #24216, #70201, #48661, #1720, #32176, #86676, #94163, #93675, #25210, #62679, #62181, #17698, #10192, #40685, #25692, #31691, #18181, #10676, #71671, #26169, #3181, #46699, #96651, #11654, #87643, #19157, #36121, #26650, #49636, #28130, #96152, #34632, #97158, #89129, #50641, #72148, #80649, #88628, #81130, #65627, #66629, #58630, #20640, #35128, #28626, #73623, #58120, #27635, #5146, #57146, #51129, #50140, #12143, #12632, #35636, #81619, #80144, #65131, #43625, #13128, #42169, #20137, #42648, #95139, #95652, #5645, #87149, #27136, #57640, #74111, #73124, #72632, #66122, #18674, #11159, #4164, #49160, #88135, #79663, #41679, #19648, #4666, #43131, #3676, #34138, #64630, #98136, #83612, #46106, #76100, #38603, #68119, #37132, #75608, #7631, #21635, #67627, #90600, #83109, #38122, #37623, #44616, #22623, #76590, #29597, #30588, #14638, #60099, #91096, #45101, #53102, #7119, #69102, #51636, #6618, #45602, #22127, #13625, #21135, #29110, #90110, #82615, #44107, #59613, #52121, #15621, #84105, #68610, #52608, #30094, #98645, #60601, #636, #14131, #89623, #82115, #8108, #97646, #15127, #75112, #139, #61093, #91603, #67121, #23119, #53591, #59113, #74618, #6132, #36638, #62068, #9576, #92575, #84599, #77082, #24099, #48051, #16097, #70085, #2598, #86074, #78565, #24596, #39100, #18069, #54568, #1609, #92090, #55576, #23618, #8593, #70577, #10075, #61579, #1111, #2104, #54083, #46584, #69591, #40076, #31574, #25093, #86566, #56071, #40576, #32058, #32563, #55061, #62561, #41072, #85084, #16592, #47069, #48548, #77567, #63061, #9083, #39597, #33052, #93065, #85579, #71073, #93559, #17093, #17586, #79048, #63548, #47575, #94057, #78071, #25579, #10561, #71567, #31084, #56553, #42060, #73508, #58011, #50524, #95539, #11053, #89018, #95030, #72523, #64032, #27520, #94544, #79554, #42532, #81021, #33537, #72040, #73016, #26062, #87047, #41573, #80535, #18558, #96036, #12523, #96538, #34028, #80034, #58509, #5032, #64525, #4549, #27029, #3570, #11539, #20527, #81507, #49527, #4057, #35519, #88023, #26539, #43025, #51012, #49050, #57035, #66010, #34518, #13011, #28013, #65011, #57528, #19536, #12034, #43508, #88521, #50032, #20024, #3079, #87537, #19050, #35013, #65514, #90480, #90975, #36517, #82499, #6500, #98024, #22508, #52491, #59499, #37509, #91484, #14017, #45482, #29478, #44497, #7004, #59987, #68002, #22017, #53473, #66513, #21513, #60486, #37008, #28515, #36011, #43996, #6021, #97530, #59009, #74498, #67009, #83983, #75984, #83494, #82998, #15508, #52980, #44985, #14516, #15013, #13515, #7513, #67504, #75492, #98528, #89997, #74998, #29981, #28989, #38004, #30471, #74006, #68497, #24, #60972, #97040, #23005, #5531, #89512, #21022 ) ),
 .UNSPECIFIED., .F., .F., .T. ) 
 B_SPLINE_SURFACE_WITH_KNOTS ( ( 2, 2 ),
 ( 3, 2, 2, 2, 2, 2, 2, 2, 2, 2, 2, 2, 2, 2, 2, 2, 2, 2, 2, 2, 2, 2, 2, 2, 2, 2, 2, 2, 2, 2, 2, 2, 2, 2, 2, 2, 2, 2, 2, 2, 2, 2, 2, 2, 2, 2, 2, 2, 2, 2, 2, 2, 2, 2, 2, 2, 2, 2, 2, 2, 2, 2, 2, 2, 2, 2, 2, 2, 2, 2, 2, 2, 2, 2, 2, 2, 2, 2, 2, 2, 2, 2, 2, 2, 2, 2, 2, 2, 2, 2, 2, 2, 2, 2, 2, 2, 2, 2, 2, 2, 2, 2, 2, 2, 2, 2, 2, 2, 2, 2, 2, 2, 2, 2, 2, 2, 2, 2, 2, 2, 2, 2, 2, 2, 2, 2, 2, 2, 2, 2, 2, 2, 2, 2, 2, 2, 2, 2, 2, 2, 2, 2, 2, 2, 2, 2, 2, 2, 2, 2, 2, 2, 2, 2, 2, 2, 2, 2, 2, 2, 2, 2, 2, 2, 2, 2, 2, 2, 2, 2, 2, 2, 2, 2, 3 ),
 ( 0.000000000000000000, 1.000000000000000000 ),
 ( 0.000000000000000000, 0.005555555555555555768, 0.01111111111111111154, 0.01666666666666666644, 0.02222222222222222307, 0.02777777777777777624, 0.03333333333333333287, 0.03888888888888888951, 0.04444444444444444614, 0.05000000000000000278, 0.05555555555555555247, 0.06111111111111110911, 0.06666666666666666574, 0.07222222222222221544, 0.07777777777777777901, 0.08333333333333332871, 0.08888888888888889228, 0.09444444444444444198, 0.1000000000000000056, 0.1055555555555555552, 0.1111111111111111049, 0.1166666666666666685, 0.1222222222222222182, 0.1277777777777777679, 0.1333333333333333315, 0.1388888888888888951, 0.1444444444444444309, 0.1499999999999999944, 0.1555555555555555580, 0.1611111111111111216, 0.1666666666666666574, 0.1722222222222222210, 0.1777777777777777846, 0.1833333333333333204, 0.1888888888888888840, 0.1944444444444444475, 0.2000000000000000111, 0.2055555555555555469, 0.2111111111111111105, 0.2166666666666666741, 0.2222222222222222099, 0.2277777777777777735, 0.2333333333333333370, 0.2388888888888889006, 0.2444444444444444364, 0.2500000000000000000, 0.2555555555555555358, 0.2611111111111111271, 0.2666666666666666630, 0.2722222222222221988, 0.2777777777777777901, 0.2833333333333333259, 0.2888888888888888618, 0.2944444444444444531, 0.2999999999999999889, 0.3055555555555555802, 0.3111111111111111160, 0.3166666666666666519, 0.3222222222222222432, 0.3277777777777777790, 0.3333333333333333148, 0.3388888888888889062, 0.3444444444444444420, 0.3499999999999999778, 0.3555555555555555691, 0.3611111111111111049, 0.3666666666666666408, 0.3722222222222222321, 0.3777777777777777679, 0.3833333333333333592, 0.3888888888888888951, 0.3944444444444444309, 0.4000000000000000222, 0.4055555555555555580, 0.4111111111111110938, 0.4166666666666666852, 0.4222222222222222210, 0.4277777777777777568, 0.4333333333333333481, 0.4388888888888888840, 0.4444444444444444198, 0.4500000000000000111, 0.4555555555555555469, 0.4611111111111111382, 0.4666666666666666741, 0.4722222222222222099, 0.4777777777777778012, 0.4833333333333333370, 0.4888888888888888729, 0.4944444444444444642, 0.5000000000000000000, 0.5055555555555555358, 0.5111111111111110716, 0.5166666666666667185, 0.5222222222222222543, 0.5277777777777777901, 0.5333333333333333259, 0.5388888888888888618, 0.5444444444444443976, 0.5500000000000000444, 0.5555555555555555802, 0.5611111111111111160, 0.5666666666666666519, 0.5722222222222221877, 0.5777777777777777235, 0.5833333333333333703, 0.5888888888888889062, 0.5944444444444444420, 0.5999999999999999778, 0.6055555555555555136, 0.6111111111111111605, 0.6166666666666666963, 0.6222222222222222321, 0.6277777777777777679, 0.6333333333333333037, 0.6388888888888888395, 0.6444444444444444864, 0.6500000000000000222, 0.6555555555555555580, 0.6611111111111110938, 0.6666666666666666297, 0.6722222222222222765, 0.6777777777777778123, 0.6833333333333333481, 0.6888888888888888840, 0.6944444444444444198, 0.6999999999999999556, 0.7055555555555556024, 0.7111111111111111382, 0.7166666666666666741, 0.7222222222222222099, 0.7277777777777777457, 0.7333333333333332815, 0.7388888888888889284, 0.7444444444444444642, 0.7500000000000000000, 0.7555555555555555358, 0.7611111111111110716, 0.7666666666666667185, 0.7722222222222222543, 0.7777777777777777901, 0.7833333333333333259, 0.7888888888888888618, 0.7944444444444443976, 0.8000000000000000444, 0.8055555555555555802, 0.8111111111111111160, 0.8166666666666666519, 0.8222222222222221877, 0.8277777777777777235, 0.8333333333333333703, 0.8388888888888889062, 0.8444444444444444420, 0.8499999999999999778, 0.8555555555555555136, 0.8611111111111111605, 0.8666666666666666963, 0.8722222222222222321, 0.8777777777777777679, 0.8833333333333333037, 0.8888888888888888395, 0.8944444444444444864, 0.9000000000000000222, 0.9055555555555555580, 0.9111111111111110938, 0.9166666666666666297, 0.9222222222222222765, 0.9277777777777778123, 0.9333333333333333481, 0.9388888888888888840, 0.9444444444444444198, 0.9499999999999999556, 0.9555555555555556024, 0.9611111111111111382, 0.9666666666666666741 ),
 .UNSPECIFIED. ) 
 GEOMETRIC_REPRESENTATION_ITEM ( )  RATIONAL_B_SPLINE_SURFACE ( (
 ( 1.000000000000000000, 0.9659258262890683122, 1.000000000000000000, 0.9659258262890683122, 1.000000000000000000, 0.9659258262890683122, 1.000000000000000000, 0.9659258262890683122, 1.000000000000000000, 0.9659258262890683122, 1.000000000000000000, 0.9659258262890683122, 1.000000000000000000, 0.9659258262890683122, 1.000000000000000000, 0.9659258262890683122, 1.000000000000000000, 0.9659258262890683122, 1.000000000000000000, 0.9659258262890683122, 1.000000000000000000, 0.9659258262890683122, 1.000000000000000000, 0.9659258262890683122, 1.000000000000000000, 0.9659258262890683122, 1.000000000000000000, 0.9659258262890683122, 1.000000000000000000, 0.9659258262890683122, 1.000000000000000000, 0.9659258262890683122, 1.000000000000000000, 0.9659258262890683122, 1.000000000000000000, 0.9659258262890683122, 1.000000000000000000, 0.9659258262890683122, 1.000000000000000000, 0.9659258262890683122, 1.000000000000000000, 0.9659258262890683122, 1.000000000000000000, 0.9659258262890683122, 1.000000000000000000, 0.9659258262890683122, 1.000000000000000000, 0.9659258262890683122, 1.000000000000000000, 0.9659258262890683122, 1.000000000000000000, 0.9659258262890683122, 1.000000000000000000, 0.9659258262890683122, 1.000000000000000000, 0.9659258262890683122, 1.000000000000000000, 0.9659258262890683122, 1.000000000000000000, 0.9659258262890683122, 1.000000000000000000, 0.9659258262890683122, 1.000000000000000000, 0.9659258262890683122, 1.000000000000000000, 0.9659258262890683122, 1.000000000000000000, 0.9659258262890683122, 1.000000000000000000, 0.9659258262890683122, 1.000000000000000000, 0.9659258262890683122, 1.000000000000000000, 0.9659258262890683122, 1.000000000000000000, 0.9659258262890683122, 1.000000000000000000, 0.9659258262890683122, 1.000000000000000000, 0.9659258262890683122, 1.000000000000000000, 0.9659258262890683122, 1.000000000000000000, 0.9659258262890683122, 1.000000000000000000, 0.9659258262890683122, 1.000000000000000000, 0.9659258262890683122, 1.000000000000000000, 0.9659258262890683122, 1.000000000000000000, 0.9659258262890683122, 1.000000000000000000, 0.9659258262890683122, 1.000000000000000000, 0.9659258262890683122, 1.000000000000000000, 0.9659258262890683122, 1.000000000000000000, 0.9659258262890683122, 1.000000000000000000, 0.9659258262890683122, 1.000000000000000000, 0.9659258262890683122, 1.000000000000000000, 0.9659258262890683122, 1.000000000000000000, 0.9659258262890683122, 1.000000000000000000, 0.9659258262890683122, 1.000000000000000000, 0.9659258262890683122, 1.000000000000000000, 0.9659258262890683122, 1.000000000000000000, 0.9659258262890683122, 1.000000000000000000, 0.9659258262890683122, 1.000000000000000000, 0.9659258262890683122, 1.000000000000000000, 0.9659258262890683122, 1.000000000000000000, 0.9659258262890683122, 1.000000000000000000, 0.9659258262890683122, 1.000000000000000000, 0.9659258262890683122, 1.000000000000000000, 0.9659258262890683122, 1.000000000000000000, 0.9659258262890683122, 1.000000000000000000, 0.9659258262890683122, 1.000000000000000000, 0.9659258262890683122, 1.000000000000000000, 0.9659258262890683122, 1.000000000000000000, 0.9659258262890683122, 1.000000000000000000, 0.9659258262890683122, 1.000000000000000000, 0.9659258262890683122, 1.000000000000000000, 0.9659258262890683122, 1.000000000000000000, 0.9659258262890683122, 1.000000000000000000, 0.9659258262890683122, 1.000000000000000000, 0.9659258262890683122, 1.000000000000000000, 0.9659258262890683122, 1.000000000000000000, 0.9659258262890683122, 1.000000000000000000, 0.9659258262890683122, 1.000000000000000000, 0.9659258262890683122, 1.000000000000000000, 0.9659258262890683122, 1.000000000000000000, 0.9659258262890683122, 1.000000000000000000, 0.9659258262890683122, 1.000000000000000000, 0.9659258262890683122, 1.000000000000000000, 0.9659258262890683122, 1.000000000000000000, 0.9659258262890683122, 1.000000000000000000, 0.9659258262890683122, 1.000000000000000000, 0.9659258262890683122, 1.000000000000000000, 0.9659258262890683122, 1.000000000000000000, 0.9659258262890683122, 1.000000000000000000, 0.9659258262890683122, 1.000000000000000000, 0.9659258262890683122, 1.000000000000000000, 0.9659258262890683122, 1.000000000000000000, 0.9659258262890683122, 1.000000000000000000, 0.9659258262890683122, 1.000000000000000000, 0.9659258262890683122, 1.000000000000000000, 0.9659258262890683122, 1.000000000000000000, 0.9659258262890683122, 1.000000000000000000, 0.9659258262890683122, 1.000000000000000000, 0.9659258262890683122, 1.000000000000000000, 0.9659258262890683122, 1.000000000000000000, 0.9659258262890683122, 1.000000000000000000, 0.9659258262890683122, 1.000000000000000000, 0.9659258262890683122, 1.000000000000000000, 0.9659258262890683122, 1.000000000000000000, 0.9659258262890683122, 1.000000000000000000, 0.9659258262890683122, 1.000000000000000000, 0.9659258262890683122, 1.000000000000000000, 0.9659258262890683122, 1.000000000000000000, 0.9659258262890683122, 1.000000000000000000, 0.9659258262890683122, 1.000000000000000000, 0.9659258262890683122, 1.000000000000000000, 0.9659258262890683122, 1.000000000000000000, 0.9659258262890683122, 1.000000000000000000, 0.9659258262890683122, 1.000000000000000000, 0.9659258262890683122, 1.000000000000000000, 0.9659258262890683122, 1.000000000000000000, 0.9659258262890683122, 1.000000000000000000, 0.9659258262890683122, 1.000000000000000000, 0.9659258262890683122, 1.000000000000000000, 0.9659258262890683122, 1.000000000000000000, 0.9659258262890683122, 1.000000000000000000, 0.9659258262890683122, 1.000000000000000000, 0.9659258262890683122, 1.000000000000000000, 0.9659258262890683122, 1.000000000000000000, 0.9659258262890683122, 1.000000000000000000, 0.9659258262890683122, 1.000000000000000000, 0.9659258262890683122, 1.000000000000000000, 0.9659258262890683122, 1.000000000000000000, 0.9659258262890683122, 1.000000000000000000, 0.9659258262890683122, 1.000000000000000000, 0.9659258262890683122, 1.000000000000000000, 0.9659258262890683122, 1.000000000000000000, 0.9659258262890683122, 1.000000000000000000, 0.9659258262890683122, 1.000000000000000000, 0.9659258262890683122, 1.000000000000000000, 0.9659258262890683122, 1.000000000000000000, 0.9659258262890683122, 1.000000000000000000, 0.9659258262890683122, 1.000000000000000000, 0.9659258262890683122, 1.000000000000000000, 0.9659258262890683122, 1.000000000000000000, 0.9659258262890683122, 1.000000000000000000, 0.9659258262890683122, 1.000000000000000000, 0.9659258262890683122, 1.000000000000000000, 0.9659258262890683122, 1.000000000000000000, 0.9659258262890683122, 1.000000000000000000, 0.9659258262890683122, 1.000000000000000000, 0.9659258262890683122, 1.000000000000000000, 0.9659258262890683122, 1.000000000000000000, 0.9659258262890683122, 1.000000000000000000, 0.9659258262890683122, 1.000000000000000000, 0.9659258262890683122, 1.000000000000000000, 0.9659258262890683122, 1.000000000000000000, 0.9659258262890683122, 1.000000000000000000, 0.9659258262890683122, 1.000000000000000000, 0.9659258262890683122, 1.000000000000000000, 0.9659258262890683122, 1.000000000000000000, 0.9659258262890683122, 1.000000000000000000, 0.9659258262890683122, 1.000000000000000000, 0.9659258262890683122, 1.000000000000000000, 0.9659258262890683122, 1.000000000000000000, 0.9659258262890683122, 1.000000000000000000, 0.9659258262890683122, 1.000000000000000000, 0.9659258262890683122, 1.000000000000000000, 0.9659258262890683122, 1.000000000000000000, 0.9659258262890683122, 1.000000000000000000, 0.9659258262890683122, 1.000000000000000000, 0.9659258262890683122, 1.000000000000000000, 0.9659258262890683122, 1.000000000000000000, 0.9659258262890683122, 1.000000000000000000, 0.9659258262890683122, 1.000000000000000000, 0.9659258262890683122, 1.000000000000000000, 0.9659258262890683122, 1.000000000000000000, 0.9659258262890683122, 1.000000000000000000),
 ( 1.000000000000000000, 0.9659258262890683122, 1.000000000000000000, 0.9659258262890683122, 1.000000000000000000, 0.9659258262890683122, 1.000000000000000000, 0.9659258262890683122, 1.000000000000000000, 0.9659258262890683122, 1.000000000000000000, 0.9659258262890683122, 1.000000000000000000, 0.9659258262890683122, 1.000000000000000000, 0.9659258262890683122, 1.000000000000000000, 0.9659258262890683122, 1.000000000000000000, 0.9659258262890683122, 1.000000000000000000, 0.9659258262890683122, 1.000000000000000000, 0.9659258262890683122, 1.000000000000000000, 0.9659258262890683122, 1.000000000000000000, 0.9659258262890683122, 1.000000000000000000, 0.9659258262890683122, 1.000000000000000000, 0.9659258262890683122, 1.000000000000000000, 0.9659258262890683122, 1.000000000000000000, 0.9659258262890683122, 1.000000000000000000, 0.9659258262890683122, 1.000000000000000000, 0.9659258262890683122, 1.000000000000000000, 0.9659258262890683122, 1.000000000000000000, 0.9659258262890683122, 1.000000000000000000, 0.9659258262890683122, 1.000000000000000000, 0.9659258262890683122, 1.000000000000000000, 0.9659258262890683122, 1.000000000000000000, 0.9659258262890683122, 1.000000000000000000, 0.9659258262890683122, 1.000000000000000000, 0.9659258262890683122, 1.000000000000000000, 0.9659258262890683122, 1.000000000000000000, 0.9659258262890683122, 1.000000000000000000, 0.9659258262890683122, 1.000000000000000000, 0.9659258262890683122, 1.000000000000000000, 0.9659258262890683122, 1.000000000000000000, 0.9659258262890683122, 1.000000000000000000, 0.9659258262890683122, 1.000000000000000000, 0.9659258262890683122, 1.000000000000000000, 0.9659258262890683122, 1.000000000000000000, 0.9659258262890683122, 1.000000000000000000, 0.9659258262890683122, 1.000000000000000000, 0.9659258262890683122, 1.000000000000000000, 0.9659258262890683122, 1.000000000000000000, 0.9659258262890683122, 1.000000000000000000, 0.9659258262890683122, 1.000000000000000000, 0.9659258262890683122, 1.000000000000000000, 0.9659258262890683122, 1.000000000000000000, 0.9659258262890683122, 1.000000000000000000, 0.9659258262890683122, 1.000000000000000000, 0.9659258262890683122, 1.000000000000000000, 0.9659258262890683122, 1.000000000000000000, 0.9659258262890683122, 1.000000000000000000, 0.9659258262890683122, 1.000000000000000000, 0.9659258262890683122, 1.000000000000000000, 0.9659258262890683122, 1.000000000000000000, 0.9659258262890683122, 1.000000000000000000, 0.9659258262890683122, 1.000000000000000000, 0.9659258262890683122, 1.000000000000000000, 0.9659258262890683122, 1.000000000000000000, 0.9659258262890683122, 1.000000000000000000, 0.9659258262890683122, 1.000000000000000000, 0.9659258262890683122, 1.000000000000000000, 0.9659258262890683122, 1.000000000000000000, 0.9659258262890683122, 1.000000000000000000, 0.9659258262890683122, 1.000000000000000000, 0.9659258262890683122, 1.000000000000000000, 0.9659258262890683122, 1.000000000000000000, 0.9659258262890683122, 1.000000000000000000, 0.9659258262890683122, 1.000000000000000000, 0.9659258262890683122, 1.000000000000000000, 0.9659258262890683122, 1.000000000000000000, 0.9659258262890683122, 1.000000000000000000, 0.9659258262890683122, 1.000000000000000000, 0.9659258262890683122, 1.000000000000000000, 0.9659258262890683122, 1.000000000000000000, 0.9659258262890683122, 1.000000000000000000, 0.9659258262890683122, 1.000000000000000000, 0.9659258262890683122, 1.000000000000000000, 0.9659258262890683122, 1.000000000000000000, 0.9659258262890683122, 1.000000000000000000, 0.9659258262890683122, 1.000000000000000000, 0.9659258262890683122, 1.000000000000000000, 0.9659258262890683122, 1.000000000000000000, 0.9659258262890683122, 1.000000000000000000, 0.9659258262890683122, 1.000000000000000000, 0.9659258262890683122, 1.000000000000000000, 0.9659258262890683122, 1.000000000000000000, 0.9659258262890683122, 1.000000000000000000, 0.9659258262890683122, 1.000000000000000000, 0.9659258262890683122, 1.000000000000000000, 0.9659258262890683122, 1.000000000000000000, 0.9659258262890683122, 1.000000000000000000, 0.9659258262890683122, 1.000000000000000000, 0.9659258262890683122, 1.000000000000000000, 0.9659258262890683122, 1.000000000000000000, 0.9659258262890683122, 1.000000000000000000, 0.9659258262890683122, 1.000000000000000000, 0.9659258262890683122, 1.000000000000000000, 0.9659258262890683122, 1.000000000000000000, 0.9659258262890683122, 1.000000000000000000, 0.9659258262890683122, 1.000000000000000000, 0.9659258262890683122, 1.000000000000000000, 0.9659258262890683122, 1.000000000000000000, 0.9659258262890683122, 1.000000000000000000, 0.9659258262890683122, 1.000000000000000000, 0.9659258262890683122, 1.000000000000000000, 0.9659258262890683122, 1.000000000000000000, 0.9659258262890683122, 1.000000000000000000, 0.9659258262890683122, 1.000000000000000000, 0.9659258262890683122, 1.000000000000000000, 0.9659258262890683122, 1.000000000000000000, 0.9659258262890683122, 1.000000000000000000, 0.9659258262890683122, 1.000000000000000000, 0.9659258262890683122, 1.000000000000000000, 0.9659258262890683122, 1.000000000000000000, 0.9659258262890683122, 1.000000000000000000, 0.9659258262890683122, 1.000000000000000000, 0.9659258262890683122, 1.000000000000000000, 0.9659258262890683122, 1.000000000000000000, 0.9659258262890683122, 1.000000000000000000, 0.9659258262890683122, 1.000000000000000000, 0.9659258262890683122, 1.000000000000000000, 0.9659258262890683122, 1.000000000000000000, 0.9659258262890683122, 1.000000000000000000, 0.9659258262890683122, 1.000000000000000000, 0.9659258262890683122, 1.000000000000000000, 0.9659258262890683122, 1.000000000000000000, 0.9659258262890683122, 1.000000000000000000, 0.9659258262890683122, 1.000000000000000000, 0.9659258262890683122, 1.000000000000000000, 0.9659258262890683122, 1.000000000000000000, 0.9659258262890683122, 1.000000000000000000, 0.9659258262890683122, 1.000000000000000000, 0.9659258262890683122, 1.000000000000000000, 0.9659258262890683122, 1.000000000000000000, 0.9659258262890683122, 1.000000000000000000, 0.9659258262890683122, 1.000000000000000000, 0.9659258262890683122, 1.000000000000000000, 0.9659258262890683122, 1.000000000000000000, 0.9659258262890683122, 1.000000000000000000, 0.9659258262890683122, 1.000000000000000000, 0.9659258262890683122, 1.000000000000000000, 0.9659258262890683122, 1.000000000000000000, 0.9659258262890683122, 1.000000000000000000, 0.9659258262890683122, 1.000000000000000000, 0.9659258262890683122, 1.000000000000000000, 0.9659258262890683122, 1.000000000000000000, 0.9659258262890683122, 1.000000000000000000, 0.9659258262890683122, 1.000000000000000000, 0.9659258262890683122, 1.000000000000000000, 0.9659258262890683122, 1.000000000000000000, 0.9659258262890683122, 1.000000000000000000, 0.9659258262890683122, 1.000000000000000000, 0.9659258262890683122, 1.000000000000000000, 0.9659258262890683122, 1.000000000000000000, 0.9659258262890683122, 1.000000000000000000, 0.9659258262890683122, 1.000000000000000000, 0.9659258262890683122, 1.000000000000000000, 0.9659258262890683122, 1.000000000000000000, 0.9659258262890683122, 1.000000000000000000, 0.9659258262890683122, 1.000000000000000000, 0.9659258262890683122, 1.000000000000000000, 0.9659258262890683122, 1.000000000000000000, 0.9659258262890683122, 1.000000000000000000, 0.9659258262890683122, 1.000000000000000000, 0.9659258262890683122, 1.000000000000000000, 0.9659258262890683122, 1.000000000000000000, 0.9659258262890683122, 1.000000000000000000, 0.9659258262890683122, 1.000000000000000000, 0.9659258262890683122, 1.000000000000000000, 0.9659258262890683122, 1.000000000000000000, 0.9659258262890683122, 1.000000000000000000, 0.9659258262890683122, 1.000000000000000000, 0.9659258262890683122, 1.000000000000000000, 0.9659258262890683122, 1.000000000000000000, 0.9659258262890683122, 1.000000000000000000) ) ) 
 REPRESENTATION_ITEM ( '' )  SURFACE ( )  );
#71785=CARTESIAN_POINT ( 'NONE',  ( 0.000000000000000000, 15.00000000000000000, 0.000000000000000000 ) ) ;
#71790=AXIS2_PLACEMENT_3D ( 'NONE', #42550, #44517, #37031 ) ;
#71792=EDGE_CURVE ( 'NONE', #34469, #83674, #35717, .T. ) ;
#71794=CARTESIAN_POINT ( 'NONE',  ( -13.82671409943298357, -0.03417435944610275333, 3.447387012295131115 ) ) ;
#71795=ORIENTED_EDGE ( 'NONE', *, *, #32623, .T. ) ;
#71797=ADVANCED_FACE ( 'NONE', ( #64717 ), #36528, .T. ) ;
#71816=CARTESIAN_POINT ( 'NONE',  ( -14.36343418943216577, 0.04922511925147166761, 3.367173657400553743 ) ) ;
#71821=ADVANCED_FACE ( 'NONE', ( #65214 ), #64229, .F. ) ;
#71833=DIRECTION ( 'NONE',  ( -0.7253743710122912969, 0.000000000000000000, 0.6883545756937501370 ) ) ;
#71838=ORIENTED_EDGE ( 'NONE', *, *, #27831, .F. ) ;
#71841=CARTESIAN_POINT ( 'NONE',  ( 0.000000000000000000, 15.00000000000000000, 0.000000000000000000 ) ) ;
#71843=VERTEX_POINT ( 'NONE', #50730 ) ;
#71846=DIRECTION ( 'NONE',  ( -0.000000000000000000, -1.000000000000000000, -0.000000000000000000 ) ) ;
#71847=CARTESIAN_POINT ( 'NONE',  ( 0.000000000000000000, 15.00000000000000000, 0.000000000000000000 ) ) ;
#71854=ORIENTED_EDGE ( 'NONE', *, *, #75076, .T. ) ;
#71858=CARTESIAN_POINT ( 'NONE',  ( -10.64017930668191170, 0.5000000000000004441, -10.57291749337230158 ) ) ;
#71865=EDGE_CURVE ( 'NONE', #29178, #28808, #74836, .T. ) ;
#71867=DIRECTION ( 'NONE',  ( 0.000000000000000000, 0.000000000000000000, 1.000000000000000000 ) ) ;
#71871=VERTEX_POINT ( 'NONE', #27718 ) ;
#71875=CARTESIAN_POINT ( 'NONE',  ( -1.087200977609965147, 0.000000000000000000, 5.343763529286919223 ) ) ;
#71877=CARTESIAN_POINT ( 'NONE',  ( -13.14228782657336581, 14.49999999999999112, -7.230509711182429022 ) ) ;
#71882=ORIENTED_EDGE ( 'NONE', *, *, #86174, .T. ) ;
#71895=FACE_OUTER_BOUND ( 'NONE', #43329, .T. ) ;
#71903=CARTESIAN_POINT ( 'NONE',  ( -10.36894250292378317, 7.428748834913971422, 10.36894250292379560 ) ) ;
#71907=EDGE_CURVE ( 'NONE', #2489, #84641, #79758, .T. ) ;
#71908=B_SPLINE_CURVE_WITH_KNOTS ( 'NONE', 3,
 ( #40597, #1132, #54101, #70106, #1631, #71094 ),
 .UNSPECIFIED., .F., .F.,
 ( 4, 2, 4 ),
 ( 0.0002800591277523079015, 0.0006862649357714276999, 0.001092470743790547498 ),
 .UNSPECIFIED. ) ;
#71912=CARTESIAN_POINT ( 'NONE',  ( -13.61464873478171533, 15.00000000000000000, 6.296136897217742501 ) ) ;
#71917=CARTESIAN_POINT ( 'NONE',  ( 10.84451454130507209, 15.00000000000000000, -9.625305416630832056 ) ) ;
#71933=EDGE_CURVE ( 'NONE', #44443, #94977, #87727, .T. ) ;
#71934=VECTOR ( 'NONE', #5717, 1000.000000000000000 ) ;
#71935=EDGE_LOOP ( 'NONE', ( #36957, #95589, #90708, #22258, #55313, #80501 ) ) ;
#71944=CARTESIAN_POINT ( 'NONE',  ( 0.000000000000000000, 15.00000000000000000, 0.000000000000000000 ) ) ;
#71950=AXIS2_PLACEMENT_3D ( 'NONE', #70089, #78075, #639 ) ;
#71952=VERTEX_POINT ( 'NONE', #13213 ) ;
#71956=FACE_OUTER_BOUND ( 'NONE', #39560, .T. ) ;
#71958=CARTESIAN_POINT ( 'NONE',  ( 13.14228782657338535, 0.3639308284105124969, 7.230509711182335764 ) ) ;
#71961=CARTESIAN_POINT ( 'NONE',  ( -8.470897558477686218, 15.00000000000000888, 11.92401951126073278 ) ) ;
#71968=LINE ( 'NONE', #3012, #57207 ) ;
#71970=DIRECTION ( 'NONE',  ( 0.9426414910921736556, 0.000000000000000000, 0.3338068592337842255 ) ) ;
#71972=CARTESIAN_POINT ( 'NONE',  ( 3.434112377981054287, -37.33469866340291077, -12.81628187352647608 ) ) ;
#71980=CARTESIAN_POINT ( 'NONE',  ( -2.962741594152892510, 15.00000000000000000, -13.93860331045676837 ) ) ;
#71987=TOROIDAL_SURFACE ( 'NONE', #87971, 14.49999999999999822, 0.5000000000000000000 ) ;
#71994=EDGE_CURVE ( 'NONE', #92979, #11604, #74913, .T. ) ;
#71998=VERTEX_POINT ( 'NONE', #6704 ) ;
#72002=CARTESIAN_POINT ( 'NONE',  ( -12.11331110855146953, 14.95077488074853456, 8.421032842869358603 ) ) ;
#72004=B_SPLINE_CURVE_WITH_KNOTS ( 'NONE', 3,
 ( #90749, #51774, #45253, #52751, #97798, #29260 ),
 .UNSPECIFIED., .F., .F.,
 ( 4, 2, 4 ),
 ( 0.0002800452451363289125, 0.0006862509172491817848, 0.001092456589362034549 ),
 .UNSPECIFIED. ) ;
#72015=AXIS2_PLACEMENT_3D ( 'NONE', #62810, #63778, #94288 ) ;
#72022=CARTESIAN_POINT ( 'NONE',  ( -10.36894250292378317, -32.57125116508603213, 10.36894250292379560 ) ) ;
#72024=EDGE_CURVE ( 'NONE', #1780, #11601, #28588, .T. ) ;
#72040=CARTESIAN_POINT ( 'NONE',  ( -2.915334737309934532, 12.02201867748817499, -10.88017736071109987 ) ) ;
#72042=CARTESIAN_POINT ( 'NONE',  ( -3.822225673302299676, 0.000000000000000000, 3.889525102760206909 ) ) ;
#72046=CARTESIAN_POINT ( 'NONE',  ( -6.689969769698787871, 15.00000000000000000, -12.58200319823979285 ) ) ;
#72050=DIRECTION ( 'NONE',  ( 0.000000000000000000, 1.000000000000000000, 0.000000000000000000 ) ) ;
#72057=AXIS2_PLACEMENT_3D ( 'NONE', #29997, #60504, #67025 ) ;
#72059=VERTEX_POINT ( 'NONE', #28707 ) ;
#72083=LINE ( 'NONE', #64566, #12531 ) ;
#72084=CARTESIAN_POINT ( 'NONE',  ( -2.638427012816840111, 4.967264484334121377, -9.846743663894590881 ) ) ;
#72085=ORIENTED_EDGE ( 'NONE', *, *, #73858, .T. ) ;
#72089=ORIENTED_EDGE ( 'NONE', *, *, #6776, .T. ) ;
#72098=EDGE_LOOP ( 'NONE', ( #25793, #56036, #65987, #20697 ) ) ;
#72110=AXIS2_PLACEMENT_3D ( 'NONE', #8598, #68126, #84110 ) ;
#72121=FACE_OUTER_BOUND ( 'NONE', #48308, .T. ) ;
#72123=CARTESIAN_POINT ( 'NONE',  ( 6.382347221874381304, 14.49999999999999112, 13.57444820018236520 ) ) ;
#72126=AXIS2_PLACEMENT_3D ( 'NONE', #83082, #98618, #60576 ) ;
#72131=DIRECTION ( 'NONE',  ( 0.000000000000000000, 1.000000000000000000, 0.000000000000000000 ) ) ;
#72134=CARTESIAN_POINT ( 'NONE',  ( 4.873787042390789637, -0.03417435944610275333, -13.39061984619918988 ) ) ;
#72139=CARTESIAN_POINT ( 'NONE',  ( 0.000000000000000000, 14.49999999999999822, 0.000000000000000000 ) ) ;
#72142=FACE_OUTER_BOUND ( 'NONE', #65800, .T. ) ;
#72144=CARTESIAN_POINT ( 'NONE',  ( 13.34948392230371361, 14.95077488074853456, 6.279918722515068552 ) ) ;
#72148=CARTESIAN_POINT ( 'NONE',  ( 7.964842623401177768, -28.81131465584515539, -7.964842623401181321 ) ) ;
#72153=DIRECTION ( 'NONE',  ( 0.000000000000000000, 0.000000000000000000, 1.000000000000000000 ) ) ;
#72166=CARTESIAN_POINT ( 'NONE',  ( 14.82629065241282262, 14.76984952913051430, 1.844815641835429121 ) ) ;
#72179=CYLINDRICAL_SURFACE ( 'NONE', #4837, 15.00000000000000000 ) ;
#72181=EDGE_LOOP ( 'NONE', ( #28675, #9645, #57574, #92217 ) ) ;
#72184=ORIENTED_EDGE ( 'NONE', *, *, #88912, .F. ) ;
#72186=CARTESIAN_POINT ( 'NONE',  ( 6.382347221874334231, 0.5000000000000004441, 13.57444820018231724 ) ) ;
#72203=CARTESIAN_POINT ( 'NONE',  ( 8.527530157486179263, -31.90773551566587685, 4.923371831947292776 ) ) ;
#72204=ORIENTED_EDGE ( 'NONE', *, *, #505, .F. ) ;
#72209=ORIENTED_EDGE ( 'NONE', *, *, #17841, .F. ) ;
#72216=CARTESIAN_POINT ( 'NONE',  ( -12.81628187352647608, 14.12363466993042671, 3.903127820947815962E-15 ) ) ;
#72220=ORIENTED_EDGE ( 'NONE', *, *, #18920, .T. ) ;
#72221=VERTEX_POINT ( 'NONE', #23202 ) ;
#72231=AXIS2_PLACEMENT_3D ( 'NONE', #95981, #42969, #36455 ) ;
#72232=CARTESIAN_POINT ( 'NONE',  ( -3.115783986955657614, 15.00000000000000000, 14.16128137375395468 ) ) ;
#72233=DIRECTION ( 'NONE',  ( -8.704148513061227277E-14, 0.000000000000000000, 1.000000000000000000 ) ) ;
#72236=FACE_OUTER_BOUND ( 'NONE', #5769, .T. ) ;
#72243=CARTESIAN_POINT ( 'NONE',  ( 7.640917710488917436, 0.04922511925146979411, 12.61992379908760853 ) ) ;
#72246=FACE_OUTER_BOUND ( 'NONE', #78449, .T. ) ;
#72254=ADVANCED_FACE ( 'NONE', ( #9163 ), #17175, .F. ) ;
#72263=CIRCLE ( 'NONE', #61061, 14.49999999999999822 ) ;
#72270=DIRECTION ( 'NONE',  ( 0.000000000000000000, 0.000000000000000000, -1.000000000000000000 ) ) ;
#72273=FACE_OUTER_BOUND ( 'NONE', #74009, .T. ) ;
#72276=DIRECTION ( 'NONE',  ( 0.000000000000000000, 1.000000000000000000, 0.000000000000000000 ) ) ;
#72279=CARTESIAN_POINT ( 'NONE',  ( -8.470897558477446410, 2.337810934421868936E-16, -11.92401951126092641 ) ) ;
#72306=CARTESIAN_POINT ( 'NONE',  ( 12.83294900548068007, 14.49999999999999112, -7.766300266068417280 ) ) ;
#72346=ORIENTED_EDGE ( 'NONE', *, *, #3302, .F. ) ;
#72349=ORIENTED_EDGE ( 'NONE', *, *, #19545, .F. ) ;
#72351=EDGE_CURVE ( 'NONE', #1450, #76280, #84442, .T. ) ;
#72356=CARTESIAN_POINT ( 'NONE',  ( 13.48255862861927312, 3.989652714533045580E-16, -5.335786055104159153 ) ) ;
#72367=EDGE_CURVE ( 'NONE', #84883, #3732, #67462, .T. ) ;
#72381=CARTESIAN_POINT ( 'NONE',  ( 14.02068044289381987, 14.49999999999999112, 5.331089937175756077 ) ) ;
#72384=ORIENTED_EDGE ( 'NONE', *, *, #56910, .T. ) ;
#72396=AXIS2_PLACEMENT_3D ( 'NONE', #56152, #86155, #3151 ) ;
#72398=DIRECTION ( 'NONE',  ( 0.9969173337331289630, 0.000000000000000000, -0.07845909572783234254 ) ) ;
#72400=ORIENTED_EDGE ( 'NONE', *, *, #61197, .T. ) ;
#72401=AXIS2_PLACEMENT_3D ( 'NONE', #22482, #52956, #53447 ) ;
#72407=CARTESIAN_POINT ( 'NONE',  ( -1.354709868695754826, 14.49999999999999112, 14.93870011653156915 ) ) ;
#72424=ORIENTED_EDGE ( 'NONE', *, *, #50446, .T. ) ;
#72436=CARTESIAN_POINT ( 'NONE',  ( 14.03351048042395632, -0.03417435944610275333, 2.474486531753810059 ) ) ;
#72448=DIRECTION ( 'NONE',  ( 0.000000000000000000, 1.000000000000000000, 0.000000000000000000 ) ) ;
#72450=EDGE_CURVE ( 'NONE', #40259, #33221, #97983, .T. ) ;
#72453=CARTESIAN_POINT ( 'NONE',  ( -11.09922568453594316, -30.45969866340291077, 6.408140936763246920 ) ) ;
#72462=FACE_OUTER_BOUND ( 'NONE', #12801, .T. ) ;
#72464=B_SPLINE_CURVE_WITH_KNOTS ( 'NONE', 3,
 ( #74695, #30167, #60671, #91169, #76177, #7698 ),
 .UNSPECIFIED., .F., .F.,
 ( 4, 2, 4 ),
 ( 3.409110551496077158E-05, 0.0004400426677367853790, 0.0008459942299586099661 ),
 .UNSPECIFIED. ) ;
#72467=EDGE_CURVE ( 'NONE', #60570, #11086, #82955, .T. ) ;
#72473=TOROIDAL_SURFACE ( 'NONE', #35802, 14.49999999999999822, 0.5000000000000000000 ) ;
#72474=ORIENTED_EDGE ( 'NONE', *, *, #31618, .T. ) ;
#72481=CARTESIAN_POINT ( 'NONE',  ( 14.48718990079892599, 4.585916678612670543E-16, -0.6093675230840440715 ) ) ;
#72484=ORIENTED_EDGE ( 'NONE', *, *, #89151, .F. ) ;
#72485=CARTESIAN_POINT ( 'NONE',  ( 5.806616290881322584, 15.00000000000000533, 13.42355087257366364 ) ) ;
#72487=EDGE_LOOP ( 'NONE', ( #10466, #18369, #52079, #91176 ) ) ;
#72496=LINE ( 'NONE', #65488, #27454 ) ;
#72499=ORIENTED_EDGE ( 'NONE', *, *, #37042, .T. ) ;
#72508=FACE_OUTER_BOUND ( 'NONE', #58753, .T. ) ;
#72523=CARTESIAN_POINT ( 'NONE',  ( 10.88017736071110164, 10.35535201082150181, 2.915334737309921209 ) ) ;
#72528=DIRECTION ( 'NONE',  ( 0.000000000000000000, 0.000000000000000000, 1.000000000000000000 ) ) ;
#72529=VECTOR ( 'NONE', #7471, 999.9999999999998863 ) ;
#72534=DIRECTION ( 'NONE',  ( -3.907985046680551022E-14, 0.000000000000000000, 1.000000000000000000 ) ) ;
#72535=CARTESIAN_POINT ( 'NONE',  ( 0.000000000000000000, 0.5000000000000004441, 0.000000000000000000 ) ) ;
#72537=ORIENTED_EDGE ( 'NONE', *, *, #83383, .T. ) ;
#72539=CIRCLE ( 'NONE', #16679, 14.49999999999999822 ) ;
#72541=FACE_OUTER_BOUND ( 'NONE', #38592, .T. ) ;
#72548=DIRECTION ( 'NONE',  ( -0.000000000000000000, -1.000000000000000000, -0.000000000000000000 ) ) ;
#72550=ADVANCED_FACE ( 'NONE', ( #83939 ), #45948, .F. ) ;
#72551=B_SPLINE_CURVE_WITH_KNOTS ( 'NONE', 3,
 ( #71917, #80900, #94419, #18436, #34893, #4427 ),
 .UNSPECIFIED., .F., .F.,
 ( 4, 2, 4 ),
 ( 0.0002800138956475372188, 0.0006862192609879400919, 0.001092424626328342965 ),
 .UNSPECIFIED. ) ;
#72555=ORIENTED_EDGE ( 'NONE', *, *, #18341, .T. ) ;
#72565=CARTESIAN_POINT ( 'NONE',  ( -9.846743663894590881, 1.217264484334116492, 2.638427012816840111 ) ) ;
#72566=VERTEX_POINT ( 'NONE', #46429 ) ;
#72571=VERTEX_POINT ( 'NONE', #38940 ) ;
#72577=CARTESIAN_POINT ( 'NONE',  ( 0.000000000000000000, 0.000000000000000000, 0.000000000000000000 ) ) ;
#72579=ADVANCED_FACE ( 'NONE', ( #39918 ), #17053, .T. ) ;
#72580=B_SPLINE_CURVE_WITH_KNOTS ( 'NONE', 3,
 ( #23542, #77009, #8521, #52049, #16523, #40001 ),
 .UNSPECIFIED., .F., .F.,
 ( 4, 2, 4 ),
 ( 3.409110551494299067E-05, 0.0004400426677367894448, 0.0008459942299586358785 ),
 .UNSPECIFIED. ) ;
#72582=ADVANCED_FACE ( 'NONE', ( #48878 ), #36161, .T. ) ;
#72583=VERTEX_POINT ( 'NONE', #78894 ) ;
#72587=ORIENTED_EDGE ( 'NONE', *, *, #50275, .T. ) ;
#72594=VERTEX_POINT ( 'NONE', #40910 ) ;
#72597=EDGE_LOOP ( 'NONE', ( #80681, #91048, #46942, #48829 ) ) ;
#72603=LINE ( 'NONE', #27107, #52355 ) ;
#72609=ORIENTED_EDGE ( 'NONE', *, *, #6234, .F. ) ;
#72615=DIRECTION ( 'NONE',  ( 0.000000000000000000, 0.000000000000000000, 1.000000000000000000 ) ) ;
#72619=TOROIDAL_SURFACE ( 'NONE', #5573, 14.49999999999999822, 0.5000000000000000000 ) ;
#72629=LINE ( 'NONE', #37127, #26453 ) ;
#72632=CARTESIAN_POINT ( 'NONE',  ( -7.964842623401172439, -21.31131465584516249, 7.964842623401183097 ) ) ;
#72636=CARTESIAN_POINT ( 'NONE',  ( -1.915564264621539392, 15.00000000000000000, 14.37291249357986445 ) ) ;
#72660=LINE ( 'NONE', #49665, #28797 ) ;
#72662=B_SPLINE_CURVE_WITH_KNOTS ( 'NONE', 3,
 ( #76888, #47372, #23910, #61389, #91898, #84410 ),
 .UNSPECIFIED., .F., .F.,
 ( 4, 2, 4 ),
 ( 0.0002800026249563253040, 0.0006862078800502578041, 0.001092413135144190304 ),
 .UNSPECIFIED. ) ;
#72665=CARTESIAN_POINT ( 'NONE',  ( -4.841283923550251167, 0.2306972965111909746, -14.13506365971153222 ) ) ;
#72666=ORIENTED_EDGE ( 'NONE', *, *, #18651, .T. ) ;
#72679=VECTOR ( 'NONE', #80369, 1000.000000000000114 ) ;
#72683=CARTESIAN_POINT ( 'NONE',  ( -2.638427012816840111, -35.03273551566588395, -9.846743663894590881 ) ) ;
#72688=ORIENTED_EDGE ( 'NONE', *, *, #83458, .F. ) ;
#72694=ADVANCED_FACE ( 'NONE', ( #39434 ), #93684, .T. ) ;
#72695=AXIS2_PLACEMENT_3D ( 'NONE', #91733, #15263, #53730 ) ;
#72697=CARTESIAN_POINT ( 'NONE',  ( 6.408140936763236262, 7.456968003263758860, -11.09922568453595026 ) ) ;
#72698=ADVANCED_FACE ( 'NONE', ( #2926 ), #68152, .T. ) ;
#72699=ORIENTED_EDGE ( 'NONE', *, *, #28024, .F. ) ;
#72709=VECTOR ( 'NONE', #80875, 1000.000000000000114 ) ;
#72713=EDGE_CURVE ( 'NONE', #42602, #66663, #28165, .T. ) ;
#72714=CARTESIAN_POINT ( 'NONE',  ( 0.000000000000000000, 0.000000000000000000, 0.000000000000000000 ) ) ;
#72716=CARTESIAN_POINT ( 'NONE',  ( 13.75543905097463337, 0.04962897369418881044, 5.333404663735670681 ) ) ;
#72719=LINE ( 'NONE', #50219, #54630 ) ;
#72726=CARTESIAN_POINT ( 'NONE',  ( -10.19513985507820486, 14.49999999999999112, -11.00268709613237306 ) ) ;
#72727=DIRECTION ( 'NONE',  ( -0.6626200482157305061, 0.000000000000000000, -0.7489557207890082946 ) ) ;
#72730=DIRECTION ( 'NONE',  ( -0.000000000000000000, 1.000000000000000000, -0.000000000000000000 ) ) ;
#72735=CARTESIAN_POINT ( 'NONE',  ( 11.22915323889574601, 15.00000000000000000, 8.773176023390684364 ) ) ;
#72739=EDGE_LOOP ( 'NONE', ( #90275, #32969, #73590, #24683, #90393, #90418 ) ) ;
#72740=CARTESIAN_POINT ( 'NONE',  ( -11.25000000000000178, 2.713468844518205803, -3.014428414850123250 ) ) ;
#72744=CARTESIAN_POINT ( 'NONE',  ( 12.50534872682727539, 3.894361491432412218E-16, 7.339363270777609749 ) ) ;
#72747=DIRECTION ( 'NONE',  ( -0.8241261886220129229, 0.000000000000000000, -0.5664062369248369366 ) ) ;
#72764=CARTESIAN_POINT ( 'NONE',  ( 7.551349515323185990, 0.000000000000000000, -12.08468537022906020 ) ) ;
#72765=DIRECTION ( 'NONE',  ( -0.9636304532086211738, 0.000000000000000000, -0.2672383760782636175 ) ) ;
#72777=ADVANCED_BREP_SHAPE_REPRESENTATION ( '', ( #8224, #27931 ), #10314 ) ;
#72783=EDGE_CURVE ( 'NONE', #9285, #26361, #88364, .T. ) ;
#72787=DIRECTION ( 'NONE',  ( 0.000000000000000000, 1.000000000000000000, 0.000000000000000000 ) ) ;
#72793=FACE_OUTER_BOUND ( 'NONE', #60492, .T. ) ;
#72805=CARTESIAN_POINT ( 'NONE',  ( -9.281709892946317098, 15.00000000000000711, -11.30302492080718579 ) ) ;
#72813=EDGE_CURVE ( 'NONE', #63992, #23413, #73844, .T. ) ;
#72814=LINE ( 'NONE', #4354, #48378 ) ;
#72819=VECTOR ( 'NONE', #29787, 1000.000000000000000 ) ;
#72825=ORIENTED_EDGE ( 'NONE', *, *, #63090, .F. ) ;
#72826=DIRECTION ( 'NONE',  ( -0.000000000000000000, -1.000000000000000000, -0.000000000000000000 ) ) ;
#72828=DIRECTION ( 'NONE',  ( 0.8703556959399044723, 0.000000000000000000, -0.4924235601034586685 ) ) ;
#72831=CARTESIAN_POINT ( 'NONE',  ( -5.888281321711915872, 1.823139558123406223, -10.37198838585826266 ) ) ;
#72836=CARTESIAN_POINT ( 'NONE',  ( 14.71525861348293596, 14.49999999999999112, 2.908807992686717192 ) ) ;
#72837=ORIENTED_EDGE ( 'NONE', *, *, #83556, .T. ) ;
#72843=ADVANCED_FACE ( 'NONE', ( #5853 ), #20363, .F. ) ;
#72845=CARTESIAN_POINT ( 'NONE',  ( 10.39692778084932812, 0.04962893796709086369, 10.46714871971205696 ) ) ;
#72857=VERTEX_POINT ( 'NONE', #41899 ) ;
#72861=CARTESIAN_POINT ( 'NONE',  ( 8.235571585149866536, 8.243033628982649574, -8.235571585149871865 ) ) ;
#72866=CARTESIAN_POINT ( 'NONE',  ( 9.240973841163532043, 4.236086333263440692E-16, 11.17382667070378943 ) ) ;
#72875=CARTESIAN_POINT ( 'NONE',  ( 0.000000000000000000, 1.823139558123437975, 0.000000000000000000 ) ) ;
#72877=VECTOR ( 'NONE', #25696, 1000.000000000000000 ) ;
#72881=AXIS2_PLACEMENT_3D ( 'NONE', #83229, #7240, #30212 ) ;
#72883=CARTESIAN_POINT ( 'NONE',  ( 14.62129639376011170, 15.00000000000000711, -0.3552502084985190156 ) ) ;
#72884=AXIS2_PLACEMENT_3D ( 'NONE', #91279, #24280, #22800 ) ;
#72888=CARTESIAN_POINT ( 'NONE',  ( 0.000000000000000000, 15.00000000000000000, 0.000000000000000000 ) ) ;
#72893=LINE ( 'NONE', #10927, #94364 ) ;
#72902=DIRECTION ( 'NONE',  ( 0.000000000000000000, 1.000000000000000000, 0.000000000000000000 ) ) ;
#72904=( BOUNDED_CURVE ( )  B_SPLINE_CURVE ( 2, ( #93489, #24026, #54494, #85009, #39518 ),
 .UNSPECIFIED., .F., .T. ) 
 B_SPLINE_CURVE_WITH_KNOTS ( ( 3, 2, 3 ),
 ( 0.6666666666666666297, 0.6722222222222222765, 0.6777069814160940897 ),
 .UNSPECIFIED. ) 
 CURVE ( )  GEOMETRIC_REPRESENTATION_ITEM ( )  RATIONAL_B_SPLINE_CURVE ( ( 1.000000000000000000, 0.9659258262890683122, 1.000000000000000000, 0.9663600452437686172, 0.9991426288945792766 ) ) 
 REPRESENTATION_ITEM ( '' )  );
#72914=EDGE_CURVE ( 'NONE', #88979, #9752, #3893, .T. ) ;
#72915=AXIS2_PLACEMENT_3D ( 'NONE', #91201, #52713, #6728 ) ;
#72916=VECTOR ( 'NONE', #22964, 1000.000000000000000 ) ;
#72924=LINE ( 'NONE', #4454, #78145 ) ;
#72931=ORIENTED_EDGE ( 'NONE', *, *, #73087, .T. ) ;
#72942=CARTESIAN_POINT ( 'NONE',  ( 0.000000000000000000, 0.000000000000000000, 0.000000000000000000 ) ) ;
#72946=FACE_OUTER_BOUND ( 'NONE', #31265, .T. ) ;
#72951=CARTESIAN_POINT ( 'NONE',  ( -12.81628187352647963, -36.08469866340291787, -3.434112377981046293 ) ) ;
#72959=CARTESIAN_POINT ( 'NONE',  ( 0.000000000000000000, 15.00000000000000000, 0.000000000000000000 ) ) ;
#72960=VECTOR ( 'NONE', #96621, 1000.000000000000000 ) ;
#72962=ORIENTED_EDGE ( 'NONE', *, *, #71757, .T. ) ;
#72964=DIRECTION ( 'NONE',  ( 0.3173046564050898688, 0.000000000000000000, 0.9483236552061999891 ) ) ;
#72970=APPLICATION_CONTEXT ( 'automotive_design' ) ;
#72976=AXIS2_PLACEMENT_3D ( 'NONE', #76065, #6584, #44579 ) ;
#72977=FACE_OUTER_BOUND ( 'NONE', #91165, .T. ) ;
#72987=PLANE ( 'NONE',  #42349 ) ;
#72993=CARTESIAN_POINT ( 'NONE',  ( -5.240416992896902215, 0.04922511925148113227, 13.79072622793298208 ) ) ;
#73000=CARTESIAN_POINT ( 'NONE',  ( 2.120353041430647512, 4.078855811979330250E-16, -14.34413130794945523 ) ) ;
#73002=CARTESIAN_POINT ( 'NONE',  ( 3.469446951953614189E-15, -36.94625116508602503, 14.16423886937410259 ) ) ;
#73006=CARTESIAN_POINT ( 'NONE',  ( -3.836325488036278930, 0.5000000000000004441, 14.50112432709419785 ) ) ;
#73012=CARTESIAN_POINT ( 'NONE',  ( -14.88232117145534517, 14.49999999999999112, -1.875237731503371030 ) ) ;
#73016=CARTESIAN_POINT ( 'NONE',  ( -5.440088680355558814, 12.23035201082151069, -9.422509992056136596 ) ) ;
#73020=ADVANCED_FACE ( 'NONE', ( #15958 ), #18792, .T. ) ;
#73024=DIRECTION ( 'NONE',  ( 0.000000000000000000, 0.000000000000000000, 1.000000000000000000 ) ) ;
#73027=EDGE_CURVE ( 'NONE', #18735, #19349, #91459, .T. ) ;
#73036=CARTESIAN_POINT ( 'NONE',  ( -11.61621867929619611, -0.03417435944610275333, 10.99731149103378058 ) ) ;
#73039=VECTOR ( 'NONE', #77521, 1000.000000000000227 ) ;
#73046=CIRCLE ( 'NONE', #95474, 15.00000000000000000 ) ;
#73048=B_SPLINE_CURVE_WITH_KNOTS ( 'NONE', 3,
 ( #95390, #80882, #94403, #13743, #18414, #44226 ),
 .UNSPECIFIED., .F., .F.,
 ( 4, 2, 4 ),
 ( 0.0002800912045164367708, 0.0006862973266905153438, 0.001092503448864594025 ),
 .UNSPECIFIED. ) ;
#73049=AXIS2_PLACEMENT_3D ( 'NONE', #51792, #67790, #97313 ) ;
#73051=EDGE_LOOP ( 'NONE', ( #59647, #38169, #73884, #5037 ) ) ;
#73056=CARTESIAN_POINT ( 'NONE',  ( -13.48255862861931043, 4.084149796850864849E-16, 5.335786055104065007 ) ) ;
#73059=CARTESIAN_POINT ( 'NONE',  ( -10.70613742633244669, 15.00000000000000000, -9.778988772285387654 ) ) ;
#73063=CARTESIAN_POINT ( 'NONE',  ( 2.638427012816835227, 2.467264484334120045, 9.846743663894590881 ) ) ;
#73064=ORIENTED_EDGE ( 'NONE', *, *, #67558, .T. ) ;
#73065=ORIENTED_EDGE ( 'NONE', *, *, #14870, .T. ) ;
#73066=VERTEX_POINT ( 'NONE', #53952 ) ;
#73075=ORIENTED_EDGE ( 'NONE', *, *, #75639, .F. ) ;
#73086=FACE_OUTER_BOUND ( 'NONE', #52199, .T. ) ;
#73087=EDGE_CURVE ( 'NONE', #38851, #36587, #7973, .T. ) ;
#73088=VECTOR ( 'NONE', #53632, 1000.000000000000227 ) ;
#73092=FACE_OUTER_BOUND ( 'NONE', #65960, .T. ) ;
#73095=ORIENTED_EDGE ( 'NONE', *, *, #74328, .T. ) ;
#73096=CARTESIAN_POINT ( 'NONE',  ( 0.000000000000000000, 0.000000000000000000, 0.000000000000000000 ) ) ;
#73097=CARTESIAN_POINT ( 'NONE',  ( 14.54804176595378706, -0.03417435944610275333, 6.650705016170673112 ) ) ;
#73106=DIRECTION ( 'NONE',  ( 0.000000000000000000, 1.000000000000000000, 0.000000000000000000 ) ) ;
#73111=VERTEX_POINT ( 'NONE', #41313 ) ;
#73124=CARTESIAN_POINT ( 'NONE',  ( -9.422509992056136596, -21.51964798917849109, 5.440088680355559703 ) ) ;
#73127=EDGE_CURVE ( 'NONE', #70759, #46734, #22985, .T. ) ;
#73129=DIRECTION ( 'NONE',  ( 0.000000000000000000, 0.000000000000000000, 1.000000000000000000 ) ) ;
#73131=CARTESIAN_POINT ( 'NONE',  ( 1.915564264621337776, 15.00000000000000000, 14.37291249357991774 ) ) ;
#73135=ADVANCED_FACE ( 'NONE', ( #11274 ), #68476, .F. ) ;
#73139=FACE_OUTER_BOUND ( 'NONE', #53905, .T. ) ;
#73141=EDGE_CURVE ( 'NONE', #57214, #44552, #32303, .T. ) ;
#73154=DIRECTION ( 'NONE',  ( -0.5948227867513371514, 0.000000000000000000, -0.8038568606172203923 ) ) ;
#73155=CARTESIAN_POINT ( 'NONE',  ( 8.209432707284861408, 0.5000000000000004441, -12.55409154915486170 ) ) ;
#73161=ORIENTED_EDGE ( 'NONE', *, *, #89986, .T. ) ;
#73163=CARTESIAN_POINT ( 'NONE',  ( 9.742785792574936821, 10.83846884451820891, -5.625000000000004441 ) ) ;
#73176=CYLINDRICAL_SURFACE ( 'NONE', #21079, 15.00000000000000000 ) ;
#73178=EDGE_CURVE ( 'NONE', #88806, #83600, #25800, .T. ) ;
#73180=LINE ( 'NONE', #95195, #15818 ) ;
#73181=ORIENTED_EDGE ( 'NONE', *, *, #40008, .T. ) ;
#73183=VERTEX_POINT ( 'NONE', #18296 ) ;
#73189=DIRECTION ( 'NONE',  ( 0.8870108331782150524, 0.000000000000000000, 0.4617486132350466788 ) ) ;
#73192=B_SPLINE_CURVE_WITH_KNOTS ( 'NONE', 3,
 ( #58922, #49945, #12926, #19937, #20935, #43421 ),
 .UNSPECIFIED., .F., .F.,
 ( 4, 2, 4 ),
 ( 3.409110551495123060E-05, 0.0004400426677367748622, 0.0008459942299585984735 ),
 .UNSPECIFIED. ) ;
#73195=CARTESIAN_POINT ( 'NONE',  ( 12.81628187352647252, 1.831968003263755085, -3.434112377981059172 ) ) ;
#73196=ORIENTED_EDGE ( 'NONE', *, *, #74509, .T. ) ;
#73200=ORIENTED_EDGE ( 'NONE', *, *, #81181, .T. ) ;
#73205=CYLINDRICAL_SURFACE ( 'NONE', #76709, 15.00000000000000000 ) ;
#73208=VERTEX_POINT ( 'NONE', #48779 ) ;
#73209=FACE_OUTER_BOUND ( 'NONE', #32212, .T. ) ;
#73212=DIRECTION ( 'NONE',  ( 0.000000000000000000, 1.000000000000000000, 0.000000000000000000 ) ) ;
#73215=CARTESIAN_POINT ( 'NONE',  ( 0.000000000000000000, 14.49999999999999822, 0.000000000000000000 ) ) ;
#73218=AXIS2_PLACEMENT_3D ( 'NONE', #26672, #12654, #88157 ) ;
#73220=CARTESIAN_POINT ( 'NONE',  ( 7.313705784284555200, 14.49999999999999112, 13.09617149020753146 ) ) ;
#73224=DIRECTION ( 'NONE',  ( 0.000000000000000000, 1.000000000000000000, 0.000000000000000000 ) ) ;
#73229=EDGE_CURVE ( 'NONE', #13064, #56877, #20260, .T. ) ;
#73235=CARTESIAN_POINT ( 'NONE',  ( -2.189666204609396427, -2.219226321806264916E-16, 14.46180170876166748 ) ) ;
#73237=ORIENTED_EDGE ( 'NONE', *, *, #27324, .T. ) ;
#73246=PLANE ( 'NONE',  #30329 ) ;
#73247=CARTESIAN_POINT ( 'NONE',  ( -4.020549461440724670, 0.000000000000000000, -3.684154808197088293 ) ) ;
#73250=CYLINDRICAL_SURFACE ( 'NONE', #78117, 15.00000000000000000 ) ;
#73253=DIRECTION ( 'NONE',  ( -0.000000000000000000, -1.000000000000000000, -0.000000000000000000 ) ) ;
#73261=EDGE_LOOP ( 'NONE', ( #63623, #28413, #57824, #9836 ) ) ;
#73264=PLANE ( 'NONE',  #40395 ) ;
#73274=DIRECTION ( 'NONE',  ( -0.000000000000000000, -1.000000000000000000, -0.000000000000000000 ) ) ;
#73280=CARTESIAN_POINT ( 'NONE',  ( 0.000000000000000000, 14.49999999999999822, 0.000000000000000000 ) ) ;
#73281=CARTESIAN_POINT ( 'NONE',  ( -9.159723438033276821, 15.00000000000000000, 10.91613331444536250 ) ) ;
#73291=CARTESIAN_POINT ( 'NONE',  ( 6.898461952320343649, 4.875757609050324087E-16, 12.75387089053313971 ) ) ;
#73301=CARTESIAN_POINT ( 'NONE',  ( 3.753761956877445627, 0.000000000000000000, 3.955639745193266776 ) ) ;
#73303=ADVANCED_FACE ( 'NONE', ( #49779 ), #48305, .F. ) ;
#73309=EDGE_LOOP ( 'NONE', ( #13680, #17765, #95359, #42667 ) ) ;
#73311=CARTESIAN_POINT ( 'NONE',  ( 13.55101055326455928, 14.76984994142753038, -6.292244619294638852 ) ) ;
#73312=CARTESIAN_POINT ( 'NONE',  ( 4.873787042390699931, -0.03417435944610275333, 13.39061984619922718 ) ) ;
#73313=ORIENTED_EDGE ( 'NONE', *, *, #52279, .T. ) ;
#73316=CARTESIAN_POINT ( 'NONE',  ( -5.056330833731841778, 15.00000000000000000, 13.58983143750696421 ) ) ;
#73323=EDGE_LOOP ( 'NONE', ( #25812, #70032, #73866, #20708, #15269, #93664 ) ) ;
#73325=DIRECTION ( 'NONE',  ( -0.4924235601034586685, 0.000000000000000000, -0.8703556959399044723 ) ) ;
#73334=DIRECTION ( 'NONE',  ( -0.9170600743851266001, 0.000000000000000000, 0.3987490689252404241 ) ) ;
#73339=VECTOR ( 'NONE', #16653, 1000.000000000000000 ) ;
#73342=DIRECTION ( 'NONE',  ( 0.000000000000000000, 1.000000000000000000, 0.000000000000000000 ) ) ;
#73348=EDGE_CURVE ( 'NONE', #80329, #94129, #40322, .T. ) ;
#73357=CARTESIAN_POINT ( 'NONE',  ( 12.07856007377819907, 15.00000000000000000, 8.022367888854917695 ) ) ;
#73366=CARTESIAN_POINT ( 'NONE',  ( -12.15129255554601428, 15.00000000000000000, -10.40305174771256524 ) ) ;
#73373=CARTESIAN_POINT ( 'NONE',  ( 10.93781366033340063, 0.5000000000000004441, 10.26470809774072634 ) ) ;
#73375=CARTESIAN_POINT ( 'NONE',  ( 14.91886229468048519, 14.76984964723650151, 0.8060919667645776165 ) ) ;
#73379=CARTESIAN_POINT ( 'NONE',  ( 0.000000000000000000, 15.00000000000000000, 0.000000000000000000 ) ) ;
#73381=CARTESIAN_POINT ( 'NONE',  ( -5.204170427930421283E-15, 6.671802177851543725, -11.25000000000000178 ) ) ;
#73384=EDGE_CURVE ( 'NONE', #73524, #51377, #28264, .T. ) ;
#73385=CARTESIAN_POINT ( 'NONE',  ( -5.204170427930422072E-15, 8.438309369127518167, -11.92686044187656513 ) ) ;
#73386=CARTESIAN_POINT ( 'NONE',  ( -13.82671409943291785, 0.000000000000000000, -3.447387012295409114 ) ) ;
#73387=VERTEX_POINT ( 'NONE', #12767 ) ;
#73388=CARTESIAN_POINT ( 'NONE',  ( 10.58223187591007886, 0.2306972965111904750, -10.54772123337530587 ) ) ;
#73393=CARTESIAN_POINT ( 'NONE',  ( 0.000000000000000000, 15.00000000000000000, 0.000000000000000000 ) ) ;
#73398=FACE_OUTER_BOUND ( 'NONE', #16499, .T. ) ;
#73414=AXIS2_PLACEMENT_3D ( 'NONE', #25639, #48116, #86623 ) ;
#73420=EDGE_CURVE ( 'NONE', #38633, #20656, #35766, .T. ) ;
#73421=AXIS2_PLACEMENT_3D ( 'NONE', #59889, #1761, #22906 ) ;
#73423=CARTESIAN_POINT ( 'NONE',  ( -5.056330833731550456, 15.00000000000000000, -13.58983143750704592 ) ) ;
#73433=DIRECTION ( 'NONE',  ( 0.000000000000000000, 1.000000000000000000, 0.000000000000000000 ) ) ;
#73436=B_SPLINE_CURVE_WITH_KNOTS ( 'NONE', 3,
 ( #88242, #50235, #80750, #12246, #73235, #35234 ),
 .UNSPECIFIED., .F., .F.,
 ( 4, 2, 4 ),
 ( 3.409110551495419861E-05, 0.0004400426677367805001, 0.0008459942299586068219 ),
 .UNSPECIFIED. ) ;
#73440=CARTESIAN_POINT ( 'NONE',  ( -5.204170427930421283E-15, -32.12636533006957507, -12.81628187352647608 ) ) ;
#73450=EDGE_LOOP ( 'NONE', ( #88069, #30029, #85568, #52921 ) ) ;
#73462=EDGE_CURVE ( 'NONE', #90286, #9752, #9277, .T. ) ;
#73464=DIRECTION ( 'NONE',  ( 0.000000000000000000, 0.000000000000000000, 1.000000000000000000 ) ) ;
#73472=UNCERTAINTY_MEASURE_WITH_UNIT (LENGTH_MEASURE( 1.000000000000000082E-05 ), #71293, 'distance_accuracy_value', 'NONE');
#73473=CARTESIAN_POINT ( 'NONE',  ( -2.962741594152892510, 0.000000000000000000, -13.93860331045676837 ) ) ;
#73476=CARTESIAN_POINT ( 'NONE',  ( -13.82671409943291785, 15.00000000000000000, -3.447387012295409114 ) ) ;
#73479=CARTESIAN_POINT ( 'NONE',  ( -5.148594389986405062, -3.608360355303317472E-16, 13.69051944078645100 ) ) ;
#73491=CARTESIAN_POINT ( 'NONE',  ( -14.16423886937409726, -27.98791783175269643, 3.795296366450320757 ) ) ;
#73495=VERTEX_POINT ( 'NONE', #50775 ) ;
#73501=CARTESIAN_POINT ( 'NONE',  ( -14.40939250470707478, 15.00000000000000000, -1.618458416369986219 ) ) ;
#73504=DIRECTION ( 'NONE',  ( -0.000000000000000000, -1.000000000000000000, -0.000000000000000000 ) ) ;
#73508=CARTESIAN_POINT ( 'NONE',  ( -5.440088680355547268, 8.897018677488176763, 9.422509992056143702 ) ) ;
#73511=ORIENTED_EDGE ( 'NONE', *, *, #60493, .F. ) ;
#73512=DIRECTION ( 'NONE',  ( 0.000000000000000000, 1.000000000000000000, 0.000000000000000000 ) ) ;
#73516=VECTOR ( 'NONE', #61190, 1000.000000000000000 ) ;
#73524=VERTEX_POINT ( 'NONE', #78216 ) ;
#73530=PLANE ( 'NONE',  #56376 ) ;
#73536=CARTESIAN_POINT ( 'NONE',  ( 13.34948392230377578, 0.04922511925147182721, -6.279918722514977958 ) ) ;
#73538=EDGE_CURVE ( 'NONE', #65046, #89050, #42745, .T. ) ;
#73540=CIRCLE ( 'NONE', #81536, 15.00000000000000000 ) ;
#73542=VERTEX_POINT ( 'NONE', #21916 ) ;
#73546=CARTESIAN_POINT ( 'NONE',  ( -4.873787042390880231, 15.00000000000000000, 13.39061984619915791 ) ) ;
#73547=DIRECTION ( 'NONE',  ( 0.000000000000000000, 1.000000000000000000, 0.000000000000000000 ) ) ;
#73550=CARTESIAN_POINT ( 'NONE',  ( 11.96291822454879750, 15.00000000000000000, -8.193813980849057543 ) ) ;
#73552=AXIS2_PLACEMENT_3D ( 'NONE', #73393, #94918, #87420 ) ;
#73555=LINE ( 'NONE', #4595, #83386 ) ;
#73556=CARTESIAN_POINT ( 'NONE',  ( 3.469446951953614189E-15, 7.258931151000791004, 9.846743663894594434 ) ) ;
#73560=ORIENTED_EDGE ( 'NONE', *, *, #16669, .T. ) ;
#73565=CARTESIAN_POINT ( 'NONE',  ( -0.3093388210927633941, 0.5000000000000004441, -14.99680997725065978 ) ) ;
#73572=EDGE_LOOP ( 'NONE', ( #29925, #31129, #42704, #18697 ) ) ;
#73578=AXIS2_PLACEMENT_3D ( 'NONE', #3563, #41568, #64519 ) ;
#73582=ORIENTED_EDGE ( 'NONE', *, *, #2694, .T. ) ;
#73588=CARTESIAN_POINT ( 'NONE',  ( 8.606322355891263598, 15.00000000000000000, 11.66967075398811282 ) ) ;
#73590=ORIENTED_EDGE ( 'NONE', *, *, #49771, .F. ) ;
#73608=EDGE_CURVE ( 'NONE', #25822, #70902, #88662, .T. ) ;
#73616=DIRECTION ( 'NONE',  ( 0.000000000000000000, 1.000000000000000000, 0.000000000000000000 ) ) ;
#73617=EDGE_CURVE ( 'NONE', #92561, #65076, #96183, .T. ) ;
#73620=CARTESIAN_POINT ( 'NONE',  ( 9.065164099344539039, 0.3640475087720985714, -11.95084933600768018 ) ) ;
#73623=CARTESIAN_POINT ( 'NONE',  ( -10.88017736071109987, -26.72798132251183034, 2.915334737309934532 ) ) ;
#73627=CARTESIAN_POINT ( 'NONE',  ( 9.159723438033129383, 0.000000000000000000, 10.91613331444548507 ) ) ;
#73628=CARTESIAN_POINT ( 'NONE',  ( -10.04755927614737843, 15.00000000000000533, -10.62803196998870803 ) ) ;
#73648=DIRECTION ( 'NONE',  ( 0.9999619230641714207, 0.000000000000000000, -0.008726535498360278933 ) ) ;
#73651=EDGE_CURVE ( 'NONE', #40543, #74503, #42199, .T. ) ;
#73652=ORIENTED_EDGE ( 'NONE', *, *, #85438, .F. ) ;
#73655=ORIENTED_EDGE ( 'NONE', *, *, #17045, .F. ) ;
#73656=ORIENTED_EDGE ( 'NONE', *, *, #79762, .F. ) ;
#73680=CARTESIAN_POINT ( 'NONE',  ( -2.602060718268879747, 0.000000000000000000, 4.792399674598840420 ) ) ;
#73683=CARTESIAN_POINT ( 'NONE',  ( -12.81628187352647608, 4.123634669930424934, 3.903127820947815962E-15 ) ) ;
#73690=ORIENTED_EDGE ( 'NONE', *, *, #41252, .T. ) ;
#73699=EDGE_CURVE ( 'NONE', #71199, #24915, #2217, .T. ) ;
#73700=CARTESIAN_POINT ( 'NONE',  ( 9.722841580490404922, -0.03417435944610275333, 12.70211588817942960 ) ) ;
#73702=CARTESIAN_POINT ( 'NONE',  ( -3.420591144908684988, 14.49999999999999112, 14.60477854057959313 ) ) ;
#73703=DIRECTION ( 'NONE',  ( -0.000000000000000000, -1.000000000000000000, -0.000000000000000000 ) ) ;
#73704=CARTESIAN_POINT ( 'NONE',  ( -9.402796353260967521, 0.5000000000000004441, -11.68706210897770248 ) ) ;
#73706=DIRECTION ( 'NONE',  ( -0.000000000000000000, 1.000000000000000000, -0.000000000000000000 ) ) ;
#73708=EDGE_CURVE ( 'NONE', #63731, #15285, #65406, .T. ) ;
#73710=CARTESIAN_POINT ( 'NONE',  ( 3.420591144908548653, 0.3640475087720985714, -14.60477854057957003 ) ) ;
#73716=B_SPLINE_CURVE_WITH_KNOTS ( 'NONE', 3,
 ( #65830, #81335, #59317, #89816, #36831, #72836 ),
 .UNSPECIFIED., .F., .F.,
 ( 4, 2, 4 ),
 ( 0.0002800421826021987559, 0.0006862478247342195751, 0.001092453466866240286 ),
 .UNSPECIFIED. ) ;
#73718=CARTESIAN_POINT ( 'NONE',  ( 2.930023131210739873, 0.000000000000000000, 4.599215049682178424 ) ) ;
#73722=FACE_OUTER_BOUND ( 'NONE', #32385, .T. ) ;
#73731=ORIENTED_EDGE ( 'NONE', *, *, #87477, .T. ) ;
#73732=CARTESIAN_POINT ( 'NONE',  ( -3.014428414850123250, 6.159700295649318313, 11.25000000000000178 ) ) ;
#73743=CARTESIAN_POINT ( 'NONE',  ( 3.795296366450306547, 10.34541550158063394, -14.16423886937410259 ) ) ;
#73750=CIRCLE ( 'NONE', #13088, 14.49999999999999822 ) ;
#73752=ORIENTED_EDGE ( 'NONE', *, *, #44824, .T. ) ;
#73779=ORIENTED_EDGE ( 'NONE', *, *, #86306, .F. ) ;
#73781=PLANE ( 'NONE',  #84350 ) ;
#73786=CARTESIAN_POINT ( 'NONE',  ( 6.715867195167361636, 4.143177415744058416E-16, 12.85095824508331930 ) ) ;
#73794=VERTEX_POINT ( 'NONE', #7149 ) ;
#73797=ORIENTED_EDGE ( 'NONE', *, *, #41162, .T. ) ;
#73812=VERTEX_POINT ( 'NONE', #28163 ) ;
#73815=EDGE_CURVE ( 'NONE', #61124, #49583, #29625, .T. ) ;
#73817=CARTESIAN_POINT ( 'NONE',  ( 0.000000000000000000, 14.49999999999999822, 0.000000000000000000 ) ) ;
#73822=ORIENTED_EDGE ( 'NONE', *, *, #77005, .T. ) ;
#73824=CARTESIAN_POINT ( 'NONE',  ( -7.882504294824035362, 1.541599964002826617E-16, 12.32089577884786458 ) ) ;
#73829=CIRCLE ( 'NONE', #5199, 15.00000000000000000 ) ;
#73835=VECTOR ( 'NONE', #37877, 1000.000000000000000 ) ;
#73841=DIRECTION ( 'NONE',  ( -0.9762960071199316969, 0.000000000000000000, -0.2164396139381103701 ) ) ;
#73842=DIRECTION ( 'NONE',  ( -0.000000000000000000, -1.000000000000000000, -0.000000000000000000 ) ) ;
#73844=LINE ( 'NONE', #97361, #47363 ) ;
#73847=VECTOR ( 'NONE', #75739, 1000.000000000000000 ) ;
#73848=CARTESIAN_POINT ( 'NONE',  ( 7.264948169187374738, 14.76930270348881180, 13.05597881399723903 ) ) ;
#73851=CARTESIAN_POINT ( 'NONE',  ( -5.093587308868599450, 15.00000000000000000, 15.16353404595993837 ) ) ;
#73854=VERTEX_POINT ( 'NONE', #5181 ) ;
#73855=CARTESIAN_POINT ( 'NONE',  ( -12.60874940350953111, 3.965829894984375834E-16, 7.160268045226943379 ) ) ;
#73858=EDGE_CURVE ( 'NONE', #48625, #87096, #14665, .T. ) ;
#73866=ORIENTED_EDGE ( 'NONE', *, *, #19545, .T. ) ;
#73873=CARTESIAN_POINT ( 'NONE',  ( 14.48718990079892066, 15.00000000000000000, 0.6093675230841449908 ) ) ;
#73878=DIRECTION ( 'NONE',  ( -0.6087614290087242086, 0.000000000000000000, 0.7933533402912323895 ) ) ;
#73884=ORIENTED_EDGE ( 'NONE', *, *, #30154, .F. ) ;
#73886=CARTESIAN_POINT ( 'NONE',  ( 14.09394518620610270, 4.258544466044566969E-16, 3.407449058785454898 ) ) ;
#73896=CARTESIAN_POINT ( 'NONE',  ( 3.836325488036183451, 15.00000000000000000, -14.50112432709422627 ) ) ;
#73897=CARTESIAN_POINT ( 'NONE',  ( -2.174473938468922896, 0.000000000000000000, -5.000947681547216916 ) ) ;
#73902=FACE_OUTER_BOUND ( 'NONE', #66547, .T. ) ;
#73906=CIRCLE ( 'NONE', #30789, 15.00000000000000000 ) ;
#73909=ORIENTED_EDGE ( 'NONE', *, *, #50981, .F. ) ;
#73934=CARTESIAN_POINT ( 'NONE',  ( 0.000000000000000000, 0.5000000000000004441, 0.000000000000000000 ) ) ;
#73938=VECTOR ( 'NONE', #33232, 1000.000000000000114 ) ;
#73940=CARTESIAN_POINT ( 'NONE',  ( -5.204170427930421283E-15, -12.12636533006957507, -12.81628187352647608 ) ) ;
#73949=FACE_OUTER_BOUND ( 'NONE', #34934, .T. ) ;
#73953=EDGE_CURVE ( 'NONE', #41669, #18731, #16196, .T. ) ;
#73956=ORIENTED_EDGE ( 'NONE', *, *, #82899, .T. ) ;
#73964=CARTESIAN_POINT ( 'NONE',  ( -1.780824192092605562, 15.00000000000000000, 14.89391369643512064 ) ) ;
#73967=ORIENTED_EDGE ( 'NONE', *, *, #51700, .T. ) ;
#73968=CARTESIAN_POINT ( 'NONE',  ( 13.82671409943296226, 15.00000000000000000, -3.447387012295225261 ) ) ;
#73971=CARTESIAN_POINT ( 'NONE',  ( 0.000000000000000000, 0.000000000000000000, -13.74999999999999467 ) ) ;
#73975=TOROIDAL_SURFACE ( 'NONE', #21321, 14.49999999999999822, 0.5000000000000000000 ) ;
#73978=CARTESIAN_POINT ( 'NONE',  ( 12.00809552683958614, 15.00000000000000000, -8.989195838243546177 ) ) ;
#73990=B_SPLINE_CURVE_WITH_KNOTS ( 'NONE', 3,
 ( #49738, #41293, #3277, #9795, #94760, #33741 ),
 .UNSPECIFIED., .F., .F.,
 ( 4, 2, 4 ),
 ( 3.409110551496095454E-05, 0.0004400426677367853790, 0.0008459942299586097492 ),
 .UNSPECIFIED. ) ;
#73991=CARTESIAN_POINT ( 'NONE',  ( 3.795296366450314540, -26.73791783175269643, 14.16423886937410082 ) ) ;
#73997=CARTESIAN_POINT ( 'NONE',  ( 10.91036564011094256, 14.76984962000323875, 10.20716212663568889 ) ) ;
#74001=CARTESIAN_POINT ( 'NONE',  ( 14.56368227077856758, 14.76930270348881180, 3.337246381125283712 ) ) ;
#74006=CARTESIAN_POINT ( 'NONE',  ( -9.422509992056145478, 32.64701867748817676, -5.440088680355541939 ) ) ;
#74008=LINE ( 'NONE', #74502, #15265 ) ;
#74009=EDGE_LOOP ( 'NONE', ( #55395, #69791, #85755, #83576, #95586, #10966 ) ) ;
#74018=CARTESIAN_POINT ( 'NONE',  ( -3.420591144908350589, 0.5000000000000004441, -14.60477854057960556 ) ) ;
#74034=EDGE_CURVE ( 'NONE', #60281, #1705, #22153, .T. ) ;
#74036=ORIENTED_EDGE ( 'NONE', *, *, #1141, .T. ) ;
#74040=CARTESIAN_POINT ( 'NONE',  ( 4.431036607602587551, 14.63606876205557050, -14.33059365769914528 ) ) ;
#74049=CARTESIAN_POINT ( 'NONE',  ( -8.527530157486182816, 15.59226448433412315, -4.923371831947288335 ) ) ;
#74050=ORIENTED_EDGE ( 'NONE', *, *, #73538, .T. ) ;
#74051=VERTEX_POINT ( 'NONE', #13655 ) ;
#74061=EDGE_CURVE ( 'NONE', #54254, #12471, #6984, .T. ) ;
#74063=VERTEX_POINT ( 'NONE', #82644 ) ;
#74066=ORIENTED_EDGE ( 'NONE', *, *, #45729, .F. ) ;
#74072=CARTESIAN_POINT ( 'NONE',  ( -11.39601241150444189, 15.00000000000000000, -11.22534175661882294 ) ) ;
#74074=CARTESIAN_POINT ( 'NONE',  ( 1.114591949025029338, 4.390405144365474573E-16, -14.45709807627964416 ) ) ;
#74077=ORIENTED_EDGE ( 'NONE', *, *, #56250, .F. ) ;
#74079=CARTESIAN_POINT ( 'NONE',  ( 14.47650479471827722, 14.49999999999999112, -3.928206833722049929 ) ) ;
#74081=ORIENTED_EDGE ( 'NONE', *, *, #21978, .T. ) ;
#74083=CARTESIAN_POINT ( 'NONE',  ( 14.04391541078763161, 4.402316570082688340E-16, 3.608107528142934228 ) ) ;
#74085=CARTESIAN_POINT ( 'NONE',  ( 14.26139399674454822, 15.00000000000000000, -2.619664342929791445 ) ) ;
#74098=VECTOR ( 'NONE', #84445, 1000.000000000000000 ) ;
#74107=CIRCLE ( 'NONE', #70930, 14.49999999999999822 ) ;
#74111=CARTESIAN_POINT ( 'NONE',  ( -10.88017736071109987, -21.72798132251182679, 2.915334737309934532 ) ) ;
#74123=CARTESIAN_POINT ( 'NONE',  ( -10.14667048435152097, 15.00000000000000000, 10.35833375027034542 ) ) ;
#74126=ORIENTED_EDGE ( 'NONE', *, *, #49280, .T. ) ;
#74137=DIRECTION ( 'NONE',  ( -0.000000000000000000, 1.000000000000000000, 0.000000000000000000 ) ) ;
#74139=AXIS2_PLACEMENT_3D ( 'NONE', #32223, #62724, #62232 ) ;
#74140=ADVANCED_FACE ( 'NONE', ( #24625 ), #29175, .T. ) ;
#74141=ORIENTED_EDGE ( 'NONE', *, *, #41586, .T. ) ;
#74146=LINE ( 'NONE', #36164, #19798 ) ;
#74158=DIRECTION ( 'NONE',  ( 0.4305110968082926370, 0.000000000000000000, 0.9025852843498617384 ) ) ;
#74161=CARTESIAN_POINT ( 'NONE',  ( -7.208316651077764980, -39.61606884899921255, -7.208316651077759651 ) ) ;
#74162=VERTEX_POINT ( 'NONE', #8139 ) ;
#74163=DIRECTION ( 'NONE',  ( 0.000000000000000000, -1.000000000000000000, 0.000000000000000000 ) ) ;
#74164=ORIENTED_EDGE ( 'NONE', *, *, #21699, .T. ) ;
#74165=ORIENTED_EDGE ( 'NONE', *, *, #90075, .T. ) ;
#74173=CIRCLE ( 'NONE', #39087, 14.49999999999999822 ) ;
#74174=CARTESIAN_POINT ( 'NONE',  ( 12.81628187352647608, 11.41530133659708568, 3.434112377981052511 ) ) ;
#74178=ADVANCED_FACE ( 'NONE', ( #91129 ), #23149, .F. ) ;
#74189=ORIENTED_EDGE ( 'NONE', *, *, #22531, .T. ) ;
#74191=CARTESIAN_POINT ( 'NONE',  ( -6.767445849361333643, 0.5000000000000004441, 13.38662304974491946 ) ) ;
#74194=DIRECTION ( 'NONE',  ( -0.000000000000000000, -1.000000000000000000, -0.000000000000000000 ) ) ;
#74198=VERTEX_POINT ( 'NONE', #84141 ) ;
#74204=B_SPLINE_CURVE_WITH_KNOTS ( 'NONE', 3,
 ( #55326, #39356, #47817, #46354, #69850, #92343 ),
 .UNSPECIFIED., .F., .F.,
 ( 4, 2, 4 ),
 ( 3.409110551494476605E-05, 0.0004400426677367897700, 0.0008459942299586347943 ),
 .UNSPECIFIED. ) ;
#74206=DIRECTION ( 'NONE',  ( 0.000000000000000000, 1.000000000000000000, 0.000000000000000000 ) ) ;
#74212=EDGE_CURVE ( 'NONE', #59079, #42731, #10510, .T. ) ;
#74217=CARTESIAN_POINT ( 'NONE',  ( -2.815433093577211832, 14.49999999999999112, 14.73340885523754551 ) ) ;
#74227=CARTESIAN_POINT ( 'NONE',  ( 7.082119434687047743, 10.13708216824730357, -12.26659068614894821 ) ) ;
#74229=B_SPLINE_CURVE_WITH_KNOTS ( 'NONE', 3,
 ( #65896, #90868, #29869, #83380, #36401, #88907 ),
 .UNSPECIFIED., .F., .F.,
 ( 4, 2, 4 ),
 ( 0.0002800001862105966138, 0.0006862054174524880035, 0.001092410648694379285 ),
 .UNSPECIFIED. ) ;
#74236=VERTEX_POINT ( 'NONE', #76619 ) ;
#74241=CARTESIAN_POINT ( 'NONE',  ( -10.93781366033354274, 14.49999999999999822, 10.26470809774057891 ) ) ;
#74244=CARTESIAN_POINT ( 'NONE',  ( 2.815433093577023538, 0.3640475087720981828, 14.73340885523752419 ) ) ;
#74247=ORIENTED_EDGE ( 'NONE', *, *, #7382, .T. ) ;
#74250=FACE_OUTER_BOUND ( 'NONE', #7174, .T. ) ;
#74265=VERTEX_POINT ( 'NONE', #4083 ) ;
#74267=CIRCLE ( 'NONE', #72695, 14.49999999999999822 ) ;
#74280=ORIENTED_EDGE ( 'NONE', *, *, #26636, .T. ) ;
#74284=ORIENTED_EDGE ( 'NONE', *, *, #34089, .F. ) ;
#74289=ORIENTED_EDGE ( 'NONE', *, *, #24390, .T. ) ;
#74293=AXIS2_PLACEMENT_3D ( 'NONE', #80663, #96165, #50655 ) ;
#74313=CARTESIAN_POINT ( 'NONE',  ( -8.157990163924880633, 0.2306972965111904472, 12.51739793958107860 ) ) ;
#74314=VECTOR ( 'NONE', #61963, 1000.000000000000000 ) ;
#74328=EDGE_CURVE ( 'NONE', #22776, #54527, #97864, .T. ) ;
#74330=ORIENTED_EDGE ( 'NONE', *, *, #29234, .F. ) ;
#74331=FACE_OUTER_BOUND ( 'NONE', #72181, .T. ) ;
#74335=DIRECTION ( 'NONE',  ( 0.9762960071199331402, 0.000000000000000000, 0.2164396139381037087 ) ) ;
#74338=DIRECTION ( 'NONE',  ( 0.000000000000000000, 1.000000000000000000, 0.000000000000000000 ) ) ;
#74344=DIRECTION ( 'NONE',  ( 0.000000000000000000, 1.000000000000000000, 0.000000000000000000 ) ) ;
#74347=ORIENTED_EDGE ( 'NONE', *, *, #34165, .T. ) ;
#74351=DIRECTION ( 'NONE',  ( -0.000000000000000000, -1.000000000000000000, -0.000000000000000000 ) ) ;
#74358=ORIENTED_EDGE ( 'NONE', *, *, #11611, .F. ) ;
#74360=DIRECTION ( 'NONE',  ( -0.000000000000000000, 1.000000000000000000, 0.000000000000000000 ) ) ;
#74361=DIRECTION ( 'NONE',  ( 0.000000000000000000, 1.000000000000000000, 0.000000000000000000 ) ) ;
#74374=DIRECTION ( 'NONE',  ( 0.000000000000000000, 0.000000000000000000, -1.000000000000000000 ) ) ;
#74379=CARTESIAN_POINT ( 'NONE',  ( 4.084234479374286408, 0.000000000000000000, 3.613425430272956262 ) ) ;
#74382=EDGE_CURVE ( 'NONE', #25445, #13755, #80066, .T. ) ;
#74389=AXIS2_PLACEMENT_3D ( 'NONE', #52305, #83794, #6808 ) ;
#74390=EDGE_CURVE ( 'NONE', #32615, #97699, #89132, .T. ) ;
#74394=ORIENTED_EDGE ( 'NONE', *, *, #28363, .F. ) ;
#74408=VERTEX_POINT ( 'NONE', #11084 ) ;
#74417=CARTESIAN_POINT ( 'NONE',  ( 8.549759589250173875, 14.76984986101048847, 12.25250350990703652 ) ) ;
#74424=CARTESIAN_POINT ( 'NONE',  ( -9.382169495545413795, -15.25136533006957684, 9.382169495545428006 ) ) ;
#74434=ADVANCED_FACE ( 'NONE', ( #42563 ), #38544, .T. ) ;
#74435=CARTESIAN_POINT ( 'NONE',  ( -14.71525861348292175, 14.49999999999999822, 2.908807992686482713 ) ) ;
#74450=LINE ( 'NONE', #5978, #15205 ) ;
#74459=AXIS2_PLACEMENT_3D ( 'NONE', #62637, #85162, #77156 ) ;
#74461=PRODUCT_DEFINITION_CONTEXT ( 'detailed design', #72970, 'design' ) ;
#74471=CARTESIAN_POINT ( 'NONE',  ( 14.40939250469964961, 3.793246902777681429E-16, 1.618458416365853747 ) ) ;
#74478=EDGE_CURVE ( 'NONE', #91030, #23318, #75523, .T. ) ;
#74479=DIRECTION ( 'NONE',  ( 0.000000000000000000, 0.000000000000000000, 1.000000000000000000 ) ) ;
#74481=AXIS2_PLACEMENT_3D ( 'NONE', #16697, #86667, #1707 ) ;
#74483=CARTESIAN_POINT ( 'NONE',  ( -14.16423886937410082, -18.19625116508602858, 4.336808689942017736E-15 ) ) ;
#74489=CARTESIAN_POINT ( 'NONE',  ( -2.930023131210709231, 0.000000000000000000, -4.599215049682199741 ) ) ;
#74491=DIRECTION ( 'NONE',  ( 0.000000000000000000, 0.000000000000000000, 1.000000000000000000 ) ) ;
#74494=DIRECTION ( 'NONE',  ( 0.000000000000000000, 1.000000000000000000, 0.000000000000000000 ) ) ;
#74496=DIRECTION ( 'NONE',  ( -0.000000000000000000, -1.000000000000000000, -0.000000000000000000 ) ) ;
#74498=CARTESIAN_POINT ( 'NONE',  ( -10.88017736071110342, 28.06368534415484817, 3.903127820947815962E-15 ) ) ;
#74502=CARTESIAN_POINT ( 'NONE',  ( 14.88232117145531141, 15.00000000000000000, -1.875237731503139438 ) ) ;
#74503=VERTEX_POINT ( 'NONE', #58043 ) ;
#74504=CIRCLE ( 'NONE', #72976, 15.00000000000000000 ) ;
#74509=EDGE_CURVE ( 'NONE', #81942, #1776, #66040, .T. ) ;
#74516=PLANE ( 'NONE',  #52792 ) ;
#74518=ORIENTED_EDGE ( 'NONE', *, *, #10862, .F. ) ;
#74522=CARTESIAN_POINT ( 'NONE',  ( 13.14228782657341732, 14.49999999999999112, 7.230509711182337540 ) ) ;
#74524=DIRECTION ( 'NONE',  ( -0.9890158633619157147, 0.000000000000000000, -0.1478094111296180124 ) ) ;
#74531=CARTESIAN_POINT ( 'NONE',  ( 14.02068044289379500, 0.3640475087720986824, -5.331089937175662818 ) ) ;
#74532=VECTOR ( 'NONE', #48236, 1000.000000000000000 ) ;
#74533=ORIENTED_EDGE ( 'NONE', *, *, #56826, .T. ) ;
#74538=CARTESIAN_POINT ( 'NONE',  ( 4.431036607602602651, 14.49999999999999112, -14.33059365769916305 ) ) ;
#74539=CARTESIAN_POINT ( 'NONE',  ( 7.595945211628331251, 3.826527677142797770E-16, -12.35117874301642082 ) ) ;
#74544=VECTOR ( 'NONE', #34727, 1000.000000000000000 ) ;
#74546=DIRECTION ( 'NONE',  ( -0.000000000000000000, -1.000000000000000000, -0.000000000000000000 ) ) ;
#74548=EDGE_CURVE ( 'NONE', #49599, #20937, #93918, .T. ) ;
#74549=FACE_OUTER_BOUND ( 'NONE', #19585, .T. ) ;
#74550=CARTESIAN_POINT ( 'NONE',  ( -4.923371831947302546, 15.17559781766746063, -8.527530157486173934 ) ) ;
#74551=EDGE_LOOP ( 'NONE', ( #52444, #20073, #88071, #81168 ) ) ;
#74553=CARTESIAN_POINT ( 'NONE',  ( -6.742022620658060461, 14.95037102811560459, -13.12259272460513770 ) ) ;
#74554=ORIENTED_EDGE ( 'NONE', *, *, #50943, .F. ) ;
#74562=AXIS2_PLACEMENT_3D ( 'NONE', #91570, #24066, #77050 ) ;
#74563=VECTOR ( 'NONE', #73648, 1000.000000000000000 ) ;
#74564=TOROIDAL_SURFACE ( 'NONE', #33018, 14.49999999999999822, 0.5000000000000000000 ) ;
#74569=ORIENTED_EDGE ( 'NONE', *, *, #40068, .T. ) ;
#74579=B_SPLINE_CURVE_WITH_KNOTS ( 'NONE', 3,
 ( #26018, #48506, #87003, #41028, #34476, #85536 ),
 .UNSPECIFIED., .F., .F.,
 ( 4, 2, 4 ),
 ( 0.0002800003243993126178, 0.0006862055569927218634, 0.001092410789586131109 ),
 .UNSPECIFIED. ) ;
#74583=DIRECTION ( 'NONE',  ( 0.000000000000000000, 1.000000000000000000, 0.000000000000000000 ) ) ;
#74587=CARTESIAN_POINT ( 'NONE',  ( -11.39900937121540814, 12.73119725676927771, -1.484196799168450376 ) ) ;
#74592=CARTESIAN_POINT ( 'NONE',  ( 0.000000000000000000, 0.5000000000000004441, 0.000000000000000000 ) ) ;
#74596=DIRECTION ( 'NONE',  ( 0.7489557207890082946, 0.000000000000000000, -0.6626200482157305061 ) ) ;
#74605=VERTEX_POINT ( 'NONE', #95622 ) ;
#74612=DIRECTION ( 'NONE',  ( -0.8949343616020323244, -0.000000000000000000, 0.4461978131097944500 ) ) ;
#74613=CARTESIAN_POINT ( 'NONE',  ( 13.34343830728402125, 14.63606867471890816, 6.852200678592722305 ) ) ;
#74618=CARTESIAN_POINT ( 'NONE',  ( 2.915334737309928315, -5.477981322511826789, 10.88017736071109987 ) ) ;
#74622=CARTESIAN_POINT ( 'NONE',  ( -8.134956207566176545, -0.03417435944610275333, 13.77315809598633756 ) ) ;
#74624=CARTESIAN_POINT ( 'NONE',  ( 14.19749592853504438, 15.00000000000000000, -7.369430493279943484 ) ) ;
#74628=ADVANCED_FACE ( 'NONE', ( #72121 ), #49793, .T. ) ;
#74630=B_SPLINE_CURVE_WITH_KNOTS ( 'NONE', 3,
 ( #63162, #86181, #39706, #93670, #48163, #24208 ),
 .UNSPECIFIED., .F., .F.,
 ( 4, 2, 4 ),
 ( 3.409110551494477282E-05, 0.0004400426677367911795, 0.0008459942299586376132 ),
 .UNSPECIFIED. ) ;
#74637=FACE_OUTER_BOUND ( 'NONE', #35343, .T. ) ;
#74647=VERTEX_POINT ( 'NONE', #21608 ) ;
#74650=VERTEX_POINT ( 'NONE', #6104 ) ;
#74652=LINE ( 'NONE', #98172, #82101 ) ;
#74668=AXIS2_PLACEMENT_3D ( 'NONE', #26265, #241, #59714 ) ;
#74670=CARTESIAN_POINT ( 'NONE',  ( -8.527530157486182816, -19.40773551566587685, -4.923371831947288335 ) ) ;
#74671=ORIENTED_EDGE ( 'NONE', *, *, #7250, .T. ) ;
#74674=VERTEX_POINT ( 'NONE', #74085 ) ;
#74680=EDGE_CURVE ( 'NONE', #18387, #31163, #65101, .T. ) ;
#74681=LINE ( 'NONE', #73680, #83138 ) ;
#74684=CARTESIAN_POINT ( 'NONE',  ( 6.408140936763236262, 27.45696800326376419, -11.09922568453595026 ) ) ;
#74687=B_SPLINE_CURVE_WITH_KNOTS ( 'NONE', 3,
 ( #42266, #95758, #50750, #87746, #42753, #13231 ),
 .UNSPECIFIED., .F., .F.,
 ( 4, 2, 4 ),
 ( 3.409110551494648044E-05, 0.0004400426677367923179, 0.0008459942299586381553 ),
 .UNSPECIFIED. ) ;
#74691=AXIS2_PLACEMENT_3D ( 'NONE', #84642, #92143, #23668 ) ;
#74695=CARTESIAN_POINT ( 'NONE',  ( 13.34343830728399283, 0.5000000000000004441, 6.852200678592689442 ) ) ;
#74696=CARTESIAN_POINT ( 'NONE',  ( 0.000000000000000000, 15.00000000000000000, 0.000000000000000000 ) ) ;
#74699=VECTOR ( 'NONE', #42523, 1000.000000000000114 ) ;
#74702=FACE_OUTER_BOUND ( 'NONE', #3114, .T. ) ;
#74707=DIRECTION ( 'NONE',  ( 0.000000000000000000, 0.000000000000000000, 1.000000000000000000 ) ) ;
#74712=CARTESIAN_POINT ( 'NONE',  ( -14.29541133317247414, 0.2306972965111896978, 4.345028136609434988 ) ) ;
#74724=CARTESIAN_POINT ( 'NONE',  ( -9.724225243420933751, 2.502569995908613620, -5.657147814151106680 ) ) ;
#74736=CARTESIAN_POINT ( 'NONE',  ( -14.16423886937410082, 16.80374883491397853, 4.336808689942017736E-15 ) ) ;
#74743=AXIS2_PLACEMENT_3D ( 'NONE', #82414, #13938, #59907 ) ;
#74747=ADVANCED_FACE ( 'NONE', ( #89596 ), #62564, .T. ) ;
#74753=CARTESIAN_POINT ( 'NONE',  ( 2.913501739333662854, 4.325554204331052541E-16, 14.20427779279537184 ) ) ;
#74756=EDGE_CURVE ( 'NONE', #73854, #37098, #97723, .T. ) ;
#74757=ORIENTED_EDGE ( 'NONE', *, *, #47359, .T. ) ;
#74772=VECTOR ( 'NONE', #22779, 1000.000000000000114 ) ;
#74776=CARTESIAN_POINT ( 'NONE',  ( 9.742785792574936821, 5.005135511184879427, 5.624999999999997335 ) ) ;
#74782=DIRECTION ( 'NONE',  ( 0.000000000000000000, 1.000000000000000000, 0.000000000000000000 ) ) ;
#74790=ORIENTED_EDGE ( 'NONE', *, *, #67432, .F. ) ;
#74794=VERTEX_POINT ( 'NONE', #68089 ) ;
#74814=ORIENTED_EDGE ( 'NONE', *, *, #50608, .T. ) ;
#74836=CIRCLE ( 'NONE', #38182, 15.00000000000000000 ) ;
#74844=EDGE_CURVE ( 'NONE', #24915, #37516, #40251, .T. ) ;
#74864=ORIENTED_EDGE ( 'NONE', *, *, #81198, .F. ) ;
#74868=CARTESIAN_POINT ( 'NONE',  ( 3.469446951953614189E-15, 9.171802177851546389, 11.25000000000000355 ) ) ;
#74873=EDGE_CURVE ( 'NONE', #23769, #1162, #25835, .T. ) ;
#74882=DIRECTION ( 'NONE',  ( -0.000000000000000000, -1.000000000000000000, -0.000000000000000000 ) ) ;
#74901=B_SPLINE_CURVE_WITH_KNOTS ( 'NONE', 3,
 ( #13994, #43967, #59962, #44469, #82970, #74471 ),
 .UNSPECIFIED., .F., .F.,
 ( 4, 2, 4 ),
 ( 3.409110551495225382E-05, 0.0004400426677367789280, 0.0008459942299586055208 ),
 .UNSPECIFIED. ) ;
#74913=CIRCLE ( 'NONE', #19034, 15.00000000000000000 ) ;
#74922=DIRECTION ( 'NONE',  ( 0.000000000000000000, 1.000000000000000000, 0.000000000000000000 ) ) ;
#74925=CARTESIAN_POINT ( 'NONE',  ( 0.000000000000000000, 0.5000000000000004441, 0.000000000000000000 ) ) ;
#74927=ORIENTED_EDGE ( 'NONE', *, *, #28407, .T. ) ;
#74929=CARTESIAN_POINT ( 'NONE',  ( -5.204170427930421283E-15, -22.12636533006957507, -12.81628187352647608 ) ) ;
#74937=AXIS2_PLACEMENT_3D ( 'NONE', #94849, #72826, #4364 ) ;
#74939=EDGE_LOOP ( 'NONE', ( #69483, #47357, #54413, #60558, #15429, #17188 ) ) ;
#74945=VECTOR ( 'NONE', #20381, 1000.000000000000000 ) ;
#74957=EDGE_CURVE ( 'NONE', #95213, #25245, #19471, .T. ) ;
#74959=DIRECTION ( 'NONE',  ( -0.000000000000000000, -1.000000000000000000, -0.000000000000000000 ) ) ;
#74964=CARTESIAN_POINT ( 'NONE',  ( -14.64921366071501119, 0.04962891916449908153, 1.748670679918064241 ) ) ;
#74975=EDGE_CURVE ( 'NONE', #32046, #48910, #40049, .T. ) ;
#74982=CARTESIAN_POINT ( 'NONE',  ( -3.795296366450322534, -14.23791783175269110, -14.16423886937409904 ) ) ;
#74987=VERTEX_POINT ( 'NONE', #70549 ) ;
#74996=DIRECTION ( 'NONE',  ( 0.000000000000000000, 0.000000000000000000, 1.000000000000000000 ) ) ;
#74998=CARTESIAN_POINT ( 'NONE',  ( 2.915334737309921209, 31.60535201082150891, -10.88017736071110164 ) ) ;
#75006=CARTESIAN_POINT ( 'NONE',  ( -13.50249619331281892, 15.00000000000000711, 5.623250243473404630 ) ) ;
#75012=CARTESIAN_POINT ( 'NONE',  ( -5.204170427930421283E-15, 11.41212336850781739, -11.92686044187656513 ) ) ;
#75036=DIRECTION ( 'NONE',  ( -0.000000000000000000, -1.000000000000000000, -0.000000000000000000 ) ) ;
#75041=DIRECTION ( 'NONE',  ( -0.4924235601034707144, 0.000000000000000000, 0.8703556959398975890 ) ) ;
#75043=CARTESIAN_POINT ( 'NONE',  ( 2.638427012816835227, 17.46726448433411960, 9.846743663894590881 ) ) ;
#75047=ORIENTED_EDGE ( 'NONE', *, *, #65118, .T. ) ;
#75057=B_SPLINE_CURVE_WITH_KNOTS ( 'NONE', 3,
 ( #12396, #94911, #4910, #57887, #19899, #42902 ),
 .UNSPECIFIED., .F., .F.,
 ( 4, 2, 4 ),
 ( 3.409110551494634492E-05, 0.0004400426677367926974, 0.0008459942299586390227 ),
 .UNSPECIFIED. ) ;
#75066=TOROIDAL_SURFACE ( 'NONE', #91050, 14.49999999999999822, 0.5000000000000000000 ) ;
#75076=EDGE_CURVE ( 'NONE', #39153, #38225, #8568, .T. ) ;
#75079=DIRECTION ( 'NONE',  ( -0.000000000000000000, -1.000000000000000000, -0.000000000000000000 ) ) ;
#75080=EDGE_CURVE ( 'NONE', #84641, #56002, #85056, .T. ) ;
#75084=DIRECTION ( 'NONE',  ( 0.000000000000000000, 1.000000000000000000, 0.000000000000000000 ) ) ;
#75086=DIRECTION ( 'NONE',  ( 0.000000000000000000, 0.000000000000000000, 1.000000000000000000 ) ) ;
#75087=ORIENTED_EDGE ( 'NONE', *, *, #30245, .F. ) ;
#75093=FACE_OUTER_BOUND ( 'NONE', #89317, .T. ) ;
#75096=ORIENTED_EDGE ( 'NONE', *, *, #29158, .F. ) ;
#75106=ADVANCED_FACE ( 'NONE', ( #62533 ), #75343, .T. ) ;
#75107=CYLINDRICAL_SURFACE ( 'NONE', #93322, 15.00000000000000000 ) ;
#75108=CARTESIAN_POINT ( 'NONE',  ( 4.547378612396773434, 0.000000000000000000, -3.009844244835506721 ) ) ;
#75112=CARTESIAN_POINT ( 'NONE',  ( -10.88017736071110164, -7.144647989178493752, -2.915334737309917212 ) ) ;
#75114=LINE ( 'NONE', #14640, #97935 ) ;
#75116=LINE ( 'NONE', #67631, #54383 ) ;
#75117=PLANE ( 'NONE',  #72110 ) ;
#75128=ORIENTED_EDGE ( 'NONE', *, *, #31526, .F. ) ;
#75138=ORIENTED_EDGE ( 'NONE', *, *, #16959, .T. ) ;
#75142=VERTEX_POINT ( 'NONE', #32537 ) ;
#75158=CARTESIAN_POINT ( 'NONE',  ( 7.208316651077762316, -20.86606884899920544, -7.208316651077764980 ) ) ;
#75159=VERTEX_POINT ( 'NONE', #69074 ) ;
#75173=CARTESIAN_POINT ( 'NONE',  ( -6.408140936763232709, 19.95696800326377129, 11.09922568453595026 ) ) ;
#75174=ORIENTED_EDGE ( 'NONE', *, *, #88860, .F. ) ;
#75176=ORIENTED_EDGE ( 'NONE', *, *, #86726, .T. ) ;
#75178=ORIENTED_EDGE ( 'NONE', *, *, #34165, .F. ) ;
#75186=CARTESIAN_POINT ( 'NONE',  ( -3.866399090317375720, 14.95077488074853811, 14.23717170745768712 ) ) ;
#75187=AXIS2_PLACEMENT_3D ( 'NONE', #79559, #11059, #86080 ) ;
#75193=CARTESIAN_POINT ( 'NONE',  ( 0.000000000000000000, 14.49999999999999822, 0.000000000000000000 ) ) ;
#75201=CARTESIAN_POINT ( 'NONE',  ( 0.000000000000000000, 14.49999999999999822, 0.000000000000000000 ) ) ;
#75213=FACE_OUTER_BOUND ( 'NONE', #49554, .T. ) ;
#75216=CARTESIAN_POINT ( 'NONE',  ( 6.761389522993794365, 0.2306972965111908080, 13.32372569557304764 ) ) ;
#75222=CARTESIAN_POINT ( 'NONE',  ( 13.78891971893207291, 14.63606857305789966, 5.904717858191650848 ) ) ;
#75228=CARTESIAN_POINT ( 'NONE',  ( 14.16423886937410437, 19.09541550158063572, 3.795296366450304770 ) ) ;
#75232=AXIS2_PLACEMENT_3D ( 'NONE', #25331, #70331, #54809 ) ;
#75252=DIRECTION ( 'NONE',  ( 0.000000000000000000, 1.000000000000000000, 0.000000000000000000 ) ) ;
#75282=ORIENTED_EDGE ( 'NONE', *, *, #18314, .T. ) ;
#75291=EDGE_CURVE ( 'NONE', #70287, #79425, #1580, .T. ) ;
#75294=VERTEX_POINT ( 'NONE', #93533 ) ;
#75298=ORIENTED_EDGE ( 'NONE', *, *, #13814, .T. ) ;
#75306=ORIENTED_EDGE ( 'NONE', *, *, #16941, .T. ) ;
#75311=EDGE_CURVE ( 'NONE', #43600, #85662, #33789, .T. ) ;
#75315=DIRECTION ( 'NONE',  ( -0.2840153447039234780, 0.000000000000000000, 0.9588197348681928300 ) ) ;
#75327=VERTEX_POINT ( 'NONE', #71543 ) ;
#75340=CARTESIAN_POINT ( 'NONE',  ( 14.04391541078763161, 15.00000000000000000, 3.608107528142933340 ) ) ;
#75343=TOROIDAL_SURFACE ( 'NONE', #315, 14.49999999999999822, 0.5000000000000000000 ) ;
#75347=CARTESIAN_POINT ( 'NONE',  ( -14.94699059465102664, 0.5000000000000004441, 1.259949270174715696 ) ) ;
#75348=EDGE_CURVE ( 'NONE', #93129, #97596, #72496, .T. ) ;
#75349=DIRECTION ( 'NONE',  ( -0.6883545756937646809, -0.000000000000000000, 0.7253743710122776411 ) ) ;
#75353=CARTESIAN_POINT ( 'NONE',  ( -13.14228782657345107, 0.5000000000000004441, 7.230509711182143917 ) ) ;
#75358=LINE ( 'NONE', #28861, #51443 ) ;
#75364=ORIENTED_EDGE ( 'NONE', *, *, #13059, .F. ) ;
#75366=CARTESIAN_POINT ( 'NONE',  ( 4.326345305608627179, 0.000000000000000000, 3.319721512309613320 ) ) ;
#75370=CARTESIAN_POINT ( 'NONE',  ( -13.07964015051230788, 0.2306972965111898921, 7.222261988160647128 ) ) ;
#75376=CARTESIAN_POINT ( 'NONE',  ( -3.115783986955356522, 15.00000000000000000, -14.16128137375399554 ) ) ;
#75386=LINE ( 'NONE', #62716, #46103 ) ;
#75393=ORIENTED_EDGE ( 'NONE', *, *, #19435, .T. ) ;
#75396=ADVANCED_FACE ( 'NONE', ( #79524 ), #50003, .F. ) ;
#75412=CARTESIAN_POINT ( 'NONE',  ( -5.200846386093611606, 0.000000000000000000, -1.639820566681014391 ) ) ;
#75417=ORIENTED_EDGE ( 'NONE', *, *, #67842, .T. ) ;
#75420=CARTESIAN_POINT ( 'NONE',  ( 3.434112377981054287, -17.33469866340290721, -12.81628187352647608 ) ) ;
#75433=VERTEX_POINT ( 'NONE', #14508 ) ;
#75438=EDGE_CURVE ( 'NONE', #24788, #55265, #34325, .T. ) ;
#75439=VERTEX_POINT ( 'NONE', #44490 ) ;
#75445=CARTESIAN_POINT ( 'NONE',  ( 14.56332774647471062, 14.95077488074853456, 2.357028871694285765 ) ) ;
#75450=ORIENTED_EDGE ( 'NONE', *, *, #1622, .T. ) ;
#75452=DIRECTION ( 'NONE',  ( 0.000000000000000000, 0.000000000000000000, 1.000000000000000000 ) ) ;
#75476=CARTESIAN_POINT ( 'NONE',  ( 12.26659068614894466, -25.27958449841936073, -7.082119434687053960 ) ) ;
#75482=CARTESIAN_POINT ( 'NONE',  ( 0.1034006766821536916, 15.00000000000000000, -14.49963131600461352 ) ) ;
#75483=CARTESIAN_POINT ( 'NONE',  ( 0.000000000000000000, 14.49999999999999822, 0.000000000000000000 ) ) ;
#75486=AXIS2_PLACEMENT_3D ( 'NONE', #226, #30182, #91688 ) ;
#75488=DIRECTION ( 'NONE',  ( 0.000000000000000000, 1.000000000000000000, 0.000000000000000000 ) ) ;
#75492=CARTESIAN_POINT ( 'NONE',  ( 9.422509992056141925, 30.98035201082152668, -5.440088680355554374 ) ) ;
#75498=DIRECTION ( 'NONE',  ( -0.000000000000000000, -1.000000000000000000, -0.000000000000000000 ) ) ;
#75499=ORIENTED_EDGE ( 'NONE', *, *, #78931, .F. ) ;
#75502=DIRECTION ( 'NONE',  ( 0.9636304532086229502, 0.000000000000000000, -0.2672383760782571227 ) ) ;
#75507=LINE ( 'NONE', #83014, #1715 ) ;
#75508=EDGE_CURVE ( 'NONE', #90778, #74063, #78643, .T. ) ;
#75516=LINE ( 'NONE', #28536, #86772 ) ;
#75520=CARTESIAN_POINT ( 'NONE',  ( 12.25993886608607752, 0.3639311184075608718, -8.642563219313650791 ) ) ;
#75523=LINE ( 'NONE', #90028, #46519 ) ;
#75527=AXIS2_PLACEMENT_3D ( 'NONE', #50728, #66713, #88219 ) ;
#75532=CARTESIAN_POINT ( 'NONE',  ( 2.393480905993157215, 0.3640475087720930203, -14.80781041047751678 ) ) ;
#75537=EDGE_CURVE ( 'NONE', #78530, #54903, #1478, .T. ) ;
#75542=CARTESIAN_POINT ( 'NONE',  ( -8.527530157486182816, 10.59226448433412493, -4.923371831947288335 ) ) ;
#75555=TOROIDAL_SURFACE ( 'NONE', #43565, 14.49999999999999822, 0.5000000000000000000 ) ;
#75556=EDGE_CURVE ( 'NONE', #62860, #86850, #91472, .T. ) ;
#75576=DIRECTION ( 'NONE',  ( -0.1822355254921513845, 0.000000000000000000, 0.9832549075639538394 ) ) ;
#75580=CARTESIAN_POINT ( 'NONE',  ( 10.58981376305282041, 15.00000000000000000, 9.535111140613782510 ) ) ;
#75586=CARTESIAN_POINT ( 'NONE',  ( 9.402796353261145157, 14.49999999999999112, -11.68706210897763320 ) ) ;
#75594=AXIS2_PLACEMENT_3D ( 'NONE', #62899, #39915, #46908 ) ;
#75596=EDGE_LOOP ( 'NONE', ( #4340, #95719, #52411, #17182, #83295, #79202 ) ) ;
#75602=CARTESIAN_POINT ( 'NONE',  ( 0.000000000000000000, 15.00000000000000000, 13.75000000000001776 ) ) ;
#75604=LINE ( 'NONE', #76096, #77262 ) ;
#75608=CARTESIAN_POINT ( 'NONE',  ( -10.88017736071109987, -16.72798132251182679, 2.915334737309934532 ) ) ;
#75613=CARTESIAN_POINT ( 'NONE',  ( -14.09394518620607606, 3.895088541583166744E-16, -3.407449058785548157 ) ) ;
#75623=DIRECTION ( 'NONE',  ( 0.000000000000000000, 1.000000000000000000, 0.000000000000000000 ) ) ;
#75636=ORIENTED_EDGE ( 'NONE', *, *, #68889, .T. ) ;
#75639=EDGE_CURVE ( 'NONE', #25555, #71703, #30795, .T. ) ;
#75640=ORIENTED_EDGE ( 'NONE', *, *, #97600, .T. ) ;
#75657=CARTESIAN_POINT ( 'NONE',  ( 8.527530157486175710, -26.07440218233254470, -4.923371831947298993 ) ) ;
#75660=ORIENTED_EDGE ( 'NONE', *, *, #95525, .F. ) ;
#75671=CARTESIAN_POINT ( 'NONE',  ( -12.81628187352647252, 19.33196800326376064, 3.434112377981066722 ) ) ;
#75681=CARTESIAN_POINT ( 'NONE',  ( -10.84451454130493708, 4.806230040756559413E-16, -9.625305416630981270 ) ) ;
#75686=VERTEX_POINT ( 'NONE', #62431 ) ;
#75688=VECTOR ( 'NONE', #67155, 1000.000000000000114 ) ;
#75689=DIRECTION ( 'NONE',  ( -0.9799247046208311440, 0.000000000000000000, 0.1993679344171901680 ) ) ;
#75691=VERTEX_POINT ( 'NONE', #24467 ) ;
#75698=CARTESIAN_POINT ( 'NONE',  ( -14.82269085861165792, 15.00000000000000000, -2.299529454047158250 ) ) ;
#75726=CARTESIAN_POINT ( 'NONE',  ( -12.26659068614894110, 22.22041550158063217, 7.082119434687058401 ) ) ;
#75739=DIRECTION ( 'NONE',  ( 0.000000000000000000, 1.000000000000000000, -0.000000000000000000 ) ) ;
#75757=ADVANCED_FACE ( 'NONE', ( #44368 ), #81380, .F. ) ;
#75760=CARTESIAN_POINT ( 'NONE',  ( 3.014428414850134796, 4.380135511184874098, 11.24999999999999822 ) ) ;
#75766=CARTESIAN_POINT ( 'NONE',  ( 1.683889348827610062E-15, 0.000000000000000000, 13.74999999999999467 ) ) ;
#75776=ORIENTED_EDGE ( 'NONE', *, *, #52463, .F. ) ;
#75779=ORIENTED_EDGE ( 'NONE', *, *, #14262, .F. ) ;
#75783=CARTESIAN_POINT ( 'NONE',  ( 7.313705784284503686, 0.5000000000000004441, 13.09617149020748705 ) ) ;
#75784=ORIENTED_EDGE ( 'NONE', *, *, #21862, .F. ) ;
#75817=DIRECTION ( 'NONE',  ( 0.000000000000000000, 0.000000000000000000, 1.000000000000000000 ) ) ;
#75821=DIRECTION ( 'NONE',  ( 0.5807029557109463225, 0.000000000000000000, -0.8141155183563145714 ) ) ;
#75829=AXIS2_PLACEMENT_3D ( 'NONE', #27851, #96879, #89838 ) ;
#75836=LINE ( 'NONE', #90327, #59939 ) ;
#75840=CARTESIAN_POINT ( 'NONE',  ( 3.468686501387198362, 0.000000000000000000, -4.207853202970280648 ) ) ;
#75846=ORIENTED_EDGE ( 'NONE', *, *, #36389, .T. ) ;
#75847=DIRECTION ( 'NONE',  ( 0.000000000000000000, 1.000000000000000000, -0.000000000000000000 ) ) ;
#75848=EDGE_CURVE ( 'NONE', #76346, #70990, #75358, .T. ) ;
#75849=CARTESIAN_POINT ( 'NONE',  ( 14.97687855664608314, 0.5000000000000004441, -0.8325315005900512100 ) ) ;
#75858=CARTESIAN_POINT ( 'NONE',  ( 1.820328553599862786, 0.000000000000000000, 5.140449258537825195 ) ) ;
#75859=CARTESIAN_POINT ( 'NONE',  ( 0.000000000000000000, 14.49999999999999822, 0.000000000000000000 ) ) ;
#75872=CARTESIAN_POINT ( 'NONE',  ( -12.00809552683946357, 15.00000000000000000, -8.989195838243713155 ) ) ;
#75878=DIRECTION ( 'NONE',  ( 0.5075383629607025382, 0.000000000000000000, -0.8616291604415267091 ) ) ;
#75881=B_SPLINE_CURVE_WITH_KNOTS ( 'NONE', 3,
 ( #9077, #92567, #85078, #16587, #30088, #85574 ),
 .UNSPECIFIED., .F., .F.,
 ( 4, 2, 4 ),
 ( 3.409110551496079869E-05, 0.0004400426677367856500, 0.0008459942299586105082 ),
 .UNSPECIFIED. ) ;
#75882=ADVANCED_FACE ( 'NONE', ( #59860 ), #14383, .F. ) ;
#75889=ADVANCED_FACE ( 'NONE', ( #6872 ), #13106, .T. ) ;
#75890=CARTESIAN_POINT ( 'NONE',  ( 5.815502996284953596, 14.76930270348881002, -13.76292046016122228 ) ) ;
#75895=EDGE_LOOP ( 'NONE', ( #34705, #86553, #86242, #58924 ) ) ;
#75908=DIRECTION ( 'NONE',  ( 0.000000000000000000, 0.000000000000000000, 1.000000000000000000 ) ) ;
#75909=AXIS2_PLACEMENT_3D ( 'NONE', #35228, #27731, #19744 ) ;
#75911=CARTESIAN_POINT ( 'NONE',  ( -14.49440716394874151, 15.00000000000000000, 0.4026921475165272657 ) ) ;
#75915=CARTESIAN_POINT ( 'NONE',  ( -3.434112377981067610, -21.91803199673624647, -12.81628187352647252 ) ) ;
#75930=DIRECTION ( 'NONE',  ( 0.000000000000000000, 0.000000000000000000, 1.000000000000000000 ) ) ;
#75941=CARTESIAN_POINT ( 'NONE',  ( 12.22506292814015261, 0.2306972965111908358, 8.589871424854795379 ) ) ;
#75942=DIRECTION ( 'NONE',  ( 0.000000000000000000, 1.000000000000000000, 0.000000000000000000 ) ) ;
#75944=ORIENTED_EDGE ( 'NONE', *, *, #78748, .F. ) ;
#75946=CARTESIAN_POINT ( 'NONE',  ( 2.827051895225787703, 0.2301501044984899935, -14.67071941139712443 ) ) ;
#75948=AXIS2_PLACEMENT_3D ( 'NONE', #17226, #77703, #63186 ) ;
#75957=CARTESIAN_POINT ( 'NONE',  ( 3.469446951953614189E-15, 4.171802177851546389, 11.25000000000000355 ) ) ;
#75963=CARTESIAN_POINT ( 'NONE',  ( 5.448048636097843733, 0.000000000000000000, 0.2378669404634861928 ) ) ;
#75967=CARTESIAN_POINT ( 'NONE',  ( 3.469446951953614189E-15, -16.94625116508602858, 14.16423886937410259 ) ) ;
#75971=AXIS2_PLACEMENT_3D ( 'NONE', #26340, #9882, #19340 ) ;
#75974=CARTESIAN_POINT ( 'NONE',  ( -13.40508947812170781, 4.272460637706398645E-16, 5.527528931046010285 ) ) ;
#75979=FACE_OUTER_BOUND ( 'NONE', #70493, .T. ) ;
#75981=CARTESIAN_POINT ( 'NONE',  ( 0.000000000000000000, 15.00000000000000000, 0.000000000000000000 ) ) ;
#75984=CARTESIAN_POINT ( 'NONE',  ( -7.964842623401172439, 28.68868534415483751, 7.964842623401183097 ) ) ;
#75990=ORIENTED_EDGE ( 'NONE', *, *, #62351, .T. ) ;
#75993=PLANE ( 'NONE',  #86409 ) ;
#76001=DIRECTION ( 'NONE',  ( 0.000000000000000000, 0.000000000000000000, 1.000000000000000000 ) ) ;
#76003=ORIENTED_EDGE ( 'NONE', *, *, #87724, .T. ) ;
#76004=EDGE_CURVE ( 'NONE', #41516, #14084, #8833, .T. ) ;
#76013=DIRECTION ( 'NONE',  ( 0.000000000000000000, 1.000000000000000000, 0.000000000000000000 ) ) ;
#76016=CARTESIAN_POINT ( 'NONE',  ( 11.96291822454881348, 3.986488846351010315E-16, -8.193813980849080636 ) ) ;
#76019=VERTEX_POINT ( 'NONE', #61339 ) ;
#76024=CARTESIAN_POINT ( 'NONE',  ( -4.391700990646977054, 14.76930270348881002, -14.28114200970196102 ) ) ;
#76025=CARTESIAN_POINT ( 'NONE',  ( 2.393480905993150998, 0.5000000000000004441, -14.80781041047751323 ) ) ;
#76030=DIRECTION ( 'NONE',  ( -0.09584575252021386438, 0.000000000000000000, -0.9953961983671798519 ) ) ;
#76033=CARTESIAN_POINT ( 'NONE',  ( -4.923371831947292776, 11.84226448433412671, 8.527530157486181039 ) ) ;
#76034=EDGE_LOOP ( 'NONE', ( #73731, #96332, #86136, #65971, #70141, #83713 ) ) ;
#76035=EDGE_LOOP ( 'NONE', ( #29535, #79832, #72499, #58086, #20922, #91770 ) ) ;
#76037=ORIENTED_EDGE ( 'NONE', *, *, #70557, .T. ) ;
#76044=ADVANCED_FACE ( 'NONE', ( #76832 ), #48288, .T. ) ;
#76045=AXIS2_PLACEMENT_3D ( 'NONE', #13423, #66918, #43908 ) ;
#76047=CIRCLE ( 'NONE', #42502, 15.00000000000000000 ) ;
#76062=ORIENTED_EDGE ( 'NONE', *, *, #39371, .F. ) ;
#76065=CARTESIAN_POINT ( 'NONE',  ( 0.000000000000000000, 0.5000000000000004441, 0.000000000000000000 ) ) ;
#76069=CARTESIAN_POINT ( 'NONE',  ( 0.000000000000000000, 0.000000000000000000, 0.000000000000000000 ) ) ;
#76074=DIRECTION ( 'NONE',  ( -0.000000000000000000, -1.000000000000000000, -0.000000000000000000 ) ) ;
#76077=VECTOR ( 'NONE', #13651, 1000.000000000000000 ) ;
#76080=CARTESIAN_POINT ( 'NONE',  ( 0.000000000000000000, 0.5000000000000004441, 0.000000000000000000 ) ) ;
#76086=ORIENTED_EDGE ( 'NONE', *, *, #61197, .F. ) ;
#76096=CARTESIAN_POINT ( 'NONE',  ( -14.02068044289371684, 15.00000000000000000, -5.331089937175857330 ) ) ;
#76100=CARTESIAN_POINT ( 'NONE',  ( -7.964842623401179544, -17.56131465584515539, -7.964842623401174215 ) ) ;
#76103=ADVANCED_FACE ( 'NONE', ( #62313 ), #15860, .F. ) ;
#76105=CARTESIAN_POINT ( 'NONE',  ( 13.14228782657340844, 0.3640475087720989600, -7.230509711182238064 ) ) ;
#76119=ORIENTED_EDGE ( 'NONE', *, *, #6118, .F. ) ;
#76121=EDGE_CURVE ( 'NONE', #15328, #24761, #23858, .T. ) ;
#76122=B_SPLINE_CURVE_WITH_KNOTS ( 'NONE', 3,
 ( #94236, #3253, #24782, #87228, #48248, #10266 ),
 .UNSPECIFIED., .F., .F.,
 ( 4, 2, 4 ),
 ( 0.0002800313526655926139, 0.0006862368888107507007, 0.001092442424955908896 ),
 .UNSPECIFIED. ) ;
#76124=DIRECTION ( 'NONE',  ( -0.07845909572784540154, 0.000000000000000000, 0.9969173337331279638 ) ) ;
#76133=AXIS2_PLACEMENT_3D ( 'NONE', #80063, #80564, #33564 ) ;
#76138=AXIS2_PLACEMENT_3D ( 'NONE', #81004, #50994, #43488 ) ;
#76151=CARTESIAN_POINT ( 'NONE',  ( 3.469446951953614189E-15, -17.74106884899920900, 9.846743663894594434 ) ) ;
#76153=CARTESIAN_POINT ( 'NONE',  ( 0.1558782227856947700, 15.00000000000000000, -14.62632331952783638 ) ) ;
#76167=CARTESIAN_POINT ( 'NONE',  ( 3.469446951953614189E-15, 25.37363466993042138, 12.81628187352647608 ) ) ;
#76177=CARTESIAN_POINT ( 'NONE',  ( 13.07734668325339200, 2.778268066994105112E-16, 6.551438809693018506 ) ) ;
#76178=DIRECTION ( 'NONE',  ( 0.000000000000000000, 0.000000000000000000, 1.000000000000000000 ) ) ;
#76187=AXIS2_PLACEMENT_3D ( 'NONE', #78537, #9546, #39071 ) ;
#76192=CARTESIAN_POINT ( 'NONE',  ( 10.64017930668204670, 14.49999999999999112, 10.57291749337225362 ) ) ;
#76194=VECTOR ( 'NONE', #69553, 1000.000000000000000 ) ;
#76195=VERTEX_POINT ( 'NONE', #24350 ) ;
#76201=DIRECTION ( 'NONE',  ( 0.6494480483301898754, 0.000000000000000000, -0.7604059656000257128 ) ) ;
#76211=CARTESIAN_POINT ( 'NONE',  ( 0.8653096853334164562, -2.809184769568886286E-15, -14.59999144042651942 ) ) ;
#76212=EDGE_CURVE ( 'NONE', #26051, #4700, #22873, .T. ) ;
#76214=EDGE_CURVE ( 'NONE', #87207, #53171, #76351, .T. ) ;
#76221=CARTESIAN_POINT ( 'NONE',  ( 0.000000000000000000, 15.00000000000000000, 0.000000000000000000 ) ) ;
#76225=DIRECTION ( 'NONE',  ( -0.000000000000000000, -1.000000000000000000, -0.000000000000000000 ) ) ;
#76229=CARTESIAN_POINT ( 'NONE',  ( 14.16423886937410082, 24.51208216824729647, -3.795296366450314096 ) ) ;
#76241=PLANE ( 'NONE',  #67964 ) ;
#76242=CIRCLE ( 'NONE', #52252, 15.00000000000000000 ) ;
#76258=AXIS2_PLACEMENT_3D ( 'NONE', #44749, #75252, #7764 ) ;
#76262=CARTESIAN_POINT ( 'NONE',  ( 11.24999999999999822, 5.630135511184877650, -3.014428414850134796 ) ) ;
#76274=AXIS2_PLACEMENT_3D ( 'NONE', #48718, #79221, #3236 ) ;
#76276=EDGE_LOOP ( 'NONE', ( #71256, #96347, #72555, #14164 ) ) ;
#76280=VERTEX_POINT ( 'NONE', #64274 ) ;
#76285=ORIENTED_EDGE ( 'NONE', *, *, #45048, .T. ) ;
#76286=TOROIDAL_SURFACE ( 'NONE', #6053, 14.49999999999999822, 0.5000000000000000000 ) ;
#76292=EDGE_LOOP ( 'NONE', ( #23057, #220, #84287, #15456 ) ) ;
#76295=CARTESIAN_POINT ( 'NONE',  ( 14.16722289976682170, 0.3640475087720934089, 4.928467845925620594 ) ) ;
#76296=DIRECTION ( 'NONE',  ( 0.7009092642998425715, 0.000000000000000000, 0.7132504491541897806 ) ) ;
#76300=ORIENTED_EDGE ( 'NONE', *, *, #2134, .F. ) ;
#76314=CARTESIAN_POINT ( 'NONE',  ( 0.000000000000000000, 15.00000000000000000, 0.000000000000000000 ) ) ;
#76326=EDGE_CURVE ( 'NONE', #35833, #15318, #62814, .T. ) ;
#76338=CARTESIAN_POINT ( 'NONE',  ( 6.767445849361251042, 0.3639308223168553624, -13.38662304974500472 ) ) ;
#76340=CARTESIAN_POINT ( 'NONE',  ( 9.876730923139225737, 0.5000000000000004441, 11.28938378619069560 ) ) ;
#76345=CARTESIAN_POINT ( 'NONE',  ( -11.22915323889586858, 15.00000000000000000, 8.773176023390528044 ) ) ;
#76346=VERTEX_POINT ( 'NONE', #18803 ) ;
#76347=EDGE_CURVE ( 'NONE', #37030, #58432, #48364, .T. ) ;
#76349=ADVANCED_FACE ( 'NONE', ( #48791 ), #80269, .T. ) ;
#76351=LINE ( 'NONE', #45353, #73835 ) ;
#76362=CARTESIAN_POINT ( 'NONE',  ( 12.00809552683953463, 14.63595249122789177, 8.989195838243631442 ) ) ;
#76368=DIRECTION ( 'NONE',  ( 0.8038568606172162845, 0.000000000000000000, 0.5948227867513425915 ) ) ;
#76370=CARTESIAN_POINT ( 'NONE',  ( 8.813102413620015341, 15.00000000000000000, 13.34940531570970457 ) ) ;
#76373=FACE_OUTER_BOUND ( 'NONE', #85641, .T. ) ;
#76383=CARTESIAN_POINT ( 'NONE',  ( 5.817157072110804350, 14.49999999999999112, -13.82608706751093663 ) ) ;
#76390=ORIENTED_EDGE ( 'NONE', *, *, #83383, .F. ) ;
#76399=CARTESIAN_POINT ( 'NONE',  ( 4.265913727722096205, 0.04962886353675406703, 14.12300574719581903 ) ) ;
#76402=DIRECTION ( 'NONE',  ( 0.000000000000000000, 0.000000000000000000, 1.000000000000000000 ) ) ;
#76408=CARTESIAN_POINT ( 'NONE',  ( -9.382169495545413795, -5.251365330069575954, 9.382169495545428006 ) ) ;
#76413=LINE ( 'NONE', #44917, #19599 ) ;
#76421=CARTESIAN_POINT ( 'NONE',  ( 0.000000000000000000, 14.49999999999999822, 0.000000000000000000 ) ) ;
#76433=CARTESIAN_POINT ( 'NONE',  ( -14.03351048042393856, -0.03417435944610275333, -2.474486531753901541 ) ) ;
#76436=CARTESIAN_POINT ( 'NONE',  ( 0.000000000000000000, 14.49999999999999822, 0.000000000000000000 ) ) ;
#76440=CARTESIAN_POINT ( 'NONE',  ( 8.235571585149866536, 3.243033628982648686, -8.235571585149871865 ) ) ;
#76441=EDGE_CURVE ( 'NONE', #952, #30382, #58059, .T. ) ;
#76445=EDGE_CURVE ( 'NONE', #66663, #71139, #87282, .T. ) ;
#76454=AXIS2_PLACEMENT_3D ( 'NONE', #14151, #23139, #30608 ) ;
#76463=CARTESIAN_POINT ( 'NONE',  ( 14.16423886937410259, -0.6962511650860301327, -2.602085213965210642E-15 ) ) ;
#76467=ORIENTED_EDGE ( 'NONE', *, *, #35977, .F. ) ;
#76475=CARTESIAN_POINT ( 'NONE',  ( -0.7375392941519102186, 14.49999999999999112, 14.98185688723476616 ) ) ;
#76486=EDGE_LOOP ( 'NONE', ( #86140, #69038, #16645, #48465, #69023, #2091 ) ) ;
#76491=AXIS2_PLACEMENT_3D ( 'NONE', #8400, #98942, #54378 ) ;
#76497=CARTESIAN_POINT ( 'NONE',  ( 13.78891971893208357, 14.49999999999999822, -5.904717858191528279 ) ) ;
#76499=ORIENTED_EDGE ( 'NONE', *, *, #19629, .T. ) ;
#76511=DIRECTION ( 'NONE',  ( -0.000000000000000000, -1.000000000000000000, -0.000000000000000000 ) ) ;
#76516=B_SPLINE_CURVE_WITH_KNOTS ( 'NONE', 3,
 ( #34393, #57400, #2472, #86921, #71443, #1971 ),
 .UNSPECIFIED., .F., .F.,
 ( 4, 2, 4 ),
 ( 3.409110551494654820E-05, 0.0004400426677367926431, 0.0008459942299586388059 ),
 .UNSPECIFIED. ) ;
#76518=CARTESIAN_POINT ( 'NONE',  ( 3.866352809135573221, 14.95037102884062996, 14.23757791217548707 ) ) ;
#76523=CARTESIAN_POINT ( 'NONE',  ( 8.564643372776551189, 14.49999999999999112, 12.31449893000752915 ) ) ;
#76526=CARTESIAN_POINT ( 'NONE',  ( -6.408140936763232709, -40.04303199673623936, 11.09922568453595026 ) ) ;
#76528=VECTOR ( 'NONE', #21153, 1000.000000000000000 ) ;
#76529=DIRECTION ( 'NONE',  ( -0.9914448613738112703, 0.000000000000000000, 0.1305261922200445235 ) ) ;
#76537=ADVANCED_FACE ( 'NONE', ( #63783 ), #11289, .F. ) ;
#76539=VERTEX_POINT ( 'NONE', #94292 ) ;
#76542=EDGE_LOOP ( 'NONE', ( #7661, #59203, #44137, #46778 ) ) ;
#76551=DIRECTION ( 'NONE',  ( 0.7716245833877192206, 0.000000000000000000, -0.6360782202777647276 ) ) ;
#76553=EDGE_CURVE ( 'NONE', #7375, #86520, #40818, .T. ) ;
#76557=B_SPLINE_CURVE_WITH_KNOTS ( 'NONE', 3,
 ( #90604, #82119, #143, #58634, #81624, #43629 ),
 .UNSPECIFIED., .F., .F.,
 ( 4, 2, 4 ),
 ( 3.409110551496222848E-05, 0.0004400426677368007205, 0.0008459942299586391311 ),
 .UNSPECIFIED. ) ;
#76561=ORIENTED_EDGE ( 'NONE', *, *, #22957, .F. ) ;
#76571=DIRECTION ( 'NONE',  ( -0.9366721892483995671, 0.000000000000000000, 0.3502073812594621027 ) ) ;
#76575=ORIENTED_EDGE ( 'NONE', *, *, #91912, .T. ) ;
#76590=CARTESIAN_POINT ( 'NONE',  ( 10.88017736071110164, -14.64464798917848753, 2.915334737309921209 ) ) ;
#76594=CARTESIAN_POINT ( 'NONE',  ( 11.62719953690064933, 0.5000000000000004441, -9.476720473301794456 ) ) ;
#76596=EDGE_CURVE ( 'NONE', #87174, #26702, #59743, .T. ) ;
#76597=LINE ( 'NONE', #38609, #5042 ) ;
#76619=CARTESIAN_POINT ( 'NONE',  ( 14.04391541078762984, 15.00000000000000000, -3.608107528142820986 ) ) ;
#76622=VERTEX_POINT ( 'NONE', #36764 ) ;
#76634=DIRECTION ( 'NONE',  ( 0.000000000000000000, 1.000000000000000000, 0.000000000000000000 ) ) ;
#76637=CARTESIAN_POINT ( 'NONE',  ( -9.846743663894590881, -23.78273551566588395, 2.638427012816840111 ) ) ;
#76638=ORIENTED_EDGE ( 'NONE', *, *, #98965, .T. ) ;
#76641=ORIENTED_EDGE ( 'NONE', *, *, #15283, .T. ) ;
#76647=CARTESIAN_POINT ( 'NONE',  ( 0.000000000000000000, 0.5000000000000004441, 0.000000000000000000 ) ) ;
#76649=EDGE_CURVE ( 'NONE', #75439, #90631, #83497, .T. ) ;
#76650=ADVANCED_FACE ( 'NONE', ( #5773 ), #81745, .F. ) ;
#76652=CARTESIAN_POINT ( 'NONE',  ( 12.81628187352647252, 21.83196800326374643, -3.434112377981059172 ) ) ;
#76653=ORIENTED_EDGE ( 'NONE', *, *, #53491, .T. ) ;
#76662=ADVANCED_FACE ( 'NONE', ( #51261 ), #73264, .F. ) ;
#76663=CARTESIAN_POINT ( 'NONE',  ( 14.91937968691865457, 14.76930270348881180, -0.8063277559918125004 ) ) ;
#76666=CARTESIAN_POINT ( 'NONE',  ( -6.689969769698787871, 15.00000000000000000, -12.58200319823979285 ) ) ;
#76667=ORIENTED_EDGE ( 'NONE', *, *, #95856, .F. ) ;
#76668=ADVANCED_FACE ( 'NONE', ( #67257 ), #90238, .F. ) ;
#76669=CARTESIAN_POINT ( 'NONE',  ( 0.000000000000000000, 0.5000000000000004441, 0.000000000000000000 ) ) ;
#76672=ORIENTED_EDGE ( 'NONE', *, *, #28457, .F. ) ;
#76674=CARTESIAN_POINT ( 'NONE',  ( 0.000000000000000000, 14.49999999999999822, 0.000000000000000000 ) ) ;
#76677=CARTESIAN_POINT ( 'NONE',  ( 0.000000000000000000, 15.00000000000000000, 0.000000000000000000 ) ) ;
#76680=DIRECTION ( 'NONE',  ( 0.000000000000000000, 1.000000000000000000, 0.000000000000000000 ) ) ;
#76690=CARTESIAN_POINT ( 'NONE',  ( 0.7375392941518169598, 0.3639308982088801936, -14.98185688723474307 ) ) ;
#76694=EDGE_LOOP ( 'NONE', ( #41215, #39206, #26497, #96599, #2911, #36739 ) ) ;
#76697=CIRCLE ( 'NONE', #30374, 15.00000000000000000 ) ;
#76704=CARTESIAN_POINT ( 'NONE',  ( 5.093587308868497310, -0.03417435944610275333, -15.16353404595997567 ) ) ;
#76707=CARTESIAN_POINT ( 'NONE',  ( -14.16423886937410082, 21.80374883491398208, 4.336808689942017736E-15 ) ) ;
#76709=AXIS2_PLACEMENT_3D ( 'NONE', #79243, #79739, #11236 ) ;
#76745=LINE ( 'NONE', #68280, #42866 ) ;
#76750=CARTESIAN_POINT ( 'NONE',  ( 1.780824192092386404, 14.49999999999999112, 14.89391369643520946 ) ) ;
#76762=EDGE_LOOP ( 'NONE', ( #47763, #17860, #84925, #21220, #90587, #1628 ) ) ;
#76766=CARTESIAN_POINT ( 'NONE',  ( 7.002992508388946824, -3.201784540621254098E-15, 12.84003923133022695 ) ) ;
#76772=ORIENTED_EDGE ( 'NONE', *, *, #54217, .T. ) ;
#76776=VERTEX_POINT ( 'NONE', #42096 ) ;
#76791=EDGE_CURVE ( 'NONE', #44200, #92170, #96079, .T. ) ;
#76795=CARTESIAN_POINT ( 'NONE',  ( 0.000000000000000000, 14.49999999999999822, 0.000000000000000000 ) ) ;
#76798=CARTESIAN_POINT ( 'NONE',  ( 14.56195259121204799, 6.403569081242508591E-16, -1.374002722866695336 ) ) ;
#76814=DIRECTION ( 'NONE',  ( 0.000000000000000000, 1.000000000000000000, 0.000000000000000000 ) ) ;
#76817=CARTESIAN_POINT ( 'NONE',  ( -0.9940297508535884674, 15.00000000000000000, -14.21528771620250886 ) ) ;
#76822=CARTESIAN_POINT ( 'NONE',  ( -5.817157072110620497, 14.49999999999999112, -13.82608706751101302 ) ) ;
#76823=DIRECTION ( 'NONE',  ( 0.000000000000000000, 1.000000000000000000, 0.000000000000000000 ) ) ;
#76827=AXIS2_PLACEMENT_3D ( 'NONE', #50649, #4172, #67125 ) ;
#76832=FACE_OUTER_BOUND ( 'NONE', #1407, .T. ) ;
#76833=CARTESIAN_POINT ( 'NONE',  ( -13.07661834287478797, 15.00000000000000711, -6.550615570651864061 ) ) ;
#76848=CARTESIAN_POINT ( 'NONE',  ( 10.09777502097884216, 14.95077488074853456, -10.75551206493379830 ) ) ;
#76849=DIRECTION ( 'NONE',  ( -0.5948227867513427025, 0.000000000000000000, 0.8038568606172163955 ) ) ;
#76855=DIRECTION ( 'NONE',  ( 0.000000000000000000, 1.000000000000000000, 0.000000000000000000 ) ) ;
#76870=ORIENTED_EDGE ( 'NONE', *, *, #27596, .F. ) ;
#76873=AXIS2_PLACEMENT_3D ( 'NONE', #82853, #92323, #61818 ) ;
#76878=VERTEX_POINT ( 'NONE', #67532 ) ;
#76880=ADVANCED_FACE ( 'NONE', ( #28037 ), #73530, .F. ) ;
#76882=TOROIDAL_SURFACE ( 'NONE', #19432, 14.49999999999999822, 0.5000000000000000000 ) ;
#76888=CARTESIAN_POINT ( 'NONE',  ( -14.09394518620614711, 15.00000000000000000, 3.407449058785264384 ) ) ;
#76889=CARTESIAN_POINT ( 'NONE',  ( -14.99847009497950978, 14.49999999999999112, 0.2142307401079103502 ) ) ;
#76902=EDGE_CURVE ( 'NONE', #59535, #45656, #3708, .T. ) ;
#76904=CARTESIAN_POINT ( 'NONE',  ( 0.000000000000000000, 14.49999999999999822, 0.000000000000000000 ) ) ;
#76910=EDGE_CURVE ( 'NONE', #74647, #69120, #69156, .T. ) ;
#76912=B_SPLINE_CURVE_WITH_KNOTS ( 'NONE', 3,
 ( #75613, #16103, #22629, #46590, #640, #83617 ),
 .UNSPECIFIED., .F., .F.,
 ( 4, 2, 4 ),
 ( 0.0002800026249563186903, 0.0006862078800502437095, 0.001092413135144168837 ),
 .UNSPECIFIED. ) ;
#76917=DIRECTION ( 'NONE',  ( 0.000000000000000000, 1.000000000000000000, 0.000000000000000000 ) ) ;
#76920=PLANE ( 'NONE',  #75594 ) ;
#76922=CARTESIAN_POINT ( 'NONE',  ( 14.99847009497944583, 15.00000000000000000, -0.2142307401080305596 ) ) ;
#76932=DIRECTION ( 'NONE',  ( -0.7253743710122912969, 0.000000000000000000, 0.6883545756937501370 ) ) ;
#76941=ORIENTED_EDGE ( 'NONE', *, *, #21041, .F. ) ;
#76943=DIRECTION ( 'NONE',  ( -0.2334453638559087496, 0.000000000000000000, 0.9723699203976758909 ) ) ;
#76948=CARTESIAN_POINT ( 'NONE',  ( -14.16423886937409726, -12.98791783175269643, 3.795296366450320757 ) ) ;
#76951=CIRCLE ( 'NONE', #67394, 14.49999999999999822 ) ;
#76963=EDGE_CURVE ( 'NONE', #13116, #17551, #13249, .T. ) ;
#76973=EDGE_CURVE ( 'NONE', #93626, #45054, #58532, .T. ) ;
#76987=DIRECTION ( 'NONE',  ( 0.000000000000000000, 0.000000000000000000, 1.000000000000000000 ) ) ;
#76988=DIRECTION ( 'NONE',  ( -0.000000000000000000, -1.000000000000000000, -0.000000000000000000 ) ) ;
#77001=VECTOR ( 'NONE', #8452, 1000.000000000000000 ) ;
#77005=EDGE_CURVE ( 'NONE', #22285, #86977, #75516, .T. ) ;
#77009=CARTESIAN_POINT ( 'NONE',  ( -10.19513985507841447, 14.63595249122789177, 11.00268709613211371 ) ) ;
#77015=CARTESIAN_POINT ( 'NONE',  ( -5.845017550302832987, 15.00000000000000000, -14.89003580495041668 ) ) ;
#77018=CARTESIAN_POINT ( 'NONE',  ( 9.382169495545419124, -39.00136533006958217, 9.382169495545417348 ) ) ;
#77019=VERTEX_POINT ( 'NONE', #34846 ) ;
#77021=ORIENTED_EDGE ( 'NONE', *, *, #10215, .T. ) ;
#77029=VECTOR ( 'NONE', #73334, 999.9999999999998863 ) ;
#77030=EDGE_CURVE ( 'NONE', #86977, #9285, #88336, .T. ) ;
#77036=ORIENTED_EDGE ( 'NONE', *, *, #77030, .T. ) ;
#77038=ORIENTED_EDGE ( 'NONE', *, *, #45390, .T. ) ;
#77049=ORIENTED_EDGE ( 'NONE', *, *, #71517, .T. ) ;
#77050=DIRECTION ( 'NONE',  ( 0.000000000000000000, 0.000000000000000000, -1.000000000000000000 ) ) ;
#77052=AXIS2_PLACEMENT_3D ( 'NONE', #36980, #34986, #52467 ) ;
#77066=VECTOR ( 'NONE', #86795, 1000.000000000000114 ) ;
#77069=VERTEX_POINT ( 'NONE', #4381 ) ;
#77070=ORIENTED_EDGE ( 'NONE', *, *, #67793, .T. ) ;
#77082=CARTESIAN_POINT ( 'NONE',  ( 9.422509992056141925, -4.019647989178490199, -5.440088680355554374 ) ) ;
#77088=DIRECTION ( 'NONE',  ( -0.2334453638559087496, 0.000000000000000000, 0.9723699203976758909 ) ) ;
#77090=TOROIDAL_SURFACE ( 'NONE', #26004, 14.49999999999999822, 0.5000000000000000000 ) ;
#77092=CYLINDRICAL_SURFACE ( 'NONE', #28105, 15.00000000000000000 ) ;
#77096=DIRECTION ( 'NONE',  ( -0.9890158633619177131, 0.000000000000000000, 0.1478094111296046342 ) ) ;
#77098=EDGE_LOOP ( 'NONE', ( #11824, #40156, #4460, #52109 ) ) ;
#77111=VERTEX_POINT ( 'NONE', #81826 ) ;
#77114=EDGE_CURVE ( 'NONE', #70392, #44443, #88355, .T. ) ;
#77126=CARTESIAN_POINT ( 'NONE',  ( 4.838527690343520149, 14.49999999999999112, 14.19819177887736927 ) ) ;
#77129=CARTESIAN_POINT ( 'NONE',  ( 8.527530157486179263, -16.90773551566587685, 4.923371831947292776 ) ) ;
#77130=VERTEX_POINT ( 'NONE', #43340 ) ;
#77142=EDGE_LOOP ( 'NONE', ( #74569, #63476, #98534, #77021 ) ) ;
#77145=ORIENTED_EDGE ( 'NONE', *, *, #94125, .T. ) ;
#77153=CARTESIAN_POINT ( 'NONE',  ( 6.767445849361247490, 0.5000000000000004441, -13.38662304974496564 ) ) ;
#77155=EDGE_CURVE ( 'NONE', #86532, #17162, #19370, .T. ) ;
#77156=DIRECTION ( 'NONE',  ( 0.000000000000000000, 0.000000000000000000, -1.000000000000000000 ) ) ;
#77158=AXIS2_PLACEMENT_3D ( 'NONE', #16924, #98973, #31897 ) ;
#77162=ORIENTED_EDGE ( 'NONE', *, *, #49690, .T. ) ;
#77163=CARTESIAN_POINT ( 'NONE',  ( 2.933660812629996339, -0.03417435944610275333, -15.72485391577589731 ) ) ;
#77171=CARTESIAN_POINT ( 'NONE',  ( -14.17193700899788134, 15.00000000000000000, -1.489530601564206247 ) ) ;
#77175=CARTESIAN_POINT ( 'NONE',  ( -11.59608414876335658, 0.2306972965111898921, -9.421724210956444523 ) ) ;
#77184=LINE ( 'NONE', #39208, #18617 ) ;
#77188=LINE ( 'NONE', #8696, #85584 ) ;
#77189=CIRCLE ( 'NONE', #18176, 15.00000000000000000 ) ;
#77190=CARTESIAN_POINT ( 'NONE',  ( 4.023424921641736596, 15.00000000000000000, -15.48190712851506667 ) ) ;
#77191=CARTESIAN_POINT ( 'NONE',  ( 3.469446951953614189E-15, 3.912123368507817833, 11.92686044187656513 ) ) ;
#77194=CARTESIAN_POINT ( 'NONE',  ( -11.62719953690071506, 0.5000000000000004441, 9.476720473301710967 ) ) ;
#77197=CIRCLE ( 'NONE', #3774, 14.49999999999999822 ) ;
#77198=CARTESIAN_POINT ( 'NONE',  ( -7.082119434687058401, 30.97041550158063927, -12.26659068614894110 ) ) ;
#77207=VERTEX_POINT ( 'NONE', #35346 ) ;
#77221=FACE_OUTER_BOUND ( 'NONE', #98363, .T. ) ;
#77223=CARTESIAN_POINT ( 'NONE',  ( 9.898881779040660689, 15.00000000000000000, 10.25059215482582786 ) ) ;
#77231=ORIENTED_EDGE ( 'NONE', *, *, #28563, .T. ) ;
#77235=EDGE_CURVE ( 'NONE', #34058, #35670, #12840, .T. ) ;
#77241=FACE_OUTER_BOUND ( 'NONE', #2037, .T. ) ;
#77244=DIRECTION ( 'NONE',  ( 0.000000000000000000, 1.000000000000000000, 0.000000000000000000 ) ) ;
#77246=EDGE_CURVE ( 'NONE', #32363, #80599, #44955, .T. ) ;
#77249=ORIENTED_EDGE ( 'NONE', *, *, #48768, .T. ) ;
#77251=ORIENTED_EDGE ( 'NONE', *, *, #96753, .F. ) ;
#77262=VECTOR ( 'NONE', #23613, 1000.000000000000000 ) ;
#77266=DIRECTION ( 'NONE',  ( 0.1132032137679039180, 0.000000000000000000, 0.9935718556765877896 ) ) ;
#77270=EDGE_CURVE ( 'NONE', #88314, #79187, #28824, .T. ) ;
#77272=ORIENTED_EDGE ( 'NONE', *, *, #21286, .F. ) ;
#77273=DIRECTION ( 'NONE',  ( 3.375077994860475883E-14, 0.000000000000000000, 1.000000000000000000 ) ) ;
#77287=CARTESIAN_POINT ( 'NONE',  ( 14.76044511231851075, 0.2301501264598460050, 2.313329003772481851 ) ) ;
#77297=DIRECTION ( 'NONE',  ( 0.000000000000000000, 0.000000000000000000, 1.000000000000000000 ) ) ;
#77299=LINE ( 'NONE', #9805, #37726 ) ;
#77309=CARTESIAN_POINT ( 'NONE',  ( -0.3093388210927633941, 14.49999999999999822, -14.99680997725065978 ) ) ;
#77315=TOROIDAL_SURFACE ( 'NONE', #62983, 14.49999999999999822, 0.5000000000000000000 ) ;
#77317=EDGE_CURVE ( 'NONE', #84883, #89457, #79945, .T. ) ;
#77328=ORIENTED_EDGE ( 'NONE', *, *, #10014, .F. ) ;
#77330=PLANE ( 'NONE',  #82183 ) ;
#77336=DIRECTION ( 'NONE',  ( 0.000000000000000000, 0.000000000000000000, 1.000000000000000000 ) ) ;
#77348=EDGE_CURVE ( 'NONE', #98073, #65284, #21251, .T. ) ;
#77350=DIRECTION ( 'NONE',  ( -0.2672383760782703344, -0.000000000000000000, 0.9636304532086192864 ) ) ;
#77359=ORIENTED_EDGE ( 'NONE', *, *, #37974, .T. ) ;
#77365=ORIENTED_EDGE ( 'NONE', *, *, #67392, .T. ) ;
#77368=CARTESIAN_POINT ( 'NONE',  ( 14.29730467489533652, 3.971653163193037558E-16, -2.416004766803220516 ) ) ;
#77369=CARTESIAN_POINT ( 'NONE',  ( -14.15281240980442945, 15.00000000000000711, -3.688687068602892971 ) ) ;
#77384=EDGE_CURVE ( 'NONE', #14921, #93129, #98850, .T. ) ;
#77392=ORIENTED_EDGE ( 'NONE', *, *, #6684, .F. ) ;
#77406=ORIENTED_EDGE ( 'NONE', *, *, #29792, .T. ) ;
#77409=AXIS2_PLACEMENT_3D ( 'NONE', #81746, #13262, #66758 ) ;
#77418=CARTESIAN_POINT ( 'NONE',  ( -2.913501739333568707, 15.00000000000000000, -14.20427779279538960 ) ) ;
#77420=EDGE_CURVE ( 'NONE', #76539, #58682, #53812, .T. ) ;
#77426=CARTESIAN_POINT ( 'NONE',  ( -12.54342190210035213, 0.2301501149690338699, -8.116945096741464027 ) ) ;
#77428=CARTESIAN_POINT ( 'NONE',  ( 14.66148682522523217, 0.2301506158824408732, -2.874551585517186147 ) ) ;
#77431=CARTESIAN_POINT ( 'NONE',  ( 10.36894250292379027, -11.32125116508602858, 10.36894250292378672 ) ) ;
#77436=ORIENTED_EDGE ( 'NONE', *, *, #14870, .F. ) ;
#77441=DIRECTION ( 'NONE',  ( 0.000000000000000000, 1.000000000000000000, 0.000000000000000000 ) ) ;
#77445=LINE ( 'NONE', #16968, #86758 ) ;
#77460=CARTESIAN_POINT ( 'NONE',  ( -5.451370222425310885, 0.000000000000000000, -0.1427491530890833693 ) ) ;
#77468=DIRECTION ( 'NONE',  ( -0.000000000000000000, -1.000000000000000000, -0.000000000000000000 ) ) ;
#77475=EDGE_CURVE ( 'NONE', #84126, #30654, #38327, .T. ) ;
#77479=DIRECTION ( 'NONE',  ( 0.000000000000000000, 1.000000000000000000, 0.000000000000000000 ) ) ;
#77485=ORIENTED_EDGE ( 'NONE', *, *, #87250, .F. ) ;
#77490=CARTESIAN_POINT ( 'NONE',  ( -8.439016546559980014, 3.939291001653719071E-16, 11.79122553964967679 ) ) ;
#77491=CARTESIAN_POINT ( 'NONE',  ( -9.402796353260978179, 14.63606911086602658, -11.68706210897773978 ) ) ;
#77496=LINE ( 'NONE', #45532, #36454 ) ;
#77498=DIRECTION ( 'NONE',  ( -3.552713678800500929E-14, 0.000000000000000000, 1.000000000000000000 ) ) ;
#77499=CARTESIAN_POINT ( 'NONE',  ( -9.846743663894594434, 26.00893115100079456, 3.469446951953614189E-15 ) ) ;
#77515=ORIENTED_EDGE ( 'NONE', *, *, #65000, .T. ) ;
#77521=DIRECTION ( 'NONE',  ( -0.2334453638558956767, 0.000000000000000000, -0.9723699203976788885 ) ) ;
#77522=ADVANCED_FACE ( 'NONE', ( #29813 ), #78776, .T. ) ;
#77524=TOROIDAL_SURFACE ( 'NONE', #67984, 14.49999999999999822, 0.5000000000000000000 ) ;
#77527=VECTOR ( 'NONE', #76932, 1000.000000000000000 ) ;
#77529=VERTEX_POINT ( 'NONE', #92783 ) ;
#77532=VECTOR ( 'NONE', #72730, 1000.000000000000000 ) ;
#77538=DIRECTION ( 'NONE',  ( 0.2503800040544389427, 0.000000000000000000, 0.9681476403781082984 ) ) ;
#77547=CARTESIAN_POINT ( 'NONE',  ( -4.880290883660354240, 0.000000000000000000, 2.433223276543825975 ) ) ;
#77549=CARTESIAN_POINT ( 'NONE',  ( 0.3093388210927633941, 14.49999999999999822, 14.99680997725065978 ) ) ;
#77551=AXIS2_PLACEMENT_3D ( 'NONE', #44727, #76225, #37252 ) ;
#77555=ADVANCED_FACE ( 'NONE', ( #64238 ), #1330, .F. ) ;
#77567=CARTESIAN_POINT ( 'NONE',  ( 3.469446951953614189E-15, 4.313685344154848167, 10.88017736071110342 ) ) ;
#77569=B_SPLINE_CURVE_WITH_KNOTS ( 'NONE', 3,
 ( #84926, #92909, #953, #75946, #29941, #61918 ),
 .UNSPECIFIED., .F., .F.,
 ( 4, 2, 4 ),
 ( 0.0002800039672440411773, 0.0006862092354666055397, 0.001092414503689169902 ),
 .UNSPECIFIED. ) ;
#77571=CARTESIAN_POINT ( 'NONE',  ( 14.49440716394873263, 4.853942851202206293E-16, 0.4026921475167233311 ) ) ;
#77572=VECTOR ( 'NONE', #4277, 1000.000000000000000 ) ;
#77578=FACE_OUTER_BOUND ( 'NONE', #28575, .T. ) ;
#77588=EDGE_CURVE ( 'NONE', #4683, #30551, #89517, .T. ) ;
#77594=CARTESIAN_POINT ( 'NONE',  ( 0.7375392941517084910, 14.63606910179106535, 14.98185688723475195 ) ) ;
#77598=CARTESIAN_POINT ( 'NONE',  ( 14.04391541078765471, 3.833537969851530006E-16, -3.608107528142839637 ) ) ;
#77612=VECTOR ( 'NONE', #90185, 1000.000000000000114 ) ;
#77615=CARTESIAN_POINT ( 'NONE',  ( -9.846743663894596210, -14.19940218233255003, -2.638427012816824124 ) ) ;
#77618=LINE ( 'NONE', #93613, #55724 ) ;
#77625=CARTESIAN_POINT ( 'NONE',  ( -9.519554572443036378, 15.00000000000000178, 11.10344954678173757 ) ) ;
#77627=ORIENTED_EDGE ( 'NONE', *, *, #4039, .F. ) ;
#77637=CARTESIAN_POINT ( 'NONE',  ( 14.73513795193453468, 14.95077488074853456, -0.7223639599946776180 ) ) ;
#77640=B_SPLINE_CURVE_WITH_KNOTS ( 'NONE', 3,
 ( #2689, #33140, #63635, #10654, #71653, #57123 ),
 .UNSPECIFIED., .F., .F.,
 ( 4, 2, 4 ),
 ( 0.0002800553958269957748, 0.0006862611673083382664, 0.001092466938789680812 ),
 .UNSPECIFIED. ) ;
#77641=AXIS2_PLACEMENT_3D ( 'NONE', #97776, #755, #98771 ) ;
#77643=B_SPLINE_CURVE_WITH_KNOTS ( 'NONE', 3,
 ( #38195, #16666, #61167, #1680, #84663, #94982 ),
 .UNSPECIFIED., .F., .F.,
 ( 4, 2, 4 ),
 ( 3.409110551494649399E-05, 0.0004400426677367928600, 0.0008459942299586392395 ),
 .UNSPECIFIED. ) ;
#77647=FACE_OUTER_BOUND ( 'NONE', #59934, .T. ) ;
#77651=CARTESIAN_POINT ( 'NONE',  ( 0.3998276802503074046, -0.03417435944610275333, 15.99117050944548879 ) ) ;
#77656=CARTESIAN_POINT ( 'NONE',  ( 14.26328062697243837, 0.04962887699556053911, -3.770429249334784849 ) ) ;
#77657=CARTESIAN_POINT ( 'NONE',  ( 7.771322705631417804, 3.835866486557528145E-16, 12.24159072199922704 ) ) ;
#77669=CARTESIAN_POINT ( 'NONE',  ( -3.195792623639463592, 8.703790035174481687, 11.92686044187660421 ) ) ;
#77681=DIRECTION ( 'NONE',  ( 1.101341240428155162E-13, 0.000000000000000000, 1.000000000000000000 ) ) ;
#77685=CARTESIAN_POINT ( 'NONE',  ( -14.16423886937410082, 31.80374883491396432, 4.336808689942017736E-15 ) ) ;
#77693=AXIS2_PLACEMENT_3D ( 'NONE', #61421, #91931, #23458 ) ;
#77696=ORIENTED_EDGE ( 'NONE', *, *, #95205, .T. ) ;
#77698=AXIS2_PLACEMENT_3D ( 'NONE', #76080, #84578, #85066 ) ;
#77702=DIRECTION ( 'NONE',  ( 0.000000000000000000, 1.000000000000000000, 0.000000000000000000 ) ) ;
#77703=DIRECTION ( 'NONE',  ( 0.5224985647159496871, 0.000000000000000000, 0.8526401643540917341 ) ) ;
#77707=ORIENTED_EDGE ( 'NONE', *, *, #80326, .T. ) ;
#77719=VECTOR ( 'NONE', #42972, 1000.000000000000000 ) ;
#77720=EDGE_CURVE ( 'NONE', #98695, #62655, #31061, .T. ) ;
#77721=FACE_BOUND ( 'NONE', #26011, .T. ) ;
#77723=ORIENTED_EDGE ( 'NONE', *, *, #73953, .F. ) ;
#77731=CARTESIAN_POINT ( 'NONE',  ( -3.897244926436033374, 3.994152527635309729E-16, -13.96644127841335958 ) ) ;
#77733=AXIS2_PLACEMENT_3D ( 'NONE', #76669, #8187, #61651 ) ;
#77736=CARTESIAN_POINT ( 'NONE',  ( -11.94720539484397115, 14.76930270348885088, -8.972309510150314082 ) ) ;
#77740=VERTEX_POINT ( 'NONE', #20236 ) ;
#77744=ORIENTED_EDGE ( 'NONE', *, *, #11642, .F. ) ;
#77752=ORIENTED_EDGE ( 'NONE', *, *, #68363, .T. ) ;
#77755=ORIENTED_EDGE ( 'NONE', *, *, #49226, .T. ) ;
#77759=CARTESIAN_POINT ( 'NONE',  ( 0.9940297508536876103, 15.00000000000000000, 14.21528771620250353 ) ) ;
#77765=AXIS2_PLACEMENT_3D ( 'NONE', #22150, #30120, #44134 ) ;
#77766=VERTEX_POINT ( 'NONE', #50740 ) ;
#77769=DIRECTION ( 'NONE',  ( 0.000000000000000000, 0.000000000000000000, -1.000000000000000000 ) ) ;
#77791=EDGE_CURVE ( 'NONE', #65924, #7321, #77197, .T. ) ;
#77796=CARTESIAN_POINT ( 'NONE',  ( -5.810202895580550475, 14.95077488074853456, 13.56051778013760689 ) ) ;
#77801=LINE ( 'NONE', #9314, #84878 ) ;
#77808=ORIENTED_EDGE ( 'NONE', *, *, #92002, .T. ) ;
#77811=DIRECTION ( 'NONE',  ( 0.8788171126619646056, 0.000000000000000000, 0.4771587602596096267 ) ) ;
#77814=CARTESIAN_POINT ( 'NONE',  ( 3.384800920124074075, 14.76930270348881180, 14.55270344038010322 ) ) ;
#77815=ORIENTED_EDGE ( 'NONE', *, *, #90094, .F. ) ;
#77820=EDGE_LOOP ( 'NONE', ( #82646, #1672, #86393, #37562 ) ) ;
#77821=DIRECTION ( 'NONE',  ( -0.000000000000000000, -1.000000000000000000, -0.000000000000000000 ) ) ;
#77828=CARTESIAN_POINT ( 'NONE',  ( 13.82192141328809676, 4.465570197798056962E-16, 4.382292601468775750 ) ) ;
#77829=EDGE_CURVE ( 'NONE', #52174, #26555, #79755, .T. ) ;
#77840=VECTOR ( 'NONE', #22712, 1000.000000000000000 ) ;
#77853=EDGE_CURVE ( 'NONE', #31539, #97319, #89712, .T. ) ;
#77856=VERTEX_POINT ( 'NONE', #41771 ) ;
#77859=VERTEX_POINT ( 'NONE', #72726 ) ;
#77862=ORIENTED_EDGE ( 'NONE', *, *, #35008, .T. ) ;
#77873=ORIENTED_EDGE ( 'NONE', *, *, #85796, .T. ) ;
#77883=AXIS2_PLACEMENT_3D ( 'NONE', #66553, #97569, #45526 ) ;
#77886=EDGE_CURVE ( 'NONE', #12702, #83059, #34229, .T. ) ;
#77887=VERTEX_POINT ( 'NONE', #51226 ) ;
#77891=VECTOR ( 'NONE', #74163, 1000.000000000000000 ) ;
#77898=DIRECTION ( 'NONE',  ( 0.000000000000000000, 0.000000000000000000, 1.000000000000000000 ) ) ;
#77903=VECTOR ( 'NONE', #90471, 999.9999999999998863 ) ;
#77907=ORIENTED_EDGE ( 'NONE', *, *, #3089, .F. ) ;
#77908=AXIS2_PLACEMENT_3D ( 'NONE', #58170, #95191, #20189 ) ;
#77915=B_SPLINE_CURVE_WITH_KNOTS ( 'NONE', 3,
 ( #60678, #37702, #89699, #82198, #36716, #90188 ),
 .UNSPECIFIED., .F., .F.,
 ( 4, 2, 4 ),
 ( 8.777993292121407760E-20, 0.0004057005074147807607, 0.0008114010148295614129 ),
 .UNSPECIFIED. ) ;
#77917=CARTESIAN_POINT ( 'NONE',  ( -14.16722289976688565, 0.5000000000000004441, 4.928467845925418089 ) ) ;
#77933=CARTESIAN_POINT ( 'NONE',  ( -3.795296366450322534, -4.237917831752698206, -14.16423886937409904 ) ) ;
#77938=B_SPLINE_CURVE_WITH_KNOTS ( 'NONE', 3,
 ( #15881, #54832, #68388, #91868, #8853, #83872 ),
 .UNSPECIFIED., .F., .F.,
 ( 4, 2, 4 ),
 ( 0.0002800808511900510487, 0.0006862868719403119808, 0.001092492892690572750 ),
 .UNSPECIFIED. ) ;
#77942=CARTESIAN_POINT ( 'NONE',  ( -8.813102413619921194, 15.00000000000000000, -13.34940531570976496 ) ) ;
#77969=DIRECTION ( 'NONE',  ( -0.000000000000000000, -1.000000000000000000, -0.000000000000000000 ) ) ;
#77971=VERTEX_POINT ( 'NONE', #13722 ) ;
#77986=CIRCLE ( 'NONE', #50860, 14.49999999999999822 ) ;
#77987=ORIENTED_EDGE ( 'NONE', *, *, #63911, .F. ) ;
#77988=ORIENTED_EDGE ( 'NONE', *, *, #47583, .T. ) ;
#78003=CARTESIAN_POINT ( 'NONE',  ( 4.923371831947295441, 29.34226448433413381, -8.527530157486179263 ) ) ;
#78012=ADVANCED_FACE ( 'NONE', ( #723 ), #6227, .F. ) ;
#78013=ORIENTED_EDGE ( 'NONE', *, *, #21116, .F. ) ;
#78014=EDGE_CURVE ( 'NONE', #11622, #89199, #14452, .T. ) ;
#78017=ORIENTED_EDGE ( 'NONE', *, *, #46213, .F. ) ;
#78023=ORIENTED_EDGE ( 'NONE', *, *, #96478, .T. ) ;
#78026=FACE_OUTER_BOUND ( 'NONE', #29087, .T. ) ;
#78030=CARTESIAN_POINT ( 'NONE',  ( -13.34343830728408697, 15.00000000000000000, 6.852200678592504701 ) ) ;
#78034=ORIENTED_EDGE ( 'NONE', *, *, #26323, .F. ) ;
#78036=ORIENTED_EDGE ( 'NONE', *, *, #23390, .T. ) ;
#78037=ORIENTED_EDGE ( 'NONE', *, *, #23510, .F. ) ;
#78038=CARTESIAN_POINT ( 'NONE',  ( -11.96291822454885612, 15.00000000000000000, 8.193813980848972278 ) ) ;
#78044=CARTESIAN_POINT ( 'NONE',  ( -4.698669664746476293, 0.000000000000000000, -2.767727949825321332 ) ) ;
#78053=LINE ( 'NONE', #91585, #26597 ) ;
#78060=ORIENTED_EDGE ( 'NONE', *, *, #56567, .T. ) ;
#78071=CARTESIAN_POINT ( 'NONE',  ( -7.964842623401179544, 7.438685344154837509, -7.964842623401174215 ) ) ;
#78073=CARTESIAN_POINT ( 'NONE',  ( 4.838527690343618737, 14.49999999999999822, -14.19819177887726624 ) ) ;
#78075=DIRECTION ( 'NONE',  ( 0.000000000000000000, 1.000000000000000000, 0.000000000000000000 ) ) ;
#78078=DIRECTION ( 'NONE',  ( 0.9588197348681964938, 0.000000000000000000, -0.2840153447039108214 ) ) ;
#78082=LINE ( 'NONE', #25589, #26868 ) ;
#78089=ORIENTED_EDGE ( 'NONE', *, *, #6450, .F. ) ;
#78098=VECTOR ( 'NONE', #84734, 1000.000000000000000 ) ;
#78104=ORIENTED_EDGE ( 'NONE', *, *, #35000, .F. ) ;
#78110=CARTESIAN_POINT ( 'NONE',  ( 3.420591144908545100, 0.5000000000000004441, -14.60477854057955938 ) ) ;
#78117=AXIS2_PLACEMENT_3D ( 'NONE', #49758, #89787, #21303 ) ;
#78118=CARTESIAN_POINT ( 'NONE',  ( 9.846743663894590881, -11.69940218233254114, 2.638427012816828565 ) ) ;
#78120=DIRECTION ( 'NONE',  ( -0.9636304532086248376, 0.000000000000000000, 0.2672383760782501838 ) ) ;
#78129=CARTESIAN_POINT ( 'NONE',  ( 0.000000000000000000, 14.49999999999999822, 0.000000000000000000 ) ) ;
#78133=ADVANCED_FACE ( 'NONE', ( #90699 ), #83705, .F. ) ;
#78138=VERTEX_POINT ( 'NONE', #82709 ) ;
#78145=VECTOR ( 'NONE', #32215, 999.9999999999998863 ) ;
#78146=DIRECTION ( 'NONE',  ( 0.000000000000000000, 1.000000000000000000, 0.000000000000000000 ) ) ;
#78153=CARTESIAN_POINT ( 'NONE',  ( -14.71525861348285957, 0.5000000000000004441, -2.908807992686776700 ) ) ;
#78156=DIRECTION ( 'NONE',  ( -0.000000000000000000, -1.000000000000000000, -0.000000000000000000 ) ) ;
#78157=CARTESIAN_POINT ( 'NONE',  ( 0.000000000000000000, 35.00000000000000000, 0.000000000000000000 ) ) ;
#78170=ORIENTED_EDGE ( 'NONE', *, *, #43319, .T. ) ;
#78176=CARTESIAN_POINT ( 'NONE',  ( -8.564643372776711061, 0.3639308585234187210, 12.31449893000738527 ) ) ;
#78181=CARTESIAN_POINT ( 'NONE',  ( -7.964842623401172439, -36.31131465584515894, 7.964842623401183097 ) ) ;
#78191=ORIENTED_EDGE ( 'NONE', *, *, #8687, .F. ) ;
#78197=LINE ( 'NONE', #9710, #88641 ) ;
#78202=VERTEX_POINT ( 'NONE', #23215 ) ;
#78203=FACE_OUTER_BOUND ( 'NONE', #81495, .T. ) ;
#78213=EDGE_CURVE ( 'NONE', #77529, #97117, #90755, .T. ) ;
#78216=CARTESIAN_POINT ( 'NONE',  ( 9.997910040112596874, 15.00000000000000000, -10.50199004140715253 ) ) ;
#78219=CARTESIAN_POINT ( 'NONE',  ( -1.915564264621232748, 15.00000000000000000, -14.37291249357993372 ) ) ;
#78227=DIRECTION ( 'NONE',  ( 0.000000000000000000, 1.000000000000000000, 0.000000000000000000 ) ) ;
#78245=EDGE_CURVE ( 'NONE', #3849, #85778, #234, .T. ) ;
#78246=CARTESIAN_POINT ( 'NONE',  ( 12.60589901313217354, 14.63595249122788999, 8.129656208642140669 ) ) ;
#78247=CARTESIAN_POINT ( 'NONE',  ( -6.408140936763232709, -5.043031996736238476, 11.09922568453595026 ) ) ;
#78248=EDGE_CURVE ( 'NONE', #16062, #60724, #9659, .T. ) ;
#78251=VERTEX_POINT ( 'NONE', #69198 ) ;
#78253=ORIENTED_EDGE ( 'NONE', *, *, #66277, .F. ) ;
#78261=AXIS2_PLACEMENT_3D ( 'NONE', #93209, #25240, #46729 ) ;
#78262=ORIENTED_EDGE ( 'NONE', *, *, #63333, .F. ) ;
#78265=FACE_OUTER_BOUND ( 'NONE', #9330, .T. ) ;
#78268=DIRECTION ( 'NONE',  ( 0.000000000000000000, 1.000000000000000000, 0.000000000000000000 ) ) ;
#78278=AXIS2_PLACEMENT_3D ( 'NONE', #19849, #50341, #88352 ) ;
#78280=LINE ( 'NONE', #86778, #21601 ) ;
#78289=DIRECTION ( 'NONE',  ( 0.000000000000000000, 1.000000000000000000, 0.000000000000000000 ) ) ;
#78298=CARTESIAN_POINT ( 'NONE',  ( 0.000000000000000000, 0.5000000000000004441, 0.000000000000000000 ) ) ;
#78308=CARTESIAN_POINT ( 'NONE',  ( -6.728956594450893114, 15.00000000000000888, 12.98689685418136186 ) ) ;
#78311=CARTESIAN_POINT ( 'NONE',  ( -8.549892366338680105, 0.2306972965111899199, -12.25305656628366791 ) ) ;
#78317=CARTESIAN_POINT ( 'NONE',  ( -14.24131928502210975, 15.00000000000000000, -0.4973178280107823923 ) ) ;
#78318=CARTESIAN_POINT ( 'NONE',  ( 2.826948239413922703, 14.76930270348881002, -14.67127868811025948 ) ) ;
#78324=DIRECTION ( 'NONE',  ( 0.000000000000000000, 0.000000000000000000, 1.000000000000000000 ) ) ;
#78334=CIRCLE ( 'NONE', #89544, 14.49999999999999822 ) ;
#78340=DIRECTION ( 'NONE',  ( 0.000000000000000000, 1.000000000000000000, 0.000000000000000000 ) ) ;
#78351=VERTEX_POINT ( 'NONE', #94142 ) ;
#78381=CYLINDRICAL_SURFACE ( 'NONE', #86599, 15.00000000000000000 ) ;
#78386=EDGE_CURVE ( 'NONE', #28832, #60175, #93653, .T. ) ;
#78391=CARTESIAN_POINT ( 'NONE',  ( 10.58171042697176567, 14.76984967302771246, -10.54749450092402441 ) ) ;
#78393=CARTESIAN_POINT ( 'NONE',  ( -14.37564666802071578, 15.00000000000000888, -2.692451322017866744 ) ) ;
#78394=CARTESIAN_POINT ( 'NONE',  ( -12.60874940350935169, 15.00000000000000000, -7.160268045227203615 ) ) ;
#78397=CARTESIAN_POINT ( 'NONE',  ( 0.9082943533636174127, 4.777657996272472852E-16, 14.47152380945585648 ) ) ;
#78402=CARTESIAN_POINT ( 'NONE',  ( 13.78891971893208890, 14.63595249122791131, -5.904717858191532720 ) ) ;
#78416=CARTESIAN_POINT ( 'NONE',  ( -2.393480905992977803, 14.49999999999999112, -14.80781041047760382 ) ) ;
#78419=EDGE_LOOP ( 'NONE', ( #85524, #95128, #82567, #23226 ) ) ;
#78421=CARTESIAN_POINT ( 'NONE',  ( 3.836325488036179454, 0.3639308251242922565, -14.50112432709426180 ) ) ;
#78425=CARTESIAN_POINT ( 'NONE',  ( -14.16423886937410437, -13.40458449841936606, -3.795296366450299885 ) ) ;
#78428=ORIENTED_EDGE ( 'NONE', *, *, #42477, .T. ) ;
#78431=DIRECTION ( 'NONE',  ( -0.000000000000000000, -1.000000000000000000, -0.000000000000000000 ) ) ;
#78433=FACE_OUTER_BOUND ( 'NONE', #38186, .T. ) ;
#78449=EDGE_LOOP ( 'NONE', ( #24238, #73652, #93899, #45020, #16013, #12210 ) ) ;
#78450=TOROIDAL_SURFACE ( 'NONE', #35331, 14.49999999999999822, 0.5000000000000000000 ) ;
#78454=DIRECTION ( 'NONE',  ( 0.000000000000000000, 1.000000000000000000, 0.000000000000000000 ) ) ;
#78465=ORIENTED_EDGE ( 'NONE', *, *, #84241, .T. ) ;
#78466=DIRECTION ( 'NONE',  ( 0.000000000000000000, 1.000000000000000000, 0.000000000000000000 ) ) ;
#78467=DIRECTION ( 'NONE',  ( -0.8141155183563146824, 0.000000000000000000, -0.5807029557109462115 ) ) ;
#78475=EDGE_LOOP ( 'NONE', ( #78524, #48157, #55123, #24065 ) ) ;
#78495=EDGE_CURVE ( 'NONE', #94488, #2423, #44164, .T. ) ;
#78498=CARTESIAN_POINT ( 'NONE',  ( -9.846743663894596210, 30.80059781766745530, -2.638427012816824124 ) ) ;
#78499=ORIENTED_EDGE ( 'NONE', *, *, #64028, .T. ) ;
#78509=ORIENTED_EDGE ( 'NONE', *, *, #44284, .T. ) ;
#78512=VERTEX_POINT ( 'NONE', #40666 ) ;
#78515=LINE ( 'NONE', #9529, #65978 ) ;
#78519=EDGE_CURVE ( 'NONE', #4697, #97173, #77640, .T. ) ;
#78521=DIRECTION ( 'NONE',  ( 0.000000000000000000, 0.000000000000000000, 1.000000000000000000 ) ) ;
#78524=ORIENTED_EDGE ( 'NONE', *, *, #73462, .F. ) ;
#78525=B_SPLINE_CURVE_WITH_KNOTS ( 'NONE', 3,
 ( #93229, #70256, #70753, #46748, #32723, #39270 ),
 .UNSPECIFIED., .F., .F.,
 ( 4, 2, 4 ),
 ( 0.0002800138956558747335, 0.0006862192609921059219, 0.001092424626328337110 ),
 .UNSPECIFIED. ) ;
#78530=VERTEX_POINT ( 'NONE', #13105 ) ;
#78531=DIRECTION ( 'NONE',  ( -0.000000000000000000, -1.000000000000000000, -0.000000000000000000 ) ) ;
#78535=EDGE_CURVE ( 'NONE', #8981, #62748, #40061, .T. ) ;
#78537=CARTESIAN_POINT ( 'NONE',  ( 0.000000000000000000, 0.5000000000000004441, 0.000000000000000000 ) ) ;
#78541=ORIENTED_EDGE ( 'NONE', *, *, #89636, .F. ) ;
#78546=CARTESIAN_POINT ( 'NONE',  ( 11.75209714983975395, 0.04922511925147050188, -8.918201205062004533 ) ) ;
#78549=CIRCLE ( 'NONE', #35429, 14.49999999999999822 ) ;
#78552=VERTEX_POINT ( 'NONE', #27116 ) ;
#78556=EDGE_CURVE ( 'NONE', #86906, #58402, #47976, .T. ) ;
#78565=CARTESIAN_POINT ( 'NONE',  ( -7.964842623401179544, -2.561314655845163823, -7.964842623401174215 ) ) ;
#78568=VECTOR ( 'NONE', #96622, 1000.000000000000000 ) ;
#78584=EDGE_LOOP ( 'NONE', ( #23925, #48394, #98610, #53683 ) ) ;
#78594=DIRECTION ( 'NONE',  ( 0.000000000000000000, 0.000000000000000000, 1.000000000000000000 ) ) ;
#78598=EDGE_LOOP ( 'NONE', ( #30200, #26670, #11677, #2048 ) ) ;
#78599=ORIENTED_EDGE ( 'NONE', *, *, #78604, .F. ) ;
#78600=TOROIDAL_SURFACE ( 'NONE', #6725, 14.49999999999999822, 0.5000000000000000000 ) ;
#78604=EDGE_CURVE ( 'NONE', #12737, #28504, #94639, .T. ) ;
#78613=CARTESIAN_POINT ( 'NONE',  ( 12.21238578216011916, 1.931235119739804773E-16, -8.049595036947129856 ) ) ;
#78614=EDGE_CURVE ( 'NONE', #42957, #81191, #96130, .T. ) ;
#78616=CARTESIAN_POINT ( 'NONE',  ( 2.638427012816829897, -10.44940218233254470, -9.846743663894592657 ) ) ;
#78619=CARTESIAN_POINT ( 'NONE',  ( 9.898881779040660689, -0.03417435944610275333, 10.25059215482582786 ) ) ;
#78620=CARTESIAN_POINT ( 'NONE',  ( 0.000000000000000000, 15.00000000000000000, 0.000000000000000000 ) ) ;
#78629=AXIS2_PLACEMENT_3D ( 'NONE', #48743, #79249, #10762 ) ;
#78632=CARTESIAN_POINT ( 'NONE',  ( -9.382169495545422677, 28.49863466993042849, -9.382169495545417348 ) ) ;
#78634=VECTOR ( 'NONE', #70790, 1000.000000000000227 ) ;
#78635=VECTOR ( 'NONE', #64608, 1000.000000000000000 ) ;
#78637=ORIENTED_EDGE ( 'NONE', *, *, #15246, .F. ) ;
#78643=CIRCLE ( 'NONE', #38677, 15.00000000000000000 ) ;
#78646=VECTOR ( 'NONE', #71705, 1000.000000000000114 ) ;
#78651=ORIENTED_EDGE ( 'NONE', *, *, #30810, .T. ) ;
#78669=DIRECTION ( 'NONE',  ( -0.000000000000000000, -1.000000000000000000, -0.000000000000000000 ) ) ;
#78670=AXIS2_PLACEMENT_3D ( 'NONE', #69911, #30415, #60424 ) ;
#78671=ORIENTED_EDGE ( 'NONE', *, *, #22411, .T. ) ;
#78673=DIRECTION ( 'NONE',  ( 0.000000000000000000, 1.000000000000000000, 0.000000000000000000 ) ) ;
#78676=DIRECTION ( 'NONE',  ( -0.9426414910921805390, 0.000000000000000000, 0.3338068592337649076 ) ) ;
#78678=CARTESIAN_POINT ( 'NONE',  ( -14.61046065509105496, 15.00000000000000533, -0.6655452423544750973 ) ) ;
#78681=CARTESIAN_POINT ( 'NONE',  ( -10.88017736071110164, -37.14464798917849464, -2.915334737309917212 ) ) ;
#78698=LINE ( 'NONE', #94178, #19962 ) ;
#78700=ADVANCED_FACE ( 'NONE', ( #12609 ), #58097, .T. ) ;
#78715=DIRECTION ( 'NONE',  ( 0.000000000000000000, 1.000000000000000000, 0.000000000000000000 ) ) ;
#78727=DIRECTION ( 'NONE',  ( 0.000000000000000000, 0.000000000000000000, 1.000000000000000000 ) ) ;
#78730=FACE_OUTER_BOUND ( 'NONE', #1077, .T. ) ;
#78731=DIRECTION ( 'NONE',  ( 0.000000000000000000, 1.000000000000000000, 0.000000000000000000 ) ) ;
#78738=CARTESIAN_POINT ( 'NONE',  ( -14.47650479471825946, 14.63595249122789177, 3.928206833721921587 ) ) ;
#78747=ORIENTED_EDGE ( 'NONE', *, *, #35325, .T. ) ;
#78748=EDGE_CURVE ( 'NONE', #57201, #90159, #3299, .T. ) ;
#78752=CARTESIAN_POINT ( 'NONE',  ( -11.09922568453595382, -1.293031996736242251, -6.408140936763226492 ) ) ;
#78754=ORIENTED_EDGE ( 'NONE', *, *, #10646, .F. ) ;
#78767=AXIS2_PLACEMENT_3D ( 'NONE', #40031, #17540, #48007 ) ;
#78776=TOROIDAL_SURFACE ( 'NONE', #35662, 14.49999999999999822, 0.5000000000000000000 ) ;
#78795=CARTESIAN_POINT ( 'NONE',  ( -5.806645064956620139, 15.00000000000000888, 13.42464971016990205 ) ) ;
#78800=FACE_OUTER_BOUND ( 'NONE', #10405, .T. ) ;
#78803=PLANE ( 'NONE',  #9793 ) ;
#78804=EDGE_LOOP ( 'NONE', ( #62117, #98925, #17664, #47134 ) ) ;
#78807=CARTESIAN_POINT ( 'NONE',  ( -10.19513985507840736, 15.00000000000000000, 11.00268709613209950 ) ) ;
#78811=EDGE_CURVE ( 'NONE', #31048, #64121, #58514, .T. ) ;
#78813=CARTESIAN_POINT ( 'NONE',  ( 0.000000000000000000, 0.5000000000000004441, 0.000000000000000000 ) ) ;
#78818=DIRECTION ( 'NONE',  ( 0.6225146366376078655, 0.000000000000000000, 0.7826081568524232424 ) ) ;
#78823=FACE_OUTER_BOUND ( 'NONE', #36062, .T. ) ;
#78826=CARTESIAN_POINT ( 'NONE',  ( -14.62617646268090432, 0.3640475087720987935, 3.327906561566782884 ) ) ;
#78829=CARTESIAN_POINT ( 'NONE',  ( 0.000000000000000000, 15.00000000000000000, 0.000000000000000000 ) ) ;
#78837=FACE_OUTER_BOUND ( 'NONE', #34582, .T. ) ;
#78846=EDGE_CURVE ( 'NONE', #28832, #74162, #55799, .T. ) ;
#78849=EDGE_LOOP ( 'NONE', ( #50859, #75174, #18236, #6162 ) ) ;
#78851=ORIENTED_EDGE ( 'NONE', *, *, #23514, .F. ) ;
#78852=CARTESIAN_POINT ( 'NONE',  ( 1.780824192092403058, 15.00000000000000000, 14.89391369643514729 ) ) ;
#78857=FACE_OUTER_BOUND ( 'NONE', #22514, .T. ) ;
#78869=DIRECTION ( 'NONE',  ( 0.000000000000000000, 0.000000000000000000, 1.000000000000000000 ) ) ;
#78873=CYLINDRICAL_SURFACE ( 'NONE', #46314, 15.00000000000000000 ) ;
#78877=CARTESIAN_POINT ( 'NONE',  ( 0.000000000000000000, 0.5000000000000004441, 0.000000000000000000 ) ) ;
#78878=ORIENTED_EDGE ( 'NONE', *, *, #73538, .F. ) ;
#78881=ORIENTED_EDGE ( 'NONE', *, *, #35665, .T. ) ;
#78887=CARTESIAN_POINT ( 'NONE',  ( 0.000000000000000000, 0.5000000000000004441, 0.000000000000000000 ) ) ;
#78889=CARTESIAN_POINT ( 'NONE',  ( -14.66148682522520019, 14.76984938411755088, -2.874551585517384211 ) ) ;
#78894=CARTESIAN_POINT ( 'NONE',  ( 3.115783986955464435, 4.832823856176936692E-16, 14.16128137375399731 ) ) ;
#78896=ORIENTED_EDGE ( 'NONE', *, *, #64209, .F. ) ;
#78901=CARTESIAN_POINT ( 'NONE',  ( 12.80781515976310203, 15.00000000000000000, 6.246788841744411513 ) ) ;
#78905=CARTESIAN_POINT ( 'NONE',  ( -12.98685442714204008, 4.660809545892429844E-16, 6.449155920600864178 ) ) ;
#78906=CIRCLE ( 'NONE', #61348, 15.00000000000000000 ) ;
#78912=DIRECTION ( 'NONE',  ( 0.000000000000000000, 1.000000000000000000, 0.000000000000000000 ) ) ;
#78916=CARTESIAN_POINT ( 'NONE',  ( 10.76493118081690881, 15.00000000000000888, -9.902252441915713632 ) ) ;
#78920=CARTESIAN_POINT ( 'NONE',  ( -5.204170427930421283E-15, 10.55374883491398030, -14.16423886937410082 ) ) ;
#78923=ADVANCED_FACE ( 'NONE', ( #29572 ), #15104, .F. ) ;
#78926=CARTESIAN_POINT ( 'NONE',  ( -12.58781651029194393, 15.00000000000000533, -7.446837378630896787 ) ) ;
#78931=EDGE_CURVE ( 'NONE', #34672, #1705, #60697, .T. ) ;
#78943=ORIENTED_EDGE ( 'NONE', *, *, #45890, .F. ) ;
#78953=DIRECTION ( 'NONE',  ( 0.000000000000000000, 0.000000000000000000, 1.000000000000000000 ) ) ;
#78983=DIRECTION ( 'NONE',  ( -0.000000000000000000, 1.000000000000000000, 0.000000000000000000 ) ) ;
#78985=CARTESIAN_POINT ( 'NONE',  ( 6.408140936763236262, -37.54303199673623936, -11.09922568453595026 ) ) ;
#78986=ORIENTED_EDGE ( 'NONE', *, *, #77317, .F. ) ;
#78987=LINE ( 'NONE', #40515, #98929 ) ;
#79001=ORIENTED_EDGE ( 'NONE', *, *, #43710, .F. ) ;
#79003=CARTESIAN_POINT ( 'NONE',  ( 3.469446951953614189E-15, 5.938309369127516391, 11.92686044187656513 ) ) ;
#79012=ORIENTED_EDGE ( 'NONE', *, *, #37290, .T. ) ;
#79016=ORIENTED_EDGE ( 'NONE', *, *, #35822, .T. ) ;
#79017=CYLINDRICAL_SURFACE ( 'NONE', #85777, 15.00000000000000000 ) ;
#79022=DIRECTION ( 'NONE',  ( -0.000000000000000000, -1.000000000000000000, -0.000000000000000000 ) ) ;
#79026=AXIS2_PLACEMENT_3D ( 'NONE', #61955, #17947, #84961 ) ;
#79032=CARTESIAN_POINT ( 'NONE',  ( 10.36894250292378850, -35.07125116508602503, -10.36894250292379027 ) ) ;
#79035=EDGE_CURVE ( 'NONE', #39649, #12953, #12932, .T. ) ;
#79036=B_SPLINE_CURVE_WITH_KNOTS ( 'NONE', 3,
 ( #69356, #68379, #45363, #877, #60857, #14893 ),
 .UNSPECIFIED., .F., .F.,
 ( 4, 2, 4 ),
 ( 0.0002800154274912493714, 0.0006862208078174524429, 0.001092426188143655677 ),
 .UNSPECIFIED. ) ;
#79042=CARTESIAN_POINT ( 'NONE',  ( 11.22915323889580463, 15.00000000000000000, -8.773176023390609757 ) ) ;
#79045=DIRECTION ( 'NONE',  ( 0.000000000000000000, 0.000000000000000000, 1.000000000000000000 ) ) ;
#79048=CARTESIAN_POINT ( 'NONE',  ( 2.915334737309921209, 6.605352010821504471, -10.88017736071110164 ) ) ;
#79054=CYLINDRICAL_SURFACE ( 'NONE', #65544, 15.00000000000000000 ) ;
#79057=CARTESIAN_POINT ( 'NONE',  ( 8.209432707284900488, 14.63606883728627217, -12.55409154915488656 ) ) ;
#79066=EDGE_LOOP ( 'NONE', ( #45284, #19680, #56944, #35334 ) ) ;
#79077=CARTESIAN_POINT ( 'NONE',  ( 13.07734668325342575, 15.00000000000000888, -6.551438809692913701 ) ) ;
#79088=AXIS2_PLACEMENT_3D ( 'NONE', #1251, #91735, #7758 ) ;
#79091=DIRECTION ( 'NONE',  ( 0.000000000000000000, 1.000000000000000000, 0.000000000000000000 ) ) ;
#79095=CARTESIAN_POINT ( 'NONE',  ( -4.850097797903872632, 14.95037102666378281, -13.93319274794287921 ) ) ;
#79098=CARTESIAN_POINT ( 'NONE',  ( -8.527530157486182816, -14.40773551566587685, -4.923371831947288335 ) ) ;
#79110=DIRECTION ( 'NONE',  ( 0.9981347984218662539, 0.000000000000000000, 0.06104853953487057033 ) ) ;
#79111=CARTESIAN_POINT ( 'NONE',  ( -9.399392868737892925, 15.00000000000000000, 11.04089732309468097 ) ) ;
#79112=CIRCLE ( 'NONE', #36001, 15.00000000000000000 ) ;
#79114=CARTESIAN_POINT ( 'NONE',  ( -12.81628187352647963, 28.91530133659709989, -3.434112377981046293 ) ) ;
#79115=ORIENTED_EDGE ( 'NONE', *, *, #48984, .T. ) ;
#79119=ORIENTED_EDGE ( 'NONE', *, *, #78213, .F. ) ;
#79124=EDGE_CURVE ( 'NONE', #8560, #765, #59452, .T. ) ;
#79126=AXIS2_PLACEMENT_3D ( 'NONE', #26166, #69703, #16212 ) ;
#79139=DIRECTION ( 'NONE',  ( 0.000000000000000000, 1.000000000000000000, 0.000000000000000000 ) ) ;
#79142=VERTEX_POINT ( 'NONE', #11534 ) ;
#79145=TOROIDAL_SURFACE ( 'NONE', #64784, 14.49999999999999822, 0.5000000000000000000 ) ;
#79148=LINE ( 'NONE', #87133, #96835 ) ;
#79151=VERTEX_POINT ( 'NONE', #3562 ) ;
#79153=PLANE ( 'NONE',  #74481 ) ;
#79159=CARTESIAN_POINT ( 'NONE',  ( -14.97687855664613465, 14.49999999999999112, -0.8325315005902816923 ) ) ;
#79160=DIRECTION ( 'NONE',  ( -0.06104853953487057033, -0.000000000000000000, 0.9981347984218662539 ) ) ;
#79163=CARTESIAN_POINT ( 'NONE',  ( 12.26659068614894821, 28.88708216824731423, 7.082119434687044190 ) ) ;
#79174=CIRCLE ( 'NONE', #36071, 14.49999999999999822 ) ;
#79175=ORIENTED_EDGE ( 'NONE', *, *, #75848, .F. ) ;
#79182=CARTESIAN_POINT ( 'NONE',  ( 5.419894505350487002, 0.5000000000000004441, 13.98659156302462314 ) ) ;
#79187=VERTEX_POINT ( 'NONE', #50028 ) ;
#79188=DIRECTION ( 'NONE',  ( 0.9426414910921782075, 0.000000000000000000, -0.3338068592337712914 ) ) ;
#79197=DIRECTION ( 'NONE',  ( 0.000000000000000000, 0.000000000000000000, 1.000000000000000000 ) ) ;
#79200=DIRECTION ( 'NONE',  ( 0.9636304532086191754, 0.000000000000000000, 0.2672383760782702788 ) ) ;
#79202=ORIENTED_EDGE ( 'NONE', *, *, #53096, .F. ) ;
#79203=CARTESIAN_POINT ( 'NONE',  ( 13.40508947812163143, 3.998652394537887614E-16, 5.527528931046191474 ) ) ;
#79214=DIRECTION ( 'NONE',  ( -0.9981347984218665870, 0.000000000000000000, -0.06104853953486361756 ) ) ;
#79218=CARTESIAN_POINT ( 'NONE',  ( 13.48255862861920562, 15.00000000000000000, 5.335786055104250636 ) ) ;
#79220=B_SPLINE_CURVE_WITH_KNOTS ( 'NONE', 3,
 ( #56396, #78393, #26865, #78889, #18392, #32394 ),
 .UNSPECIFIED., .F., .F.,
 ( 4, 2, 4 ),
 ( 0.0002800421825936724816, 0.0006862478247299561669, 0.001092453466866239852 ),
 .UNSPECIFIED. ) ;
#79221=DIRECTION ( 'NONE',  ( 0.8949343616020292158, 0.000000000000000000, -0.4461978131098006672 ) ) ;
#79224=VERTEX_POINT ( 'NONE', #87041 ) ;
#79231=CARTESIAN_POINT ( 'NONE',  ( 14.93875075227008864, 0.2301502577613178946, 0.2365588874160677868 ) ) ;
#79232=CARTESIAN_POINT ( 'NONE',  ( 3.434112377981060948, -9.418031996736241140, 12.81628187352647430 ) ) ;
#79236=ORIENTED_EDGE ( 'NONE', *, *, #36474, .T. ) ;
#79243=CARTESIAN_POINT ( 'NONE',  ( 0.000000000000000000, 15.00000000000000000, 0.000000000000000000 ) ) ;
#79247=VECTOR ( 'NONE', #49220, 999.9999999999998863 ) ;
#79248=EDGE_CURVE ( 'NONE', #83600, #92022, #65470, .T. ) ;
#79249=DIRECTION ( 'NONE',  ( 0.000000000000000000, 1.000000000000000000, 0.000000000000000000 ) ) ;
#79250=CARTESIAN_POINT ( 'NONE',  ( 4.494156999534633989, 0.000000000000000000, -3.088748530746214360 ) ) ;
#79255=EDGE_CURVE ( 'NONE', #23745, #15318, #35006, .T. ) ;
#79259=DIRECTION ( 'NONE',  ( -0.000000000000000000, -1.000000000000000000, -0.000000000000000000 ) ) ;
#79263=CARTESIAN_POINT ( 'NONE',  ( 14.82269085861170943, 0.3639308522293639436, 2.299529454047053445 ) ) ;
#79271=VECTOR ( 'NONE', #29429, 1000.000000000000114 ) ;
#79282=EDGE_CURVE ( 'NONE', #74987, #25279, #61939, .T. ) ;
#79292=DIRECTION ( 'NONE',  ( 0.000000000000000000, 1.000000000000000000, 0.000000000000000000 ) ) ;
#79296=ORIENTED_EDGE ( 'NONE', *, *, #21596, .T. ) ;
#79299=DIRECTION ( 'NONE',  ( 0.000000000000000000, 0.000000000000000000, 1.000000000000000000 ) ) ;
#79309=DIRECTION ( 'NONE',  ( 0.000000000000000000, 0.000000000000000000, 1.000000000000000000 ) ) ;
#79310=DIRECTION ( 'NONE',  ( 0.000000000000000000, 1.000000000000000000, 0.000000000000000000 ) ) ;
#79315=CARTESIAN_POINT ( 'NONE',  ( -7.640917710488839276, 0.04922511925147159823, -12.61992379908765649 ) ) ;
#79317=CARTESIAN_POINT ( 'NONE',  ( -14.62617646268089899, 0.5000000000000004441, 3.327906561566782440 ) ) ;
#79319=CARTESIAN_POINT ( 'NONE',  ( 0.000000000000000000, 14.49999999999999822, 0.000000000000000000 ) ) ;
#79331=CIRCLE ( 'NONE', #76187, 15.00000000000000000 ) ;
#79332=CYLINDRICAL_SURFACE ( 'NONE', #55038, 15.00000000000000000 ) ;
#79342=ORIENTED_EDGE ( 'NONE', *, *, #54750, .T. ) ;
#79344=LINE ( 'NONE', #3350, #69710 ) ;
#79345=AXIS2_PLACEMENT_3D ( 'NONE', #32916, #93921, #40441 ) ;
#79348=AXIS2_PLACEMENT_3D ( 'NONE', #25124, #63577, #18585 ) ;
#79361=ORIENTED_EDGE ( 'NONE', *, *, #492, .F. ) ;
#79366=DIRECTION ( 'NONE',  ( 0.000000000000000000, 1.000000000000000000, 0.000000000000000000 ) ) ;
#79372=CARTESIAN_POINT ( 'NONE',  ( 0.000000000000000000, 15.00000000000000000, 0.000000000000000000 ) ) ;
#79373=ORIENTED_EDGE ( 'NONE', *, *, #1622, .F. ) ;
#79376=EDGE_CURVE ( 'NONE', #73812, #22448, #14137, .T. ) ;
#79378=ORIENTED_EDGE ( 'NONE', *, *, #28407, .F. ) ;
#79384=CARTESIAN_POINT ( 'NONE',  ( 14.35840480524199947, 0.5000000000000004441, -4.340070442838851683 ) ) ;
#79385=CARTESIAN_POINT ( 'NONE',  ( -13.07964015051215156, 14.76930270348881180, -7.222261988160926016 ) ) ;
#79388=DIRECTION ( 'NONE',  ( 0.000000000000000000, 0.000000000000000000, 1.000000000000000000 ) ) ;
#79395=ADVANCED_FACE ( 'NONE', ( #28510 ), #30466, .F. ) ;
#79396=CARTESIAN_POINT ( 'NONE',  ( -13.75543905097471153, 14.95037102630581316, 5.333404663735480611 ) ) ;
#79405=EDGE_CURVE ( 'NONE', #2722, #21313, #52974, .T. ) ;
#79411=CARTESIAN_POINT ( 'NONE',  ( 2.962741594152983993, -0.03417435944610275333, 13.93860331045674883 ) ) ;
#79414=AXIS2_PLACEMENT_3D ( 'NONE', #63500, #65454, #41514 ) ;
#79417=CARTESIAN_POINT ( 'NONE',  ( 10.70613742633256926, 15.00000000000000000, -9.778988772285213571 ) ) ;
#79421=CARTESIAN_POINT ( 'NONE',  ( -3.795296366450322534, 0.7620821682473031267, -14.16423886937409904 ) ) ;
#79424=CARTESIAN_POINT ( 'NONE',  ( -15.67879934938584263, 15.00000000000000000, 3.170591017105712339 ) ) ;
#79425=VERTEX_POINT ( 'NONE', #14012 ) ;
#79427=CARTESIAN_POINT ( 'NONE',  ( 14.35840480524199947, 15.00000000000000000, -4.340070442838851683 ) ) ;
#79434=DIRECTION ( 'NONE',  ( -0.000000000000000000, -1.000000000000000000, -0.000000000000000000 ) ) ;
#79440=DIRECTION ( 'NONE',  ( -0.000000000000000000, -1.000000000000000000, -0.000000000000000000 ) ) ;
#79462=ORIENTED_EDGE ( 'NONE', *, *, #46641, .T. ) ;
#79464=ADVANCED_FACE ( 'NONE', ( #98522 ), #40139, .T. ) ;
#79467=CIRCLE ( 'NONE', #26773, 15.00000000000000000 ) ;
#79468=ORIENTED_EDGE ( 'NONE', *, *, #45855, .T. ) ;
#79469=CARTESIAN_POINT ( 'NONE',  ( 12.87930560075669284, 0.04962897030442307150, 7.195887444332472072 ) ) ;
#79472=CARTESIAN_POINT ( 'NONE',  ( 0.000000000000000000, 15.00000000000000000, 0.000000000000000000 ) ) ;
#79483=CARTESIAN_POINT ( 'NONE',  ( -6.408140936763232709, -30.04303199673624292, 11.09922568453595026 ) ) ;
#79495=ADVANCED_FACE ( 'NONE', ( #60480 ), #92797, .T. ) ;
#79497=ORIENTED_EDGE ( 'NONE', *, *, #32039, .F. ) ;
#79502=ORIENTED_EDGE ( 'NONE', *, *, #30600, .T. ) ;
#79511=ORIENTED_EDGE ( 'NONE', *, *, #53761, .F. ) ;
#79514=ORIENTED_EDGE ( 'NONE', *, *, #8485, .F. ) ;
#79516=DIRECTION ( 'NONE',  ( -0.4305110968082861977, 0.000000000000000000, -0.9025852843498647360 ) ) ;
#79517=EDGE_CURVE ( 'NONE', #39559, #38526, #67998, .T. ) ;
#79524=FACE_OUTER_BOUND ( 'NONE', #85035, .T. ) ;
#79536=CARTESIAN_POINT ( 'NONE',  ( -14.16423886937410437, -33.40458449841936783, -3.795296366450299885 ) ) ;
#79554=CARTESIAN_POINT ( 'NONE',  ( 7.964842623401177768, 11.18868534415484106, -7.964842623401181321 ) ) ;
#79558=DIRECTION ( 'NONE',  ( -0.000000000000000000, -1.000000000000000000, -0.000000000000000000 ) ) ;
#79559=CARTESIAN_POINT ( 'NONE',  ( 0.9940297508537879745, -0.03417435944610275333, -14.21528771620249820 ) ) ;
#79560=VECTOR ( 'NONE', #17019, 1000.000000000000114 ) ;
#79563=FACE_OUTER_BOUND ( 'NONE', #33494, .T. ) ;
#79564=B_SPLINE_CURVE_WITH_KNOTS ( 'NONE', 3,
 ( #60440, #949, #75941, #16432, #61913, #14969 ),
 .UNSPECIFIED., .F., .F.,
 ( 4, 2, 4 ),
 ( 3.409110551496115783E-05, 0.0004400426677367857043, 0.0008459942299586101829 ),
 .UNSPECIFIED. ) ;
#79565=CYLINDRICAL_SURFACE ( 'NONE', #12463, 15.00000000000000000 ) ;
#79581=CARTESIAN_POINT ( 'NONE',  ( 13.34343830728404967, 14.63595249122789177, -6.852200678592606842 ) ) ;
#79584=ADVANCED_FACE ( 'NONE', ( #52007 ), #32121, .T. ) ;
#79586=DIRECTION ( 'NONE',  ( 0.000000000000000000, 0.000000000000000000, 1.000000000000000000 ) ) ;
#79598=CARTESIAN_POINT ( 'NONE',  ( 4.923371831947295441, -0.6577355156658776236, -8.527530157486179263 ) ) ;
#79599=EDGE_LOOP ( 'NONE', ( #55636, #73967, #22807, #23787, #21269, #43082 ) ) ;
#79600=DIRECTION ( 'NONE',  ( -0.4771587602596037980, 0.000000000000000000, -0.8788171126619679363 ) ) ;
#79607=LINE ( 'NONE', #26592, #13570 ) ;
#79608=CARTESIAN_POINT ( 'NONE',  ( -14.17193700899788134, 0.000000000000000000, -1.489530601564206247 ) ) ;
#79610=EDGE_CURVE ( 'NONE', #54489, #36938, #83488, .T. ) ;
#79612=VERTEX_POINT ( 'NONE', #15007 ) ;
#79623=CIRCLE ( 'NONE', #82825, 15.00000000000000000 ) ;
#79624=CIRCLE ( 'NONE', #3001, 15.00000000000000000 ) ;
#79627=VERTEX_POINT ( 'NONE', #45477 ) ;
#79632=ADVANCED_FACE ( 'NONE', ( #75979 ), #7508, .T. ) ;
#79634=AXIS2_PLACEMENT_3D ( 'NONE', #14214, #67205, #51713 ) ;
#79638=CARTESIAN_POINT ( 'NONE',  ( -0.1034006766821534140, 4.816303916663454299E-16, 14.49963131600461175 ) ) ;
#79645=EDGE_CURVE ( 'NONE', #29027, #189, #68491, .T. ) ;
#79652=DIRECTION ( 'NONE',  ( 0.09584575252022037306, 0.000000000000000000, 0.9953961983671790748 ) ) ;
#79655=CARTESIAN_POINT ( 'NONE',  ( 9.128857603258678566, 12.89891393428310806, -7.267056389305773578 ) ) ;
#79659=CARTESIAN_POINT ( 'NONE',  ( -11.62719953690051788, 0.5000000000000004441, -9.476720473301954328 ) ) ;
#79663=CARTESIAN_POINT ( 'NONE',  ( 9.422509992056141925, -19.85298132251182324, 5.440088680355547268 ) ) ;
#79678=CARTESIAN_POINT ( 'NONE',  ( 14.64921366071501119, 14.95037108083552368, 1.748670679918272741 ) ) ;
#79682=ORIENTED_EDGE ( 'NONE', *, *, #13155, .F. ) ;
#79695=VERTEX_POINT ( 'NONE', #31935 ) ;
#79699=ORIENTED_EDGE ( 'NONE', *, *, #72813, .T. ) ;
#79705=DIRECTION ( 'NONE',  ( -0.7009092642998475675, 0.000000000000000000, -0.7132504491541847846 ) ) ;
#79710=DIRECTION ( 'NONE',  ( 3.197442310920451468E-14, 0.000000000000000000, 1.000000000000000000 ) ) ;
#79711=CARTESIAN_POINT ( 'NONE',  ( 0.7375392941518293943, 14.49999999999999822, -14.98185688723470932 ) ) ;
#79714=CARTESIAN_POINT ( 'NONE',  ( -9.846743663894590881, -33.78273551566586974, 2.638427012816840111 ) ) ;
#79715=ORIENTED_EDGE ( 'NONE', *, *, #81754, .F. ) ;
#79719=VERTEX_POINT ( 'NONE', #31449 ) ;
#79724=CARTESIAN_POINT ( 'NONE',  ( 14.71525861348287734, 0.5000000000000004441, 2.908807992686682109 ) ) ;
#79728=CARTESIAN_POINT ( 'NONE',  ( 11.09922568453595026, -8.793031996736241140, 6.408140936763232709 ) ) ;
#79739=DIRECTION ( 'NONE',  ( -0.000000000000000000, -1.000000000000000000, -0.000000000000000000 ) ) ;
#79744=FACE_OUTER_BOUND ( 'NONE', #96619, .T. ) ;
#79746=CARTESIAN_POINT ( 'NONE',  ( 14.02068044289375415, 0.5000000000000004441, 5.331089937175756965 ) ) ;
#79755=LINE ( 'NONE', #42256, #94754 ) ;
#79758=B_SPLINE_CURVE_WITH_KNOTS ( 'NONE', 3,
 ( #89213, #58199, #19240, #48745, #88715, #3763 ),
 .UNSPECIFIED., .F., .F.,
 ( 4, 2, 4 ),
 ( 3.409110551493088148E-05, 0.0004400426677367781148, 0.0008459942299586253617 ),
 .UNSPECIFIED. ) ;
#79762=EDGE_CURVE ( 'NONE', #9609, #41967, #70955, .T. ) ;
#79780=CARTESIAN_POINT ( 'NONE',  ( 13.82671409943293739, 0.000000000000000000, 3.447387012295318076 ) ) ;
#79782=CARTESIAN_POINT ( 'NONE',  ( 0.000000000000000000, 14.49999999999999822, 0.000000000000000000 ) ) ;
#79797=CARTESIAN_POINT ( 'NONE',  ( -12.67122524790580762, 0.04922511925147277784, -7.555537761805941166 ) ) ;
#79803=FACE_OUTER_BOUND ( 'NONE', #84071, .T. ) ;
#79805=DIRECTION ( 'NONE',  ( 0.000000000000000000, 0.000000000000000000, 1.000000000000000000 ) ) ;
#79806=DIRECTION ( 'NONE',  ( 0.000000000000000000, 0.000000000000000000, 1.000000000000000000 ) ) ;
#79811=CARTESIAN_POINT ( 'NONE',  ( 0.000000000000000000, 0.5000000000000004441, 0.000000000000000000 ) ) ;
#79832=ORIENTED_EDGE ( 'NONE', *, *, #70598, .T. ) ;
#79834=LINE ( 'NONE', #19339, #43592 ) ;
#79842=ORIENTED_EDGE ( 'NONE', *, *, #65694, .T. ) ;
#79847=CARTESIAN_POINT ( 'NONE',  ( -10.27090289957521207, -3.117928278843078365E-15, -10.41235154178118805 ) ) ;
#79854=CIRCLE ( 'NONE', #36688, 14.49999999999999822 ) ;
#79872=CARTESIAN_POINT ( 'NONE',  ( 13.55255535720591986, -0.03417435944610275333, 4.403492169843056914 ) ) ;
#79877=VERTEX_POINT ( 'NONE', #33897 ) ;
#79880=CARTESIAN_POINT ( 'NONE',  ( -13.61802159414306423, 15.00000000000000533, 5.334603887713395665 ) ) ;
#79889=DIRECTION ( 'NONE',  ( -0.5664062369248259454, 0.000000000000000000, -0.8241261886220204724 ) ) ;
#79899=CARTESIAN_POINT ( 'NONE',  ( -0.3093388210927642268, 0.5000000000000004441, 14.99680997725065978 ) ) ;
#79900=ORIENTED_EDGE ( 'NONE', *, *, #2514, .F. ) ;
#79903=CARTESIAN_POINT ( 'NONE',  ( -10.93781366033334557, 14.63606902047462199, -10.26470809774084181 ) ) ;
#79912=LINE ( 'NONE', #49908, #45836 ) ;
#79915=CARTESIAN_POINT ( 'NONE',  ( 14.49440716394870954, 15.00000000000000000, 0.4026921475167317688 ) ) ;
#79922=EDGE_CURVE ( 'NONE', #59678, #54738, #75057, .T. ) ;
#79926=EDGE_CURVE ( 'NONE', #58432, #44471, #72893, .T. ) ;
#79929=EDGE_CURVE ( 'NONE', #17551, #56358, #72551, .T. ) ;
#79933=DIRECTION ( 'NONE',  ( 0.000000000000000000, 0.000000000000000000, -1.000000000000000000 ) ) ;
#79934=ORIENTED_EDGE ( 'NONE', *, *, #44715, .F. ) ;
#79942=AXIS2_PLACEMENT_3D ( 'NONE', #93069, #8112, #24103 ) ;
#79944=ORIENTED_EDGE ( 'NONE', *, *, #29563, .T. ) ;
#79945=B_SPLINE_CURVE_WITH_KNOTS ( 'NONE', 3,
 ( #67837, #14848, #37839, #60322, #76798, #31291 ),
 .UNSPECIFIED., .F., .F.,
 ( 4, 2, 4 ),
 ( 3.409110551333654864E-05, 0.0004400426677351659062, 0.0008459942299569952638 ),
 .UNSPECIFIED. ) ;
#79946=TOROIDAL_SURFACE ( 'NONE', #8162, 14.49999999999999822, 0.5000000000000000000 ) ;
#79950=ORIENTED_EDGE ( 'NONE', *, *, #80162, .T. ) ;
#79964=EDGE_CURVE ( 'NONE', #46643, #60588, #26906, .T. ) ;
#79966=CARTESIAN_POINT ( 'NONE',  ( 3.434112377981060948, -34.41803199673624647, 12.81628187352647430 ) ) ;
#79975=CARTESIAN_POINT ( 'NONE',  ( 14.16722289976686966, 14.49999999999999112, 4.928467845925658786 ) ) ;
#79976=EDGE_CURVE ( 'NONE', #28751, #46643, #15400, .T. ) ;
#79979=EDGE_LOOP ( 'NONE', ( #36473, #81567, #18371, #64686 ) ) ;
#79985=ORIENTED_EDGE ( 'NONE', *, *, #17637, .F. ) ;
#79995=EDGE_LOOP ( 'NONE', ( #79462, #38591, #75138, #53256 ) ) ;
#79997=ORIENTED_EDGE ( 'NONE', *, *, #66199, .F. ) ;
#80000=CARTESIAN_POINT ( 'NONE',  ( 14.67697702673042848, 15.00000000000000000, -6.361111679013412790 ) ) ;
#80007=ORIENTED_EDGE ( 'NONE', *, *, #68311, .F. ) ;
#80016=FACE_OUTER_BOUND ( 'NONE', #65940, .T. ) ;
#80018=CARTESIAN_POINT ( 'NONE',  ( 7.082119434687054849, -36.52958449841936783, 12.26659068614894288 ) ) ;
#80022=ORIENTED_EDGE ( 'NONE', *, *, #70069, .T. ) ;
#80034=CARTESIAN_POINT ( 'NONE',  ( 3.469446951953614189E-15, 14.31368534415484284, 10.88017736071110342 ) ) ;
#80040=VECTOR ( 'NONE', #96658, 1000.000000000000114 ) ;
#80042=LINE ( 'NONE', #28021, #63231 ) ;
#80043=EDGE_CURVE ( 'NONE', #45188, #55250, #23401, .T. ) ;
#80056=CARTESIAN_POINT ( 'NONE',  ( 11.12471383767606525, 12.50000000000035527, 1.674288514511126591 ) ) ;
#80063=CARTESIAN_POINT ( 'NONE',  ( 0.000000000000000000, 15.00000000000000000, 0.000000000000000000 ) ) ;
#80065=B_SPLINE_CURVE_WITH_KNOTS ( 'NONE', 3,
 ( #26686, #41717, #56699, #18713, #49675, #72186 ),
 .UNSPECIFIED., .F., .F.,
 ( 4, 2, 4 ),
 ( 0.0002800858945027856570, 0.0006862919646584887288, 0.001092498034814191801 ),
 .UNSPECIFIED. ) ;
#80066=CIRCLE ( 'NONE', #67516, 15.00000000000000000 ) ;
#80073=DIRECTION ( 'NONE',  ( 0.6087614290087186575, 0.000000000000000000, 0.7933533402912366084 ) ) ;
#80074=FACE_OUTER_BOUND ( 'NONE', #41734, .T. ) ;
#80078=DIRECTION ( 'NONE',  ( -0.5519369853120617009, 0.000000000000000000, 0.8338858220671657717 ) ) ;
#80081=CARTESIAN_POINT ( 'NONE',  ( 4.923371831947301658, 7.675597817667460632, 8.527530157486175710 ) ) ;
#80097=VERTEX_POINT ( 'NONE', #16952 ) ;
#80103=DIRECTION ( 'NONE',  ( -0.4305110968082862533, 0.000000000000000000, -0.9025852843498647360 ) ) ;
#80114=FACE_OUTER_BOUND ( 'NONE', #19092, .T. ) ;
#80121=ORIENTED_EDGE ( 'NONE', *, *, #64138, .F. ) ;
#80122=CARTESIAN_POINT ( 'NONE',  ( 0.000000000000000000, 15.00000000000000000, 0.000000000000000000 ) ) ;
#80128=CARTESIAN_POINT ( 'NONE',  ( 11.62719953690061558, 14.49999999999999112, 9.476720473301933012 ) ) ;
#80138=CARTESIAN_POINT ( 'NONE',  ( 8.265815358934768042, 12.95537237636708916, -8.294953093294440194 ) ) ;
#80144=CARTESIAN_POINT ( 'NONE',  ( 10.88017736071110519, -24.43631465584515539, -2.602085213965210642E-15 ) ) ;
#80162=EDGE_CURVE ( 'NONE', #68316, #21109, #18425, .T. ) ;
#80175=CARTESIAN_POINT ( 'NONE',  ( 3.753761956877525119, 0.000000000000000000, -3.955639745193192169 ) ) ;
#80178=ORIENTED_EDGE ( 'NONE', *, *, #26045, .F. ) ;
#80194=AXIS2_PLACEMENT_3D ( 'NONE', #95625, #18647, #41167 ) ;
#80195=FACE_OUTER_BOUND ( 'NONE', #54256, .T. ) ;
#80196=AXIS2_PLACEMENT_3D ( 'NONE', #80575, #12071, #30021 ) ;
#80198=ADVANCED_FACE ( 'NONE', ( #70447 ), #1964, .F. ) ;
#80201=AXIS2_PLACEMENT_3D ( 'NONE', #51381, #81868, #73878 ) ;
#80202=ORIENTED_EDGE ( 'NONE', *, *, #31726, .F. ) ;
#80212=CARTESIAN_POINT ( 'NONE',  ( -9.382169495545413795, 9.748634669930417829, 9.382169495545428006 ) ) ;
#80213=ORIENTED_EDGE ( 'NONE', *, *, #91022, .T. ) ;
#80216=ORIENTED_EDGE ( 'NONE', *, *, #43799, .T. ) ;
#80217=ORIENTED_EDGE ( 'NONE', *, *, #45864, .T. ) ;
#80234=CARTESIAN_POINT ( 'NONE',  ( 3.270119481323678468, 0.04922511925147240314, -14.38584091150421607 ) ) ;
#80236=CARTESIAN_POINT ( 'NONE',  ( -11.10136736363541488, 0.04922511925147367295, 9.716261771424836269 ) ) ;
#80248=ADVANCED_FACE ( 'NONE', ( #20395 ), #76882, .T. ) ;
#80257=LINE ( 'NONE', #89724, #40965 ) ;
#80261=CARTESIAN_POINT ( 'NONE',  ( 0.000000000000000000, 15.00000000000000000, 0.000000000000000000 ) ) ;
#80267=B_SPLINE_CURVE_WITH_KNOTS ( 'NONE', 3,
 ( #68239, #38231, #61208, #54191, #84225, #1230 ),
 .UNSPECIFIED., .F., .F.,
 ( 4, 2, 4 ),
 ( 0.0002800032591452402829, 0.0006862085204419963568, 0.001092413781738752485 ),
 .UNSPECIFIED. ) ;
#80269=TOROIDAL_SURFACE ( 'NONE', #11608, 14.49999999999999822, 0.5000000000000000000 ) ;
#80276=CARTESIAN_POINT ( 'NONE',  ( 11.49658347684016491, 14.95037108522383384, 9.245857368719866187 ) ) ;
#80278=EDGE_CURVE ( 'NONE', #74063, #47699, #38065, .T. ) ;
#80288=EDGE_CURVE ( 'NONE', #9175, #18711, #52386, .T. ) ;
#80289=ORIENTED_EDGE ( 'NONE', *, *, #49771, .T. ) ;
#80290=DIRECTION ( 'NONE',  ( 0.8338858220671735433, 0.000000000000000000, -0.5519369853120501546 ) ) ;
#80296=LINE ( 'NONE', #4311, #35150 ) ;
#80324=DIRECTION ( 'NONE',  ( 0.6626200482157461602, 0.000000000000000000, -0.7489557207889945278 ) ) ;
#80325=DIRECTION ( 'NONE',  ( 0.000000000000000000, 0.000000000000000000, -1.000000000000000000 ) ) ;
#80326=EDGE_CURVE ( 'NONE', #27971, #48509, #86913, .T. ) ;
#80329=VERTEX_POINT ( 'NONE', #58870 ) ;
#80332=CARTESIAN_POINT ( 'NONE',  ( 13.61464873478166737, 15.00000000000000000, -6.296136897217838424 ) ) ;
#80337=TOROIDAL_SURFACE ( 'NONE', #37242, 14.49999999999999822, 0.5000000000000000000 ) ;
#80341=EDGE_LOOP ( 'NONE', ( #69976, #31489, #31640, #19064 ) ) ;
#80355=LINE ( 'NONE', #82314, #53111 ) ;
#80361=CARTESIAN_POINT ( 'NONE',  ( -7.674335239599376912, 14.76930270348882068, 12.81961907869210648 ) ) ;
#80362=CARTESIAN_POINT ( 'NONE',  ( 0.000000000000000000, 14.49999999999999822, 0.000000000000000000 ) ) ;
#80364=CARTESIAN_POINT ( 'NONE',  ( 10.27090289957528135, -3.182726299308032341E-15, 10.41235154178112055 ) ) ;
#80368=DIRECTION ( 'NONE',  ( 0.9999619230641713097, 0.000000000000000000, 0.008726535498374267744 ) ) ;
#80369=DIRECTION ( 'NONE',  ( 0.8870108331782150524, 0.000000000000000000, 0.4617486132350466788 ) ) ;
#80370=TOROIDAL_SURFACE ( 'NONE', #37286, 14.49999999999999822, 0.5000000000000000000 ) ;
#80380=EDGE_CURVE ( 'NONE', #50878, #51412, #22891, .T. ) ;
#80398=CARTESIAN_POINT ( 'NONE',  ( -0.3998276802501956606, 15.00000000000000000, -15.99117050944549234 ) ) ;
#80400=CARTESIAN_POINT ( 'NONE',  ( 14.97687855664611867, 14.63606903414041227, 0.8325315005901734455 ) ) ;
#80402=ADVANCED_FACE ( 'NONE', ( #41346 ), #85343, .T. ) ;
#80407=CYLINDRICAL_SURFACE ( 'NONE', #10547, 15.00000000000000000 ) ;
#80419=DIRECTION ( 'NONE',  ( 0.9426414910921736556, 0.000000000000000000, 0.3338068592337842255 ) ) ;
#80422=DIRECTION ( 'NONE',  ( -0.000000000000000000, 1.000000000000000000, -0.000000000000000000 ) ) ;
#80423=CARTESIAN_POINT ( 'NONE',  ( 12.58781651029204163, -3.396178602016116026E-15, -7.446837378630719151 ) ) ;
#80427=CARTESIAN_POINT ( 'NONE',  ( 13.82671409943296226, 0.000000000000000000, -3.447387012295225261 ) ) ;
#80438=LINE ( 'NONE', #64914, #22974 ) ;
#80450=DIRECTION ( 'NONE',  ( -6.217248937900876626E-14, 0.000000000000000000, 1.000000000000000000 ) ) ;
#80457=CYLINDRICAL_SURFACE ( 'NONE', #65165, 15.00000000000000000 ) ;
#80461=CARTESIAN_POINT ( 'NONE',  ( 0.000000000000000000, 14.49999999999999822, 0.000000000000000000 ) ) ;
#80465=CARTESIAN_POINT ( 'NONE',  ( 12.81628187352647608, -33.37636533006957507, -2.602085213965210642E-15 ) ) ;
#80476=VECTOR ( 'NONE', #42202, 1000.000000000000114 ) ;
#80486=CARTESIAN_POINT ( 'NONE',  ( -12.34557190004687044, 0.04922511925147153578, 8.076692058882407821 ) ) ;
#80496=ORIENTED_EDGE ( 'NONE', *, *, #72367, .T. ) ;
#80497=EDGE_CURVE ( 'NONE', #23460, #37318, #39107, .T. ) ;
#80498=CARTESIAN_POINT ( 'NONE',  ( 0.000000000000000000, 14.49999999999999822, 0.000000000000000000 ) ) ;
#80501=ORIENTED_EDGE ( 'NONE', *, *, #23207, .F. ) ;
#80511=ORIENTED_EDGE ( 'NONE', *, *, #49332, .F. ) ;
#80521=CARTESIAN_POINT ( 'NONE',  ( -3.795296366450322534, -29.23791783175269288, -14.16423886937409904 ) ) ;
#80535=CARTESIAN_POINT ( 'NONE',  ( -10.88017736071110342, 13.06368534415484817, 3.903127820947815962E-15 ) ) ;
#80554=VECTOR ( 'NONE', #86563, 1000.000000000000000 ) ;
#80555=B_SPLINE_CURVE_WITH_KNOTS ( 'NONE', 3,
 ( #48217, #69267, #71232, #33211, #63705, #23283 ),
 .UNSPECIFIED., .F., .F.,
 ( 4, 2, 4 ),
 ( 3.409110551496104263E-05, 0.0004400426677367865174, 0.0008459942299586119176 ),
 .UNSPECIFIED. ) ;
#80558=CARTESIAN_POINT ( 'NONE',  ( 0.000000000000000000, 15.00000000000000000, 0.000000000000000000 ) ) ;
#80564=DIRECTION ( 'NONE',  ( 0.000000000000000000, 1.000000000000000000, 0.000000000000000000 ) ) ;
#80568=ORIENTED_EDGE ( 'NONE', *, *, #10179, .T. ) ;
#80575=CARTESIAN_POINT ( 'NONE',  ( 0.000000000000000000, 0.000000000000000000, 0.000000000000000000 ) ) ;
#80578=CARTESIAN_POINT ( 'NONE',  ( 10.04755927614752942, -3.129363223631011419E-15, -10.62803196998856592 ) ) ;
#80580=CARTESIAN_POINT ( 'NONE',  ( 9.846743663894590881, -1.282735515665884174, -2.638427012816833894 ) ) ;
#80585=CARTESIAN_POINT ( 'NONE',  ( 0.000000000000000000, 15.00000000000000000, 0.000000000000000000 ) ) ;
#80586=ORIENTED_EDGE ( 'NONE', *, *, #63911, .T. ) ;
#80596=ORIENTED_EDGE ( 'NONE', *, *, #20438, .T. ) ;
#80599=VERTEX_POINT ( 'NONE', #42799 ) ;
#80605=CIRCLE ( 'NONE', #79026, 15.00000000000000000 ) ;
#80608=CARTESIAN_POINT ( 'NONE',  ( -6.336100170401012477, 14.76984879808201434, 13.53056138701883881 ) ) ;
#80610=ORIENTED_EDGE ( 'NONE', *, *, #58802, .T. ) ;
#80612=B_SPLINE_CURVE_WITH_KNOTS ( 'NONE', 3,
 ( #6873, #76833, #22380, #38362, #22874, #7867 ),
 .UNSPECIFIED., .F., .F.,
 ( 4, 2, 4 ),
 ( 0.0002800760588349135915, 0.0006862820326511982327, 0.001092488006467482982 ),
 .UNSPECIFIED. ) ;
#80617=CARTESIAN_POINT ( 'NONE',  ( 14.15369600240091330, 15.00000000000000888, -3.689340892730248012 ) ) ;
#80620=ORIENTED_EDGE ( 'NONE', *, *, #70198, .F. ) ;
#80621=CARTESIAN_POINT ( 'NONE',  ( -1.236172813752151045, 14.95077488074853811, -14.70095156538448755 ) ) ;
#80641=PLANE ( 'NONE',  #60909 ) ;
#80644=DIRECTION ( 'NONE',  ( -0.8526401643540953978, 0.000000000000000000, 0.5224985647159435809 ) ) ;
#80645=DIRECTION ( 'NONE',  ( 0.000000000000000000, 0.000000000000000000, 1.000000000000000000 ) ) ;
#80649=CARTESIAN_POINT ( 'NONE',  ( 5.440088680355549045, -28.60298132251182679, -9.422509992056141925 ) ) ;
#80653=FACE_OUTER_BOUND ( 'NONE', #95200, .T. ) ;
#80656=CARTESIAN_POINT ( 'NONE',  ( 10.58981376305282041, 0.000000000000000000, 9.535111140613782510 ) ) ;
#80659=B_SPLINE_CURVE_WITH_KNOTS ( 'NONE', 3,
 ( #35729, #6228, #96249, #59707, #14228, #60205 ),
 .UNSPECIFIED., .F., .F.,
 ( 4, 2, 4 ),
 ( 0.0002800392683685237944, 0.0006862448819815547638, 0.001092450495594585571 ),
 .UNSPECIFIED. ) ;
#80663=CARTESIAN_POINT ( 'NONE',  ( -7.551349515323020789, -0.03417435944610275333, -12.08468537022916323 ) ) ;
#80667=ORIENTED_EDGE ( 'NONE', *, *, #22728, .F. ) ;
#80676=DIRECTION ( 'NONE',  ( 0.000000000000000000, 0.000000000000000000, 1.000000000000000000 ) ) ;
#80680=EDGE_LOOP ( 'NONE', ( #36877, #30726, #76062, #88741 ) ) ;
#80681=ORIENTED_EDGE ( 'NONE', *, *, #83069, .F. ) ;
#80694=AXIS2_PLACEMENT_3D ( 'NONE', #56397, #17424, #41415 ) ;
#80698=CARTESIAN_POINT ( 'NONE',  ( 9.846743663894594434, -36.49106884899921255, -2.168404344971008868E-15 ) ) ;
#80706=ADVANCED_FACE ( 'NONE', ( #48220 ), #85745, .F. ) ;
#80707=DIRECTION ( 'NONE',  ( -0.8788171126619616080, 0.000000000000000000, -0.4771587602596153999 ) ) ;
#80709=MECHANICAL_DESIGN_GEOMETRIC_PRESENTATION_REPRESENTATION('',(#865),#37608);
#80711=CARTESIAN_POINT ( 'NONE',  ( -12.81628187352647963, 3.915301336597085680, -3.434112377981046293 ) ) ;
#80716=VERTEX_POINT ( 'NONE', #40733 ) ;
#80723=VECTOR ( 'NONE', #70193, 1000.000000000000000 ) ;
#80725=EDGE_CURVE ( 'NONE', #37516, #59170, #26002, .T. ) ;
#80729=DIRECTION ( 'NONE',  ( 0.8526401643540846287, 0.000000000000000000, 0.5224985647159611224 ) ) ;
#80731=ADVANCED_FACE ( 'NONE', ( #16757 ), #78600, .T. ) ;
#80733=CARTESIAN_POINT ( 'NONE',  ( 0.000000000000000000, 15.00000000000000000, 0.000000000000000000 ) ) ;
#80750=CARTESIAN_POINT ( 'NONE',  ( -2.361410439757430701, 0.2306972965111891150, 14.75336556272935162 ) ) ;
#80754=CARTESIAN_POINT ( 'NONE',  ( 3.469446951953614189E-15, 4.171802177851546389, 11.25000000000000355 ) ) ;
#80758=CARTESIAN_POINT ( 'NONE',  ( -14.71525861348291997, 15.00000000000000000, 2.908807992686483601 ) ) ;
#80773=EDGE_LOOP ( 'NONE', ( #12099, #79373, #48208, #98580, #58188, #46991 ) ) ;
#80774=AXIS2_PLACEMENT_3D ( 'NONE', #40683, #2212, #41188 ) ;
#80777=DIRECTION ( 'NONE',  ( 0.000000000000000000, 1.000000000000000000, 0.000000000000000000 ) ) ;
#80783=ORIENTED_EDGE ( 'NONE', *, *, #65705, .T. ) ;
#80791=CARTESIAN_POINT ( 'NONE',  ( -13.21272562212263502, 14.99999999999808686, 6.271554226548477828 ) ) ;
#80800=ORIENTED_EDGE ( 'NONE', *, *, #23608, .F. ) ;
#80818=DIRECTION ( 'NONE',  ( 0.000000000000000000, 0.000000000000000000, 1.000000000000000000 ) ) ;
#80819=EDGE_CURVE ( 'NONE', #94458, #86688, #38634, .T. ) ;
#80824=VECTOR ( 'NONE', #89794, 999.9999999999998863 ) ;
#80830=AXIS2_PLACEMENT_3D ( 'NONE', #20219, #12715, #96732 ) ;
#80842=AXIS2_PLACEMENT_3D ( 'NONE', #31188, #83220, #92678 ) ;
#80844=EDGE_CURVE ( 'NONE', #77069, #26051, #41858, .T. ) ;
#80853=CARTESIAN_POINT ( 'NONE',  ( -11.36220558718868290, 15.00000000000000000, 9.008345252845137097 ) ) ;
#80860=CARTESIAN_POINT ( 'NONE',  ( -14.48718990079890290, 15.00000000000000000, 0.6093675230839377122 ) ) ;
#80861=CYLINDRICAL_SURFACE ( 'NONE', #83830, 15.00000000000000000 ) ;
#80864=DIRECTION ( 'NONE',  ( -0.4305110968082861977, 0.000000000000000000, -0.9025852843498647360 ) ) ;
#80866=ORIENTED_EDGE ( 'NONE', *, *, #42403, .F. ) ;
#80867=CARTESIAN_POINT ( 'NONE',  ( -1.780824192092605562, 0.5000000000000004441, 14.89391369643512064 ) ) ;
#80870=CARTESIAN_POINT ( 'NONE',  ( 6.898461952320432466, 4.226027835726576547E-16, -12.75387089053309175 ) ) ;
#80873=DIRECTION ( 'NONE',  ( 0.2503800040544526539, 0.000000000000000000, -0.9681476403781048568 ) ) ;
#80875=DIRECTION ( 'NONE',  ( 0.8526401643540917341, 0.000000000000000000, -0.5224985647159495761 ) ) ;
#80882=CARTESIAN_POINT ( 'NONE',  ( -13.50171220565091090, -3.121739927105722716E-15, 5.622479820943727447 ) ) ;
#80884=ORIENTED_EDGE ( 'NONE', *, *, #38681, .T. ) ;
#80887=ADVANCED_FACE ( 'NONE', ( #78730 ), #10240, .F. ) ;
#80888=LINE ( 'NONE', #12386, #53927 ) ;
#80889=CIRCLE ( 'NONE', #47337, 14.49999999999999822 ) ;
#80891=CARTESIAN_POINT ( 'NONE',  ( 14.93875075227017213, 14.76984974223857172, -0.2365588874159303689 ) ) ;
#80893=EDGE_LOOP ( 'NONE', ( #21323, #35075, #66328, #72184 ) ) ;
#80895=VECTOR ( 'NONE', #20603, 999.9999999999998863 ) ;
#80896=CARTESIAN_POINT ( 'NONE',  ( -14.56368227077854272, 14.76930270348881002, -3.337246381125379191 ) ) ;
#80900=CARTESIAN_POINT ( 'NONE',  ( 10.97221242068710012, 15.00000000000000533, -9.670525607392798761 ) ) ;
#80902=LINE ( 'NONE', #12888, #90484 ) ;
#80904=CARTESIAN_POINT ( 'NONE',  ( 10.64017930668205736, 0.5000000000000004441, -10.57291749337215592 ) ) ;
#80910=LINE ( 'NONE', #26915, #35079 ) ;
#80911=CARTESIAN_POINT ( 'NONE',  ( -5.204170427930421283E-15, 8.438309369127518167, -11.92686044187656513 ) ) ;
#80915=CARTESIAN_POINT ( 'NONE',  ( 14.02068044289381987, 14.49999999999999112, 5.331089937175756077 ) ) ;
#80917=AXIS2_PLACEMENT_3D ( 'NONE', #71841, #50307, #12319 ) ;
#80929=DIRECTION ( 'NONE',  ( 0.1993679344171971901, 0.000000000000000000, 0.9799247046208295897 ) ) ;
#80937=EDGE_CURVE ( 'NONE', #20205, #8435, #6863, .T. ) ;
#80939=CARTESIAN_POINT ( 'NONE',  ( -12.21130863673212197, 15.00000000000000533, 8.049375889232891268 ) ) ;
#80941=ORIENTED_EDGE ( 'NONE', *, *, #74680, .F. ) ;
#80948=EDGE_CURVE ( 'NONE', #1705, #19380, #25864, .T. ) ;
#80950=DIRECTION ( 'NONE',  ( 0.6225146366376079765, 0.000000000000000000, 0.7826081568524232424 ) ) ;
#80955=CARTESIAN_POINT ( 'NONE',  ( -9.382169495545413795, -35.25136533006957507, 9.382169495545428006 ) ) ;
#80964=AXIS2_PLACEMENT_3D ( 'NONE', #61064, #91065, #53068 ) ;
#80971=EDGE_CURVE ( 'NONE', #90286, #22448, #28181, .T. ) ;
#80972=ORIENTED_EDGE ( 'NONE', *, *, #45046, .F. ) ;
#80977=CARTESIAN_POINT ( 'NONE',  ( 4.838527690343521925, 15.00000000000000000, 14.19819177887730177 ) ) ;
#80980=CARTESIAN_POINT ( 'NONE',  ( 11.22915323889574601, 15.00000000000000000, 8.773176023390684364 ) ) ;
#80984=VECTOR ( 'NONE', #83137, 1000.000000000000000 ) ;
#80985=CARTESIAN_POINT ( 'NONE',  ( -3.166711953933203372, 0.000000000000000000, -4.439566422914469790 ) ) ;
#80989=CARTESIAN_POINT ( 'NONE',  ( -12.50534872682722565, 15.00000000000000000, -7.339363270777700343 ) ) ;
#81004=CARTESIAN_POINT ( 'NONE',  ( 0.000000000000000000, 14.49999999999999822, 0.000000000000000000 ) ) ;
#81005=ADVANCED_FACE ( 'NONE', ( #3727 ), #73176, .T. ) ;
#81007=CARTESIAN_POINT ( 'NONE',  ( 14.16423886937410082, -30.48791783175269288, -3.795296366450314096 ) ) ;
#81011=AXIS2_PLACEMENT_3D ( 'NONE', #34280, #34788, #79805 ) ;
#81021=CARTESIAN_POINT ( 'NONE',  ( 2.915334737309921209, 11.60535201082150714, -10.88017736071110164 ) ) ;
#81023=ORIENTED_EDGE ( 'NONE', *, *, #47534, .F. ) ;
#81033=CARTESIAN_POINT ( 'NONE',  ( -14.09394518620614711, 15.00000000000000000, 3.407449058785264384 ) ) ;
#81039=PLANE ( 'NONE',  #95723 ) ;
#81041=CARTESIAN_POINT ( 'NONE',  ( 0.000000000000000000, 15.00000000000000000, 0.000000000000000000 ) ) ;
#81049=AXIS2_PLACEMENT_3D ( 'NONE', #54166, #16188, #8676 ) ;
#81059=DIRECTION ( 'NONE',  ( -0.9304175679820255729, 0.000000000000000000, 0.3665012267242946931 ) ) ;
#81060=CARTESIAN_POINT ( 'NONE',  ( -12.25993886608597094, 14.49999999999999112, -8.642563219313844414 ) ) ;
#81065=CARTESIAN_POINT ( 'NONE',  ( -13.48086198287156101, 15.00000000000000000, -8.610676897597642210 ) ) ;
#81068=CARTESIAN_POINT ( 'NONE',  ( -3.469446951953614189E-15, 4.758931151000789228, -9.846743663894594434 ) ) ;
#81069=VERTEX_POINT ( 'NONE', #96703 ) ;
#81071=CARTESIAN_POINT ( 'NONE',  ( 12.83294900548058415, 15.00000000000000000, 7.766300266068450142 ) ) ;
#81078=DIRECTION ( 'NONE',  ( -0.8141155183563145714, 0.000000000000000000, -0.5807029557109463225 ) ) ;
#81080=VERTEX_POINT ( 'NONE', #57689 ) ;
#81090=CARTESIAN_POINT ( 'NONE',  ( 0.000000000000000000, 0.000000000000000000, 0.000000000000000000 ) ) ;
#81092=CARTESIAN_POINT ( 'NONE',  ( -5.991992585808713301, 15.00000000000000000, 13.20401548210291054 ) ) ;
#81093=DIRECTION ( 'NONE',  ( -0.000000000000000000, -1.000000000000000000, -0.000000000000000000 ) ) ;
#81102=CARTESIAN_POINT ( 'NONE',  ( -9.705452947461466806, 12.49999999999999289, -5.689172442861226031 ) ) ;
#81108=DIRECTION ( 'NONE',  ( 0.000000000000000000, 0.000000000000000000, 1.000000000000000000 ) ) ;
#81113=DIRECTION ( 'NONE',  ( 0.000000000000000000, 1.000000000000000000, 0.000000000000000000 ) ) ;
#81118=ORIENTED_EDGE ( 'NONE', *, *, #89195, .T. ) ;
#81130=CARTESIAN_POINT ( 'NONE',  ( -5.204170427930421283E-15, -28.18631465584515894, -10.88017736071110342 ) ) ;
#81135=CARTESIAN_POINT ( 'NONE',  ( -9.997910040112463648, 15.00000000000000000, -10.50199004140731773 ) ) ;
#81136=EDGE_CURVE ( 'NONE', #84772, #41516, #73555, .T. ) ;
#81138=CARTESIAN_POINT ( 'NONE',  ( 13.82671409943293739, 15.00000000000000000, 3.447387012295318076 ) ) ;
#81146=DIRECTION ( 'NONE',  ( 0.000000000000000000, 0.000000000000000000, 1.000000000000000000 ) ) ;
#81150=DIRECTION ( 'NONE',  ( 0.6087614290087186575, -0.000000000000000000, 0.7933533402912366084 ) ) ;
#81161=ORIENTED_EDGE ( 'NONE', *, *, #19580, .F. ) ;
#81163=SHAPE_REPRESENTATION ( '1.3 Adjustment Nut', ( #27931 ), #10314 ) ;
#81168=ORIENTED_EDGE ( 'NONE', *, *, #28883, .F. ) ;
#81181=EDGE_CURVE ( 'NONE', #27759, #87330, #76951, .T. ) ;
#81184=CARTESIAN_POINT ( 'NONE',  ( -14.71525861348291997, 0.5000000000000004441, 2.908807992686483601 ) ) ;
#81187=CARTESIAN_POINT ( 'NONE',  ( 3.469446951953614189E-15, -32.74106884899921255, 9.846743663894594434 ) ) ;
#81191=VERTEX_POINT ( 'NONE', #35058 ) ;
#81195=AXIS2_PLACEMENT_3D ( 'NONE', #98302, #6285, #36788 ) ;
#81196=DIRECTION ( 'NONE',  ( 0.000000000000000000, 0.000000000000000000, 1.000000000000000000 ) ) ;
#81198=EDGE_CURVE ( 'NONE', #765, #31971, #48180, .T. ) ;
#81200=CARTESIAN_POINT ( 'NONE',  ( -12.81628187352647252, 9.331968003263757083, 3.434112377981066722 ) ) ;
#81216=LINE ( 'NONE', #44192, #91391 ) ;
#81217=CARTESIAN_POINT ( 'NONE',  ( -9.322910753577803078, 0.04922511925148240902, -11.43369735623891081 ) ) ;
#81218=CARTESIAN_POINT ( 'NONE',  ( 1.780824192092501423, 0.5000000000000004441, -14.89391369643513485 ) ) ;
#81223=AXIS2_PLACEMENT_3D ( 'NONE', #11181, #41701, #20158 ) ;
#81225=CARTESIAN_POINT ( 'NONE',  ( -13.34343830728394309, 0.5000000000000004441, -6.852200678592783589 ) ) ;
#81232=FACE_OUTER_BOUND ( 'NONE', #81289, .T. ) ;
#81238=VERTEX_POINT ( 'NONE', #51060 ) ;
#81250=CARTESIAN_POINT ( 'NONE',  ( 14.62617646268085281, 0.5000000000000004441, 3.327906561566980503 ) ) ;
#81251=CARTESIAN_POINT ( 'NONE',  ( -3.795296366450300773, 7.845415501580634832, 14.16423886937410437 ) ) ;
#81270=ORIENTED_EDGE ( 'NONE', *, *, #61286, .F. ) ;
#81272=CARTESIAN_POINT ( 'NONE',  ( -11.35178980618960409, 0.5000000000000004441, -9.804941009312079458 ) ) ;
#81283=CARTESIAN_POINT ( 'NONE',  ( -11.75249112336564394, 14.95037104119133886, 8.918310463590344739 ) ) ;
#81289=EDGE_LOOP ( 'NONE', ( #24671, #54023, #92559, #65590 ) ) ;
#81297=B_SPLINE_CURVE_WITH_KNOTS ( 'NONE', 3,
 ( #89708, #36220, #20232, #80236, #35724, #89222 ),
 .UNSPECIFIED., .F., .F.,
 ( 4, 2, 4 ),
 ( 3.409110551463477909E-05, 0.0004400426677364613652, 0.0008459942299582879580 ),
 .UNSPECIFIED. ) ;
#81298=ADVANCED_FACE ( 'NONE', ( #74549 ), #58060, .T. ) ;
#81306=ORIENTED_EDGE ( 'NONE', *, *, #93354, .T. ) ;
#81310=VERTEX_POINT ( 'NONE', #50571 ) ;
#81313=LINE ( 'NONE', #59787, #88736 ) ;
#81317=CARTESIAN_POINT ( 'NONE',  ( -11.92686044187656336, 12.87045670184115487, 3.195792623639540864 ) ) ;
#81318=EDGE_CURVE ( 'NONE', #37243, #91269, #29055, .T. ) ;
#81319=ADVANCED_FACE ( 'NONE', ( #14066 ), #57816, .T. ) ;
#81325=ORIENTED_EDGE ( 'NONE', *, *, #42056, .F. ) ;
#81330=DIRECTION ( 'NONE',  ( 0.1650476058606878405, 0.000000000000000000, -0.9862856015372296614 ) ) ;
#81335=CARTESIAN_POINT ( 'NONE',  ( 14.37564666802670921, 14.99999999999801759, 2.692451322021577553 ) ) ;
#81339=ORIENTED_EDGE ( 'NONE', *, *, #45437, .T. ) ;
#81340=CARTESIAN_POINT ( 'NONE',  ( -7.684764310694972345, 14.63595249122790598, 12.88194075009929840 ) ) ;
#81344=CARTESIAN_POINT ( 'NONE',  ( 10.14667048435138064, 4.748928130477084912E-16, 10.35833375027048042 ) ) ;
#81345=CARTESIAN_POINT ( 'NONE',  ( -7.002992508389124460, 15.00000000000000533, 12.84003923133013458 ) ) ;
#81348=CARTESIAN_POINT ( 'NONE',  ( 10.97221242068703262, -3.201784540621254098E-15, 9.670525607392866263 ) ) ;
#81360=CARTESIAN_POINT ( 'NONE',  ( 8.502626202121348342, 14.95077488074853811, -12.05617882333536528 ) ) ;
#81367=CARTESIAN_POINT ( 'NONE',  ( -3.420591144908647241, 15.00000000000000000, 14.60477854057953451 ) ) ;
#81374=EDGE_CURVE ( 'NONE', #60724, #61703, #20067, .T. ) ;
#81375=LINE ( 'NONE', #5399, #28373 ) ;
#81377=CARTESIAN_POINT ( 'NONE',  ( 14.75001642003106817, 14.95037105299814506, -0.3071237627329282960 ) ) ;
#81380=PLANE ( 'NONE',  #80201 ) ;
#81387=ORIENTED_EDGE ( 'NONE', *, *, #89151, .T. ) ;
#81389=DIRECTION ( 'NONE',  ( 0.8141155183563107967, 0.000000000000000000, 0.5807029557109515405 ) ) ;
#81400=DIRECTION ( 'NONE',  ( 0.000000000000000000, 1.000000000000000000, -0.000000000000000000 ) ) ;
#81417=VECTOR ( 'NONE', #55119, 1000.000000000000000 ) ;
#81423=DIRECTION ( 'NONE',  ( -0.9762960071199346945, 0.000000000000000000, 0.2164396139380971307 ) ) ;
#81426=DIRECTION ( 'NONE',  ( 0.000000000000000000, 0.000000000000000000, 1.000000000000000000 ) ) ;
#81429=CARTESIAN_POINT ( 'NONE',  ( -9.240973841163452107, 15.00000000000000000, -11.17382667070385160 ) ) ;
#81437=B_SPLINE_CURVE_WITH_KNOTS ( 'NONE', 3,
 ( #13237, #97260, #67231, #90213, #21746, #42756 ),
 .UNSPECIFIED., .F., .F.,
 ( 4, 2, 4 ),
 ( 3.409110551487192799E-05, 0.0004400426677366973418, 0.0008459942299585226878 ),
 .UNSPECIFIED. ) ;
#81438=ORIENTED_EDGE ( 'NONE', *, *, #81572, .F. ) ;
#81439=LINE ( 'NONE', #43437, #49508 ) ;
#81441=CARTESIAN_POINT ( 'NONE',  ( 11.09922568453594671, -22.95969866340291077, -6.408140936763241591 ) ) ;
#81451=CARTESIAN_POINT ( 'NONE',  ( -13.30119215211286132, 0.2301510699511994940, 6.804450086557105593 ) ) ;
#81452=ORIENTED_EDGE ( 'NONE', *, *, #1567, .T. ) ;
#81467=EDGE_LOOP ( 'NONE', ( #53799, #57790, #19118, #72587 ) ) ;
#81468=VECTOR ( 'NONE', #71700, 1000.000000000000000 ) ;
#81475=CARTESIAN_POINT ( 'NONE',  ( 0.000000000000000000, 14.49999999999999822, 0.000000000000000000 ) ) ;
#81478=DIRECTION ( 'NONE',  ( 0.9890158633619187123, 0.000000000000000000, -0.1478094111295981949 ) ) ;
#81485=AXIS2_PLACEMENT_3D ( 'NONE', #17773, #87229, #50719 ) ;
#81489=EDGE_CURVE ( 'NONE', #39153, #56002, #15065, .T. ) ;
#81491=CARTESIAN_POINT ( 'NONE',  ( 12.26659068614894821, -26.11291783175269288, 7.082119434687044190 ) ) ;
#81495=EDGE_LOOP ( 'NONE', ( #82359, #62822, #32010, #5950, #66308, #35805 ) ) ;
#81507=CARTESIAN_POINT ( 'NONE',  ( 7.964842623401177768, 16.18868534415483396, -7.964842623401181321 ) ) ;
#81520=CARTESIAN_POINT ( 'NONE',  ( 14.16722289976686966, 14.49999999999999112, 4.928467845925658786 ) ) ;
#81536=AXIS2_PLACEMENT_3D ( 'NONE', #67018, #57039, #50530 ) ;
#81547=CARTESIAN_POINT ( 'NONE',  ( -14.71525861348291997, 0.5000000000000004441, 2.908807992686483601 ) ) ;
#81552=CARTESIAN_POINT ( 'NONE',  ( -7.208316651077756099, 21.63393115100078390, 7.208316651077766757 ) ) ;
#81554=ORIENTED_EDGE ( 'NONE', *, *, #44340, .F. ) ;
#81556=CIRCLE ( 'NONE', #52800, 15.00000000000000000 ) ;
#81565=EDGE_CURVE ( 'NONE', #28808, #26148, #71342, .T. ) ;
#81567=ORIENTED_EDGE ( 'NONE', *, *, #84063, .F. ) ;
#81570=ORIENTED_EDGE ( 'NONE', *, *, #68966, .F. ) ;
#81572=EDGE_CURVE ( 'NONE', #26555, #93626, #96161, .T. ) ;
#81573=ORIENTED_EDGE ( 'NONE', *, *, #45060, .F. ) ;
#81580=LINE ( 'NONE', #95611, #80895 ) ;
#81581=ORIENTED_EDGE ( 'NONE', *, *, #28706, .F. ) ;
#81588=CARTESIAN_POINT ( 'NONE',  ( -10.76421366023792103, 12.61593446625853865, -3.660229437423404342 ) ) ;
#81592=CARTESIAN_POINT ( 'NONE',  ( 4.096035146093531587, 15.00000000000000000, -13.90943910019259278 ) ) ;
#81593=VERTEX_POINT ( 'NONE', #28456 ) ;
#81596=CARTESIAN_POINT ( 'NONE',  ( -14.04867373755345561, -0.03417435944610275333, -7.649324326489842285 ) ) ;
#81599=DIRECTION ( 'NONE',  ( 5.151434834260726979E-14, 0.000000000000000000, 1.000000000000000000 ) ) ;
#81600=ADVANCED_FACE ( 'NONE', ( #73949 ), #29424, .F. ) ;
#81604=CONICAL_SURFACE ( 'NONE', #49700, 11.25000000000000178, 0.7853981633974497223 ) ;
#81607=VERTEX_POINT ( 'NONE', #19963 ) ;
#81619=CARTESIAN_POINT ( 'NONE',  ( 10.88017736071110164, -24.64464798917849109, 2.915334737309921209 ) ) ;
#81624=CARTESIAN_POINT ( 'NONE',  ( 10.97324858046193619, 15.00000000000000711, 9.670892530813269161 ) ) ;
#81629=EDGE_CURVE ( 'NONE', #7169, #96379, #48645, .T. ) ;
#81632=CARTESIAN_POINT ( 'NONE',  ( 3.927832320392154575, -0.03417435944610275333, 13.69797916712106733 ) ) ;
#81636=ORIENTED_EDGE ( 'NONE', *, *, #55444, .T. ) ;
#81645=DIRECTION ( 'NONE',  ( 0.000000000000000000, 0.000000000000000000, -1.000000000000000000 ) ) ;
#81647=EDGE_LOOP ( 'NONE', ( #64337, #91728, #31044, #8237, #80596, #17035 ) ) ;
#81650=ORIENTED_EDGE ( 'NONE', *, *, #92072, .F. ) ;
#81651=VERTEX_POINT ( 'NONE', #81941 ) ;
#81667=CARTESIAN_POINT ( 'NONE',  ( -4.923371831947292776, -33.15773551566587685, 8.527530157486181039 ) ) ;
#81669=CARTESIAN_POINT ( 'NONE',  ( 0.3093388210927754400, 14.63745559856262624, -14.99680997725068821 ) ) ;
#81671=ORIENTED_EDGE ( 'NONE', *, *, #88643, .T. ) ;
#81675=CARTESIAN_POINT ( 'NONE',  ( 13.55255535720591986, 15.00000000000000000, 4.403492169843056914 ) ) ;
#81679=CARTESIAN_POINT ( 'NONE',  ( 3.434112377981060948, 5.581968003263752642, 12.81628187352647430 ) ) ;
#81680=ORIENTED_EDGE ( 'NONE', *, *, #70473, .F. ) ;
#81691=AXIS2_PLACEMENT_3D ( 'NONE', #3649, #79139, #3157 ) ;
#81695=B_SPLINE_CURVE_WITH_KNOTS ( 'NONE', 3,
 ( #44730, #15249, #67242, #29230, #14249, #53223 ),
 .UNSPECIFIED., .F., .F.,
 ( 4, 2, 4 ),
 ( 3.409110551493951444E-05, 0.0004400426677367878184, 0.0008459942299586360953 ),
 .UNSPECIFIED. ) ;
#81697=ORIENTED_EDGE ( 'NONE', *, *, #18083, .F. ) ;
#81699=PLANE ( 'NONE',  #57834 ) ;
#81701=DIRECTION ( 'NONE',  ( 0.000000000000000000, 0.000000000000000000, 1.000000000000000000 ) ) ;
#81704=ORIENTED_EDGE ( 'NONE', *, *, #95410, .F. ) ;
#81706=CARTESIAN_POINT ( 'NONE',  ( -13.34343830728394842, 0.3640475087720989600, -6.852200678592788918 ) ) ;
#81719=ADVANCED_FACE ( 'NONE', ( #28931 ), #43936, .T. ) ;
#81723=CARTESIAN_POINT ( 'NONE',  ( -4.289191146912808207E-15, 3.868033628982651795, -11.25000000000000178 ) ) ;
#81727=CARTESIAN_POINT ( 'NONE',  ( 0.000000000000000000, 0.5000000000000004441, 0.000000000000000000 ) ) ;
#81734=CARTESIAN_POINT ( 'NONE',  ( -12.26659068614894110, 7.220415501580639273, 7.082119434687058401 ) ) ;
#81738=CARTESIAN_POINT ( 'NONE',  ( 0.000000000000000000, 14.49999999999999822, 0.000000000000000000 ) ) ;
#81745=PLANE ( 'NONE',  #27592 ) ;
#81746=CARTESIAN_POINT ( 'NONE',  ( 0.000000000000000000, 0.000000000000000000, 0.000000000000000000 ) ) ;
#81754=EDGE_CURVE ( 'NONE', #45067, #92561, #70681, .T. ) ;
#81770=EDGE_CURVE ( 'NONE', #42002, #20489, #66544, .T. ) ;
#81777=DIRECTION ( 'NONE',  ( 0.000000000000000000, 0.000000000000000000, 1.000000000000000000 ) ) ;
#81792=EDGE_LOOP ( 'NONE', ( #89079, #31, #77406 ) ) ;
#81794=AXIS2_PLACEMENT_3D ( 'NONE', #35456, #27952, #58445 ) ;
#81795=CARTESIAN_POINT ( 'NONE',  ( -5.963430220938290560, 11.82879003517447281, -10.32896413005679648 ) ) ;
#81797=ORIENTED_EDGE ( 'NONE', *, *, #94013, .F. ) ;
#81813=ORIENTED_EDGE ( 'NONE', *, *, #52829, .F. ) ;
#81816=CARTESIAN_POINT ( 'NONE',  ( -7.771322705631588335, 4.175205849424987664E-16, 12.24159072199911868 ) ) ;
#81821=AXIS2_PLACEMENT_3D ( 'NONE', #51945, #59922, #82430 ) ;
#81824=AXIS2_PLACEMENT_3D ( 'NONE', #96785, #43753, #21771 ) ;
#81826=CARTESIAN_POINT ( 'NONE',  ( 3.927832320392247389, 0.000000000000000000, -13.69797916712104602 ) ) ;
#81830=DIRECTION ( 'NONE',  ( 0.000000000000000000, 1.000000000000000000, 0.000000000000000000 ) ) ;
#81837=ADVANCED_FACE ( 'NONE', ( #98465 ), #15923, .T. ) ;
#81852=CARTESIAN_POINT ( 'NONE',  ( -10.93781366033355695, 0.3639309795253648505, 10.26470809774060911 ) ) ;
#81853=DIRECTION ( 'NONE',  ( 0.000000000000000000, 0.000000000000000000, 1.000000000000000000 ) ) ;
#81857=ORIENTED_EDGE ( 'NONE', *, *, #4197, .F. ) ;
#81859=DIRECTION ( 'NONE',  ( 0.000000000000000000, 1.000000000000000000, 0.000000000000000000 ) ) ;
#81867=CARTESIAN_POINT ( 'NONE',  ( -14.62617646268090077, 14.49999999999999112, -3.327906561567068433 ) ) ;
#81868=DIRECTION ( 'NONE',  ( -0.7933533402912325005, 0.000000000000000000, -0.6087614290087243196 ) ) ;
#81875=VERTEX_POINT ( 'NONE', #84906 ) ;
#81877=ADVANCED_FACE ( 'NONE', ( #38431 ), #29118, .T. ) ;
#81888=DIRECTION ( 'NONE',  ( -0.000000000000000000, -1.000000000000000000, -0.000000000000000000 ) ) ;
#81889=DIRECTION ( 'NONE',  ( -0.1650476058606676344, 0.000000000000000000, -0.9862856015372331031 ) ) ;
#81900=ORIENTED_EDGE ( 'NONE', *, *, #62762, .T. ) ;
#81915=ORIENTED_EDGE ( 'NONE', *, *, #72783, .F. ) ;
#81920=CARTESIAN_POINT ( 'NONE',  ( 14.82269085861168811, 0.5000000000000004441, -2.299529454046961519 ) ) ;
#81925=DIRECTION ( 'NONE',  ( 0.000000000000000000, 1.000000000000000000, 0.000000000000000000 ) ) ;
#81931=CARTESIAN_POINT ( 'NONE',  ( -3.434112377981047626, -24.83469866340290721, 12.81628187352647963 ) ) ;
#81940=AXIS2_PLACEMENT_3D ( 'NONE', #47655, #71639, #62639 ) ;
#81941=CARTESIAN_POINT ( 'NONE',  ( -14.49440716394874151, 3.911302179139366829E-16, 0.4026921475165256004 ) ) ;
#81942=VERTEX_POINT ( 'NONE', #46895 ) ;
#81960=DIRECTION ( 'NONE',  ( -2.131628207280300873E-14, 0.000000000000000000, 1.000000000000000000 ) ) ;
#81961=EDGE_CURVE ( 'NONE', #42454, #18033, #68960, .T. ) ;
#81969=AXIS2_PLACEMENT_3D ( 'NONE', #71428, #10912, #19395 ) ;
#81971=B_SPLINE_CURVE_WITH_KNOTS ( 'NONE', 3,
 ( #93421, #95388, #47910, #26391, #18912, #40437 ),
 .UNSPECIFIED., .F., .F.,
 ( 4, 2, 4 ),
 ( 0.0002800047503720853067, 0.0006862100262544242307, 0.001092415302136763317 ),
 .UNSPECIFIED. ) ;
#81977=CARTESIAN_POINT ( 'NONE',  ( -5.419894505350681513, 0.3640475087720754788, 13.98659156302455209 ) ) ;
#81981=CARTESIAN_POINT ( 'NONE',  ( 5.148594389986301145, 1.711006553453686685E-16, -13.69051944078647054 ) ) ;
#81986=FACE_OUTER_BOUND ( 'NONE', #65804, .T. ) ;
#81988=CARTESIAN_POINT ( 'NONE',  ( -7.082119434687044190, -17.36291783175269288, 12.26659068614894998 ) ) ;
#81996=CARTESIAN_POINT ( 'NONE',  ( 0.000000000000000000, 0.5000000000000004441, 0.000000000000000000 ) ) ;
#81999=CARTESIAN_POINT ( 'NONE',  ( 0.000000000000000000, 0.5000000000000004441, 0.000000000000000000 ) ) ;
#82001=LINE ( 'NONE', #43994, #39031 ) ;
#82003=CARTESIAN_POINT ( 'NONE',  ( 4.494156999534569152, 0.000000000000000000, 3.088748530746300958 ) ) ;
#82007=CARTESIAN_POINT ( 'NONE',  ( 2.393480905993052854, 15.00000000000000000, 14.80781041047752922 ) ) ;
#82008=ORIENTED_EDGE ( 'NONE', *, *, #50446, .F. ) ;
#82009=CIRCLE ( 'NONE', #43682, 15.00000000000000000 ) ;
#82018=CARTESIAN_POINT ( 'NONE',  ( 5.963430220938279902, 10.99545670184114066, -10.32896413005680181 ) ) ;
#82019=CYLINDRICAL_SURFACE ( 'NONE', #72057, 15.00000000000000000 ) ;
#82031=CARTESIAN_POINT ( 'NONE',  ( -9.997910040112669705, 15.00000000000000000, 10.50199004140708325 ) ) ;
#82035=CARTESIAN_POINT ( 'NONE',  ( 14.02068044289378967, 0.5000000000000004441, -5.331089937175664595 ) ) ;
#82045=DIRECTION ( 'NONE',  ( 0.7132504491541897806, 0.000000000000000000, -0.7009092642998425715 ) ) ;
#82047=VECTOR ( 'NONE', #28622, 1000.000000000000000 ) ;
#82048=DIRECTION ( 'NONE',  ( 0.000000000000000000, 1.000000000000000000, 0.000000000000000000 ) ) ;
#82049=CARTESIAN_POINT ( 'NONE',  ( -9.846743663894594434, 16.00893115100079100, 3.469446951953614189E-15 ) ) ;
#82050=ORIENTED_EDGE ( 'NONE', *, *, #54085, .T. ) ;
#82053=CARTESIAN_POINT ( 'NONE',  ( -6.728851239468925272, 15.00000000000000711, -12.98580270086209865 ) ) ;
#82064=B_SPLINE_CURVE_WITH_KNOTS ( 'NONE', 3,
 ( #43551, #96581, #60533, #13557, #83540, #73550 ),
 .UNSPECIFIED., .F., .F.,
 ( 4, 2, 4 ),
 ( 3.409110551443771857E-05, 0.0004400426677362852365, 0.0008459942299581327003 ),
 .UNSPECIFIED. ) ;
#82066=ORIENTED_EDGE ( 'NONE', *, *, #78556, .F. ) ;
#82070=ORIENTED_EDGE ( 'NONE', *, *, #12569, .F. ) ;
#82074=PLANE ( 'NONE',  #13649 ) ;
#82077=PLANE ( 'NONE',  #88888 ) ;
#82084=EDGE_CURVE ( 'NONE', #15233, #86853, #85027, .T. ) ;
#82087=CARTESIAN_POINT ( 'NONE',  ( -11.50383178867919298, 12.89949214739216465, 1.921679737233346730 ) ) ;
#82089=CARTESIAN_POINT ( 'NONE',  ( 0.000000000000000000, 0.5000000000000004441, 0.000000000000000000 ) ) ;
#82091=FACE_OUTER_BOUND ( 'NONE', #53751, .T. ) ;
#82093=CARTESIAN_POINT ( 'NONE',  ( 9.322910753577957621, 14.95077488074852390, -11.43369735623877226 ) ) ;
#82101=VECTOR ( 'NONE', #12670, 1000.000000000000000 ) ;
#82110=VECTOR ( 'NONE', #83979, 1000.000000000000000 ) ;
#82115=CARTESIAN_POINT ( 'NONE',  ( -2.915334737309934532, -7.977981322511819684, -10.88017736071109987 ) ) ;
#82119=CARTESIAN_POINT ( 'NONE',  ( 11.35178980618968048, 14.63595249122790598, 9.804941009312001299 ) ) ;
#82140=DIRECTION ( 'NONE',  ( -0.000000000000000000, -1.000000000000000000, -0.000000000000000000 ) ) ;
#82142=AXIS2_PLACEMENT_3D ( 'NONE', #57307, #34295, #18834 ) ;
#82144=CARTESIAN_POINT ( 'NONE',  ( 0.000000000000000000, 15.00000000000000000, 0.000000000000000000 ) ) ;
#82146=ORIENTED_EDGE ( 'NONE', *, *, #81565, .T. ) ;
#82163=CARTESIAN_POINT ( 'NONE',  ( 3.469446951953614189E-15, -22.74106884899921255, 9.846743663894594434 ) ) ;
#82164=ORIENTED_EDGE ( 'NONE', *, *, #14633, .F. ) ;
#82173=LINE ( 'NONE', #5703, #94120 ) ;
#82174=ADVANCED_FACE ( 'NONE', ( #26360 ), #30689, .T. ) ;
#82177=ADVANCED_FACE ( 'NONE', ( #47877 ), #63853, .T. ) ;
#82178=VECTOR ( 'NONE', #70450, 1000.000000000000000 ) ;
#82180=CARTESIAN_POINT ( 'NONE',  ( -12.81628187352647963, 13.91530133659708746, -3.434112377981046293 ) ) ;
#82183=AXIS2_PLACEMENT_3D ( 'NONE', #31336, #84847, #399 ) ;
#82191=DIRECTION ( 'NONE',  ( -0.02617694830786282401, 0.000000000000000000, -0.9996573249755575929 ) ) ;
#82192=ADVANCED_FACE ( 'NONE', ( #71393 ), #78381, .T. ) ;
#82197=CIRCLE ( 'NONE', #34288, 15.00000000000000000 ) ;
#82198=CARTESIAN_POINT ( 'NONE',  ( -0.2851878892742317761, 0.2306287049188357752, -14.93850447011040750 ) ) ;
#82205=DIRECTION ( 'NONE',  ( 0.000000000000000000, 0.000000000000000000, 1.000000000000000000 ) ) ;
#82208=CARTESIAN_POINT ( 'NONE',  ( 10.19513985507825637, 15.00000000000000000, 11.00268709613223983 ) ) ;
#82212=DIRECTION ( 'NONE',  ( 0.09584575252023383451, 0.000000000000000000, -0.9953961983671778535 ) ) ;
#82227=DIRECTION ( 'NONE',  ( -0.4305110968082986878, 0.000000000000000000, 0.9025852843498588518 ) ) ;
#82233=DIRECTION ( 'NONE',  ( 0.000000000000000000, 1.000000000000000000, 0.000000000000000000 ) ) ;
#82234=CARTESIAN_POINT ( 'NONE',  ( 3.795296366450314540, 8.262082168247296465, 14.16423886937410082 ) ) ;
#82239=ADVANCED_FACE ( 'NONE', ( #25405 ), #45109, .T. ) ;
#82245=DIRECTION ( 'NONE',  ( 0.000000000000000000, 0.000000000000000000, 1.000000000000000000 ) ) ;
#82266=VERTEX_POINT ( 'NONE', #55891 ) ;
#82269=CARTESIAN_POINT ( 'NONE',  ( 8.235571585149873641, 4.796802177851536619, 8.235571585149866536 ) ) ;
#82282=ORIENTED_EDGE ( 'NONE', *, *, #49726, .T. ) ;
#82287=AXIS2_PLACEMENT_3D ( 'NONE', #29337, #38834, #37858 ) ;
#82290=EDGE_CURVE ( 'NONE', #5292, #78351, #37141, .T. ) ;
#82292=AXIS2_PLACEMENT_3D ( 'NONE', #87659, #4679, #49652 ) ;
#82293=EDGE_CURVE ( 'NONE', #14929, #16647, #62886, .T. ) ;
#82295=ORIENTED_EDGE ( 'NONE', *, *, #70069, .F. ) ;
#82300=EDGE_LOOP ( 'NONE', ( #590, #76467, #92342, #36428, #72699, #78599 ) ) ;
#82302=CARTESIAN_POINT ( 'NONE',  ( -12.15129255554601428, -0.03417435944610275333, -10.40305174771256524 ) ) ;
#82308=ADVANCED_FACE ( 'NONE', ( #86873 ), #93010, .T. ) ;
#82310=CIRCLE ( 'NONE', #47192, 15.00000000000000000 ) ;
#82314=CARTESIAN_POINT ( 'NONE',  ( -5.361923921558562789, 0.000000000000000000, -0.9937738586172705224 ) ) ;
#82322=CARTESIAN_POINT ( 'NONE',  ( 9.065164099344530158, 15.00000000000000000, -11.95084933600767307 ) ) ;
#82331=EDGE_CURVE ( 'NONE', #4363, #48181, #6803, .T. ) ;
#82337=DIRECTION ( 'NONE',  ( -0.000000000000000000, 1.000000000000000000, -0.000000000000000000 ) ) ;
#82341=CARTESIAN_POINT ( 'NONE',  ( -0.8060400322139609219, 0.000000000000000000, 5.393339789881734347 ) ) ;
#82347=DIRECTION ( 'NONE',  ( -0.000000000000000000, -1.000000000000000000, -0.000000000000000000 ) ) ;
#82351=ORIENTED_EDGE ( 'NONE', *, *, #48740, .F. ) ;
#82352=TOROIDAL_SURFACE ( 'NONE', #61584, 14.49999999999999822, 0.5000000000000000000 ) ;
#82354=DIRECTION ( 'NONE',  ( 0.000000000000000000, 0.000000000000000000, 1.000000000000000000 ) ) ;
#82358=DIRECTION ( 'NONE',  ( -0.000000000000000000, -1.000000000000000000, -0.000000000000000000 ) ) ;
#82359=ORIENTED_EDGE ( 'NONE', *, *, #92884, .T. ) ;
#82368=VERTEX_POINT ( 'NONE', #87843 ) ;
#82370=FACE_OUTER_BOUND ( 'NONE', #47018, .T. ) ;
#82380=CARTESIAN_POINT ( 'NONE',  ( -11.81378540890942119, 0.000000000000000000, 7.968498874458034287 ) ) ;
#82381=DIRECTION ( 'NONE',  ( -0.9366721892483949041, 0.000000000000000000, -0.3502073812594748148 ) ) ;
#82385=VECTOR ( 'NONE', #82337, 1000.000000000000000 ) ;
#82388=CARTESIAN_POINT ( 'NONE',  ( 15.41943733314631793, 15.00000000000000000, -4.256565371896342320 ) ) ;
#82390=VECTOR ( 'NONE', #97729, 1000.000000000000000 ) ;
#82395=CARTESIAN_POINT ( 'NONE',  ( 3.927832320392154575, 15.00000000000000000, 13.69797916712106733 ) ) ;
#82402=EDGE_CURVE ( 'NONE', #64121, #89795, #2046, .T. ) ;
#82411=EDGE_CURVE ( 'NONE', #61124, #74408, #58824, .T. ) ;
#82414=CARTESIAN_POINT ( 'NONE',  ( 0.000000000000000000, 14.49999999999999822, 0.000000000000000000 ) ) ;
#82419=CARTESIAN_POINT ( 'NONE',  ( 0.000000000000000000, 0.5000000000000004441, 0.000000000000000000 ) ) ;
#82423=VERTEX_POINT ( 'NONE', #88346 ) ;
#82425=CARTESIAN_POINT ( 'NONE',  ( 6.408140936763236262, -17.54303199673624292, -11.09922568453595026 ) ) ;
#82430=DIRECTION ( 'NONE',  ( 0.000000000000000000, 0.000000000000000000, 1.000000000000000000 ) ) ;
#82435=CIRCLE ( 'NONE', #39337, 14.49999999999999822 ) ;
#82436=EDGE_CURVE ( 'NONE', #51651, #53171, #47524, .T. ) ;
#82442=CARTESIAN_POINT ( 'NONE',  ( 0.000000000000000000, 13.17686044187655270, 0.000000000000000000 ) ) ;
#82453=CARTESIAN_POINT ( 'NONE',  ( 9.402796353261145157, 14.49999999999999112, -11.68706210897763320 ) ) ;
#82466=CARTESIAN_POINT ( 'NONE',  ( 0.000000000000000000, 15.00000000000000000, 0.000000000000000000 ) ) ;
#82473=CARTESIAN_POINT ( 'NONE',  ( -5.377205135396049940, 0.2306972965111756257, 13.94000429068777791 ) ) ;
#82485=CARTESIAN_POINT ( 'NONE',  ( 12.26659068614894466, -15.27958449841936073, -7.082119434687053960 ) ) ;
#82490=ORIENTED_EDGE ( 'NONE', *, *, #30121, .T. ) ;
#82498=CARTESIAN_POINT ( 'NONE',  ( 1.326515405096035494, 14.76930270348881002, 14.88215077106016437 ) ) ;
#82499=CARTESIAN_POINT ( 'NONE',  ( -7.964842623401179544, 22.43868534415484817, -7.964842623401174215 ) ) ;
#82514=AXIS2_PLACEMENT_3D ( 'NONE', #14546, #7545, #38035 ) ;
#82520=ORIENTED_EDGE ( 'NONE', *, *, #30312, .F. ) ;
#82521=FACE_OUTER_BOUND ( 'NONE', #67845, .T. ) ;
#82536=EDGE_CURVE ( 'NONE', #41530, #8435, #80355, .T. ) ;
#82539=CARTESIAN_POINT ( 'NONE',  ( 4.391347328463013788, 14.76984910450983257, -14.28069739540080896 ) ) ;
#82540=CARTESIAN_POINT ( 'NONE',  ( 0.000000000000000000, 14.49999999999999822, 0.000000000000000000 ) ) ;
#82544=AXIS2_PLACEMENT_3D ( 'NONE', #46673, #83701, #54170 ) ;
#82547=CARTESIAN_POINT ( 'NONE',  ( -10.14667048435128294, 15.00000000000000000, -10.35833375027054082 ) ) ;
#82549=DIRECTION ( 'NONE',  ( 0.000000000000000000, 0.000000000000000000, 1.000000000000000000 ) ) ;
#82550=CARTESIAN_POINT ( 'NONE',  ( 2.638427012816829897, 14.55059781766744997, -9.846743663894592657 ) ) ;
#82552=ORIENTED_EDGE ( 'NONE', *, *, #30255, .F. ) ;
#82555=VECTOR ( 'NONE', #9941, 1000.000000000000114 ) ;
#82564=AXIS2_PLACEMENT_3D ( 'NONE', #90567, #39067, #14602 ) ;
#82567=ORIENTED_EDGE ( 'NONE', *, *, #62672, .F. ) ;
#82570=ORIENTED_EDGE ( 'NONE', *, *, #53750, .F. ) ;
#82577=CARTESIAN_POINT ( 'NONE',  ( -0.1034006766853582671, 15.00000000000000000, 14.49963131601234956 ) ) ;
#82581=ORIENTED_EDGE ( 'NONE', *, *, #36141, .T. ) ;
#82586=CARTESIAN_POINT ( 'NONE',  ( -11.28404003980378612, 12.70269222139743803, -2.038315274784799236 ) ) ;
#82587=CARTESIAN_POINT ( 'NONE',  ( 0.000000000000000000, 15.00000000000000000, 0.000000000000000000 ) ) ;
#82590=LINE ( 'NONE', #98108, #65833 ) ;
#82591=CARTESIAN_POINT ( 'NONE',  ( -8.731067818237036704, 4.063309369127505732, -8.731067818237033151 ) ) ;
#82593=CARTESIAN_POINT ( 'NONE',  ( -13.34343830728408697, 14.49999999999999822, 6.852200678592504701 ) ) ;
#82601=ORIENTED_EDGE ( 'NONE', *, *, #95856, .T. ) ;
#82609=CARTESIAN_POINT ( 'NONE',  ( 0.000000000000000000, 0.000000000000000000, 0.000000000000000000 ) ) ;
#82610=DIRECTION ( 'NONE',  ( -0.9366721892483995671, 0.000000000000000000, 0.3502073812594621027 ) ) ;
#82615=CARTESIAN_POINT ( 'NONE',  ( -2.915334737309917656, -10.89464798917849286, 10.88017736071110164 ) ) ;
#82617=CARTESIAN_POINT ( 'NONE',  ( 14.49440716394873618, 4.800686736885023475E-16, -0.4026921475166205244 ) ) ;
#82621=CIRCLE ( 'NONE', #7576, 15.00000000000000000 ) ;
#82622=LINE ( 'NONE', #74624, #80040 ) ;
#82641=CARTESIAN_POINT ( 'NONE',  ( 9.065164099344587001, 14.49999999999999112, -11.95084933600771038 ) ) ;
#82644=CARTESIAN_POINT ( 'NONE',  ( -0.3093388210927642268, 0.5000000000000004441, 14.99680997725065978 ) ) ;
#82646=ORIENTED_EDGE ( 'NONE', *, *, #13814, .F. ) ;
#82661=DIRECTION ( 'NONE',  ( 0.09584575252023383451, 0.000000000000000000, -0.9953961983671779645 ) ) ;
#82663=CIRCLE ( 'NONE', #36336, 14.49999999999999822 ) ;
#82664=CARTESIAN_POINT ( 'NONE',  ( -2.638427012816840111, -25.03273551566587685, -9.846743663894590881 ) ) ;
#82666=CARTESIAN_POINT ( 'NONE',  ( 13.61464873478162652, 0.5000000000000004441, 6.296136897217931683 ) ) ;
#82669=EDGE_LOOP ( 'NONE', ( #16625, #35588, #37883, #40263, #69136, #46158 ) ) ;
#82670=CARTESIAN_POINT ( 'NONE',  ( -11.22915323889568562, 15.00000000000000000, -8.773176023390764300 ) ) ;
#82675=CARTESIAN_POINT ( 'NONE',  ( 3.927832320392247389, 15.00000000000000000, -13.69797916712104602 ) ) ;
#82678=CARTESIAN_POINT ( 'NONE',  ( 9.382169495545415572, 17.24863466993042138, -9.382169495545422677 ) ) ;
#82679=ORIENTED_EDGE ( 'NONE', *, *, #88474, .T. ) ;
#82683=ORIENTED_EDGE ( 'NONE', *, *, #59050, .T. ) ;
#82693=AXIS2_PLACEMENT_3D ( 'NONE', #93671, #86182, #39707 ) ;
#82696=CARTESIAN_POINT ( 'NONE',  ( 0.000000000000000000, 0.000000000000000000, 0.000000000000000000 ) ) ;
#82698=CARTESIAN_POINT ( 'NONE',  ( -10.58521204051718101, 15.00000000000000000, -11.99294302885424024 ) ) ;
#82701=DIRECTION ( 'NONE',  ( -0.000000000000000000, -1.000000000000000000, -0.000000000000000000 ) ) ;
#82704=FACE_OUTER_BOUND ( 'NONE', #11733, .T. ) ;
#82709=CARTESIAN_POINT ( 'NONE',  ( -9.399392868737892925, 15.00000000000000000, 11.04089732309468097 ) ) ;
#82710=FACE_OUTER_BOUND ( 'NONE', #33931, .T. ) ;
#82712=LINE ( 'NONE', #20737, #77532 ) ;
#82716=B_SPLINE_CURVE_WITH_KNOTS ( 'NONE', 3,
 ( #50904, #7398, #37896, #53365, #92841, #23386 ),
 .UNSPECIFIED., .F., .F.,
 ( 4, 2, 4 ),
 ( 3.409110551495873193E-05, 0.0004400426677367972510, 0.0008459942299586357701 ),
 .UNSPECIFIED. ) ;
#82725=CARTESIAN_POINT ( 'NONE',  ( 11.92686044187656691, 5.162123368507804955, -2.602085213965210642E-15 ) ) ;
#82731=CARTESIAN_POINT ( 'NONE',  ( -3.795296366450300773, 17.84541550158062861, 14.16423886937410437 ) ) ;
#82737=EDGE_CURVE ( 'NONE', #87966, #37275, #73716, .T. ) ;
#82740=ORIENTED_EDGE ( 'NONE', *, *, #77235, .F. ) ;
#82745=DIRECTION ( 'NONE',  ( 0.9999619230641713097, 0.000000000000000000, 0.008726535498374266009 ) ) ;
#82747=CYLINDRICAL_SURFACE ( 'NONE', #79088, 15.00000000000000000 ) ;
#82748=CARTESIAN_POINT ( 'NONE',  ( 2.863845842055826818, 0.04922511925147237538, 14.47219703936415591 ) ) ;
#82751=ORIENTED_EDGE ( 'NONE', *, *, #87605, .F. ) ;
#82768=B_SPLINE_CURVE_WITH_KNOTS ( 'NONE', 3,
 ( #65923, #96451, #58415, #27923, #90392, #6917 ),
 .UNSPECIFIED., .F., .F.,
 ( 4, 2, 4 ),
 ( 0.0002800452451301706442, 0.0006862509172429716916, 0.001092456589355772847 ),
 .UNSPECIFIED. ) ;
#82771=CARTESIAN_POINT ( 'NONE',  ( 8.235571585149870089, 6.046802177851540172, -8.235571585149873641 ) ) ;
#82777=DIRECTION ( 'NONE',  ( 8.659560562354910671E-17, -0.7071067811865492381, 0.7071067811865457964 ) ) ;
#82784=ADVANCED_FACE ( 'NONE', ( #52805 ), #67544, .T. ) ;
#82786=ORIENTED_EDGE ( 'NONE', *, *, #36598, .F. ) ;
#82793=FACE_OUTER_BOUND ( 'NONE', #47561, .T. ) ;
#82794=ORIENTED_EDGE ( 'NONE', *, *, #78495, .T. ) ;
#82802=DIRECTION ( 'NONE',  ( 0.000000000000000000, 0.000000000000000000, 1.000000000000000000 ) ) ;
#82809=ORIENTED_EDGE ( 'NONE', *, *, #68966, .T. ) ;
#82812=CARTESIAN_POINT ( 'NONE',  ( -1.326515405096241107, 0.2306972965111871998, 14.88215077106014306 ) ) ;
#82818=CARTESIAN_POINT ( 'NONE',  ( 0.000000000000000000, 0.5000000000000004441, 0.000000000000000000 ) ) ;
#82825=AXIS2_PLACEMENT_3D ( 'NONE', #62608, #41127, #18127 ) ;
#82830=VECTOR ( 'NONE', #80950, 999.9999999999998863 ) ;
#82839=EDGE_CURVE ( 'NONE', #81238, #74503, #68319, .T. ) ;
#82840=LINE ( 'NONE', #59342, #2632 ) ;
#82853=CARTESIAN_POINT ( 'NONE',  ( -14.67697702673046933, -0.03417435944610275333, 6.361111679013309761 ) ) ;
#82857=EDGE_CURVE ( 'NONE', #34814, #42118, #45189, .T. ) ;
#82862=DIRECTION ( 'NONE',  ( 0.000000000000000000, 0.000000000000000000, 1.000000000000000000 ) ) ;
#82865=EDGE_CURVE ( 'NONE', #16073, #74198, #33162, .T. ) ;
#82875=ORIENTED_EDGE ( 'NONE', *, *, #30256, .F. ) ;
#82877=LINE ( 'NONE', #75366, #12714 ) ;
#82880=CARTESIAN_POINT ( 'NONE',  ( -9.972640495195461696, 15.00000000000000000, 12.50695158660338890 ) ) ;
#82886=CARTESIAN_POINT ( 'NONE',  ( -3.193136578976892626, 15.00000000000000888, -14.27383009353655119 ) ) ;
#82891=CARTESIAN_POINT ( 'NONE',  ( 5.448048636097845510, 0.000000000000000000, -0.2378669404634490003 ) ) ;
#82899=EDGE_CURVE ( 'NONE', #77019, #23582, #69796, .T. ) ;
#82904=VERTEX_POINT ( 'NONE', #344 ) ;
#82906=VECTOR ( 'NONE', #35063, 1000.000000000000000 ) ;
#82909=DIRECTION ( 'NONE',  ( 0.000000000000000000, 0.000000000000000000, 1.000000000000000000 ) ) ;
#82919=DIRECTION ( 'NONE',  ( 0.6360782202777648386, 0.000000000000000000, 0.7716245833877193316 ) ) ;
#82925=CARTESIAN_POINT ( 'NONE',  ( -12.81628187352647608, -15.87636533006957507, 3.903127820947815962E-15 ) ) ;
#82936=CARTESIAN_POINT ( 'NONE',  ( -14.66196617519561052, 14.76930270348882068, 2.874856965127719377 ) ) ;
#82944=B_SPLINE_CURVE_WITH_KNOTS ( 'NONE', 3,
 ( #23625, #38128, #68616, #22132, #60607, #91101 ),
 .UNSPECIFIED., .F., .F.,
 ( 4, 2, 4 ),
 ( 0.0002800715030460580518, 0.0006862774322447752397, 0.001092483361443492536 ),
 .UNSPECIFIED. ) ;
#82955=LINE ( 'NONE', #21975, #53722 ) ;
#82959=CARTESIAN_POINT ( 'NONE',  ( 0.000000000000000000, 15.00000000000000000, 0.000000000000000000 ) ) ;
#82970=CARTESIAN_POINT ( 'NONE',  ( 14.52941021839284375, -2.151463686025920889E-16, 1.683622718073147562 ) ) ;
#82981=CARTESIAN_POINT ( 'NONE',  ( 14.16423886937410082, -25.48791783175269643, -3.795296366450314096 ) ) ;
#82984=EDGE_CURVE ( 'NONE', #82423, #51651, #64300, .T. ) ;
#82986=ORIENTED_EDGE ( 'NONE', *, *, #66249, .F. ) ;
#82998=CARTESIAN_POINT ( 'NONE',  ( -2.915334737309917656, 29.10535201082149825, 10.88017736071110164 ) ) ;
#83003=CARTESIAN_POINT ( 'NONE',  ( -14.82269085861170232, 0.5000000000000004441, 2.299529454046861154 ) ) ;
#83009=DIRECTION ( 'NONE',  ( -0.9999619230641713097, 0.000000000000000000, 0.008726535498367547425 ) ) ;
#83014=CARTESIAN_POINT ( 'NONE',  ( 14.24131928502211686, -0.03417435944610275333, -0.4973178280105898241 ) ) ;
#83017=ORIENTED_EDGE ( 'NONE', *, *, #9622, .F. ) ;
#83033=VERTEX_POINT ( 'NONE', #17291 ) ;
#83034=ORIENTED_EDGE ( 'NONE', *, *, #35977, .T. ) ;
#83039=CARTESIAN_POINT ( 'NONE',  ( -4.096035146093331747, 15.00000000000000000, -13.90943910019262653 ) ) ;
#83047=CARTESIAN_POINT ( 'NONE',  ( 9.846743663894594434, 18.50893115100080166, -2.168404344971008868E-15 ) ) ;
#83059=VERTEX_POINT ( 'NONE', #72232 ) ;
#83069=EDGE_CURVE ( 'NONE', #3928, #42348, #49813, .T. ) ;
#83074=CARTESIAN_POINT ( 'NONE',  ( 4.922013193295424749, 0.000000000000000000, 2.347679864819481654 ) ) ;
#83077=ORIENTED_EDGE ( 'NONE', *, *, #75076, .F. ) ;
#83082=CARTESIAN_POINT ( 'NONE',  ( 0.000000000000000000, 0.000000000000000000, 0.000000000000000000 ) ) ;
#83084=CARTESIAN_POINT ( 'NONE',  ( 1.114591949025029338, 4.390405144365474573E-16, -14.45709807627964416 ) ) ;
#83088=CARTESIAN_POINT ( 'NONE',  ( 10.93781366033349833, 14.49999999999999112, -10.26470809774071569 ) ) ;
#83094=EDGE_CURVE ( 'NONE', #58939, #84500, #85092, .T. ) ;
#83097=EDGE_CURVE ( 'NONE', #4700, #43197, #18761, .T. ) ;
#83103=CARTESIAN_POINT ( 'NONE',  ( 0.000000000000000000, 14.49999999999999822, 0.000000000000000000 ) ) ;
#83105=CARTESIAN_POINT ( 'NONE',  ( 7.002992508389039195, 15.00000000000000533, -12.84003923133018077 ) ) ;
#83106=DIRECTION ( 'NONE',  ( -0.000000000000000000, 1.000000000000000000, 0.000000000000000000 ) ) ;
#83109=CARTESIAN_POINT ( 'NONE',  ( 3.469446951953614189E-15, -15.68631465584515539, 10.88017736071110342 ) ) ;
#83114=LINE ( 'NONE', #145, #22685 ) ;
#83124=VECTOR ( 'NONE', #24972, 1000.000000000000000 ) ;
#83126=ORIENTED_EDGE ( 'NONE', *, *, #92578, .F. ) ;
#83128=PLANE ( 'NONE',  #87640 ) ;
#83129=EDGE_CURVE ( 'NONE', #49599, #41530, #17778, .T. ) ;
#83137=DIRECTION ( 'NONE',  ( 0.000000000000000000, 1.000000000000000000, 0.000000000000000000 ) ) ;
#83138=VECTOR ( 'NONE', #80707, 1000.000000000000114 ) ;
#83142=ORIENTED_EDGE ( 'NONE', *, *, #50795, .F. ) ;
#83144=DIRECTION ( 'NONE',  ( -0.3173046564050965856, 0.000000000000000000, 0.9483236552061978797 ) ) ;
#83159=CARTESIAN_POINT ( 'NONE',  ( -7.208316651077764980, -19.61606884899921255, -7.208316651077759651 ) ) ;
#83161=DIRECTION ( 'NONE',  ( 0.000000000000000000, 0.000000000000000000, -1.000000000000000000 ) ) ;
#83164=EDGE_LOOP ( 'NONE', ( #11950, #92771, #89219, #81438 ) ) ;
#83171=CARTESIAN_POINT ( 'NONE',  ( -2.189108318723844704, 15.00000000000000178, 14.46085460646896870 ) ) ;
#83174=CARTESIAN_POINT ( 'NONE',  ( 12.81628187352647608, 16.41530133659708923, 3.434112377981052511 ) ) ;
#83188=ADVANCED_FACE ( 'NONE', ( #78265 ), #40277, .T. ) ;
#83190=CIRCLE ( 'NONE', #95979, 15.00000000000000000 ) ;
#83193=DIRECTION ( 'NONE',  ( -0.9099612708765455471, 0.000000000000000000, 0.4146932426562339735 ) ) ;
#83194=DIRECTION ( 'NONE',  ( 0.000000000000000000, 0.000000000000000000, 1.000000000000000000 ) ) ;
#83195=ORIENTED_EDGE ( 'NONE', *, *, #73651, .F. ) ;
#83201=CARTESIAN_POINT ( 'NONE',  ( -6.382347221874512755, 0.5000000000000004441, 13.57444820018223375 ) ) ;
#83204=CARTESIAN_POINT ( 'NONE',  ( -5.419894505350392855, 15.00000000000000000, -13.98659156302466045 ) ) ;
#83215=LINE ( 'NONE', #44714, #57103 ) ;
#83219=EDGE_CURVE ( 'NONE', #90159, #14667, #64142, .T. ) ;
#83220=DIRECTION ( 'NONE',  ( 0.000000000000000000, 1.000000000000000000, 0.000000000000000000 ) ) ;
#83229=CARTESIAN_POINT ( 'NONE',  ( -3.927832320392339316, -0.03417435944610275333, 13.69797916712101404 ) ) ;
#83230=CARTESIAN_POINT ( 'NONE',  ( 10.36894250292379027, 13.67874883491396254, 10.36894250292378672 ) ) ;
#83234=DIRECTION ( 'NONE',  ( 0.000000000000000000, 1.000000000000000000, 0.000000000000000000 ) ) ;
#83246=CARTESIAN_POINT ( 'NONE',  ( -11.62719953690073282, 0.3639310419529863116, 9.476720473301741166 ) ) ;
#83248=DIRECTION ( 'NONE',  ( -0.3665012267243009103, 0.000000000000000000, 0.9304175679820230194 ) ) ;
#83251=ORIENTED_EDGE ( 'NONE', *, *, #63713, .T. ) ;
#83254=CARTESIAN_POINT ( 'NONE',  ( -14.76044511231987322, 14.76984987353748835, 2.313329003771987136 ) ) ;
#83269=CARTESIAN_POINT ( 'NONE',  ( 11.81378540890936080, 15.00000000000000000, -7.968498874458115999 ) ) ;
#83274=CARTESIAN_POINT ( 'NONE',  ( 0.000000000000000000, 15.00000000000000000, 0.000000000000000000 ) ) ;
#83286=ORIENTED_EDGE ( 'NONE', *, *, #36054, .T. ) ;
#83292=CARTESIAN_POINT ( 'NONE',  ( 3.836325488036175457, 14.49999999999999112, -14.50112432709429378 ) ) ;
#83295=ORIENTED_EDGE ( 'NONE', *, *, #16157, .F. ) ;
#83302=CARTESIAN_POINT ( 'NONE',  ( 0.000000000000000000, 15.00000000000000000, 0.000000000000000000 ) ) ;
#83306=EDGE_CURVE ( 'NONE', #40720, #76622, #98740, .T. ) ;
#83307=ORIENTED_EDGE ( 'NONE', *, *, #49054, .T. ) ;
#83310=CARTESIAN_POINT ( 'NONE',  ( 0.000000000000000000, 0.5000000000000004441, 0.000000000000000000 ) ) ;
#83312=CARTESIAN_POINT ( 'NONE',  ( 0.000000000000000000, 0.5000000000000004441, 0.000000000000000000 ) ) ;
#83319=DIRECTION ( 'NONE',  ( 0.000000000000000000, 0.000000000000000000, 1.000000000000000000 ) ) ;
#83330=ORIENTED_EDGE ( 'NONE', *, *, #83097, .F. ) ;
#83331=AXIS2_PLACEMENT_3D ( 'NONE', #21436, #28436, #65440 ) ;
#83333=ADVANCED_FACE ( 'NONE', ( #62766 ), #86760, .T. ) ;
#83342=LINE ( 'NONE', #23347, #5651 ) ;
#83355=B_SPLINE_CURVE_WITH_KNOTS ( 'NONE', 3,
 ( #65584, #19607, #2298, #4127, #13085, #74074 ),
 .UNSPECIFIED., .F., .F.,
 ( 4, 2, 4 ),
 ( 3.409110551361852929E-05, 0.0004400426677354470398, 0.0008459942299572755300 ),
 .UNSPECIFIED. ) ;
#83367=VERTEX_POINT ( 'NONE', #97237 ) ;
#83369=LINE ( 'NONE', #14391, #3981 ) ;
#83370=LINE ( 'NONE', #37393, #38295 ) ;
#83375=CARTESIAN_POINT ( 'NONE',  ( 0.000000000000000000, 14.49999999999999822, 0.000000000000000000 ) ) ;
#83380=CARTESIAN_POINT ( 'NONE',  ( -5.815488105659849083, 0.2301500539507708720, 13.76235181012714293 ) ) ;
#83383=EDGE_CURVE ( 'NONE', #935, #75686, #8044, .T. ) ;
#83386=VECTOR ( 'NONE', #36059, 1000.000000000000114 ) ;
#83401=EDGE_LOOP ( 'NONE', ( #62699, #89064, #47218, #39701, #42286, #87592 ) ) ;
#83411=CARTESIAN_POINT ( 'NONE',  ( -14.47650479471820439, 14.63606881343827126, -3.928206833722228453 ) ) ;
#83417=CARTESIAN_POINT ( 'NONE',  ( -14.93875075227017213, 14.76984974223857172, 0.2365588874158334465 ) ) ;
#83422=CARTESIAN_POINT ( 'NONE',  ( 9.382169495545415572, -17.75136533006957862, -9.382169495545422677 ) ) ;
#83423=AXIS2_PLACEMENT_3D ( 'NONE', #88890, #66374, #96908 ) ;
#83433=ADVANCED_FACE ( 'NONE', ( #43210 ), #19729, .F. ) ;
#83439=ORIENTED_EDGE ( 'NONE', *, *, #25771, .F. ) ;
#83444=CARTESIAN_POINT ( 'NONE',  ( 14.43100913237647731, 15.00000000000000000, -1.412789942450803027 ) ) ;
#83450=VERTEX_POINT ( 'NONE', #42733 ) ;
#83458=EDGE_CURVE ( 'NONE', #7455, #37030, #27717, .T. ) ;
#83472=CARTESIAN_POINT ( 'NONE',  ( -9.876730923139158236, 14.63595249122788999, -11.28938378619077376 ) ) ;
#83475=CARTESIAN_POINT ( 'NONE',  ( 10.36894250292378850, -20.07125116508603213, -10.36894250292379027 ) ) ;
#83476=CIRCLE ( 'NONE', #22815, 14.49999999999999822 ) ;
#83480=ORIENTED_EDGE ( 'NONE', *, *, #55648, .T. ) ;
#83485=AXIS2_PLACEMENT_3D ( 'NONE', #80733, #57233, #56747 ) ;
#83487=AXIS2_PLACEMENT_3D ( 'NONE', #21488, #98000, #51985 ) ;
#83488=LINE ( 'NONE', #45984, #49674 ) ;
#83492=FACE_OUTER_BOUND ( 'NONE', #14068, .T. ) ;
#83494=CARTESIAN_POINT ( 'NONE',  ( -5.440088680355547268, 28.89701867748817321, 9.422509992056143702 ) ) ;
#83497=CIRCLE ( 'NONE', #81824, 15.00000000000000000 ) ;
#83505=DIRECTION ( 'NONE',  ( 0.000000000000000000, 0.000000000000000000, 1.000000000000000000 ) ) ;
#83510=DIRECTION ( 'NONE',  ( 0.000000000000000000, 0.000000000000000000, -1.000000000000000000 ) ) ;
#83513=VERTEX_POINT ( 'NONE', #51215 ) ;
#83523=DIRECTION ( 'NONE',  ( 0.000000000000000000, 0.000000000000000000, 1.000000000000000000 ) ) ;
#83525=AXIS2_PLACEMENT_3D ( 'NONE', #34143, #3681, #49640 ) ;
#83535=CARTESIAN_POINT ( 'NONE',  ( 3.836325488036079534, 14.63606917487430970, 14.50112432709429378 ) ) ;
#83540=CARTESIAN_POINT ( 'NONE',  ( 12.03829478939427666, 15.00000000000000888, -8.307695547791400514 ) ) ;
#83543=CARTESIAN_POINT ( 'NONE',  ( 4.923371831947301658, 12.67559781766745886, 8.527530157486175710 ) ) ;
#83545=ORIENTED_EDGE ( 'NONE', *, *, #98535, .F. ) ;
#83546=CARTESIAN_POINT ( 'NONE',  ( 0.04758788293972446987, 0.000000000000000000, -5.453031268574422441 ) ) ;
#83556=EDGE_CURVE ( 'NONE', #88170, #56402, #21212, .T. ) ;
#83559=ORIENTED_EDGE ( 'NONE', *, *, #70129, .T. ) ;
#83570=VECTOR ( 'NONE', #36841, 1000.000000000000000 ) ;
#83572=DIRECTION ( 'NONE',  ( 0.000000000000000000, 0.000000000000000000, -1.000000000000000000 ) ) ;
#83574=VERTEX_POINT ( 'NONE', #89701 ) ;
#83576=ORIENTED_EDGE ( 'NONE', *, *, #33865, .T. ) ;
#83595=ADVANCED_FACE ( 'NONE', ( #57227 ), #77090, .T. ) ;
#83596=LINE ( 'NONE', #67612, #509 ) ;
#83600=VERTEX_POINT ( 'NONE', #91682 ) ;
#83608=CARTESIAN_POINT ( 'NONE',  ( -9.997910040112463648, 15.00000000000000000, -10.50199004140731773 ) ) ;
#83612=CARTESIAN_POINT ( 'NONE',  ( -2.915334737309934532, -17.97798132251182324, -10.88017736071109987 ) ) ;
#83616=CARTESIAN_POINT ( 'NONE',  ( 14.43100913236846772, 15.00000000000000000, 1.412789942453269054 ) ) ;
#83617=CARTESIAN_POINT ( 'NONE',  ( -14.62617646268082972, 0.5000000000000004441, -3.327906561567078647 ) ) ;
#83626=CARTESIAN_POINT ( 'NONE',  ( -9.876730923139378504, 0.5000000000000004441, 11.28938378619056415 ) ) ;
#83632=PLANE ( 'NONE',  #76454 ) ;
#83637=DIRECTION ( 'NONE',  ( 0.6755902076156493630, 0.000000000000000000, 0.7372773368101340763 ) ) ;
#83643=ORIENTED_EDGE ( 'NONE', *, *, #7626, .F. ) ;
#83655=CARTESIAN_POINT ( 'NONE',  ( -6.689969769699040114, 15.00000000000000000, 12.58200319823965785 ) ) ;
#83657=CARTESIAN_POINT ( 'NONE',  ( 9.846743663894590881, -26.69940218233254470, 2.638427012816828565 ) ) ;
#83659=DIRECTION ( 'NONE',  ( -0.2503800040544453820, 0.000000000000000000, 0.9681476403781066331 ) ) ;
#83661=DIRECTION ( 'NONE',  ( 0.000000000000000000, 1.000000000000000000, 0.000000000000000000 ) ) ;
#83671=EDGE_CURVE ( 'NONE', #34469, #48237, #92665, .T. ) ;
#83672=CARTESIAN_POINT ( 'NONE',  ( -12.81628187352647963, 23.91530133659708213, -3.434112377981046293 ) ) ;
#83674=VERTEX_POINT ( 'NONE', #92173 ) ;
#83686=CARTESIAN_POINT ( 'NONE',  ( 3.469446951953614189E-15, 3.912123368507817833, 11.92686044187656513 ) ) ;
#83694=DIRECTION ( 'NONE',  ( 0.000000000000000000, 0.000000000000000000, 1.000000000000000000 ) ) ;
#83699=CARTESIAN_POINT ( 'NONE',  ( -10.64017930668218881, 14.49999999999999112, 10.57291749337211151 ) ) ;
#83700=CARTESIAN_POINT ( 'NONE',  ( -5.451370222425315326, 0.000000000000000000, 0.1427491530889740401 ) ) ;
#83701=DIRECTION ( 'NONE',  ( 0.000000000000000000, 1.000000000000000000, 0.000000000000000000 ) ) ;
#83705=PLANE ( 'NONE',  #52759 ) ;
#83711=DIRECTION ( 'NONE',  ( 0.9170600743851238246, 0.000000000000000000, -0.3987490689252466414 ) ) ;
#83713=ORIENTED_EDGE ( 'NONE', *, *, #74478, .F. ) ;
#83718=DIRECTION ( 'NONE',  ( 0.5519369853120560387, 0.000000000000000000, 0.8338858220671695465 ) ) ;
#83727=CARTESIAN_POINT ( 'NONE',  ( -12.26659068614895354, 16.38708216824731068, -7.082119434687038861 ) ) ;
#83731=VECTOR ( 'NONE', #30748, 1000.000000000000227 ) ;
#83736=ORIENTED_EDGE ( 'NONE', *, *, #21475, .F. ) ;
#83741=FACE_OUTER_BOUND ( 'NONE', #47883, .T. ) ;
#83753=DIRECTION ( 'NONE',  ( 0.000000000000000000, 1.000000000000000000, 0.000000000000000000 ) ) ;
#83756=DIRECTION ( 'NONE',  ( 0.000000000000000000, 1.000000000000000000, 0.000000000000000000 ) ) ;
#83760=B_SPLINE_CURVE_WITH_KNOTS ( 'NONE', 3,
 ( #29520, #44539, #76024, #37551, #7555, #83039 ),
 .UNSPECIFIED., .F., .F.,
 ( 4, 2, 4 ),
 ( 3.409110551494652110E-05, 0.0004400426677367922637, 0.0008459942299586379385 ),
 .UNSPECIFIED. ) ;
#83761=ORIENTED_EDGE ( 'NONE', *, *, #39371, .T. ) ;
#83762=EDGE_LOOP ( 'NONE', ( #85366, #6211, #35089, #56031 ) ) ;
#83777=ORIENTED_EDGE ( 'NONE', *, *, #71070, .T. ) ;
#83781=ORIENTED_EDGE ( 'NONE', *, *, #95894, .F. ) ;
#83785=CARTESIAN_POINT ( 'NONE',  ( 3.897244926436223444, 15.00000000000000000, -13.96644127841327787 ) ) ;
#83790=B_SPLINE_CURVE_WITH_KNOTS ( 'NONE', 3,
 ( #63135, #47143, #56144, #25172, #9157, #25651 ),
 .UNSPECIFIED., .F., .F.,
 ( 4, 2, 4 ),
 ( 3.252606517456513784E-19, 0.0004056965545342626793, 0.0008113931090685250333 ),
 .UNSPECIFIED. ) ;
#83792=EDGE_LOOP ( 'NONE', ( #64741, #2170, #42566, #70423, #49149, #11180 ) ) ;
#83794=DIRECTION ( 'NONE',  ( 0.000000000000000000, 1.000000000000000000, 0.000000000000000000 ) ) ;
#83795=ORIENTED_EDGE ( 'NONE', *, *, #93272, .T. ) ;
#83800=LINE ( 'NONE', #68312, #14343 ) ;
#83804=ORIENTED_EDGE ( 'NONE', *, *, #79517, .F. ) ;
#83805=CARTESIAN_POINT ( 'NONE',  ( -7.154372922009654800, -0.03417435944610275333, 14.30707323420372035 ) ) ;
#83821=CARTESIAN_POINT ( 'NONE',  ( 7.551349515323100725, -0.03417435944610275333, 12.08468537022911349 ) ) ;
#83830=AXIS2_PLACEMENT_3D ( 'NONE', #20360, #73842, #97859 ) ;
#83832=DIRECTION ( 'NONE',  ( -0.000000000000000000, 1.000000000000000000, -0.000000000000000000 ) ) ;
#83842=DIRECTION ( 'NONE',  ( 0.4305110968083047940, 0.000000000000000000, -0.9025852843498560762 ) ) ;
#83844=CARTESIAN_POINT ( 'NONE',  ( 0.000000000000000000, 0.000000000000000000, 0.000000000000000000 ) ) ;
#83853=CARTESIAN_POINT ( 'NONE',  ( 4.265659168453209915, 14.95077488074853456, 14.12268572233453590 ) ) ;
#83862=CARTESIAN_POINT ( 'NONE',  ( -11.29222593019763288, 14.76930270348881535, -9.783848334571407790 ) ) ;
#83868=CARTESIAN_POINT ( 'NONE',  ( 14.61046065509105674, -2.732951804315999255E-15, -0.6655452423542743690 ) ) ;
#83872=CARTESIAN_POINT ( 'NONE',  ( 5.419894505350628222, 14.49999999999999112, -13.98659156302463735 ) ) ;
#83873=CARTESIAN_POINT ( 'NONE',  ( -11.92686044187656513, 2.662123368507809840, 3.903127820947815962E-15 ) ) ;
#83875=VECTOR ( 'NONE', #76814, 1000.000000000000000 ) ;
#83886=CARTESIAN_POINT ( 'NONE',  ( -13.78891971893199830, 0.5000000000000004441, -5.904717858191724567 ) ) ;
#83897=CIRCLE ( 'NONE', #40791, 14.49999999999999822 ) ;
#83908=DIRECTION ( 'NONE',  ( -5.240252676230738871E-14, 0.000000000000000000, 1.000000000000000000 ) ) ;
#83912=CARTESIAN_POINT ( 'NONE',  ( -11.09922568453594316, -0.4596986634029104346, 6.408140936763246920 ) ) ;
#83932=DIRECTION ( 'NONE',  ( 0.000000000000000000, 0.000000000000000000, 1.000000000000000000 ) ) ;
#83933=VECTOR ( 'NONE', #82227, 1000.000000000000114 ) ;
#83939=FACE_OUTER_BOUND ( 'NONE', #8301, .T. ) ;
#83941=ORIENTED_EDGE ( 'NONE', *, *, #65715, .F. ) ;
#83943=CARTESIAN_POINT ( 'NONE',  ( 11.42945456197617915, 15.00000000000000711, -9.127207413380702405 ) ) ;
#83945=CIRCLE ( 'NONE', #40843, 14.49999999999999822 ) ;
#83948=CARTESIAN_POINT ( 'NONE',  ( 11.42945456197613119, 1.694065894508600678E-16, 9.127207413380800105 ) ) ;
#83959=DIRECTION ( 'NONE',  ( -0.5372996083468194461, 0.000000000000000000, -0.8433914458128884961 ) ) ;
#83961=CARTESIAN_POINT ( 'NONE',  ( 14.37564666802075131, -2.797749824780953231E-15, -2.692451322017675786 ) ) ;
#83963=CARTESIAN_POINT ( 'NONE',  ( 3.795296366450314540, -6.737917831752698206, 14.16423886937410082 ) ) ;
#83967=CIRCLE ( 'NONE', #61607, 14.49999999999999822 ) ;
#83970=EDGE_LOOP ( 'NONE', ( #66295, #76086, #71640, #81797 ) ) ;
#83972=AXIS2_PLACEMENT_3D ( 'NONE', #35914, #96943, #66411 ) ;
#83977=CARTESIAN_POINT ( 'NONE',  ( 2.863771337576428433, 14.95037103301162063, 14.47259902956231770 ) ) ;
#83979=DIRECTION ( 'NONE',  ( -0.000000000000000000, 1.000000000000000000, -0.000000000000000000 ) ) ;
#83980=DIRECTION ( 'NONE',  ( 0.000000000000000000, 1.000000000000000000, 0.000000000000000000 ) ) ;
#83983=CARTESIAN_POINT ( 'NONE',  ( -9.422509992056136596, 28.48035201082149825, 5.440088680355559703 ) ) ;
#83990=VERTEX_POINT ( 'NONE', #62144 ) ;
#83992=ADVANCED_FACE ( 'NONE', ( #77647 ), #59597, .T. ) ;
#83997=ADVANCED_FACE ( 'NONE', ( #1197 ), #24519, .T. ) ;
#84002=CARTESIAN_POINT ( 'NONE',  ( 0.000000000000000000, 15.00000000000000000, 14.25000000000000000 ) ) ;
#84015=DIRECTION ( 'NONE',  ( 0.9981347984218670311, 0.000000000000000000, -0.06104853953485662316 ) ) ;
#84017=VECTOR ( 'NONE', #67147, 999.9999999999998863 ) ;
#84020=LINE ( 'NONE', #31000, #37651 ) ;
#84028=DIRECTION ( 'NONE',  ( 0.000000000000000000, 0.000000000000000000, 1.000000000000000000 ) ) ;
#84035=EDGE_CURVE ( 'NONE', #14939, #69916, #2677, .T. ) ;
#84036=CARTESIAN_POINT ( 'NONE',  ( -4.923371831947292776, 31.84226448433413736, 8.527530157486181039 ) ) ;
#84037=ORIENTED_EDGE ( 'NONE', *, *, #79922, .F. ) ;
#84038=DIRECTION ( 'NONE',  ( 0.000000000000000000, 1.000000000000000000, 0.000000000000000000 ) ) ;
#84054=ORIENTED_EDGE ( 'NONE', *, *, #9865, .F. ) ;
#84060=DIRECTION ( 'NONE',  ( 0.000000000000000000, 0.000000000000000000, 1.000000000000000000 ) ) ;
#84063=EDGE_CURVE ( 'NONE', #45054, #52174, #16516, .T. ) ;
#84067=ORIENTED_EDGE ( 'NONE', *, *, #20131, .F. ) ;
#84069=AXIS2_PLACEMENT_3D ( 'NONE', #46805, #73106, #72615 ) ;
#84071=EDGE_LOOP ( 'NONE', ( #55562, #39584, #74036, #34104, #46156, #32238 ) ) ;
#84078=CARTESIAN_POINT ( 'NONE',  ( -8.209432707284690878, 0.5000000000000004441, -12.55409154915497183 ) ) ;
#84080=VERTEX_POINT ( 'NONE', #17173 ) ;
#84092=EDGE_LOOP ( 'NONE', ( #88569, #77988, #67679, #67564, #37755, #47532 ) ) ;
#84099=DIRECTION ( 'NONE',  ( 0.000000000000000000, 0.000000000000000000, 1.000000000000000000 ) ) ;
#84101=CARTESIAN_POINT ( 'NONE',  ( -14.29484424893239414, 0.2301500622783318739, -4.345072767107323486 ) ) ;
#84105=CARTESIAN_POINT ( 'NONE',  ( 9.422509992056141925, -9.852981322511819684, 5.440088680355547268 ) ) ;
#84107=CARTESIAN_POINT ( 'NONE',  ( 13.50171220565087182, -3.186537947570676692E-15, -5.622479820943826034 ) ) ;
#84110=DIRECTION ( 'NONE',  ( 0.3665012267243071276, 0.000000000000000000, -0.9304175679820205769 ) ) ;
#84112=CARTESIAN_POINT ( 'NONE',  ( -14.97687855664615064, 14.49999999999999112, 0.8325315005899805998 ) ) ;
#84126=VERTEX_POINT ( 'NONE', #44449 ) ;
#84130=CARTESIAN_POINT ( 'NONE',  ( 15.41943733314631793, -0.03417435944610275333, -4.256565371896342320 ) ) ;
#84139=AXIS2_PLACEMENT_3D ( 'NONE', #70942, #54922, #86908 ) ;
#84141=CARTESIAN_POINT ( 'NONE',  ( -1.114591949025130369, 3.902037737440774503E-16, 14.45709807627963706 ) ) ;
#84144=VERTEX_POINT ( 'NONE', #52449 ) ;
#84152=CARTESIAN_POINT ( 'NONE',  ( 0.000000000000000000, 14.49999999999999822, 0.000000000000000000 ) ) ;
#84159=DIRECTION ( 'NONE',  ( 0.000000000000000000, 0.000000000000000000, 1.000000000000000000 ) ) ;
#84163=CARTESIAN_POINT ( 'NONE',  ( -9.846743663894596210, -29.19940218233254470, -2.638427012816824124 ) ) ;
#84164=ORIENTED_EDGE ( 'NONE', *, *, #492, .T. ) ;
#84174=CARTESIAN_POINT ( 'NONE',  ( -2.361121941889217979, 14.76984946027100243, 14.75287579053847509 ) ) ;
#84176=CARTESIAN_POINT ( 'NONE',  ( -3.434112377981047626, 15.16530133659708390, 12.81628187352647963 ) ) ;
#84187=CARTESIAN_POINT ( 'NONE',  ( 0.000000000000000000, 15.00000000000000000, 0.000000000000000000 ) ) ;
#84189=DIRECTION ( 'NONE',  ( 0.000000000000000000, 1.000000000000000000, 0.000000000000000000 ) ) ;
#84200=ORIENTED_EDGE ( 'NONE', *, *, #68363, .F. ) ;
#84202=CARTESIAN_POINT ( 'NONE',  ( -0.7375392941516176748, 15.00000000000000000, -14.98185688723471820 ) ) ;
#84207=CARTESIAN_POINT ( 'NONE',  ( -4.391347328463997002, 14.76984910450705257, 14.28069739540189254 ) ) ;
#84218=CARTESIAN_POINT ( 'NONE',  ( -3.195792623639539531, 6.620456701841148650, -11.92686044187656513 ) ) ;
#84225=CARTESIAN_POINT ( 'NONE',  ( -7.684764310694977674, 0.3639308364404307827, 12.88194075009933393 ) ) ;
#84231=CARTESIAN_POINT ( 'NONE',  ( 7.082119434687054849, 23.47041550158063217, 12.26659068614894288 ) ) ;
#84233=EDGE_CURVE ( 'NONE', #30157, #42828, #66460, .T. ) ;
#84235=CARTESIAN_POINT ( 'NONE',  ( 2.261421327065715303, 0.000000000000000000, 4.962236210031257144 ) ) ;
#84241=EDGE_CURVE ( 'NONE', #61376, #7648, #61668, .T. ) ;
#84242=ORIENTED_EDGE ( 'NONE', *, *, #24656, .F. ) ;
#84247=CARTESIAN_POINT ( 'NONE',  ( 14.71525861348287734, 0.5000000000000004441, 2.908807992686682109 ) ) ;
#84254=ORIENTED_EDGE ( 'NONE', *, *, #65117, .F. ) ;
#84263=CARTESIAN_POINT ( 'NONE',  ( 5.806645064956438063, 8.233160247311797324E-16, 13.42464971017000330 ) ) ;
#84277=CARTESIAN_POINT ( 'NONE',  ( 14.35840480524198171, 14.63595249122788999, 4.340070442838947606 ) ) ;
#84282=ADVANCED_FACE ( 'NONE', ( #7462 ), #76920, .F. ) ;
#84285=ORIENTED_EDGE ( 'NONE', *, *, #85831, .F. ) ;
#84287=ORIENTED_EDGE ( 'NONE', *, *, #6093, .T. ) ;
#84288=VECTOR ( 'NONE', #74351, 1000.000000000000000 ) ;
#84302=ORIENTED_EDGE ( 'NONE', *, *, #18604, .F. ) ;
#84307=CARTESIAN_POINT ( 'NONE',  ( 0.000000000000000000, 0.5000000000000004441, 0.000000000000000000 ) ) ;
#84311=ORIENTED_EDGE ( 'NONE', *, *, #7626, .T. ) ;
#84323=CARTESIAN_POINT ( 'NONE',  ( 2.393480905993150998, 15.00000000000000000, -14.80781041047751323 ) ) ;
#84324=CARTESIAN_POINT ( 'NONE',  ( 0.000000000000000000, 15.00000000000000000, 0.000000000000000000 ) ) ;
#84327=CARTESIAN_POINT ( 'NONE',  ( 7.684764310694801814, 14.49999999999999112, 12.88194075009947248 ) ) ;
#84343=CIRCLE ( 'NONE', #12454, 14.49999999999999822 ) ;
#84345=DIRECTION ( 'NONE',  ( 0.000000000000000000, 0.000000000000000000, 1.000000000000000000 ) ) ;
#84350=AXIS2_PLACEMENT_3D ( 'NONE', #96315, #49797, #5311 ) ;
#84351=CARTESIAN_POINT ( 'NONE',  ( -12.60874940350938189, 3.923185800807110140E-16, -7.160268045227207168 ) ) ;
#84356=ADVANCED_FACE ( 'NONE', ( #1444 ), #89937, .T. ) ;
#84360=CARTESIAN_POINT ( 'NONE',  ( 11.36220558718857276, 15.00000000000000000, 9.008345252845320061 ) ) ;
#84370=CARTESIAN_POINT ( 'NONE',  ( 13.78891971893204271, 0.5000000000000004441, 5.904717858191622426 ) ) ;
#84371=CARTESIAN_POINT ( 'NONE',  ( 11.94720539484406707, 14.76930270348881535, 8.972309510150243028 ) ) ;
#84376=DIRECTION ( 'NONE',  ( 0.000000000000000000, 0.000000000000000000, 1.000000000000000000 ) ) ;
#84377=DIRECTION ( 'NONE',  ( -0.000000000000000000, -1.000000000000000000, -0.000000000000000000 ) ) ;
#84381=CARTESIAN_POINT ( 'NONE',  ( 5.147851794455788443, -2.778691583467731473E-15, 13.68970903997130328 ) ) ;
#84382=DIRECTION ( 'NONE',  ( -0.3007057995042635157, 0.000000000000000000, -0.9537169507482300412 ) ) ;
#84402=AXIS2_PLACEMENT_3D ( 'NONE', #96459, #6417, #36930 ) ;
#84406=CARTESIAN_POINT ( 'NONE',  ( 4.431036607602466759, 0.5000000000000004441, 14.33059365769913818 ) ) ;
#84410=CARTESIAN_POINT ( 'NONE',  ( -14.62617646268096827, 14.49999999999999112, 3.327906561566773558 ) ) ;
#84431=ORIENTED_EDGE ( 'NONE', *, *, #77720, .T. ) ;
#84442=LINE ( 'NONE', #37469, #63274 ) ;
#84445=DIRECTION ( 'NONE',  ( 0.9636304532086229502, 0.000000000000000000, -0.2672383760782571227 ) ) ;
#84456=CIRCLE ( 'NONE', #86025, 15.00000000000000000 ) ;
#84460=DIRECTION ( 'NONE',  ( 0.9366721892484018985, 0.000000000000000000, -0.3502073812594559410 ) ) ;
#84462=DIRECTION ( 'NONE',  ( -0.000000000000000000, -1.000000000000000000, -0.000000000000000000 ) ) ;
#84465=CARTESIAN_POINT ( 'NONE',  ( 12.26659068614894821, -11.11291783175269465, 7.082119434687044190 ) ) ;
#84470=ORIENTED_EDGE ( 'NONE', *, *, #63163, .T. ) ;
#84473=CARTESIAN_POINT ( 'NONE',  ( 1.796787675079331459, 0.2301501525782880253, -14.83218748772976525 ) ) ;
#84479=DIRECTION ( 'NONE',  ( 0.9762960071199360268, 0.000000000000000000, -0.2164396139380907191 ) ) ;
#84491=CARTESIAN_POINT ( 'NONE',  ( 13.03370038005726705, -0.03417435944610275333, -9.273621236547697322 ) ) ;
#84492=AXIS2_PLACEMENT_3D ( 'NONE', #37224, #67709, #98222 ) ;
#84497=CARTESIAN_POINT ( 'NONE',  ( 13.07661834287487501, -3.129363223631011419E-15, -6.550615570651680208 ) ) ;
#84498=DIRECTION ( 'NONE',  ( 0.000000000000000000, 0.000000000000000000, 1.000000000000000000 ) ) ;
#84500=VERTEX_POINT ( 'NONE', #54408 ) ;
#84506=DIRECTION ( 'NONE',  ( -0.000000000000000000, -1.000000000000000000, -0.000000000000000000 ) ) ;
#84509=DIRECTION ( 'NONE',  ( 0.000000000000000000, 0.000000000000000000, 1.000000000000000000 ) ) ;
#84531=CARTESIAN_POINT ( 'NONE',  ( 3.434112377981060948, -39.41803199673623936, 12.81628187352647430 ) ) ;
#84543=ORIENTED_EDGE ( 'NONE', *, *, #50576, .T. ) ;
#84555=CARTESIAN_POINT ( 'NONE',  ( -4.265659168453410643, 0.04922511925147263212, 14.12268572233449149 ) ) ;
#84560=ORIENTED_EDGE ( 'NONE', *, *, #3280, .T. ) ;
#84572=ORIENTED_EDGE ( 'NONE', *, *, #76963, .F. ) ;
#84578=DIRECTION ( 'NONE',  ( 0.000000000000000000, 1.000000000000000000, 0.000000000000000000 ) ) ;
#84585=ORIENTED_EDGE ( 'NONE', *, *, #13094, .T. ) ;
#84591=CARTESIAN_POINT ( 'NONE',  ( 9.402796353261127393, 0.5000000000000004441, -11.68706210897757103 ) ) ;
#84593=EDGE_CURVE ( 'NONE', #61703, #67320, #31408, .T. ) ;
#84594=PLANE ( 'NONE',  #59778 ) ;
#84595=VECTOR ( 'NONE', #90836, 1000.000000000000114 ) ;
#84599=CARTESIAN_POINT ( 'NONE',  ( 10.88017736071109987, -4.227981322511823237, -2.915334737309928315 ) ) ;
#84603=CARTESIAN_POINT ( 'NONE',  ( 8.375939845167756914, -0.03417435944610275333, -11.52849216984298941 ) ) ;
#84606=CARTESIAN_POINT ( 'NONE',  ( 0.000000000000000000, 15.00000000000000000, 0.000000000000000000 ) ) ;
#84610=FACE_OUTER_BOUND ( 'NONE', #61063, .T. ) ;
#84625=EDGE_LOOP ( 'NONE', ( #1297, #11381, #16510, #21317, #88719, #57924 ) ) ;
#84640=CARTESIAN_POINT ( 'NONE',  ( 2.638427012816829897, -5.449402182332544697, -9.846743663894592657 ) ) ;
#84641=VERTEX_POINT ( 'NONE', #38444 ) ;
#84642=CARTESIAN_POINT ( 'NONE',  ( -9.898881779040587858, -0.03417435944610275333, -10.25059215482589714 ) ) ;
#84645=ORIENTED_EDGE ( 'NONE', *, *, #63155, .T. ) ;
#84651=CARTESIAN_POINT ( 'NONE',  ( -13.61464873478165138, 14.49999999999999112, -6.296136897218031159 ) ) ;
#84655=VERTEX_POINT ( 'NONE', #23453 ) ;
#84657=ORIENTED_EDGE ( 'NONE', *, *, #71364, .F. ) ;
#84663=CARTESIAN_POINT ( 'NONE',  ( 10.27191093752554529, 15.00000000000000888, 10.41278984915632400 ) ) ;
#84666=ADVANCED_FACE ( 'NONE', ( #84920 ), #45436, .F. ) ;
#84667=CYLINDRICAL_SURFACE ( 'NONE', #34484, 15.00000000000000000 ) ;
#84668=ORIENTED_EDGE ( 'NONE', *, *, #29623, .T. ) ;
#84669=CARTESIAN_POINT ( 'NONE',  ( 0.000000000000000000, 0.5000000000000004441, 0.000000000000000000 ) ) ;
#84672=ORIENTED_EDGE ( 'NONE', *, *, #42248, .F. ) ;
#84673=EDGE_CURVE ( 'NONE', #36587, #96742, #93893, .T. ) ;
#84680=VERTEX_POINT ( 'NONE', #17905 ) ;
#84681=DIRECTION ( 'NONE',  ( -0.000000000000000000, -1.000000000000000000, -0.000000000000000000 ) ) ;
#84693=CARTESIAN_POINT ( 'NONE',  ( 12.58781651029199189, 15.00000000000000533, 7.446837378630806192 ) ) ;
#84694=VECTOR ( 'NONE', #49189, 1000.000000000000114 ) ;
#84697=ORIENTED_EDGE ( 'NONE', *, *, #93272, .F. ) ;
#84706=CARTESIAN_POINT ( 'NONE',  ( 5.963430220938287007, 4.328790035174473694, 10.32896413005679825 ) ) ;
#84707=AXIS2_PLACEMENT_3D ( 'NONE', #17969, #48455, #78953 ) ;
#84709=FACE_OUTER_BOUND ( 'NONE', #3382, .T. ) ;
#84712=CARTESIAN_POINT ( 'NONE',  ( -5.204170427930421283E-15, 25.55374883491398563, -14.16423886937410082 ) ) ;
#84714=AXIS2_PLACEMENT_3D ( 'NONE', #6696, #14709, #28698 ) ;
#84722=VERTEX_POINT ( 'NONE', #95367 ) ;
#84734=DIRECTION ( 'NONE',  ( -0.000000000000000000, 1.000000000000000000, -0.000000000000000000 ) ) ;
#84735=CARTESIAN_POINT ( 'NONE',  ( 14.36383853300408475, 14.95037103067321915, -3.367113227848937740 ) ) ;
#84744=AXIS2_PLACEMENT_3D ( 'NONE', #17088, #630, #84099 ) ;
#84747=ORIENTED_EDGE ( 'NONE', *, *, #6143, .F. ) ;
#84764=CARTESIAN_POINT ( 'NONE',  ( -14.26295192185813221, 14.95077488074853456, 3.770186020344923339 ) ) ;
#84772=VERTEX_POINT ( 'NONE', #34852 ) ;
#84779=CIRCLE ( 'NONE', #14564, 14.49999999999999822 ) ;
#84789=DIRECTION ( 'NONE',  ( -0.000000000000000000, -1.000000000000000000, -0.000000000000000000 ) ) ;
#84796=CARTESIAN_POINT ( 'NONE',  ( 9.742785792574936821, 12.20136696231599061, 5.624999999999996447 ) ) ;
#84799=DIRECTION ( 'NONE',  ( 0.1650476058606741014, 0.000000000000000000, 0.9862856015372319929 ) ) ;
#84806=ADVANCED_FACE ( 'NONE', ( #49370 ), #32891, .F. ) ;
#84807=AXIS2_PLACEMENT_3D ( 'NONE', #93303, #41798, #47302 ) ;
#84814=AXIS2_PLACEMENT_3D ( 'NONE', #38487, #13510, #43992 ) ;
#84820=EDGE_CURVE ( 'NONE', #25555, #39153, #2922, .T. ) ;
#84823=CARTESIAN_POINT ( 'NONE',  ( 9.641087339108837639, 14.95077488074853456, 11.16671550067055385 ) ) ;
#84832=TOROIDAL_SURFACE ( 'NONE', #60841, 14.49999999999999822, 0.5000000000000000000 ) ;
#84834=VERTEX_POINT ( 'NONE', #57362 ) ;
#84838=DIRECTION ( 'NONE',  ( 0.000000000000000000, 0.000000000000000000, 1.000000000000000000 ) ) ;
#84843=ORIENTED_EDGE ( 'NONE', *, *, #29798, .F. ) ;
#84846=ORIENTED_EDGE ( 'NONE', *, *, #93932, .F. ) ;
#84847=DIRECTION ( 'NONE',  ( 0.4617486132350345773, 0.000000000000000000, 0.8870108331782213806 ) ) ;
#84853=CARTESIAN_POINT ( 'NONE',  ( 9.641450013144471143, 14.95037107666755638, -11.16690429682349439 ) ) ;
#84859=VECTOR ( 'NONE', #13158, 1000.000000000000000 ) ;
#84866=CARTESIAN_POINT ( 'NONE',  ( -13.34343830728394309, 0.5000000000000004441, -6.852200678592783589 ) ) ;
#84878=VECTOR ( 'NONE', #39821, 999.9999999999998863 ) ;
#84879=EDGE_LOOP ( 'NONE', ( #72085, #36686, #29624, #30975, #66955, #42217 ) ) ;
#84880=ADVANCED_FACE ( 'NONE', ( #33371 ), #26362, .T. ) ;
#84883=VERTEX_POINT ( 'NONE', #3890 ) ;
#84891=CARTESIAN_POINT ( 'NONE',  ( -14.35840480524209894, 14.49999999999999112, 4.340070442838745102 ) ) ;
#84893=CARTESIAN_POINT ( 'NONE',  ( -13.75801628063875803, 4.618045246005505222E-16, -4.578972376164643698 ) ) ;
#84895=EDGE_LOOP ( 'NONE', ( #27807, #36317, #49362, #94184 ) ) ;
#84899=DIRECTION ( 'NONE',  ( 0.000000000000000000, 0.000000000000000000, 1.000000000000000000 ) ) ;
#84903=VECTOR ( 'NONE', #63553, 1000.000000000000000 ) ;
#84904=EDGE_CURVE ( 'NONE', #42454, #56421, #18393, .T. ) ;
#84906=CARTESIAN_POINT ( 'NONE',  ( 7.595945211628325922, 15.00000000000000000, -12.35117874301639240 ) ) ;
#84907=ORIENTED_EDGE ( 'NONE', *, *, #62317, .T. ) ;
#84910=EDGE_CURVE ( 'NONE', #42957, #18747, #25157, .T. ) ;
#84911=VECTOR ( 'NONE', #32852, 1000.000000000000000 ) ;
#84920=FACE_OUTER_BOUND ( 'NONE', #4000, .T. ) ;
#84925=ORIENTED_EDGE ( 'NONE', *, *, #70198, .T. ) ;
#84926=CARTESIAN_POINT ( 'NONE',  ( 2.913501739333757889, 3.989000423594319145E-16, -14.20427779279535230 ) ) ;
#84937=CARTESIAN_POINT ( 'NONE',  ( -2.815433093576920509, 14.63606915880330206, -14.73340885523757748 ) ) ;
#84942=CARTESIAN_POINT ( 'NONE',  ( -1.909764518474394990, 0.000000000000000000, -5.107897229450617971 ) ) ;
#84947=CARTESIAN_POINT ( 'NONE',  ( -5.204170427930421283E-15, -9.446251165086030355, -14.16423886937410082 ) ) ;
#84954=DIRECTION ( 'NONE',  ( 0.9990482215818573541, 0.000000000000000000, 0.04361938736534638067 ) ) ;
#84955=CARTESIAN_POINT ( 'NONE',  ( 0.000000000000000000, 15.00000000000000000, 0.000000000000000000 ) ) ;
#84960=DIRECTION ( 'NONE',  ( -0.4461978131098006117, 0.000000000000000000, -0.8949343616020291048 ) ) ;
#84961=DIRECTION ( 'NONE',  ( 0.000000000000000000, 0.000000000000000000, 1.000000000000000000 ) ) ;
#84969=ORIENTED_EDGE ( 'NONE', *, *, #33326, .F. ) ;
#84972=CARTESIAN_POINT ( 'NONE',  ( 0.000000000000000000, 14.49999999999999822, 0.000000000000000000 ) ) ;
#84983=ORIENTED_EDGE ( 'NONE', *, *, #33632, .F. ) ;
#84984=CARTESIAN_POINT ( 'NONE',  ( 0.000000000000000000, 14.49999999999999822, 0.000000000000000000 ) ) ;
#84995=EDGE_LOOP ( 'NONE', ( #68573, #59794, #8499, #58795 ) ) ;
#84998=CARTESIAN_POINT ( 'NONE',  ( 3.927832320392154575, 15.00000000000000000, 13.69797916712106733 ) ) ;
#85009=CARTESIAN_POINT ( 'NONE',  ( -8.201146098718011146, 12.29405489584603828, -8.255447149008286800 ) ) ;
#85010=CARTESIAN_POINT ( 'NONE',  ( 0.000000000000000000, 14.49999999999999822, 0.000000000000000000 ) ) ;
#85015=CARTESIAN_POINT ( 'NONE',  ( -4.096035146093331747, 15.00000000000000000, -13.90943910019262653 ) ) ;
#85017=DIRECTION ( 'NONE',  ( -0.000000000000000000, -1.000000000000000000, -0.000000000000000000 ) ) ;
#85018=CARTESIAN_POINT ( 'NONE',  ( -12.81628187352647963, -41.08469866340290366, -3.434112377981046293 ) ) ;
#85019=ORIENTED_EDGE ( 'NONE', *, *, #47511, .T. ) ;
#85027=CIRCLE ( 'NONE', #17936, 15.00000000000000000 ) ;
#85028=ADVANCED_FACE ( 'NONE', ( #35352 ), #43830, .F. ) ;
#85033=ADVANCED_FACE ( 'NONE', ( #59819 ), #80861, .T. ) ;
#85035=EDGE_LOOP ( 'NONE', ( #67810, #20011, #20195, #50383, #48600, #58597 ) ) ;
#85037=ORIENTED_EDGE ( 'NONE', *, *, #74844, .F. ) ;
#85039=CARTESIAN_POINT ( 'NONE',  ( 8.731067818237036704, 6.563309369127505732, 8.731067818237033151 ) ) ;
#85044=ORIENTED_EDGE ( 'NONE', *, *, #77853, .F. ) ;
#85050=VECTOR ( 'NONE', #86424, 1000.000000000000000 ) ;
#85056=LINE ( 'NONE', #69565, #21052 ) ;
#85059=B_SPLINE_CURVE_WITH_KNOTS ( 'NONE', 3,
 ( #29608, #8119, #45614, #47082, #60112, #15633 ),
 .UNSPECIFIED., .F., .F.,
 ( 4, 2, 4 ),
 ( 0.0002800671705680612489, 0.0006862730573397339204, 0.001092478944111406483 ),
 .UNSPECIFIED. ) ;
#85061=VECTOR ( 'NONE', #64764, 1000.000000000000000 ) ;
#85065=EDGE_CURVE ( 'NONE', #31048, #75691, #6334, .T. ) ;
#85066=DIRECTION ( 'NONE',  ( 0.000000000000000000, 0.000000000000000000, 1.000000000000000000 ) ) ;
#85069=DIRECTION ( 'NONE',  ( 0.000000000000000000, 1.000000000000000000, 0.000000000000000000 ) ) ;
#85078=CARTESIAN_POINT ( 'NONE',  ( 14.56368227077858357, 0.2306972965111892260, -3.337246381125186456 ) ) ;
#85080=FACE_OUTER_BOUND ( 'NONE', #73261, .T. ) ;
#85081=VECTOR ( 'NONE', #59451, 1000.000000000000114 ) ;
#85084=CARTESIAN_POINT ( 'NONE',  ( -9.422509992056136596, 3.480352010821509356, 5.440088680355559703 ) ) ;
#85089=CARTESIAN_POINT ( 'NONE',  ( 1.377727649040772586E-15, 12.49999999999999112, 11.25000000000000178 ) ) ;
#85092=CIRCLE ( 'NONE', #91523, 14.49999999999999822 ) ;
#85099=CARTESIAN_POINT ( 'NONE',  ( -10.58223187591015169, 0.2306972965111903362, 10.54772123337523837 ) ) ;
#85101=EDGE_LOOP ( 'NONE', ( #29987, #81387, #75298, #1570, #55048, #69384 ) ) ;
#85109=CARTESIAN_POINT ( 'NONE',  ( -4.431036607602660382, 15.00000000000000000, 14.33059365769907956 ) ) ;
#85114=CARTESIAN_POINT ( 'NONE',  ( -4.873787042390880231, 0.000000000000000000, 13.39061984619915791 ) ) ;
#85128=CIRCLE ( 'NONE', #11673, 14.49999999999999822 ) ;
#85129=CARTESIAN_POINT ( 'NONE',  ( 12.54397927573569049, 0.2306972965111904195, -8.117058495689017050 ) ) ;
#85133=CARTESIAN_POINT ( 'NONE',  ( -9.846743663894594434, -3.991068848999211660, 3.469446951953614189E-15 ) ) ;
#85134=ORIENTED_EDGE ( 'NONE', *, *, #56782, .F. ) ;
#85137=DIRECTION ( 'NONE',  ( -0.9681476403781084095, 0.000000000000000000, 0.2503800040544389982 ) ) ;
#85146=ADVANCED_FACE ( 'NONE', ( #37843 ), #63051, .T. ) ;
#85150=VERTEX_POINT ( 'NONE', #8318 ) ;
#85151=EDGE_CURVE ( 'NONE', #30913, #7321, #68334, .T. ) ;
#85153=VERTEX_POINT ( 'NONE', #84327 ) ;
#85162=DIRECTION ( 'NONE',  ( -0.000000000000000000, -1.000000000000000000, -0.000000000000000000 ) ) ;
#85163=VECTOR ( 'NONE', #56148, 1000.000000000000000 ) ;
#85172=LINE ( 'NONE', #93152, #4417 ) ;
#85184=CARTESIAN_POINT ( 'NONE',  ( 12.83294900548062678, 14.49999999999999112, 7.766300266068507874 ) ) ;
#85187=TOROIDAL_SURFACE ( 'NONE', #42099, 14.49999999999999822, 0.5000000000000000000 ) ;
#85190=FACE_OUTER_BOUND ( 'NONE', #67696, .T. ) ;
#85194=CARTESIAN_POINT ( 'NONE',  ( -8.439016546559980014, 3.939291001653719071E-16, 11.79122553964967679 ) ) ;
#85195=AXIS2_PLACEMENT_3D ( 'NONE', #16993, #17491, #85484 ) ;
#85196=EDGE_CURVE ( 'NONE', #23413, #92402, #12024, .T. ) ;
#85198=LINE ( 'NONE', #85687, #53353 ) ;
#85204=CARTESIAN_POINT ( 'NONE',  ( 10.36894250292379027, 28.67874883491397142, 10.36894250292378672 ) ) ;
#85221=CARTESIAN_POINT ( 'NONE',  ( 14.88232117145533628, 14.63606897487930425, 1.875237731503260452 ) ) ;
#85226=ORIENTED_EDGE ( 'NONE', *, *, #67277, .F. ) ;
#85228=DIRECTION ( 'NONE',  ( -0.9588197348681947174, 0.000000000000000000, 0.2840153447039170387 ) ) ;
#85232=FACE_OUTER_BOUND ( 'NONE', #81792, .T. ) ;
#85239=ORIENTED_EDGE ( 'NONE', *, *, #6438, .F. ) ;
#85241=CARTESIAN_POINT ( 'NONE',  ( 4.096035146093422341, 15.00000000000000000, 13.90943910019259810 ) ) ;
#85247=LINE ( 'NONE', #25254, #61378 ) ;
#85248=EDGE_CURVE ( 'NONE', #52573, #56319, #59644, .T. ) ;
#85251=CARTESIAN_POINT ( 'NONE',  ( 12.80781515976310203, -0.03417435944610275333, 6.246788841744411513 ) ) ;
#85256=ORIENTED_EDGE ( 'NONE', *, *, #45046, .T. ) ;
#85258=ORIENTED_EDGE ( 'NONE', *, *, #704, .T. ) ;
#85259=ADVANCED_FACE ( 'NONE', ( #8802 ), #53313, .F. ) ;
#85268=ADVANCED_FACE ( 'NONE', ( #62282 ), #85299, .T. ) ;
#85269=VECTOR ( 'NONE', #55216, 1000.000000000000000 ) ;
#85273=AXIS2_PLACEMENT_3D ( 'NONE', #33879, #56892, #33391 ) ;
#85274=ORIENTED_EDGE ( 'NONE', *, *, #54887, .T. ) ;
#85282=DIRECTION ( 'NONE',  ( -0.7253743710122912969, 0.000000000000000000, 0.6883545756937501370 ) ) ;
#85288=ORIENTED_EDGE ( 'NONE', *, *, #81572, .T. ) ;
#85289=CARTESIAN_POINT ( 'NONE',  ( 11.48952521350018685, 4.805858850777305443E-16, 8.845383562533823962 ) ) ;
#85299=CYLINDRICAL_SURFACE ( 'NONE', #50336, 15.00000000000000000 ) ;
#85316=DIRECTION ( 'NONE',  ( 0.04361938736534638067, 0.000000000000000000, -0.9990482215818573541 ) ) ;
#85325=CARTESIAN_POINT ( 'NONE',  ( 13.14228782657335870, 14.63595249122788999, 7.230509711182328658 ) ) ;
#85340=CARTESIAN_POINT ( 'NONE',  ( 14.35840480524200657, 0.3639308199838637292, 4.340070442838945830 ) ) ;
#85343=CYLINDRICAL_SURFACE ( 'NONE', #6652, 15.00000000000000000 ) ;
#85355=DIRECTION ( 'NONE',  ( 0.000000000000000000, 1.000000000000000000, 0.000000000000000000 ) ) ;
#85366=ORIENTED_EDGE ( 'NONE', *, *, #47982, .F. ) ;
#85373=ORIENTED_EDGE ( 'NONE', *, *, #72351, .F. ) ;
#85385=EDGE_CURVE ( 'NONE', #88316, #84655, #95429, .T. ) ;
#85395=EDGE_CURVE ( 'NONE', #77130, #69916, #7, .T. ) ;
#85399=ORIENTED_EDGE ( 'NONE', *, *, #85476, .F. ) ;
#85405=AXIS2_PLACEMENT_3D ( 'NONE', #62789, #17311, #16812 ) ;
#85409=DIRECTION ( 'NONE',  ( 0.000000000000000000, 1.000000000000000000, 0.000000000000000000 ) ) ;
#85410=CARTESIAN_POINT ( 'NONE',  ( -14.02068044289375592, 0.3639308153356248243, -5.331089937175855553 ) ) ;
#85420=VECTOR ( 'NONE', #88891, 999.9999999999998863 ) ;
#85432=CARTESIAN_POINT ( 'NONE',  ( 1.354709868695649577, 14.49999999999999112, -14.93870011653157448 ) ) ;
#85436=FACE_OUTER_BOUND ( 'NONE', #26136, .T. ) ;
#85437=VECTOR ( 'NONE', #24820, 1000.000000000000000 ) ;
#85438=EDGE_CURVE ( 'NONE', #84834, #20560, #64242, .T. ) ;
#85439=DIRECTION ( 'NONE',  ( 0.000000000000000000, 0.000000000000000000, 1.000000000000000000 ) ) ;
#85442=CARTESIAN_POINT ( 'NONE',  ( -14.16423886937410082, -8.196251165086030355, 4.336808689942017736E-15 ) ) ;
#85446=ORIENTED_EDGE ( 'NONE', *, *, #17197, .F. ) ;
#85450=DIRECTION ( 'NONE',  ( -0.2334453638558956767, 0.000000000000000000, -0.9723699203976788885 ) ) ;
#85456=CARTESIAN_POINT ( 'NONE',  ( 14.82269085861167035, 15.00000000000000000, 2.299529454047060550 ) ) ;
#85459=VECTOR ( 'NONE', #52010, 1000.000000000000000 ) ;
#85468=ORIENTED_EDGE ( 'NONE', *, *, #44718, .T. ) ;
#85472=EDGE_CURVE ( 'NONE', #67824, #49583, #78280, .T. ) ;
#85476=EDGE_CURVE ( 'NONE', #70888, #18498, #73990, .T. ) ;
#85484=DIRECTION ( 'NONE',  ( 0.000000000000000000, 0.000000000000000000, 1.000000000000000000 ) ) ;
#85485=DIRECTION ( 'NONE',  ( 0.000000000000000000, 0.000000000000000000, 1.000000000000000000 ) ) ;
#85502=DIRECTION ( 'NONE',  ( 0.4461978131097943945, 0.000000000000000000, 0.8949343616020322134 ) ) ;
#85510=ADVANCED_FACE ( 'NONE', ( #72246 ), #34233, .F. ) ;
#85511=CARTESIAN_POINT ( 'NONE',  ( 0.000000000000000000, 15.00000000000000000, 0.000000000000000000 ) ) ;
#85512=CARTESIAN_POINT ( 'NONE',  ( -9.846743663894590881, 31.21726448433413736, 2.638427012816840111 ) ) ;
#85513=ORIENTED_EDGE ( 'NONE', *, *, #61551, .T. ) ;
#85514=CARTESIAN_POINT ( 'NONE',  ( -6.767445849361070742, 14.63606917768312954, -13.38662304974510064 ) ) ;
#85524=ORIENTED_EDGE ( 'NONE', *, *, #19990, .F. ) ;
#85527=ORIENTED_EDGE ( 'NONE', *, *, #4569, .F. ) ;
#85536=CARTESIAN_POINT ( 'NONE',  ( -4.838527690343713772, 0.5000000000000004441, 14.19819177887723605 ) ) ;
#85555=VERTEX_POINT ( 'NONE', #32276 ) ;
#85563=CARTESIAN_POINT ( 'NONE',  ( -6.336512077239976115, 0.2306972965111889207, 13.53095227201380801 ) ) ;
#85565=AXIS2_PLACEMENT_3D ( 'NONE', #36118, #28125, #97153 ) ;
#85568=ORIENTED_EDGE ( 'NONE', *, *, #55341, .F. ) ;
#85574=CARTESIAN_POINT ( 'NONE',  ( 14.09394518620612224, 3.883508853191620072E-16, -3.407449058785360752 ) ) ;
#85579=CARTESIAN_POINT ( 'NONE',  ( 10.88017736071110519, 5.563685344154841950, -2.602085213965210642E-15 ) ) ;
#85581=CARTESIAN_POINT ( 'NONE',  ( 4.838527690343616960, 14.63595249122790598, -14.19819177887726980 ) ) ;
#85584=VECTOR ( 'NONE', #62174, 1000.000000000000000 ) ;
#85589=DIRECTION ( 'NONE',  ( 0.000000000000000000, 0.000000000000000000, -1.000000000000000000 ) ) ;
#85590=EDGE_CURVE ( 'NONE', #30551, #62241, #67926, .T. ) ;
#85608=DIRECTION ( 'NONE',  ( 0.000000000000000000, 0.000000000000000000, 1.000000000000000000 ) ) ;
#85612=AXIS2_PLACEMENT_3D ( 'NONE', #41380, #18855, #24891 ) ;
#85613=ORIENTED_EDGE ( 'NONE', *, *, #29685, .T. ) ;
#85627=CARTESIAN_POINT ( 'NONE',  ( -7.208316651077764980, -9.616068848999210772, -7.208316651077759651 ) ) ;
#85629=DIRECTION ( 'NONE',  ( -0.000000000000000000, -1.000000000000000000, -0.000000000000000000 ) ) ;
#85637=CARTESIAN_POINT ( 'NONE',  ( -14.16722289976682170, 14.63606870530283643, -4.928467845925730728 ) ) ;
#85641=EDGE_LOOP ( 'NONE', ( #56950, #40492, #33332, #32482, #25567, #69297 ) ) ;
#85643=ORIENTED_EDGE ( 'NONE', *, *, #98297, .T. ) ;
#85655=VERTEX_POINT ( 'NONE', #12238 ) ;
#85658=DIRECTION ( 'NONE',  ( 0.000000000000000000, 1.000000000000000000, 0.000000000000000000 ) ) ;
#85662=VERTEX_POINT ( 'NONE', #88729 ) ;
#85676=CARTESIAN_POINT ( 'NONE',  ( 13.07751017357383994, 4.340377266345630487E-16, -6.263284095430506682 ) ) ;
#85678=ORIENTED_EDGE ( 'NONE', *, *, #90385, .F. ) ;
#85684=TOROIDAL_SURFACE ( 'NONE', #2484, 14.49999999999999822, 0.5000000000000000000 ) ;
#85686=CARTESIAN_POINT ( 'NONE',  ( -3.897244926436313150, 4.087811286569849197E-16, 13.96644127841328142 ) ) ;
#85687=CARTESIAN_POINT ( 'NONE',  ( 12.34086200392821908, 15.00000000000000000, 7.125000000000058620 ) ) ;
#85691=CARTESIAN_POINT ( 'NONE',  ( -14.16423886937409726, 27.01208216824730712, 3.795296366450320757 ) ) ;
#85701=AXIS2_PLACEMENT_3D ( 'NONE', #33858, #1940, #70916 ) ;
#85704=VERTEX_POINT ( 'NONE', #34735 ) ;
#85711=CARTESIAN_POINT ( 'NONE',  ( -8.564643372776718167, 14.49999999999999112, 12.31449893000741369 ) ) ;
#85712=CARTESIAN_POINT ( 'NONE',  ( 4.862001128006681938, 4.613545383394330660E-16, 13.66056166602463229 ) ) ;
#85718=CARTESIAN_POINT ( 'NONE',  ( 14.62617646268094518, 14.49999999999999112, -3.327906561566873478 ) ) ;
#85727=VECTOR ( 'NONE', #9232, 1000.000000000000227 ) ;
#85731=ORIENTED_EDGE ( 'NONE', *, *, #71933, .T. ) ;
#85733=DIRECTION ( 'NONE',  ( 0.000000000000000000, 0.000000000000000000, 1.000000000000000000 ) ) ;
#85743=AXIS2_PLACEMENT_3D ( 'NONE', #84669, #84189, #31160 ) ;
#85745=PLANE ( 'NONE',  #17866 ) ;
#85746=CARTESIAN_POINT ( 'NONE',  ( 0.000000000000000000, 0.000000000000000000, 0.000000000000000000 ) ) ;
#85751=ORIENTED_EDGE ( 'NONE', *, *, #56782, .T. ) ;
#85752=CARTESIAN_POINT ( 'NONE',  ( -1.236355250167165964, 0.04962892728883445959, -14.70131747622450114 ) ) ;
#85753=VERTEX_POINT ( 'NONE', #13725 ) ;
#85755=ORIENTED_EDGE ( 'NONE', *, *, #11758, .T. ) ;
#85759=ADVANCED_FACE ( 'NONE', ( #73722 ), #44210, .T. ) ;
#85760=DIRECTION ( 'NONE',  ( -0.000000000000000000, -1.000000000000000000, -0.000000000000000000 ) ) ;
#85764=CARTESIAN_POINT ( 'NONE',  ( 12.81628187352647608, 1.415301336597085013, 3.434112377981052511 ) ) ;
#85765=EDGE_LOOP ( 'NONE', ( #95253, #24161, #96413, #40539 ) ) ;
#85768=ORIENTED_EDGE ( 'NONE', *, *, #1740, .F. ) ;
#85777=AXIS2_PLACEMENT_3D ( 'NONE', #62527, #78531, #63029 ) ;
#85778=VERTEX_POINT ( 'NONE', #58724 ) ;
#85784=CARTESIAN_POINT ( 'NONE',  ( 0.000000000000000000, 15.00000000000000000, 0.000000000000000000 ) ) ;
#85792=CARTESIAN_POINT ( 'NONE',  ( 4.862001128006681050, 15.00000000000000000, 13.66056166602463229 ) ) ;
#85796=EDGE_CURVE ( 'NONE', #45156, #85704, #53556, .T. ) ;
#85813=CARTESIAN_POINT ( 'NONE',  ( -5.803070148808147088, 3.900978891399319278E-16, -13.28812917035395813 ) ) ;
#85816=CARTESIAN_POINT ( 'NONE',  ( 8.606322355898619492, 15.00000000000000000, -11.66967075399251996 ) ) ;
#85821=ADVANCED_FACE ( 'NONE', ( #81232 ), #2495, .T. ) ;
#85826=CARTESIAN_POINT ( 'NONE',  ( -15.81765804549835330, -0.03417435944610275333, -2.383084218347030880 ) ) ;
#85831=EDGE_CURVE ( 'NONE', #98827, #95512, #69226, .T. ) ;
#85833=FACE_OUTER_BOUND ( 'NONE', #696, .T. ) ;
#85834=LINE ( 'NONE', #63793, #30052 ) ;
#85838=AXIS2_PLACEMENT_3D ( 'NONE', #78619, #32612, #10128 ) ;
#85840=FACE_OUTER_BOUND ( 'NONE', #13934, .T. ) ;
#85848=CIRCLE ( 'NONE', #65041, 14.49999999999999822 ) ;
#85850=VECTOR ( 'NONE', #73841, 1000.000000000000000 ) ;
#85870=EDGE_CURVE ( 'NONE', #50110, #47708, #82712, .T. ) ;
#85876=DIRECTION ( 'NONE',  ( 0.000000000000000000, 0.000000000000000000, 1.000000000000000000 ) ) ;
#85885=LINE ( 'NONE', #47867, #12614 ) ;
#85889=CARTESIAN_POINT ( 'NONE',  ( 6.336512077239798479, 14.76930270348881002, 13.53095227201389328 ) ) ;
#85894=CARTESIAN_POINT ( 'NONE',  ( 0.000000000000000000, 15.00000000000000000, 0.000000000000000000 ) ) ;
#85899=ORIENTED_EDGE ( 'NONE', *, *, #67189, .T. ) ;
#85900=DIRECTION ( 'NONE',  ( 0.000000000000000000, 1.000000000000000000, 0.000000000000000000 ) ) ;
#85907=CARTESIAN_POINT ( 'NONE',  ( -1.847237859018842299, 0.04962896072145024651, 14.63711110085118783 ) ) ;
#85919=CARTESIAN_POINT ( 'NONE',  ( 13.59943737456458024, 14.95077488074853456, -5.718514076972845750 ) ) ;
#85922=LINE ( 'NONE', #33380, #56835 ) ;
#85927=CARTESIAN_POINT ( 'NONE',  ( 0.000000000000000000, 0.000000000000000000, 0.000000000000000000 ) ) ;
#85938=CARTESIAN_POINT ( 'NONE',  ( 3.843542995449656718, 0.2301500725087332888, -14.43777707752878925 ) ) ;
#85939=DIRECTION ( 'NONE',  ( 0.000000000000000000, 0.000000000000000000, -1.000000000000000000 ) ) ;
#85942=CARTESIAN_POINT ( 'NONE',  ( -7.082119434687058401, -4.029584498419364280, -12.26659068614894110 ) ) ;
#85946=EDGE_CURVE ( 'NONE', #25822, #78552, #51328, .T. ) ;
#85971=CIRCLE ( 'NONE', #6094, 15.00000000000000000 ) ;
#85977=CARTESIAN_POINT ( 'NONE',  ( 10.93781366033340596, 0.3640475087720985159, 10.26470809774073700 ) ) ;
#85979=ORIENTED_EDGE ( 'NONE', *, *, #62557, .T. ) ;
#85980=FACE_OUTER_BOUND ( 'NONE', #90907, .T. ) ;
#85993=DIRECTION ( 'NONE',  ( 0.000000000000000000, 0.000000000000000000, 1.000000000000000000 ) ) ;
#86001=CARTESIAN_POINT ( 'NONE',  ( -13.55157833323639238, 0.2306972965111898921, 6.292279346205288171 ) ) ;
#86009=CARTESIAN_POINT ( 'NONE',  ( -8.527530157486182816, 25.59226448433413026, -4.923371831947288335 ) ) ;
#86022=EDGE_LOOP ( 'NONE', ( #5864, #69820, #82351, #63727 ) ) ;
#86025=AXIS2_PLACEMENT_3D ( 'NONE', #19177, #43153, #49657 ) ;
#86027=ADVANCED_FACE ( 'NONE', ( #36014 ), #43511, .F. ) ;
#86031=SURFACE_STYLE_FILL_AREA ( #18025 ) ;
#86036=CARTESIAN_POINT ( 'NONE',  ( -9.065164099344613646, 0.5000000000000004441, 11.95084933600761445 ) ) ;
#86038=ORIENTED_EDGE ( 'NONE', *, *, #3671, .T. ) ;
#86040=LINE ( 'NONE', #56521, #60210 ) ;
#86042=EDGE_CURVE ( 'NONE', #44839, #23568, #79112, .T. ) ;
#86062=ORIENTED_EDGE ( 'NONE', *, *, #94080, .F. ) ;
#86063=EDGE_LOOP ( 'NONE', ( #12176, #1224, #94716, #83941 ) ) ;
#86071=EDGE_CURVE ( 'NONE', #40720, #50188, #68007, .T. ) ;
#86074=CARTESIAN_POINT ( 'NONE',  ( -5.440088680355558814, -2.769647989178489311, -9.422509992056136596 ) ) ;
#86080=DIRECTION ( 'NONE',  ( 0.3173046564050899243, 0.000000000000000000, 0.9483236552061999891 ) ) ;
#86084=CARTESIAN_POINT ( 'NONE',  ( 10.32896413005679825, 12.60497603579417714, -5.963430220938286119 ) ) ;
#86099=VECTOR ( 'NONE', #90947, 1000.000000000000000 ) ;
#86101=CARTESIAN_POINT ( 'NONE',  ( 13.16740645155971201, 14.95077488074853456, -6.653232860246546920 ) ) ;
#86103=B_SPLINE_CURVE_WITH_KNOTS ( 'NONE', 3,
 ( #38273, #68766, #297, #91754, #23276, #53753 ),
 .UNSPECIFIED., .F., .F.,
 ( 4, 2, 4 ),
 ( 0.0002800225282622560924, 0.0006862279780598563861, 0.001092433427857456571 ),
 .UNSPECIFIED. ) ;
#86104=DIRECTION ( 'NONE',  ( 0.000000000000000000, 1.000000000000000000, 0.000000000000000000 ) ) ;
#86121=CARTESIAN_POINT ( 'NONE',  ( -2.638427012816840111, -15.03273551566587685, -9.846743663894590881 ) ) ;
#86124=FACE_OUTER_BOUND ( 'NONE', #91540, .T. ) ;
#86125=DIRECTION ( 'NONE',  ( 0.000000000000000000, 1.000000000000000000, 0.000000000000000000 ) ) ;
#86136=ORIENTED_EDGE ( 'NONE', *, *, #67304, .T. ) ;
#86138=ORIENTED_EDGE ( 'NONE', *, *, #26216, .F. ) ;
#86140=ORIENTED_EDGE ( 'NONE', *, *, #97321, .T. ) ;
#86142=AXIS2_PLACEMENT_3D ( 'NONE', #58688, #89681, #73189 ) ;
#86149=DIRECTION ( 'NONE',  ( -0.000000000000000000, 1.000000000000000000, -0.000000000000000000 ) ) ;
#86150=ORIENTED_EDGE ( 'NONE', *, *, #6509, .T. ) ;
#86151=EDGE_CURVE ( 'NONE', #38777, #73854, #74008, .T. ) ;
#86155=DIRECTION ( 'NONE',  ( 0.000000000000000000, 1.000000000000000000, 0.000000000000000000 ) ) ;
#86158=LINE ( 'NONE', #1206, #18755 ) ;
#86174=EDGE_CURVE ( 'NONE', #37579, #65662, #17863, .T. ) ;
#86177=PLANE ( 'NONE',  #7424 ) ;
#86181=CARTESIAN_POINT ( 'NONE',  ( 14.16722289976685722, 14.63595249122789177, -4.928467845925526447 ) ) ;
#86182=DIRECTION ( 'NONE',  ( -0.000000000000000000, -1.000000000000000000, -0.000000000000000000 ) ) ;
#86185=CARTESIAN_POINT ( 'NONE',  ( -14.16722289976689630, 14.63595249122789532, 4.928467845925427859 ) ) ;
#86188=CARTESIAN_POINT ( 'NONE',  ( 7.082119434687047743, 30.13708216824731423, -12.26659068614894821 ) ) ;
#86197=ORIENTED_EDGE ( 'NONE', *, *, #60532, .F. ) ;
#86209=DIRECTION ( 'NONE',  ( 0.000000000000000000, 0.000000000000000000, 1.000000000000000000 ) ) ;
#86210=CIRCLE ( 'NONE', #62210, 15.00000000000000000 ) ;
#86219=CARTESIAN_POINT ( 'NONE',  ( -8.157527544167827216, 14.76984925468920196, 12.51706795611529621 ) ) ;
#86238=ORIENTED_EDGE ( 'NONE', *, *, #89636, .T. ) ;
#86239=CARTESIAN_POINT ( 'NONE',  ( -14.15369600240089909, 15.00000000000000888, 3.689340892730124555 ) ) ;
#86242=ORIENTED_EDGE ( 'NONE', *, *, #67747, .F. ) ;
#86246=EDGE_CURVE ( 'NONE', #60661, #15080, #44990, .T. ) ;
#86248=ORIENTED_EDGE ( 'NONE', *, *, #98035, .T. ) ;
#86250=CARTESIAN_POINT ( 'NONE',  ( 12.34557190004675320, 14.95077488074853633, 8.076692058882576575 ) ) ;
#86251=CARTESIAN_POINT ( 'NONE',  ( -6.408140936763246032, -1.709698663402911656, -11.09922568453594316 ) ) ;
#86259=LINE ( 'NONE', #18258, #41886 ) ;
#86260=FACE_OUTER_BOUND ( 'NONE', #26719, .T. ) ;
#86263=VECTOR ( 'NONE', #26801, 1000.000000000000000 ) ;
#86264=EDGE_CURVE ( 'NONE', #74198, #42986, #20084, .T. ) ;
#86265=DIRECTION ( 'NONE',  ( -0.3665012267242880872, 0.000000000000000000, -0.9304175679820281264 ) ) ;
#86267=CARTESIAN_POINT ( 'NONE',  ( 0.000000000000000000, 15.00000000000000000, 0.000000000000000000 ) ) ;
#86281=CARTESIAN_POINT ( 'NONE',  ( -4.084234479374336146, 0.000000000000000000, 3.613425430272898975 ) ) ;
#86290=FILL_AREA_STYLE_COLOUR ( '', #39085 ) ;
#86293=ORIENTED_EDGE ( 'NONE', *, *, #71757, .F. ) ;
#86304=LINE ( 'NONE', #48782, #32995 ) ;
#86306=EDGE_CURVE ( 'NONE', #70448, #63236, #61471, .T. ) ;
#86308=DIRECTION ( 'NONE',  ( 0.000000000000000000, 1.000000000000000000, 0.000000000000000000 ) ) ;
#86310=AXIS2_PLACEMENT_3D ( 'NONE', #53688, #8204, #15714 ) ;
#86312=VERTEX_POINT ( 'NONE', #39965 ) ;
#86323=LINE ( 'NONE', #32319, #24545 ) ;
#86329=DIRECTION ( 'NONE',  ( -0.000000000000000000, -1.000000000000000000, -0.000000000000000000 ) ) ;
#86339=AXIS2_PLACEMENT_3D ( 'NONE', #64528, #16599, #2110 ) ;
#86357=ORIENTED_EDGE ( 'NONE', *, *, #87058, .T. ) ;
#86358=AXIS2_PLACEMENT_3D ( 'NONE', #91662, #45667, #98200 ) ;
#86360=ORIENTED_EDGE ( 'NONE', *, *, #97677, .T. ) ;
#86361=CARTESIAN_POINT ( 'NONE',  ( -9.240973841163681257, 4.382479893023984083E-16, 11.17382667070366331 ) ) ;
#86364=ORIENTED_EDGE ( 'NONE', *, *, #41252, .F. ) ;
#86368=LINE ( 'NONE', #70880, #28072 ) ;
#86375=ORIENTED_EDGE ( 'NONE', *, *, #49716, .T. ) ;
#86382=FACE_OUTER_BOUND ( 'NONE', #58063, .T. ) ;
#86389=ORIENTED_EDGE ( 'NONE', *, *, #65153, .F. ) ;
#86393=ORIENTED_EDGE ( 'NONE', *, *, #81565, .F. ) ;
#86394=FACE_OUTER_BOUND ( 'NONE', #87974, .T. ) ;
#86399=FACE_OUTER_BOUND ( 'NONE', #73309, .T. ) ;
#86402=CARTESIAN_POINT ( 'NONE',  ( 0.000000000000000000, 0.5000000000000004441, 0.000000000000000000 ) ) ;
#86406=DIRECTION ( 'NONE',  ( 0.000000000000000000, 0.000000000000000000, 1.000000000000000000 ) ) ;
#86409=AXIS2_PLACEMENT_3D ( 'NONE', #60982, #7522, #60497 ) ;
#86416=TOROIDAL_SURFACE ( 'NONE', #51218, 14.49999999999999822, 0.5000000000000000000 ) ;
#86418=CARTESIAN_POINT ( 'NONE',  ( -13.86102707272226731, -2.652907190800467873E-15, 4.666951904077105695 ) ) ;
#86424=DIRECTION ( 'NONE',  ( -0.000000000000000000, 1.000000000000000000, 0.000000000000000000 ) ) ;
#86425=CARTESIAN_POINT ( 'NONE',  ( -8.157527544166347511, 0.2301507453079257859, -12.51706795611459100 ) ) ;
#86427=ORIENTED_EDGE ( 'NONE', *, *, #19935, .F. ) ;
#86434=CARTESIAN_POINT ( 'NONE',  ( -7.082119434687044190, 12.63708216824730535, 12.26659068614894998 ) ) ;
#86452=CARTESIAN_POINT ( 'NONE',  ( -14.43100913236848371, 4.112960668137814512E-16, -1.412789942453356318 ) ) ;
#86459=ORIENTED_EDGE ( 'NONE', *, *, #39203, .F. ) ;
#86474=CARTESIAN_POINT ( 'NONE',  ( 0.000000000000000000, 0.5000000000000004441, 0.000000000000000000 ) ) ;
#86479=EDGE_CURVE ( 'NONE', #28504, #87109, #41480, .T. ) ;
#86489=VERTEX_POINT ( 'NONE', #7416 ) ;
#86493=CARTESIAN_POINT ( 'NONE',  ( 13.50249619331273720, -1.423015351387222844E-16, 5.623250243473579602 ) ) ;
#86497=EDGE_CURVE ( 'NONE', #39436, #37440, #90883, .T. ) ;
#86502=AXIS2_PLACEMENT_3D ( 'NONE', #21037, #7022, #51527 ) ;
#86505=CARTESIAN_POINT ( 'NONE',  ( 6.408140936763236262, -32.54303199673623936, -11.09922568453595026 ) ) ;
#86520=VERTEX_POINT ( 'NONE', #89901 ) ;
#86529=VECTOR ( 'NONE', #61024, 1000.000000000000000 ) ;
#86532=VERTEX_POINT ( 'NONE', #20431 ) ;
#86537=DIRECTION ( 'NONE',  ( 0.7489557207889945278, 0.000000000000000000, 0.6626200482157461602 ) ) ;
#86545=ADVANCED_FACE ( 'NONE', ( #52886 ), #50918, .F. ) ;
#86548=CARTESIAN_POINT ( 'NONE',  ( 14.16423886937410437, -30.90458449841936073, 3.795296366450304770 ) ) ;
#86553=ORIENTED_EDGE ( 'NONE', *, *, #83094, .F. ) ;
#86558=VECTOR ( 'NONE', #27824, 1000.000000000000000 ) ;
#86563=DIRECTION ( 'NONE',  ( 0.000000000000000000, 1.000000000000000000, 0.000000000000000000 ) ) ;
#86566=CARTESIAN_POINT ( 'NONE',  ( -5.204170427930421283E-15, 1.813685344154845946, -10.88017736071110342 ) ) ;
#86567=CARTESIAN_POINT ( 'NONE',  ( 3.822225673302248605, 0.000000000000000000, 3.889525102760262865 ) ) ;
#86569=CARTESIAN_POINT ( 'NONE',  ( -11.48952521350012113, 4.018634162980579609E-16, -8.845383562533903898 ) ) ;
#86575=CARTESIAN_POINT ( 'NONE',  ( 3.195792623639533758, 11.14664270246084499, 11.92686044187656158 ) ) ;
#86599=AXIS2_PLACEMENT_3D ( 'NONE', #33840, #10387, #9901 ) ;
#86603=PLANE ( 'NONE',  #92243 ) ;
#86609=ADVANCED_FACE ( 'NONE', ( #811 ), #95159, .T. ) ;
#86610=DIRECTION ( 'NONE',  ( 0.000000000000000000, 0.000000000000000000, -1.000000000000000000 ) ) ;
#86612=CARTESIAN_POINT ( 'NONE',  ( -2.638427012816840111, -10.03273551566587507, -9.846743663894590881 ) ) ;
#86616=CYLINDRICAL_SURFACE ( 'NONE', #26942, 15.00000000000000000 ) ;
#86623=DIRECTION ( 'NONE',  ( 0.000000000000000000, 0.000000000000000000, -1.000000000000000000 ) ) ;
#86625=CARTESIAN_POINT ( 'NONE',  ( -9.382169495545413795, 29.74863466993043559, 9.382169495545428006 ) ) ;
#86629=VERTEX_POINT ( 'NONE', #7804 ) ;
#86633=ORIENTED_EDGE ( 'NONE', *, *, #52829, .T. ) ;
#86647=DIRECTION ( 'NONE',  ( -4.352074256530613638E-14, 0.000000000000000000, 1.000000000000000000 ) ) ;
#86648=AXIS2_PLACEMENT_3D ( 'NONE', #80558, #12547, #90017 ) ;
#86654=DIRECTION ( 'NONE',  ( 0.000000000000000000, 0.000000000000000000, 1.000000000000000000 ) ) ;
#86655=ORIENTED_EDGE ( 'NONE', *, *, #82839, .F. ) ;
#86658=CARTESIAN_POINT ( 'NONE',  ( -7.771322705631315664, 15.00000000000000000, -12.24159072199926257 ) ) ;
#86663=CARTESIAN_POINT ( 'NONE',  ( -11.92686044187656869, 7.453790035174482576, -3.195792623639521768 ) ) ;
#86664=VECTOR ( 'NONE', #44805, 1000.000000000000000 ) ;
#86665=ORIENTED_EDGE ( 'NONE', *, *, #86306, .T. ) ;
#86667=DIRECTION ( 'NONE',  ( -0.1305261922200445512, 0.000000000000000000, -0.9914448613738113814 ) ) ;
#86671=CARTESIAN_POINT ( 'NONE',  ( 6.898461952320431578, 15.00000000000000000, -12.75387089053309175 ) ) ;
#86672=PLANE ( 'NONE',  #26164 ) ;
#86676=CARTESIAN_POINT ( 'NONE',  ( 7.964842623401181321, -35.06131465584515183, 7.964842623401174215 ) ) ;
#86688=VERTEX_POINT ( 'NONE', #52790 ) ;
#86693=DIRECTION ( 'NONE',  ( -0.7716245833877148907, 0.000000000000000000, -0.6360782202777701677 ) ) ;
#86699=EDGE_LOOP ( 'NONE', ( #60748, #80213, #28968, #66582 ) ) ;
#86708=VECTOR ( 'NONE', #51835, 1000.000000000000114 ) ;
#86709=CARTESIAN_POINT ( 'NONE',  ( 12.00809552683952752, 15.00000000000000000, 8.989195838243626113 ) ) ;
#86715=CARTESIAN_POINT ( 'NONE',  ( 0.000000000000000000, 14.49999999999999822, 0.000000000000000000 ) ) ;
#86726=EDGE_CURVE ( 'NONE', #68457, #89588, #14320, .T. ) ;
#86728=CARTESIAN_POINT ( 'NONE',  ( -4.391347328462822830, 0.2301508954901552439, -14.28069739540086580 ) ) ;
#86734=ORIENTED_EDGE ( 'NONE', *, *, #71994, .F. ) ;
#86735=CARTESIAN_POINT ( 'NONE',  ( -6.689969769698787871, -0.03417435944610275333, -12.58200319823979285 ) ) ;
#86745=CARTESIAN_POINT ( 'NONE',  ( 3.434112377981060948, 0.5819680032637514211, 12.81628187352647430 ) ) ;
#86748=ORIENTED_EDGE ( 'NONE', *, *, #37970, .F. ) ;
#86755=LINE ( 'NONE', #18260, #49575 ) ;
#86758=VECTOR ( 'NONE', #84960, 1000.000000000000114 ) ;
#86760=CYLINDRICAL_SURFACE ( 'NONE', #75527, 15.00000000000000000 ) ;
#86763=VECTOR ( 'NONE', #34347, 1000.000000000000000 ) ;
#86766=DIRECTION ( 'NONE',  ( -0.000000000000000000, -1.000000000000000000, -0.000000000000000000 ) ) ;
#86772=VECTOR ( 'NONE', #90019, 1000.000000000000000 ) ;
#86775=DIRECTION ( 'NONE',  ( 0.000000000000000000, 1.000000000000000000, 0.000000000000000000 ) ) ;
#86778=CARTESIAN_POINT ( 'NONE',  ( -9.898881779040801021, 15.00000000000000000, 10.25059215482569641 ) ) ;
#86783=( LENGTH_UNIT ( ) NAMED_UNIT ( * ) SI_UNIT ( .MILLI., .METRE. ) );
#86791=CARTESIAN_POINT ( 'NONE',  ( -5.817157072110894056, 14.63595249122789177, 13.82608706751083893 ) ) ;
#86795=DIRECTION ( 'NONE',  ( -0.8788171126619616080, 0.000000000000000000, -0.4771587602596153999 ) ) ;
#86798=CARTESIAN_POINT ( 'NONE',  ( -1.548803529117957822, 0.000000000000000000, -5.228673087012116305 ) ) ;
#86815=ORIENTED_EDGE ( 'NONE', *, *, #24182, .F. ) ;
#86816=DIRECTION ( 'NONE',  ( 0.000000000000000000, 1.000000000000000000, 0.000000000000000000 ) ) ;
#86817=CARTESIAN_POINT ( 'NONE',  ( 2.913501739333762774, 15.00000000000000000, -14.20427779279532565 ) ) ;
#86826=CARTESIAN_POINT ( 'NONE',  ( -12.00809552683969272, 14.63606912728209508, 8.989195838243468017 ) ) ;
#86840=EDGE_CURVE ( 'NONE', #91650, #71473, #26580, .T. ) ;
#86843=DIRECTION ( 'NONE',  ( -0.000000000000000000, 1.000000000000000000, -0.000000000000000000 ) ) ;
#86850=VERTEX_POINT ( 'NONE', #27714 ) ;
#86853=VERTEX_POINT ( 'NONE', #57224 ) ;
#86856=CARTESIAN_POINT ( 'NONE',  ( 0.000000000000000000, 0.5000000000000004441, 0.000000000000000000 ) ) ;
#86863=ORIENTED_EDGE ( 'NONE', *, *, #43644, .T. ) ;
#86873=FACE_OUTER_BOUND ( 'NONE', #70757, .T. ) ;
#86883=CARTESIAN_POINT ( 'NONE',  ( 5.056330833731752072, 3.901243639414221473E-16, -13.58983143750699973 ) ) ;
#86886=DIRECTION ( 'NONE',  ( 0.000000000000000000, 0.000000000000000000, 1.000000000000000000 ) ) ;
#86888=ORIENTED_EDGE ( 'NONE', *, *, #93932, .T. ) ;
#86893=CARTESIAN_POINT ( 'NONE',  ( -14.02068044289389626, 14.49999999999999112, 5.331089937175563342 ) ) ;
#86896=CARTESIAN_POINT ( 'NONE',  ( 13.48086198287162141, 15.00000000000000000, 8.610676897597548063 ) ) ;
#86897=CIRCLE ( 'NONE', #43785, 15.00000000000000000 ) ;
#86903=DIRECTION ( 'NONE',  ( 0.000000000000000000, 0.000000000000000000, 1.000000000000000000 ) ) ;
#86906=VERTEX_POINT ( 'NONE', #58196 ) ;
#86908=DIRECTION ( 'NONE',  ( 0.000000000000000000, 0.000000000000000000, 1.000000000000000000 ) ) ;
#86909=CARTESIAN_POINT ( 'NONE',  ( 0.000000000000000000, 15.00000000000000000, 0.000000000000000000 ) ) ;
#86913=B_SPLINE_CURVE_WITH_KNOTS ( 'NONE', 3,
 ( #42406, #72883, #81377, #80891, #43858, #27878 ),
 .UNSPECIFIED., .F., .F.,
 ( 4, 2, 4 ),
 ( 0.0002800154274984798615, 0.0006862208078247625676, 0.001092426188151045165 ),
 .UNSPECIFIED. ) ;
#86914=CARTESIAN_POINT ( 'NONE',  ( 12.26659068614894466, 9.720415501580641049, -7.082119434687053960 ) ) ;
#86921=CARTESIAN_POINT ( 'NONE',  ( -6.189644032515588812, 14.95077488074853456, -13.39157970158804645 ) ) ;
#86929=CARTESIAN_POINT ( 'NONE',  ( -1.114591949025129258, 15.00000000000000000, 14.45709807627963706 ) ) ;
#86936=VERTEX_POINT ( 'NONE', #4738 ) ;
#86947=CARTESIAN_POINT ( 'NONE',  ( 3.420591144908486481, 14.49999999999999112, 14.60477854057964109 ) ) ;
#86960=CARTESIAN_POINT ( 'NONE',  ( 12.60874940350942985, 3.897725180921639224E-16, 7.160268045227119238 ) ) ;
#86963=DIRECTION ( 'NONE',  ( 0.000000000000000000, 0.000000000000000000, 1.000000000000000000 ) ) ;
#86974=DIRECTION ( 'NONE',  ( 0.000000000000000000, 0.000000000000000000, 1.000000000000000000 ) ) ;
#86976=CARTESIAN_POINT ( 'NONE',  ( -3.434112377981047626, -34.83469866340291077, 12.81628187352647963 ) ) ;
#86977=VERTEX_POINT ( 'NONE', #51211 ) ;
#86987=EDGE_CURVE ( 'NONE', #60992, #1556, #29707, .T. ) ;
#86995=EDGE_CURVE ( 'NONE', #62224, #2288, #76047, .T. ) ;
#86998=CARTESIAN_POINT ( 'NONE',  ( 14.97687855664609202, 14.63595249122789177, -0.8325315005900555398 ) ) ;
#87003=CARTESIAN_POINT ( 'NONE',  ( -4.850097797904361130, 0.04962897333335897221, 13.93319274793799600 ) ) ;
#87011=CARTESIAN_POINT ( 'NONE',  ( 0.000000000000000000, 15.00000000000000000, 0.000000000000000000 ) ) ;
#87026=ADVANCED_FACE ( 'NONE', ( #4246 ), #51711, .F. ) ;
#87028=CARTESIAN_POINT ( 'NONE',  ( -14.16423886937410082, -33.19625116508603213, 4.336808689942017736E-15 ) ) ;
#87039=( BOUNDED_CURVE ( )  B_SPLINE_CURVE ( 2, ( #14793, #75760, #61730, #82269, #74776, #92248, #52273, #76262, #37293, #82771, #15771, #38274, #97810 ),
 .UNSPECIFIED., .F., .F. ) 
 B_SPLINE_CURVE_WITH_KNOTS ( ( 3, 2, 2, 2, 2, 2, 3 ),
 ( 0.5666666666666666519, 0.5722222222222221877, 0.5777777777777777235, 0.5833333333333333703, 0.5888888888888889062, 0.5944444444444444420, 0.5999999999999999778 ),
 .UNSPECIFIED. ) 
 CURVE ( )  GEOMETRIC_REPRESENTATION_ITEM ( )  RATIONAL_B_SPLINE_CURVE ( ( 1.000000000000000000, 0.9659258262890683122, 1.000000000000000000, 0.9659258262890683122, 1.000000000000000000, 0.9659258262890683122, 1.000000000000000000, 0.9659258262890683122, 1.000000000000000000, 0.9659258262890683122, 1.000000000000000000, 0.9659258262890683122, 1.000000000000000000 ) ) 
 REPRESENTATION_ITEM ( '' )  );
#87041=CARTESIAN_POINT ( 'NONE',  ( 13.82192141328807011, 15.00000000000000000, 4.382292601468777526 ) ) ;
#87047=CARTESIAN_POINT ( 'NONE',  ( -9.422509992056145478, 12.64701867748818032, -5.440088680355541939 ) ) ;
#87050=CARTESIAN_POINT ( 'NONE',  ( -11.62006642627350672, -3.693487166502375051E-15, -8.881585844847300848 ) ) ;
#87052=CARTESIAN_POINT ( 'NONE',  ( -13.61464873478158211, 0.5000000000000004441, -6.296136897218027606 ) ) ;
#87058=EDGE_CURVE ( 'NONE', #38990, #71998, #51559, .T. ) ;
#87076=LINE ( 'NONE', #19564, #4351 ) ;
#87079=CARTESIAN_POINT ( 'NONE',  ( 12.60589901313221439, 15.00000000000000000, -8.129656208642048298 ) ) ;
#87084=AXIS2_PLACEMENT_3D ( 'NONE', #4180, #89142, #42663 ) ;
#87093=CARTESIAN_POINT ( 'NONE',  ( -9.846743663894594434, 1.008931151000792781, 3.469446951953614189E-15 ) ) ;
#87096=VERTEX_POINT ( 'NONE', #76666 ) ;
#87101=CARTESIAN_POINT ( 'NONE',  ( 14.17193700899789022, -0.03417435944610275333, 1.489530601564113654 ) ) ;
#87102=EDGE_CURVE ( 'NONE', #97319, #39036, #16174, .T. ) ;
#87109=VERTEX_POINT ( 'NONE', #30664 ) ;
#87115=AXIS2_PLACEMENT_3D ( 'NONE', #94161, #79160, #39216 ) ;
#87117=ORIENTED_EDGE ( 'NONE', *, *, #14262, .T. ) ;
#87120=CARTESIAN_POINT ( 'NONE',  ( 14.71525861348289865, 15.00000000000000000, -2.908807992686582633 ) ) ;
#87122=EDGE_CURVE ( 'NONE', #90793, #54280, #25366, .T. ) ;
#87123=DIRECTION ( 'NONE',  ( 0.000000000000000000, 1.000000000000000000, 0.000000000000000000 ) ) ;
#87130=CARTESIAN_POINT ( 'NONE',  ( -7.771322705638593398, 15.00000000000000000, 12.24159072200411380 ) ) ;
#87133=CARTESIAN_POINT ( 'NONE',  ( -1.820328553599896981, 0.000000000000000000, -5.140449258537809207 ) ) ;
#87138=ORIENTED_EDGE ( 'NONE', *, *, #64037, .F. ) ;
#87145=DIRECTION ( 'NONE',  ( 0.000000000000000000, 0.000000000000000000, 1.000000000000000000 ) ) ;
#87149=CARTESIAN_POINT ( 'NONE',  ( -9.422509992056145478, -22.35298132251182324, -5.440088680355541939 ) ) ;
#87153=CARTESIAN_POINT ( 'NONE',  ( 8.502626202121271959, 0.04922511925147034229, 12.05617882333543633 ) ) ;
#87158=AXIS2_PLACEMENT_3D ( 'NONE', #52408, #67413, #82909 ) ;
#87174=VERTEX_POINT ( 'NONE', #7198 ) ;
#87175=ADVANCED_FACE ( 'NONE', ( #37701 ), #84667, .T. ) ;
#87180=LINE ( 'NONE', #57170, #46151 ) ;
#87190=FACE_OUTER_BOUND ( 'NONE', #45117, .T. ) ;
#87196=FACE_OUTER_BOUND ( 'NONE', #33497, .T. ) ;
#87202=CARTESIAN_POINT ( 'NONE',  ( 0.000000000000000000, 0.5000000000000004441, 0.000000000000000000 ) ) ;
#87203=CARTESIAN_POINT ( 'NONE',  ( 6.715867195167361636, 15.00000000000000000, 12.85095824508331930 ) ) ;
#87206=CARTESIAN_POINT ( 'NONE',  ( -4.923371831947292776, -38.15773551566587685, 8.527530157486181039 ) ) ;
#87207=VERTEX_POINT ( 'NONE', #69182 ) ;
#87209=ORIENTED_EDGE ( 'NONE', *, *, #19577, .T. ) ;
#87211=ORIENTED_EDGE ( 'NONE', *, *, #87350, .T. ) ;
#87212=TOROIDAL_SURFACE ( 'NONE', #13779, 14.49999999999999822, 0.5000000000000000000 ) ;
#87219=CARTESIAN_POINT ( 'NONE',  ( -9.382169495545413795, -10.25136533006957507, 9.382169495545428006 ) ) ;
#87228=CARTESIAN_POINT ( 'NONE',  ( 14.82629065241269473, 0.2301504708692996282, -1.844815641835253928 ) ) ;
#87229=DIRECTION ( 'NONE',  ( 0.9723699203976742256, 0.000000000000000000, 0.2334453638559156052 ) ) ;
#87232=ADVANCED_FACE ( 'NONE', ( #52198 ), #52071, .T. ) ;
#87233=AXIS2_PLACEMENT_3D ( 'NONE', #79782, #41322, #11284 ) ;
#87234=AXIS2_PLACEMENT_3D ( 'NONE', #9303, #78289, #7845 ) ;
#87237=DIRECTION ( 'NONE',  ( 0.000000000000000000, 0.000000000000000000, 1.000000000000000000 ) ) ;
#87241=DIRECTION ( 'NONE',  ( 0.8433914458128849434, 0.000000000000000000, 0.5372996083468249973 ) ) ;
#87250=EDGE_CURVE ( 'NONE', #89676, #4865, #61649, .T. ) ;
#87259=EDGE_CURVE ( 'NONE', #41402, #37243, #65881, .T. ) ;
#87276=LINE ( 'NONE', #24340, #32180 ) ;
#87282=LINE ( 'NONE', #78807, #33932 ) ;
#87285=CARTESIAN_POINT ( 'NONE',  ( -8.439016546561676435, 15.00000000000000000, -11.79122553965791553 ) ) ;
#87286=VECTOR ( 'NONE', #62475, 1000.000000000000000 ) ;
#87299=CARTESIAN_POINT ( 'NONE',  ( 0.000000000000000000, 15.00000000000000000, 0.000000000000000000 ) ) ;
#87316=FACE_OUTER_BOUND ( 'NONE', #33006, .T. ) ;
#87317=CIRCLE ( 'NONE', #44194, 15.00000000000000000 ) ;
#87322=CARTESIAN_POINT ( 'NONE',  ( -14.94699059465102664, 0.5000000000000004441, 1.259949270174715696 ) ) ;
#87326=VERTEX_POINT ( 'NONE', #83686 ) ;
#87328=AXIS2_PLACEMENT_3D ( 'NONE', #38749, #7767, #90748 ) ;
#87330=VERTEX_POINT ( 'NONE', #15203 ) ;
#87339=CARTESIAN_POINT ( 'NONE',  ( -5.204170427930422072E-15, 11.41212336850781739, -11.92686044187656513 ) ) ;
#87350=EDGE_CURVE ( 'NONE', #47878, #1561, #10527, .T. ) ;
#87355=CARTESIAN_POINT ( 'NONE',  ( -9.705452947461587598, 2.500000000000008438, -5.689172442861014645 ) ) ;
#87358=ADVANCED_FACE ( 'NONE', ( #33610 ), #26134, .F. ) ;
#87361=CARTESIAN_POINT ( 'NONE',  ( 0.000000000000000000, 0.5000000000000004441, 0.000000000000000000 ) ) ;
#87365=ORIENTED_EDGE ( 'NONE', *, *, #45729, .T. ) ;
#87366=LINE ( 'NONE', #94863, #86763 ) ;
#87373=CARTESIAN_POINT ( 'NONE',  ( 13.95806775979399461, 2.168404344971008868E-16, -4.371577651620736304 ) ) ;
#87380=EDGE_CURVE ( 'NONE', #88318, #85778, #40648, .T. ) ;
#87387=ADVANCED_FACE ( 'NONE', ( #48132 ), #70167, .T. ) ;
#87395=CARTESIAN_POINT ( 'NONE',  ( 0.000000000000000000, 14.49999999999999822, 0.000000000000000000 ) ) ;
#87396=CARTESIAN_POINT ( 'NONE',  ( 14.97687855664608314, 15.00000000000000000, -0.8325315005900512100 ) ) ;
#87403=LINE ( 'NONE', #80398, #55429 ) ;
#87408=CARTESIAN_POINT ( 'NONE',  ( -14.61146088927471176, 15.00000000000000711, 0.6660010753333497346 ) ) ;
#87420=DIRECTION ( 'NONE',  ( 0.000000000000000000, 0.000000000000000000, -1.000000000000000000 ) ) ;
#87427=ORIENTED_EDGE ( 'NONE', *, *, #1974, .T. ) ;
#87434=AXIS2_PLACEMENT_3D ( 'NONE', #12355, #88358, #50347 ) ;
#87439=DIRECTION ( 'NONE',  ( 0.000000000000000000, 1.000000000000000000, 0.000000000000000000 ) ) ;
#87450=CARTESIAN_POINT ( 'NONE',  ( -5.377205135395773716, 14.76930270348882068, -13.94000429068789160 ) ) ;
#87467=CARTESIAN_POINT ( 'NONE',  ( 11.09922568453595026, -33.79303199673624647, 6.408140936763232709 ) ) ;
#87469=ORIENTED_EDGE ( 'NONE', *, *, #9279, .F. ) ;
#87477=EDGE_CURVE ( 'NONE', #91030, #47550, #47652, .T. ) ;
#87483=CARTESIAN_POINT ( 'NONE',  ( -5.795997163830251431, 15.00000000000000000, 13.01802277140702024 ) ) ;
#87486=VERTEX_POINT ( 'NONE', #39177 ) ;
#87489=CARTESIAN_POINT ( 'NONE',  ( 14.09394518620607428, 15.00000000000000000, 3.407449058785458451 ) ) ;
#87497=ORIENTED_EDGE ( 'NONE', *, *, #47875, .T. ) ;
#87499=ADVANCED_FACE ( 'NONE', ( #54645 ), #20224, .T. ) ;
#87501=ORIENTED_EDGE ( 'NONE', *, *, #74680, .T. ) ;
#87506=CARTESIAN_POINT ( 'NONE',  ( 2.120353041430552921, 4.509079855230530718E-16, 14.34413130794947122 ) ) ;
#87520=CARTESIAN_POINT ( 'NONE',  ( 12.26659068614894821, -31.11291783175269643, 7.082119434687044190 ) ) ;
#87523=ORIENTED_EDGE ( 'NONE', *, *, #17287, .F. ) ;
#87524=ORIENTED_EDGE ( 'NONE', *, *, #66459, .T. ) ;
#87531=CARTESIAN_POINT ( 'NONE',  ( 15.67879934938582664, -0.03417435944610275333, -3.170591017105818921 ) ) ;
#87537=CARTESIAN_POINT ( 'NONE',  ( 9.422509992056141925, 20.98035201082151957, -5.440088680355554374 ) ) ;
#87540=EDGE_CURVE ( 'NONE', #89266, #65919, #71145, .T. ) ;
#87551=CARTESIAN_POINT ( 'NONE',  ( -12.00809552683965187, 0.5000000000000004441, 8.989195838243462688 ) ) ;
#87552=DIRECTION ( 'NONE',  ( -0.000000000000000000, 1.000000000000000000, -0.000000000000000000 ) ) ;
#87554=ORIENTED_EDGE ( 'NONE', *, *, #23056, .F. ) ;
#87563=CARTESIAN_POINT ( 'NONE',  ( -4.862001128006864903, 4.306586084822671512E-16, 13.66056166602457012 ) ) ;
#87567=ORIENTED_EDGE ( 'NONE', *, *, #93846, .F. ) ;
#87568=ORIENTED_EDGE ( 'NONE', *, *, #49280, .F. ) ;
#87573=FACE_OUTER_BOUND ( 'NONE', #79599, .T. ) ;
#87577=LINE ( 'NONE', #71118, #38106 ) ;
#87578=CARTESIAN_POINT ( 'NONE',  ( -2.638427012816840111, -0.03273551566588039224, -9.846743663894590881 ) ) ;
#87579=VERTEX_POINT ( 'NONE', #40152 ) ;
#87582=ORIENTED_EDGE ( 'NONE', *, *, #66946, .T. ) ;
#87592=ORIENTED_EDGE ( 'NONE', *, *, #55233, .F. ) ;
#87603=VECTOR ( 'NONE', #90687, 1000.000000000000000 ) ;
#87604=LINE ( 'NONE', #4625, #90443 ) ;
#87605=EDGE_CURVE ( 'NONE', #15967, #19871, #83790, .T. ) ;
#87610=CARTESIAN_POINT ( 'NONE',  ( 1.354709868695618935, 15.00000000000000000, -14.93870011653151586 ) ) ;
#87613=CARTESIAN_POINT ( 'NONE',  ( 1.829604203029677523, 15.00000000000000000, -15.89119079541585755 ) ) ;
#87619=CARTESIAN_POINT ( 'NONE',  ( 0.000000000000000000, 0.5000000000000004441, 0.000000000000000000 ) ) ;
#87637=CARTESIAN_POINT ( 'NONE',  ( 10.56735866240293653, 12.77290477899395071, -4.606545654699560899 ) ) ;
#87639=DIRECTION ( 'NONE',  ( -0.5224985647159436919, 0.000000000000000000, -0.8526401643540955089 ) ) ;
#87640=AXIS2_PLACEMENT_3D ( 'NONE', #84130, #76124, #46124 ) ;
#87643=CARTESIAN_POINT ( 'NONE',  ( -5.440088680355547268, -31.10298132251182324, 9.422509992056143702 ) ) ;
#87647=CARTESIAN_POINT ( 'NONE',  ( 12.87930560075675324, 14.95037102969557452, -7.195887444332383254 ) ) ;
#87648=CARTESIAN_POINT ( 'NONE',  ( -13.34343830728398927, 14.49999999999999112, -6.852200678592835104 ) ) ;
#87650=ADVANCED_FACE ( 'NONE', ( #1192 ), #93140, .F. ) ;
#87659=CARTESIAN_POINT ( 'NONE',  ( 6.138934250732054565, -0.03417435944610275333, -14.77128574976607389 ) ) ;
#87662=ORIENTED_EDGE ( 'NONE', *, *, #39906, .T. ) ;
#87663=CARTESIAN_POINT ( 'NONE',  ( 4.326345305608651159, 0.000000000000000000, -3.319721512309584011 ) ) ;
#87677=EDGE_LOOP ( 'NONE', ( #57930, #74814, #34117, #62547 ) ) ;
#87691=DIRECTION ( 'NONE',  ( -0.000000000000000000, -1.000000000000000000, -0.000000000000000000 ) ) ;
#87693=CARTESIAN_POINT ( 'NONE',  ( -8.527530157486173934, -38.57440218233254825, 4.923371831947302546 ) ) ;
#87695=CARTESIAN_POINT ( 'NONE',  ( 0.000000000000000000, 15.00000000000000000, 0.000000000000000000 ) ) ;
#87708=CARTESIAN_POINT ( 'NONE',  ( -11.09922568453595382, 13.70696800326375708, -6.408140936763226492 ) ) ;
#87709=VERTEX_POINT ( 'NONE', #95102 ) ;
#87711=ORIENTED_EDGE ( 'NONE', *, *, #47881, .F. ) ;
#87722=VECTOR ( 'NONE', #81389, 1000.000000000000114 ) ;
#87724=EDGE_CURVE ( 'NONE', #4086, #30837, #81580, .T. ) ;
#87727=LINE ( 'NONE', #82698, #87603 ) ;
#87731=CARTESIAN_POINT ( 'NONE',  ( 3.384800920124170887, 0.2306972965111907803, -14.55270344038008190 ) ) ;
#87738=CARTESIAN_POINT ( 'NONE',  ( 9.898881779040660689, 15.00000000000000000, 10.25059215482582786 ) ) ;
#87741=DIRECTION ( 'NONE',  ( 0.4617486132350405170, 0.000000000000000000, -0.8870108331782183830 ) ) ;
#87746=CARTESIAN_POINT ( 'NONE',  ( 14.74963345907814372, 14.95077488074853456, 0.3072669459661709346 ) ) ;
#87761=CARTESIAN_POINT ( 'NONE',  ( -12.00809552683965720, 0.3640475087720476677, 8.989195838243462688 ) ) ;
#87763=DIRECTION ( 'NONE',  ( 0.000000000000000000, 0.000000000000000000, 1.000000000000000000 ) ) ;
#87764=EDGE_CURVE ( 'NONE', #71459, #27523, #38457, .T. ) ;
#87774=CARTESIAN_POINT ( 'NONE',  ( 5.056330833731640162, 15.00000000000000000, 13.58983143750701394 ) ) ;
#87779=ORIENTED_EDGE ( 'NONE', *, *, #6348, .T. ) ;
#87794=CARTESIAN_POINT ( 'NONE',  ( -4.431036607602373500, 0.5000000000000004441, -14.33059365769916838 ) ) ;
#87799=LINE ( 'NONE', #20306, #27830 ) ;
#87815=ORIENTED_EDGE ( 'NONE', *, *, #92072, .T. ) ;
#87817=EDGE_CURVE ( 'NONE', #21605, #11587, #87604, .T. ) ;
#87831=ORIENTED_EDGE ( 'NONE', *, *, #88779, .T. ) ;
#87835=CARTESIAN_POINT ( 'NONE',  ( -13.61912076658538240, 15.00000000000000711, -5.334594295381093865 ) ) ;
#87843=CARTESIAN_POINT ( 'NONE',  ( -3.897244926436033374, 15.00000000000000000, -13.96644127841335958 ) ) ;
#87852=CARTESIAN_POINT ( 'NONE',  ( -9.898881779040587858, 15.00000000000000000, -10.25059215482589714 ) ) ;
#87857=DIRECTION ( 'NONE',  ( 0.000000000000000000, 0.000000000000000000, 1.000000000000000000 ) ) ;
#87870=CARTESIAN_POINT ( 'NONE',  ( 8.564643372776618691, 14.63595249122790598, -12.31449893000741369 ) ) ;
#87885=CIRCLE ( 'NONE', #44787, 14.49999999999999822 ) ;
#87886=ORIENTED_EDGE ( 'NONE', *, *, #74975, .F. ) ;
#87899=AXIS2_PLACEMENT_3D ( 'NONE', #36025, #45002, #68017 ) ;
#87905=FACE_OUTER_BOUND ( 'NONE', #77142, .T. ) ;
#87906=CARTESIAN_POINT ( 'NONE',  ( 4.431036607602565347, 0.3640475087720985159, -14.33059365769911864 ) ) ;
#87913=AXIS2_PLACEMENT_3D ( 'NONE', #93241, #33709, #24767 ) ;
#87915=ADVANCED_FACE ( 'NONE', ( #67085 ), #82077, .F. ) ;
#87922=CARTESIAN_POINT ( 'NONE',  ( -4.838527690343710219, 14.49999999999999112, 14.19819177887730355 ) ) ;
#87923=ORIENTED_EDGE ( 'NONE', *, *, #12207, .T. ) ;
#87925=CARTESIAN_POINT ( 'NONE',  ( 10.19513985507828302, 14.49999999999999112, 11.00268709613230200 ) ) ;
#87931=ORIENTED_EDGE ( 'NONE', *, *, #60181, .F. ) ;
#87935=DIRECTION ( 'NONE',  ( 0.000000000000000000, 0.000000000000000000, -1.000000000000000000 ) ) ;
#87938=DIRECTION ( 'NONE',  ( 0.000000000000000000, 1.000000000000000000, 0.000000000000000000 ) ) ;
#87943=CARTESIAN_POINT ( 'NONE',  ( -8.439016546559974685, 15.00000000000000000, 11.79122553964965014 ) ) ;
#87949=CARTESIAN_POINT ( 'NONE',  ( 5.795997163830165277, 0.000000000000000000, -13.01802277140705932 ) ) ;
#87954=CARTESIAN_POINT ( 'NONE',  ( -11.09922568453595382, -31.29303199673623936, -6.408140936763226492 ) ) ;
#87966=VERTEX_POINT ( 'NONE', #53056 ) ;
#87971=AXIS2_PLACEMENT_3D ( 'NONE', #98291, #14281, #60255 ) ;
#87973=EDGE_CURVE ( 'NONE', #59795, #54039, #68079, .T. ) ;
#87974=EDGE_LOOP ( 'NONE', ( #72089, #75784, #23363, #14713, #29345, #64760 ) ) ;
#87980=CARTESIAN_POINT ( 'NONE',  ( 0.000000000000000000, 0.5000000000000004441, 0.000000000000000000 ) ) ;
#87983=ORIENTED_EDGE ( 'NONE', *, *, #77791, .F. ) ;
#87984=DIRECTION ( 'NONE',  ( 0.6225146366376183016, 0.000000000000000000, -0.7826081568524148047 ) ) ;
#87987=ORIENTED_EDGE ( 'NONE', *, *, #55694, .F. ) ;
#87990=CARTESIAN_POINT ( 'NONE',  ( 2.361121941889016362, 0.2301505397289888843, 14.75287579053850706 ) ) ;
#87992=B_SPLINE_CURVE_WITH_KNOTS ( 'NONE', 3,
 ( #19996, #81977, #82473, #72993, #73479, #13489 ),
 .UNSPECIFIED., .F., .F.,
 ( 4, 2, 4 ),
 ( 3.409110551421259754E-05, 0.0004400426677360415621, 0.0008459942299578705402 ),
 .UNSPECIFIED. ) ;
#88002=VECTOR ( 'NONE', #82358, 1000.000000000000000 ) ;
#88009=CARTESIAN_POINT ( 'NONE',  ( -3.795296366450322534, -39.23791783175269643, -14.16423886937409904 ) ) ;
#88011=VECTOR ( 'NONE', #91477, 1000.000000000000000 ) ;
#88013=VERTEX_POINT ( 'NONE', #38567 ) ;
#88023=CARTESIAN_POINT ( 'NONE',  ( -2.915334737309934532, 17.02201867748817321, -10.88017736071109987 ) ) ;
#88024=CARTESIAN_POINT ( 'NONE',  ( -12.00809552683946357, 0.5000000000000004441, -8.989195838243713155 ) ) ;
#88025=AXIS2_PLACEMENT_3D ( 'NONE', #43721, #36225, #21227 ) ;
#88028=CARTESIAN_POINT ( 'NONE',  ( 0.000000000000000000, 15.00000000000000000, 0.000000000000000000 ) ) ;
#88030=CIRCLE ( 'NONE', #76827, 14.49999999999999822 ) ;
#88044=DIRECTION ( 'NONE',  ( -0.3987490689252404241, 0.000000000000000000, -0.9170600743851266001 ) ) ;
#88051=LINE ( 'NONE', #19073, #26660 ) ;
#88065=EDGE_CURVE ( 'NONE', #40449, #45767, #17785, .T. ) ;
#88066=CARTESIAN_POINT ( 'NONE',  ( 0.000000000000000000, 15.00000000000000000, 0.000000000000000000 ) ) ;
#88068=CARTESIAN_POINT ( 'NONE',  ( -4.923371831947302546, 5.175597817667458855, -8.527530157486173934 ) ) ;
#88069=ORIENTED_EDGE ( 'NONE', *, *, #20020, .F. ) ;
#88071=ORIENTED_EDGE ( 'NONE', *, *, #78811, .F. ) ;
#88080=CARTESIAN_POINT ( 'NONE',  ( 15.94536257719940409, 15.00000000000000000, 1.273895096820067296 ) ) ;
#88094=CARTESIAN_POINT ( 'NONE',  ( 1.354709868695531894, 0.3639309939382489034, 14.93870011653156027 ) ) ;
#88104=CARTESIAN_POINT ( 'NONE',  ( 12.07856007377828078, 15.00000000000000000, -8.022367888854837759 ) ) ;
#88105=AXIS2_PLACEMENT_3D ( 'NONE', #8777, #334, #39294 ) ;
#88108=PLANE ( 'NONE',  #96906 ) ;
#88112=ORIENTED_EDGE ( 'NONE', *, *, #95985, .F. ) ;
#88113=CARTESIAN_POINT ( 'NONE',  ( -7.264948169187551485, 0.2306972965111897256, 13.05597881399713955 ) ) ;
#88114=VECTOR ( 'NONE', #24573, 1000.000000000000000 ) ;
#88122=DIRECTION ( 'NONE',  ( 0.000000000000000000, -1.000000000000000000, 0.000000000000000000 ) ) ;
#88129=CARTESIAN_POINT ( 'NONE',  ( 11.32537994190320418, 12.61453919175019678, -1.000888968711507676 ) ) ;
#88132=CARTESIAN_POINT ( 'NONE',  ( -4.431036607602414357, 14.49999999999999112, -14.33059365769922167 ) ) ;
#88135=CARTESIAN_POINT ( 'NONE',  ( 7.964842623401181321, -20.06131465584516249, 7.964842623401174215 ) ) ;
#88139=CARTESIAN_POINT ( 'NONE',  ( -4.746257547686163925, 0.000000000000000000, -2.685303318749144186 ) ) ;
#88146=AXIS2_PLACEMENT_3D ( 'NONE', #47732, #33695, #79710 ) ;
#88151=CARTESIAN_POINT ( 'NONE',  ( -8.375939845167600595, 15.00000000000000000, -11.52849216984310310 ) ) ;
#88157=DIRECTION ( 'NONE',  ( 0.000000000000000000, 0.000000000000000000, 1.000000000000000000 ) ) ;
#88163=CARTESIAN_POINT ( 'NONE',  ( -13.55255535720598026, 15.00000000000000000, 4.403492169842870396 ) ) ;
#88164=CARTESIAN_POINT ( 'NONE',  ( 7.882504294823946545, 2.625802136488331051E-16, -12.32089577884791787 ) ) ;
#88166=TOROIDAL_SURFACE ( 'NONE', #45064, 14.49999999999999822, 0.5000000000000000000 ) ;
#88170=VERTEX_POINT ( 'NONE', #62776 ) ;
#88171=CARTESIAN_POINT ( 'NONE',  ( 3.014428414850127691, 11.46346884451820713, -11.25000000000000000 ) ) ;
#88184=CARTESIAN_POINT ( 'NONE',  ( -2.815433093576926282, 0.3640475087720981828, -14.73340885523754196 ) ) ;
#88186=CARTESIAN_POINT ( 'NONE',  ( 0.8218345515129070744, 14.95077488074852923, -14.72992491912910573 ) ) ;
#88189=CARTESIAN_POINT ( 'NONE',  ( -9.846743663894594434, -33.99106884899921255, 3.469446951953614189E-15 ) ) ;
#88203=CARTESIAN_POINT ( 'NONE',  ( 6.408140936763243367, 5.790301336597095450, 11.09922568453594494 ) ) ;
#88204=ORIENTED_EDGE ( 'NONE', *, *, #71251, .T. ) ;
#88208=EDGE_CURVE ( 'NONE', #10227, #59535, #11249, .T. ) ;
#88215=EDGE_CURVE ( 'NONE', #65562, #23769, #32764, .T. ) ;
#88216=CARTESIAN_POINT ( 'NONE',  ( -12.79448242979012562, 14.76930270348881002, 7.716169648622011046 ) ) ;
#88217=AXIS2_PLACEMENT_3D ( 'NONE', #76904, #24419, #37947 ) ;
#88219=DIRECTION ( 'NONE',  ( 0.000000000000000000, 0.000000000000000000, -1.000000000000000000 ) ) ;
#88220=CARTESIAN_POINT ( 'NONE',  ( 0.000000000000000000, 35.00000000000000000, 0.000000000000000000 ) ) ;
#88225=EDGE_CURVE ( 'NONE', #76195, #73208, #3771, .T. ) ;
#88227=CARTESIAN_POINT ( 'NONE',  ( -14.93928340878672323, 0.2306972965111904195, 0.2363597353048689786 ) ) ;
#88231=CARTESIAN_POINT ( 'NONE',  ( 0.000000000000000000, 15.00000000000000000, 0.000000000000000000 ) ) ;
#88235=DIRECTION ( 'NONE',  ( 0.000000000000000000, 0.000000000000000000, -1.000000000000000000 ) ) ;
#88236=ORIENTED_EDGE ( 'NONE', *, *, #65798, .F. ) ;
#88242=CARTESIAN_POINT ( 'NONE',  ( -2.393480905993250918, 0.5000000000000004441, 14.80781041047749724 ) ) ;
#88245=VERTEX_POINT ( 'NONE', #33733 ) ;
#88246=CARTESIAN_POINT ( 'NONE',  ( -9.742785792574931492, 5.534700295649322754, 5.625000000000008882 ) ) ;
#88250=LINE ( 'NONE', #80758, #31253 ) ;
#88265=B_SPLINE_CURVE_WITH_KNOTS ( 'NONE', 3,
 ( #65541, #41601, #95056, #4081, #48578, #64060 ),
 .UNSPECIFIED., .F., .F.,
 ( 4, 2, 4 ),
 ( 0.0002800065468475842123, 0.0006862118402974218614, 0.001092417133747259619 ),
 .UNSPECIFIED. ) ;
#88271=CARTESIAN_POINT ( 'NONE',  ( -12.83294900548052730, 0.5000000000000004441, -7.766300266068542513 ) ) ;
#88278=ORIENTED_EDGE ( 'NONE', *, *, #77829, .F. ) ;
#88283=AXIS2_PLACEMENT_3D ( 'NONE', #93363, #26339, #16394 ) ;
#88287=CARTESIAN_POINT ( 'NONE',  ( 2.962741594153077251, 15.00000000000000000, -13.93860331045673107 ) ) ;
#88297=ORIENTED_EDGE ( 'NONE', *, *, #26710, .T. ) ;
#88305=DIRECTION ( 'NONE',  ( -0.000000000000000000, -1.000000000000000000, -0.000000000000000000 ) ) ;
#88314=VERTEX_POINT ( 'NONE', #73220 ) ;
#88316=VERTEX_POINT ( 'NONE', #4748 ) ;
#88318=VERTEX_POINT ( 'NONE', #65718 ) ;
#88320=DIRECTION ( 'NONE',  ( -0.000000000000000000, -1.000000000000000000, -0.000000000000000000 ) ) ;
#88325=CARTESIAN_POINT ( 'NONE',  ( -10.32896413005680536, 12.24545670184114243, -5.963430220938272797 ) ) ;
#88333=VERTEX_POINT ( 'NONE', #43716 ) ;
#88336=CIRCLE ( 'NONE', #93115, 15.00000000000000000 ) ;
#88338=DIRECTION ( 'NONE',  ( -0.000000000000000000, -1.000000000000000000, -0.000000000000000000 ) ) ;
#88343=EDGE_CURVE ( 'NONE', #47253, #14084, #81297, .T. ) ;
#88346=CARTESIAN_POINT ( 'NONE',  ( -8.564643372776702179, 0.5000000000000004441, 12.31449893000734797 ) ) ;
#88350=B_SPLINE_CURVE_WITH_KNOTS ( 'NONE', 3,
 ( #82593, #52100, #7100, #58606, #44592, #36100 ),
 .UNSPECIFIED., .F., .F.,
 ( 4, 2, 4 ),
 ( 3.409110551496223525E-05, 0.0004400426677367995820, 0.0008459942299586368543 ),
 .UNSPECIFIED. ) ;
#88352=DIRECTION ( 'NONE',  ( 0.000000000000000000, 0.000000000000000000, 1.000000000000000000 ) ) ;
#88355=LINE ( 'NONE', #87852, #86708 ) ;
#88358=DIRECTION ( 'NONE',  ( -0.000000000000000000, -1.000000000000000000, -0.000000000000000000 ) ) ;
#88364=LINE ( 'NONE', #21349, #93623 ) ;
#88371=CARTESIAN_POINT ( 'NONE',  ( 9.742785792574933268, 8.034700295649317425, -5.625000000000003553 ) ) ;
#88374=B_SPLINE_CURVE_WITH_KNOTS ( 'NONE', 3,
 ( #77657, #70670, #48634, #94634, #18157, #63630 ),
 .UNSPECIFIED., .F., .F.,
 ( 4, 2, 4 ),
 ( 0.0002800518438628033847, 0.0006862575805706614372, 0.001092463317278519544 ),
 .UNSPECIFIED. ) ;
#88375=DIRECTION ( 'NONE',  ( 0.6087614290087186575, 0.000000000000000000, 0.7933533402912366084 ) ) ;
#88377=CARTESIAN_POINT ( 'NONE',  ( 12.79448242979007411, 14.76930270348881002, -7.716169648622100752 ) ) ;
#88381=DIRECTION ( 'NONE',  ( -0.4924235601034587240, 0.000000000000000000, -0.8703556959399044723 ) ) ;
#88392=AXIS2_PLACEMENT_3D ( 'NONE', #25465, #54451, #53969 ) ;
#88398=CARTESIAN_POINT ( 'NONE',  ( -2.393480905992944496, 0.5000000000000004441, -14.80781041047754520 ) ) ;
#88403=DIRECTION ( 'NONE',  ( 0.1132032137679171296, 0.000000000000000000, -0.9935718556765863463 ) ) ;
#88409=LINE ( 'NONE', #42422, #36682 ) ;
#88420=EDGE_CURVE ( 'NONE', #91650, #27523, #4256, .T. ) ;
#88426=CARTESIAN_POINT ( 'NONE',  ( 13.21236992757673789, 15.00000000000000000, -5.338143956176714333 ) ) ;
#88430=EDGE_CURVE ( 'NONE', #20387, #88013, #15607, .T. ) ;
#88437=CARTESIAN_POINT ( 'NONE',  ( -12.07856007377833407, 15.00000000000000000, 8.022367888854752493 ) ) ;
#88443=CARTESIAN_POINT ( 'NONE',  ( -8.549892366338930572, 14.76930270348881002, 12.25305656628349382 ) ) ;
#88453=CARTESIAN_POINT ( 'NONE',  ( 9.382169495545415572, -27.75136533006957862, -9.382169495545422677 ) ) ;
#88462=ORIENTED_EDGE ( 'NONE', *, *, #52392, .F. ) ;
#88472=B_SPLINE_CURVE_WITH_KNOTS ( 'NONE', 3,
 ( #7711, #92178, #37707, #8193, #29686, #23704 ),
 .UNSPECIFIED., .F., .F.,
 ( 4, 2, 4 ),
 ( 0.0002800011564896245269, 0.0006862063972211604468, 0.001092411637952696475 ),
 .UNSPECIFIED. ) ;
#88474=EDGE_CURVE ( 'NONE', #51046, #59600, #2528, .T. ) ;
#88481=DIRECTION ( 'NONE',  ( 0.000000000000000000, 0.000000000000000000, -1.000000000000000000 ) ) ;
#88483=ORIENTED_EDGE ( 'NONE', *, *, #9513, .F. ) ;
#88484=ORIENTED_EDGE ( 'NONE', *, *, #92124, .T. ) ;
#88488=LINE ( 'NONE', #34488, #71123 ) ;
#88494=ORIENTED_EDGE ( 'NONE', *, *, #1082, .F. ) ;
#88499=ORIENTED_EDGE ( 'NONE', *, *, #93931, .F. ) ;
#88505=CARTESIAN_POINT ( 'NONE',  ( -12.26659068614894110, -37.77958449841936783, 7.082119434687058401 ) ) ;
#88507=EDGE_CURVE ( 'NONE', #85704, #81651, #47810, .T. ) ;
#88511=EDGE_CURVE ( 'NONE', #1901, #32046, #59205, .T. ) ;
#88521=CARTESIAN_POINT ( 'NONE',  ( 9.422509992056141925, 20.14701867748818032, 5.440088680355547268 ) ) ;
#88524=ORIENTED_EDGE ( 'NONE', *, *, #19770, .T. ) ;
#88530=VECTOR ( 'NONE', #66969, 1000.000000000000000 ) ;
#88541=DIRECTION ( 'NONE',  ( -0.9170600743851266001, 0.000000000000000000, 0.3987490689252404241 ) ) ;
#88542=EDGE_CURVE ( 'NONE', #84080, #95213, #71736, .T. ) ;
#88549=CARTESIAN_POINT ( 'NONE',  ( 13.55157833323634797, 0.2306972965111905305, -6.292279346205384094 ) ) ;
#88553=ORIENTED_EDGE ( 'NONE', *, *, #88511, .F. ) ;
#88560=DIRECTION ( 'NONE',  ( 0.000000000000000000, 1.000000000000000000, -0.000000000000000000 ) ) ;
#88564=DIRECTION ( 'NONE',  ( 0.9762960071199360268, 0.000000000000000000, -0.2164396139380906636 ) ) ;
#88565=CARTESIAN_POINT ( 'NONE',  ( -2.638427012816824124, 7.050597817667457079, 9.846743663894596210 ) ) ;
#88567=ORIENTED_EDGE ( 'NONE', *, *, #65569, .T. ) ;
#88569=ORIENTED_EDGE ( 'NONE', *, *, #98157, .T. ) ;
#88577=ORIENTED_EDGE ( 'NONE', *, *, #13361, .F. ) ;
#88595=CARTESIAN_POINT ( 'NONE',  ( 0.000000000000000000, 0.5000000000000004441, 0.000000000000000000 ) ) ;
#88596=DIRECTION ( 'NONE',  ( -0.000000000000000000, -1.000000000000000000, -0.000000000000000000 ) ) ;
#88598=CARTESIAN_POINT ( 'NONE',  ( -3.115783986955370732, 3.816680036666981737E-16, -14.16128137375401685 ) ) ;
#88601=DIRECTION ( 'NONE',  ( 0.02617694830786938473, 0.000000000000000000, 0.9996573249755574819 ) ) ;
#88605=CARTESIAN_POINT ( 'NONE',  ( 6.728956594450806072, 15.00000000000000888, -12.98689685418140627 ) ) ;
#88606=VERTEX_POINT ( 'NONE', #7716 ) ;
#88609=DIRECTION ( 'NONE',  ( -0.9799247046208282574, 0.000000000000000000, -0.1993679344172039347 ) ) ;
#88614=AXIS2_PLACEMENT_3D ( 'NONE', #60242, #8718, #44742 ) ;
#88615=ORIENTED_EDGE ( 'NONE', *, *, #58593, .F. ) ;
#88616=ADVANCED_FACE ( 'NONE', ( #23211 ), #37875, .T. ) ;
#88622=DIRECTION ( 'NONE',  ( 0.000000000000000000, 0.000000000000000000, 1.000000000000000000 ) ) ;
#88628=CARTESIAN_POINT ( 'NONE',  ( 2.915334737309921209, -28.39464798917849819, -10.88017736071110164 ) ) ;
#88632=DIRECTION ( 'NONE',  ( 0.000000000000000000, 1.000000000000000000, 0.000000000000000000 ) ) ;
#88637=B_SPLINE_CURVE_WITH_KNOTS ( 'NONE', 3,
 ( #67622, #83105, #98640, #60093, #8104, #632 ),
 .UNSPECIFIED., .F., .F.,
 ( 4, 2, 4 ),
 ( 0.0002800671705680388059, 0.0006862730573397204763, 0.001092478944111402147 ),
 .UNSPECIFIED. ) ;
#88641=VECTOR ( 'NONE', #40208, 1000.000000000000000 ) ;
#88643=EDGE_CURVE ( 'NONE', #62748, #98433, #96718, .T. ) ;
#88659=DIRECTION ( 'NONE',  ( -0.000000000000000000, -1.000000000000000000, -0.000000000000000000 ) ) ;
#88660=CARTESIAN_POINT ( 'NONE',  ( 7.771322705631503069, 4.156677014937179135E-16, -12.24159072199917375 ) ) ;
#88662=LINE ( 'NONE', #33680, #53084 ) ;
#88666=CARTESIAN_POINT ( 'NONE',  ( 0.000000000000000000, 0.5000000000000004441, 0.000000000000000000 ) ) ;
#88681=CARTESIAN_POINT ( 'NONE',  ( -2.815433093576927170, 0.5000000000000004441, -14.73340885523753663 ) ) ;
#88682=CARTESIAN_POINT ( 'NONE',  ( 0.7575892234031803563, 14.76930270348881535, -14.92193396517713566 ) ) ;
#88686=VERTEX_POINT ( 'NONE', #15710 ) ;
#88695=CARTESIAN_POINT ( 'NONE',  ( -9.382169495545413795, 4.748634669930419605, 9.382169495545428006 ) ) ;
#88698=ORIENTED_EDGE ( 'NONE', *, *, #48034, .F. ) ;
#88705=DIRECTION ( 'NONE',  ( -0.4924235601034586685, 0.000000000000000000, -0.8703556959399044723 ) ) ;
#88708=EDGE_CURVE ( 'NONE', #65339, #61713, #60688, .T. ) ;
#88715=CARTESIAN_POINT ( 'NONE',  ( 1.881370533971287617, 15.00000000000000888, -14.50512983964826574 ) ) ;
#88719=ORIENTED_EDGE ( 'NONE', *, *, #27686, .F. ) ;
#88729=CARTESIAN_POINT ( 'NONE',  ( 13.48255862861923937, 4.031870098369226268E-16, 5.335786055104250636 ) ) ;
#88736=VECTOR ( 'NONE', #12321, 1000.000000000000000 ) ;
#88737=CIRCLE ( 'NONE', #55188, 14.49999999999999822 ) ;
#88741=ORIENTED_EDGE ( 'NONE', *, *, #21596, .F. ) ;
#88742=CARTESIAN_POINT ( 'NONE',  ( -8.235571585149862983, 5.743033628982648686, 8.235571585149875418 ) ) ;
#88753=CARTESIAN_POINT ( 'NONE',  ( 7.082119434687047743, 0.1370821682473086223, -12.26659068614894821 ) ) ;
#88761=ORIENTED_EDGE ( 'NONE', *, *, #76553, .F. ) ;
#88762=CIRCLE ( 'NONE', #55217, 14.49999999999999822 ) ;
#88772=CARTESIAN_POINT ( 'NONE',  ( -12.83294900548052730, 0.5000000000000004441, -7.766300266068542513 ) ) ;
#88778=CARTESIAN_POINT ( 'NONE',  ( -0.7375392941516041301, 14.63606910178966913, -14.98185688723475906 ) ) ;
#88779=EDGE_CURVE ( 'NONE', #94453, #52640, #69679, .T. ) ;
#88789=ADVANCED_FACE ( 'NONE', ( #1210 ), #71351, .T. ) ;
#88793=CARTESIAN_POINT ( 'NONE',  ( -0.3329122712636025105, 0.000000000000000000, 5.443067521379386875 ) ) ;
#88806=VERTEX_POINT ( 'NONE', #77171 ) ;
#88809=ORIENTED_EDGE ( 'NONE', *, *, #74957, .F. ) ;
#88813=VECTOR ( 'NONE', #9421, 1000.000000000000000 ) ;
#88817=CARTESIAN_POINT ( 'NONE',  ( -11.92686044187656869, 12.45379003517447636, -3.195792623639521768 ) ) ;
#88829=CARTESIAN_POINT ( 'NONE',  ( -7.551349515323269479, -0.03417435944610275333, 12.08468537022900868 ) ) ;
#88832=ADVANCED_FACE ( 'NONE', ( #82704 ), #12305, .T. ) ;
#88834=AXIS2_PLACEMENT_3D ( 'NONE', #28830, #89348, #80864 ) ;
#88836=AXIS2_PLACEMENT_3D ( 'NONE', #9555, #69084, #76571 ) ;
#88847=DIRECTION ( 'NONE',  ( -0.000000000000000000, 1.000000000000000000, -0.000000000000000000 ) ) ;
#88851=CARTESIAN_POINT ( 'NONE',  ( -10.64017930668216749, 14.63606904708525747, 10.57291749337210085 ) ) ;
#88853=DIRECTION ( 'NONE',  ( 0.8949343616020259962, 0.000000000000000000, 0.4461978131098069955 ) ) ;
#88858=CYLINDRICAL_SURFACE ( 'NONE', #75829, 15.00000000000000000 ) ;
#88860=EDGE_CURVE ( 'NONE', #10376, #9175, #66556, .T. ) ;
#88866=ORIENTED_EDGE ( 'NONE', *, *, #10097, .F. ) ;
#88868=ADVANCED_FACE ( 'NONE', ( #61186 ), #28212, .T. ) ;
#88874=CARTESIAN_POINT ( 'NONE',  ( 3.541595367958660479, 0.000000000000000000, 4.146675399920616734 ) ) ;
#88882=DIRECTION ( 'NONE',  ( 0.5075383629606904368, 0.000000000000000000, 0.8616291604415338146 ) ) ;
#88886=ORIENTED_EDGE ( 'NONE', *, *, #12492, .F. ) ;
#88888=AXIS2_PLACEMENT_3D ( 'NONE', #59578, #21595, #14091 ) ;
#88890=CARTESIAN_POINT ( 'NONE',  ( -12.34086200392816757, -0.03417435944610275333, -7.125000000000143885 ) ) ;
#88891=DIRECTION ( 'NONE',  ( 0.3007057995042832221, 0.000000000000000000, -0.9537169507482238240 ) ) ;
#88894=CARTESIAN_POINT ( 'NONE',  ( -8.731067818237029599, 10.31330936912750396, 8.731067818237042033 ) ) ;
#88897=ORIENTED_EDGE ( 'NONE', *, *, #74390, .T. ) ;
#88907=CARTESIAN_POINT ( 'NONE',  ( -5.817157072110893168, 0.5000000000000004441, 13.82608706751082828 ) ) ;
#88908=DIRECTION ( 'NONE',  ( 0.9170600743851238246, 0.000000000000000000, -0.3987490689252466414 ) ) ;
#88912=EDGE_CURVE ( 'NONE', #91250, #38990, #87317, .T. ) ;
#88914=TOROIDAL_SURFACE ( 'NONE', #5912, 14.49999999999999822, 0.5000000000000000000 ) ;
#88927=ORIENTED_EDGE ( 'NONE', *, *, #47675, .T. ) ;
#88930=CARTESIAN_POINT ( 'NONE',  ( -5.240416992896607340, 14.95077488074853811, -13.79072622793306913 ) ) ;
#88936=DIRECTION ( 'NONE',  ( 5.329070518200751394E-14, 0.000000000000000000, 1.000000000000000000 ) ) ;
#88938=CARTESIAN_POINT ( 'NONE',  ( 0.000000000000000000, 14.49999999999999822, 0.000000000000000000 ) ) ;
#88942=CARTESIAN_POINT ( 'NONE',  ( 0.000000000000000000, 15.00000000000000000, 0.000000000000000000 ) ) ;
#88949=CARTESIAN_POINT ( 'NONE',  ( -3.434112377981067610, -16.91803199673624647, -12.81628187352647252 ) ) ;
#88957=EDGE_CURVE ( 'NONE', #60892, #42806, #41653, .T. ) ;
#88966=ORIENTED_EDGE ( 'NONE', *, *, #69829, .T. ) ;
#88968=AXIS2_PLACEMENT_3D ( 'NONE', #7324, #45308, #37827 ) ;
#88979=VERTEX_POINT ( 'NONE', #56638 ) ;
#88984=ORIENTED_EDGE ( 'NONE', *, *, #45293, .F. ) ;
#88987=FACE_OUTER_BOUND ( 'NONE', #59930, .T. ) ;
#89004=CARTESIAN_POINT ( 'NONE',  ( -7.082119434687058401, -24.02958449841936073, -12.26659068614894110 ) ) ;
#89018=CARTESIAN_POINT ( 'NONE',  ( 7.964842623401181321, 9.938685344154839285, 7.964842623401174215 ) ) ;
#89026=TOROIDAL_SURFACE ( 'NONE', #96978, 14.49999999999999822, 0.5000000000000000000 ) ;
#89032=CARTESIAN_POINT ( 'NONE',  ( 8.731067818237038480, 10.78712336850781739, -8.731067818237040257 ) ) ;
#89050=VERTEX_POINT ( 'NONE', #2684 ) ;
#89059=CARTESIAN_POINT ( 'NONE',  ( -14.49154782522702867, 0.04962890019108593537, 2.766288502466858201 ) ) ;
#89062=CARTESIAN_POINT ( 'NONE',  ( -2.638427012816824124, -2.949402182332543365, 9.846743663894596210 ) ) ;
#89064=ORIENTED_EDGE ( 'NONE', *, *, #87973, .T. ) ;
#89075=EDGE_CURVE ( 'NONE', #86688, #74051, #88374, .T. ) ;
#89079=ORIENTED_EDGE ( 'NONE', *, *, #61081, .T. ) ;
#89085=LINE ( 'NONE', #64591, #2675 ) ;
#89092=ORIENTED_EDGE ( 'NONE', *, *, #77420, .T. ) ;
#89095=EDGE_CURVE ( 'NONE', #37098, #40499, #47664, .T. ) ;
#89097=VECTOR ( 'NONE', #64116, 999.9999999999998863 ) ;
#89100=LINE ( 'NONE', #50111, #72960 ) ;
#89103=DIRECTION ( 'NONE',  ( -0.8870108331782182720, 0.000000000000000000, -0.4617486132350404615 ) ) ;
#89104=EDGE_LOOP ( 'NONE', ( #46070, #40229, #77145, #96527, #33223, #14625 ) ) ;
#89107=PLANE ( 'NONE',  #10036 ) ;
#89125=CARTESIAN_POINT ( 'NONE',  ( -13.75801628063882909, 15.00000000000000000, 4.578972376164350599 ) ) ;
#89129=CARTESIAN_POINT ( 'NONE',  ( 10.88017736071109987, -29.22798132251182679, -2.915334737309928315 ) ) ;
#89132=B_SPLINE_CURVE_WITH_KNOTS ( 'NONE', 3,
 ( #63579, #65043, #57068, #10108, #48084, #19077 ),
 .UNSPECIFIED., .F., .F.,
 ( 4, 2, 4 ),
 ( 0.0002800111042666545411, 0.0006862164423004639587, 0.001092421780334273214 ),
 .UNSPECIFIED. ) ;
#89134=CARTESIAN_POINT ( 'NONE',  ( 14.88640444357869796, 14.76930270348881180, 1.277895705730344833 ) ) ;
#89137=CARTESIAN_POINT ( 'NONE',  ( 1.780824192092392400, 14.63606913465075365, 14.89391369643518637 ) ) ;
#89142=DIRECTION ( 'NONE',  ( 0.000000000000000000, 1.000000000000000000, 0.000000000000000000 ) ) ;
#89151=EDGE_CURVE ( 'NONE', #22386, #32242, #66092, .T. ) ;
#89155=CARTESIAN_POINT ( 'NONE',  ( 13.78891971893204271, 15.00000000000000000, 5.904717858191622426 ) ) ;
#89158=ORIENTED_EDGE ( 'NONE', *, *, #52734, .T. ) ;
#89163=ORIENTED_EDGE ( 'NONE', *, *, #60292, .T. ) ;
#89164=LINE ( 'NONE', #13162, #62907 ) ;
#89176=DIRECTION ( 'NONE',  ( 0.000000000000000000, 1.000000000000000000, 0.000000000000000000 ) ) ;
#89177=CARTESIAN_POINT ( 'NONE',  ( -12.98685442714190508, 15.00000000000000000, -6.449155920601135072 ) ) ;
#89182=CARTESIAN_POINT ( 'NONE',  ( 13.07751017357379730, 4.171195230237741069E-16, 6.263284095430596388 ) ) ;
#89184=ORIENTED_EDGE ( 'NONE', *, *, #98249, .T. ) ;
#89194=CARTESIAN_POINT ( 'NONE',  ( -11.09922568453594316, 9.540301336597091009, 6.408140936763246920 ) ) ;
#89195=EDGE_CURVE ( 'NONE', #77740, #73794, #89100, .T. ) ;
#89196=ORIENTED_EDGE ( 'NONE', *, *, #60187, .T. ) ;
#89199=VERTEX_POINT ( 'NONE', #20613 ) ;
#89213=CARTESIAN_POINT ( 'NONE',  ( 1.780824192092484326, 14.49999999999999112, -14.89391369643520058 ) ) ;
#89217=B_SPLINE_CURVE_WITH_KNOTS ( 'NONE', 3,
 ( #1314, #76295, #61282, #44795, #37328, #23312 ),
 .UNSPECIFIED., .F., .F.,
 ( 4, 2, 4 ),
 ( 3.409110551479961170E-05, 0.0004400426677366258386, 0.0008459942299584519978 ),
 .UNSPECIFIED. ) ;
#89218=ADVANCED_FACE ( 'NONE', ( #35099 ), #88108, .F. ) ;
#89219=ORIENTED_EDGE ( 'NONE', *, *, #49726, .F. ) ;
#89222=CARTESIAN_POINT ( 'NONE',  ( -10.84451454130513426, 4.265732461173792237E-16, 9.625305416630759225 ) ) ;
#89228=CARTESIAN_POINT ( 'NONE',  ( -10.70613742633244669, 4.850979303660538556E-16, -9.778988772285387654 ) ) ;
#89234=DIRECTION ( 'NONE',  ( -0.000000000000000000, 1.000000000000000000, -0.000000000000000000 ) ) ;
#89236=B_SPLINE_CURVE_WITH_KNOTS ( 'NONE', 3,
 ( #26652, #19650, #57148, #35130, #52123, #82617 ),
 .UNSPECIFIED., .F., .F.,
 ( 4, 2, 4 ),
 ( 3.409110551496096132E-05, 0.0004400426677367866800, 0.0008459942299586124597 ),
 .UNSPECIFIED. ) ;
#89238=CARTESIAN_POINT ( 'NONE',  ( -9.742785792574940373, 4.701366962315984388, -5.624999999999991118 ) ) ;
#89242=LINE ( 'NONE', #13241, #77572 ) ;
#89245=FACE_OUTER_BOUND ( 'NONE', #58202, .T. ) ;
#89248=CARTESIAN_POINT ( 'NONE',  ( 3.795296366450306547, 0.3454155015806399942, -14.16423886937410259 ) ) ;
#89251=CARTESIAN_POINT ( 'NONE',  ( 12.79448242979001371, 0.2306972965111889762, 7.716169648622186905 ) ) ;
#89254=CIRCLE ( 'NONE', #76491, 15.00000000000000000 ) ;
#89261=DIRECTION ( 'NONE',  ( -0.000000000000000000, -1.000000000000000000, -0.000000000000000000 ) ) ;
#89266=VERTEX_POINT ( 'NONE', #66600 ) ;
#89268=CARTESIAN_POINT ( 'NONE',  ( -12.79448242978996220, 0.2306972965111912799, -7.716169648622273947 ) ) ;
#89269=DIRECTION ( 'NONE',  ( -0.000000000000000000, -1.000000000000000000, -0.000000000000000000 ) ) ;
#89274=CARTESIAN_POINT ( 'NONE',  ( -0.7577696756369834974, 14.76984978199062581, -14.92139465029885237 ) ) ;
#89280=CARTESIAN_POINT ( 'NONE',  ( 5.817157072110704874, 15.00000000000000000, 13.82608706751090821 ) ) ;
#89298=FACE_OUTER_BOUND ( 'NONE', #59903, .T. ) ;
#89303=ORIENTED_EDGE ( 'NONE', *, *, #72914, .F. ) ;
#89310=DIRECTION ( 'NONE',  ( 0.000000000000000000, 1.000000000000000000, 0.000000000000000000 ) ) ;
#89311=ORIENTED_EDGE ( 'NONE', *, *, #72450, .F. ) ;
#89314=CARTESIAN_POINT ( 'NONE',  ( 11.81378540890936080, -0.03417435944610275333, -7.968498874458115999 ) ) ;
#89317=EDGE_LOOP ( 'NONE', ( #31769, #11117, #76672, #47022 ) ) ;
#89320=EDGE_LOOP ( 'NONE', ( #605, #89742, #3698, #84242 ) ) ;
#89324=CARTESIAN_POINT ( 'NONE',  ( 2.361121941889117171, 14.76984946027100420, -14.75287579053849463 ) ) ;
#89326=CARTESIAN_POINT ( 'NONE',  ( -13.75503023589401863, 14.95077488074853811, -5.333408231410926348 ) ) ;
#89329=B_SPLINE_CURVE_WITH_KNOTS ( 'NONE', 3,
 ( #97451, #6421, #12939, #74417, #28916, #43433 ),
 .UNSPECIFIED., .F., .F.,
 ( 4, 2, 4 ),
 ( 0.0002800065468392932098, 0.0006862118402932773902, 0.001092417133747261571 ),
 .UNSPECIFIED. ) ;
#89336=EDGE_LOOP ( 'NONE', ( #34363, #73822, #77036, #43187 ) ) ;
#89337=TOROIDAL_SURFACE ( 'NONE', #51083, 14.49999999999999822, 0.5000000000000000000 ) ;
#89344=CARTESIAN_POINT ( 'NONE',  ( -10.39692778084947022, 14.95037106203290733, 10.46714871971192018 ) ) ;
#89345=EDGE_CURVE ( 'NONE', #15452, #14809, #34701, .T. ) ;
#89348=DIRECTION ( 'NONE',  ( 0.9025852843498648470, 0.000000000000000000, -0.4305110968082862533 ) ) ;
#89354=CARTESIAN_POINT ( 'NONE',  ( -4.838527690343713772, 0.5000000000000004441, 14.19819177887723605 ) ) ;
#89357=CARTESIAN_POINT ( 'NONE',  ( 0.000000000000000000, 15.00000000000000000, 0.000000000000000000 ) ) ;
#89364=CARTESIAN_POINT ( 'NONE',  ( 0.000000000000000000, 15.00000000000000000, 0.000000000000000000 ) ) ;
#89371=DIRECTION ( 'NONE',  ( -0.000000000000000000, -1.000000000000000000, -0.000000000000000000 ) ) ;
#89386=EDGE_LOOP ( 'NONE', ( #77862, #45869, #48943, #49782 ) ) ;
#89387=DIRECTION ( 'NONE',  ( 0.000000000000000000, 1.000000000000000000, -0.000000000000000000 ) ) ;
#89400=EDGE_CURVE ( 'NONE', #92653, #72857, #90572, .T. ) ;
#89413=CIRCLE ( 'NONE', #8064, 15.00000000000000000 ) ;
#89417=CIRCLE ( 'NONE', #94193, 15.00000000000000000 ) ;
#89422=PLANE ( 'NONE',  #52068 ) ;
#89430=DIRECTION ( 'NONE',  ( -0.000000000000000000, -1.000000000000000000, -0.000000000000000000 ) ) ;
#89433=DIRECTION ( 'NONE',  ( -0.9935718556765871234, 0.000000000000000000, -0.1132032137679106348 ) ) ;
#89434=B_SPLINE_CURVE_WITH_KNOTS ( 'NONE', 3,
 ( #56905, #95405, #94906, #19406, #87408, #64397 ),
 .UNSPECIFIED., .F., .F.,
 ( 4, 2, 4 ),
 ( 3.409110551494641268E-05, 0.0004400426677367945405, 0.0008459942299586426006 ),
 .UNSPECIFIED. ) ;
#89441=CARTESIAN_POINT ( 'NONE',  ( -12.81628187352647963, -21.08469866340291432, -3.434112377981046293 ) ) ;
#89452=VERTEX_POINT ( 'NONE', #31053 ) ;
#89457=VERTEX_POINT ( 'NONE', #36607 ) ;
#89463=DIRECTION ( 'NONE',  ( 0.8141155183563186792, 0.000000000000000000, -0.5807029557109404383 ) ) ;
#89475=AXIS2_PLACEMENT_3D ( 'NONE', #28399, #74882, #97409 ) ;
#89479=ADVANCED_FACE ( 'NONE', ( #45076 ), #22099, .T. ) ;
#89496=CARTESIAN_POINT ( 'NONE',  ( 7.082119434687054849, -26.52958449841936428, 12.26659068614894288 ) ) ;
#89500=ORIENTED_EDGE ( 'NONE', *, *, #73027, .T. ) ;
#89506=DIRECTION ( 'NONE',  ( -0.9304175679820231304, 0.000000000000000000, -0.3665012267243009103 ) ) ;
#89508=CARTESIAN_POINT ( 'NONE',  ( -0.8649609010934330433, 15.00000000000000888, 14.60103384664008885 ) ) ;
#89509=AXIS2_PLACEMENT_3D ( 'NONE', #74622, #97162, #37627 ) ;
#89512=CARTESIAN_POINT ( 'NONE',  ( -2.915334737309917656, 34.10535201082151957, 10.88017736071110164 ) ) ;
#89516=ORIENTED_EDGE ( 'NONE', *, *, #6116, .F. ) ;
#89517=B_SPLINE_CURVE_WITH_KNOTS ( 'NONE', 3,
 ( #48755, #93772, #94756, #77287, #79263, #26257 ),
 .UNSPECIFIED., .F., .F.,
 ( 4, 2, 4 ),
 ( 0.0002800056097769411802, 0.0006862108940652274832, 0.001092416178353513949 ),
 .UNSPECIFIED. ) ;
#89518=VECTOR ( 'NONE', #26534, 1000.000000000000000 ) ;
#89527=CARTESIAN_POINT ( 'NONE',  ( 14.11874224319628013, 14.76984899115444527, 4.887061453530134436 ) ) ;
#89544=AXIS2_PLACEMENT_3D ( 'NONE', #88028, #73512, #13523 ) ;
#89545=VERTEX_POINT ( 'NONE', #75580 ) ;
#89546=VERTEX_POINT ( 'NONE', #14101 ) ;
#89556=AXIS2_PLACEMENT_3D ( 'NONE', #70848, #2361, #60863 ) ;
#89559=CARTESIAN_POINT ( 'NONE',  ( 0.000000000000000000, 15.00000000000000000, 0.000000000000000000 ) ) ;
#89560=CARTESIAN_POINT ( 'NONE',  ( 9.846743663894594434, 13.50893115100078923, -2.168404344971008868E-15 ) ) ;
#89562=ORIENTED_EDGE ( 'NONE', *, *, #61852, .T. ) ;
#89570=ORIENTED_EDGE ( 'NONE', *, *, #64952, .F. ) ;
#89575=VERTEX_POINT ( 'NONE', #23091 ) ;
#89585=EDGE_LOOP ( 'NONE', ( #82809, #35924, #45695, #51724 ) ) ;
#89588=VERTEX_POINT ( 'NONE', #54054 ) ;
#89596=FACE_OUTER_BOUND ( 'NONE', #48621, .T. ) ;
#89599=DIRECTION ( 'NONE',  ( -0.000000000000000000, -1.000000000000000000, -0.000000000000000000 ) ) ;
#89600=ORIENTED_EDGE ( 'NONE', *, *, #26972, .T. ) ;
#89603=DIRECTION ( 'NONE',  ( -0.000000000000000000, 1.000000000000000000, -0.000000000000000000 ) ) ;
#89610=ORIENTED_EDGE ( 'NONE', *, *, #16528, .F. ) ;
#89620=CARTESIAN_POINT ( 'NONE',  ( 14.24131928502211331, 15.00000000000000000, 0.4973178280106892446 ) ) ;
#89623=CARTESIAN_POINT ( 'NONE',  ( -5.204170427930421283E-15, -8.186314655845155386, -10.88017736071110342 ) ) ;
#89627=CARTESIAN_POINT ( 'NONE',  ( 12.74414838903278557, 6.606856988583540673E-16, -7.178093659841974450 ) ) ;
#89635=ADVANCED_FACE ( 'NONE', ( #21607 ), #52093, .T. ) ;
#89636=EDGE_CURVE ( 'NONE', #59040, #7312, #79331, .T. ) ;
#89641=CARTESIAN_POINT ( 'NONE',  ( -9.876730923139145801, 15.00000000000000000, -11.28938378619076843 ) ) ;
#89649=CARTESIAN_POINT ( 'NONE',  ( 0.000000000000000000, 0.5000000000000004441, 0.000000000000000000 ) ) ;
#89656=ORIENTED_EDGE ( 'NONE', *, *, #66158, .F. ) ;
#89671=EDGE_CURVE ( 'NONE', #44083, #77740, #1579, .T. ) ;
#89673=CARTESIAN_POINT ( 'NONE',  ( 2.638427012816835227, -17.53273551566588040, 9.846743663894590881 ) ) ;
#89674=VERTEX_POINT ( 'NONE', #17063 ) ;
#89675=FACE_OUTER_BOUND ( 'NONE', #1043, .T. ) ;
#89676=VERTEX_POINT ( 'NONE', #25062 ) ;
#89677=ORIENTED_EDGE ( 'NONE', *, *, #58336, .T. ) ;
#89681=DIRECTION ( 'NONE',  ( -0.4617486132350466788, -0.000000000000000000, 0.8870108331782150524 ) ) ;
#89683=AXIS2_PLACEMENT_3D ( 'NONE', #71367, #35310, #80818 ) ;
#89684=CARTESIAN_POINT ( 'NONE',  ( 12.81628187352647252, 11.83196800326375708, -3.434112377981059172 ) ) ;
#89685=ORIENTED_EDGE ( 'NONE', *, *, #67641, .T. ) ;
#89689=ORIENTED_EDGE ( 'NONE', *, *, #29282, .T. ) ;
#89696=DIRECTION ( 'NONE',  ( 0.000000000000000000, 0.000000000000000000, 1.000000000000000000 ) ) ;
#89698=ORIENTED_EDGE ( 'NONE', *, *, #78535, .T. ) ;
#89699=CARTESIAN_POINT ( 'NONE',  ( -0.2074183518478776300, 0.04876363957840557789, -14.75075219811622596 ) ) ;
#89700=FACE_OUTER_BOUND ( 'NONE', #39746, .T. ) ;
#89701=CARTESIAN_POINT ( 'NONE',  ( -3.836325488036278930, 0.5000000000000004441, 14.50112432709419785 ) ) ;
#89708=CARTESIAN_POINT ( 'NONE',  ( -11.35178980618980304, 0.5000000000000004441, 9.804941009311846756 ) ) ;
#89712=LINE ( 'NONE', #73718, #34078 ) ;
#89724=CARTESIAN_POINT ( 'NONE',  ( -11.35178980618980304, 15.00000000000000000, 9.804941009311846756 ) ) ;
#89728=DIRECTION ( 'NONE',  ( 0.000000000000000000, 0.000000000000000000, 1.000000000000000000 ) ) ;
#89733=CARTESIAN_POINT ( 'NONE',  ( -12.26659068614894110, 2.220415501580634388, 7.082119434687058401 ) ) ;
#89735=EDGE_CURVE ( 'NONE', #76019, #61376, #31499, .T. ) ;
#89741=EDGE_CURVE ( 'NONE', #27523, #84834, #10743, .T. ) ;
#89742=ORIENTED_EDGE ( 'NONE', *, *, #60295, .F. ) ;
#89752=ORIENTED_EDGE ( 'NONE', *, *, #16662, .F. ) ;
#89754=VECTOR ( 'NONE', #80324, 999.9999999999998863 ) ;
#89771=EDGE_LOOP ( 'NONE', ( #31948, #37354, #35840, #34609 ) ) ;
#89778=CYLINDRICAL_SURFACE ( 'NONE', #56814, 15.00000000000000000 ) ;
#89785=ADVANCED_FACE ( 'NONE', ( #93039 ), #62532, .F. ) ;
#89787=DIRECTION ( 'NONE',  ( -0.000000000000000000, -1.000000000000000000, -0.000000000000000000 ) ) ;
#89788=VERTEX_POINT ( 'NONE', #55547 ) ;
#89791=EDGE_LOOP ( 'NONE', ( #32797, #12208, #25244, #88278, #18306, #81857 ) ) ;
#89794=DIRECTION ( 'NONE',  ( -0.04361938736533987893, 0.000000000000000000, 0.9990482215818576872 ) ) ;
#89795=VERTEX_POINT ( 'NONE', #8567 ) ;
#89798=EDGE_LOOP ( 'NONE', ( #60431, #96707, #19413, #32125, #36968, #94104 ) ) ;
#89801=ORIENTED_EDGE ( 'NONE', *, *, #85196, .T. ) ;
#89803=ORIENTED_EDGE ( 'NONE', *, *, #60838, .F. ) ;
#89805=B_SPLINE_CURVE_WITH_KNOTS ( 'NONE', 3,
 ( #80904, #20407, #73388, #33412, #94421, #25937 ),
 .UNSPECIFIED., .F., .F.,
 ( 4, 2, 4 ),
 ( 3.409110551496046665E-05, 0.0004400426677367835358, 0.0008459942299586066050 ),
 .UNSPECIFIED. ) ;
#89812=AXIS2_PLACEMENT_3D ( 'NONE', #60868, #411, #84382 ) ;
#89813=ORIENTED_EDGE ( 'NONE', *, *, #97896, .F. ) ;
#89816=CARTESIAN_POINT ( 'NONE',  ( 14.66148682522639568, 14.76984938411481352, 2.874551585518038355 ) ) ;
#89819=CIRCLE ( 'NONE', #41885, 15.00000000000000000 ) ;
#89820=TOROIDAL_SURFACE ( 'NONE', #54701, 14.49999999999999822, 0.5000000000000000000 ) ;
#89833=DIRECTION ( 'NONE',  ( 0.7253743710122867450, 0.000000000000000000, -0.6883545756937550220 ) ) ;
#89835=EDGE_LOOP ( 'NONE', ( #41700, #24640, #76638, #22748, #53432, #32880 ) ) ;
#89838=DIRECTION ( 'NONE',  ( 0.000000000000000000, 0.000000000000000000, -1.000000000000000000 ) ) ;
#89851=CARTESIAN_POINT ( 'NONE',  ( -3.115783986955356522, 15.00000000000000000, -14.16128137375399554 ) ) ;
#89852=CARTESIAN_POINT ( 'NONE',  ( 7.684764310694797373, 14.63606916355816878, 12.88194075009944584 ) ) ;
#89855=ORIENTED_EDGE ( 'NONE', *, *, #69035, .T. ) ;
#89857=DIRECTION ( 'NONE',  ( 0.000000000000000000, 1.000000000000000000, 0.000000000000000000 ) ) ;
#89864=CARTESIAN_POINT ( 'NONE',  ( -8.606322355891206755, 3.940577227621431661E-16, -11.66967075398818743 ) ) ;
#89865=ORIENTED_EDGE ( 'NONE', *, *, #97611, .F. ) ;
#89869=CARTESIAN_POINT ( 'NONE',  ( -5.624999999999997335, 8.755135511184874986, 9.742785792574938597 ) ) ;
#89877=DIRECTION ( 'NONE',  ( 0.5664062369248205053, 0.000000000000000000, 0.8241261886220241362 ) ) ;
#89878=CARTESIAN_POINT ( 'NONE',  ( -3.836325488035988052, 15.00000000000000000, -14.50112432709427424 ) ) ;
#89882=DIRECTION ( 'NONE',  ( 0.3338068592337776197, 0.000000000000000000, -0.9426414910921760981 ) ) ;
#89886=DIRECTION ( 'NONE',  ( -0.4461978131098131573, 0.000000000000000000, 0.8949343616020228875 ) ) ;
#89891=CARTESIAN_POINT ( 'NONE',  ( 0.000000000000000000, 0.5000000000000004441, 0.000000000000000000 ) ) ;
#89899=CARTESIAN_POINT ( 'NONE',  ( -2.913501739333859586, 15.00000000000000000, 14.20427779279530434 ) ) ;
#89901=CARTESIAN_POINT ( 'NONE',  ( -10.93781366033354097, 0.5000000000000004441, 10.26470809774057713 ) ) ;
#89913=VERTEX_POINT ( 'NONE', #43477 ) ;
#89923=CARTESIAN_POINT ( 'NONE',  ( 14.97653319723437626, -0.03417435944610275333, 5.619684139539351975 ) ) ;
#89928=CARTESIAN_POINT ( 'NONE',  ( 9.382169495545415572, -22.75136533006957862, -9.382169495545422677 ) ) ;
#89937=TOROIDAL_SURFACE ( 'NONE', #77158, 14.49999999999999822, 0.5000000000000000000 ) ;
#89944=EDGE_LOOP ( 'NONE', ( #40408, #69171, #44746, #60053, #9208, #19683 ) ) ;
#89949=CARTESIAN_POINT ( 'NONE',  ( 14.43063482171891465, 15.00000000000000888, 2.386446184883126875 ) ) ;
#89951=EDGE_CURVE ( 'NONE', #18862, #77019, #4028, .T. ) ;
#89956=ORIENTED_EDGE ( 'NONE', *, *, #90769, .F. ) ;
#89960=TOROIDAL_SURFACE ( 'NONE', #88392, 14.49999999999999822, 0.5000000000000000000 ) ;
#89964=DIRECTION ( 'NONE',  ( 0.000000000000000000, 1.000000000000000000, 0.000000000000000000 ) ) ;
#89982=CARTESIAN_POINT ( 'NONE',  ( 14.16423886937410082, -15.48791783175269643, -3.795296366450314096 ) ) ;
#89986=EDGE_CURVE ( 'NONE', #29326, #39731, #57499, .T. ) ;
#89993=CARTESIAN_POINT ( 'NONE',  ( 9.898881779040729967, -0.03417435944610275333, -10.25059215482576214 ) ) ;
#89997=CARTESIAN_POINT ( 'NONE',  ( 5.440088680355549045, 31.39701867748817676, -9.422509992056141925 ) ) ;
#90005=DIRECTION ( 'NONE',  ( 0.000000000000000000, 1.000000000000000000, 0.000000000000000000 ) ) ;
#90011=FACE_OUTER_BOUND ( 'NONE', #31728, .T. ) ;
#90014=ORIENTED_EDGE ( 'NONE', *, *, #11098, .F. ) ;
#90017=DIRECTION ( 'NONE',  ( 0.000000000000000000, 0.000000000000000000, 1.000000000000000000 ) ) ;
#90019=DIRECTION ( 'NONE',  ( 0.000000000000000000, 1.000000000000000000, 0.000000000000000000 ) ) ;
#90026=LINE ( 'NONE', #13543, #63377 ) ;
#90028=CARTESIAN_POINT ( 'NONE',  ( 5.171435456984222689, 0.000000000000000000, 1.730338099014012476 ) ) ;
#90042=DIRECTION ( 'NONE',  ( 0.000000000000000000, 1.000000000000000000, 0.000000000000000000 ) ) ;
#90045=CARTESIAN_POINT ( 'NONE',  ( 0.000000000000000000, 0.000000000000000000, 0.000000000000000000 ) ) ;
#90046=CARTESIAN_POINT ( 'NONE',  ( 9.846743663894590881, 13.71726448433412493, -2.638427012816833894 ) ) ;
#90048=ORIENTED_EDGE ( 'NONE', *, *, #82290, .F. ) ;
#90059=EDGE_LOOP ( 'NONE', ( #61594, #64216, #51597, #40756 ) ) ;
#90062=ORIENTED_EDGE ( 'NONE', *, *, #17199, .F. ) ;
#90064=ORIENTED_EDGE ( 'NONE', *, *, #67149, .F. ) ;
#90070=DIRECTION ( 'NONE',  ( 0.4924235601034648302, 0.000000000000000000, 0.8703556959399010307 ) ) ;
#90075=EDGE_CURVE ( 'NONE', #40424, #42957, #42291, .T. ) ;
#90076=DIRECTION ( 'NONE',  ( -0.000000000000000000, -1.000000000000000000, -0.000000000000000000 ) ) ;
#90077=B_SPLINE_CURVE_WITH_KNOTS ( 'NONE', 3,
 ( #97142, #28612, #85563, #1592, #92557, #55044 ),
 .UNSPECIFIED., .F., .F.,
 ( 4, 2, 4 ),
 ( 3.409110551491190117E-05, 0.0004400426677367364815, 0.0008459942299585610686 ),
 .UNSPECIFIED. ) ;
#90088=CARTESIAN_POINT ( 'NONE',  ( -2.518025504887084765, 0.000000000000000000, -4.837081990145629007 ) ) ;
#90094=EDGE_CURVE ( 'NONE', #8246, #2122, #46944, .T. ) ;
#90096=EDGE_LOOP ( 'NONE', ( #45090, #92025, #52543, #62193 ) ) ;
#90105=B_SPLINE_CURVE_WITH_KNOTS ( 'NONE', 3,
 ( #65364, #27373, #88377, #49873, #57865, #19874 ),
 .UNSPECIFIED., .F., .F.,
 ( 4, 2, 4 ),
 ( 3.409110551494643978E-05, 0.0004400426677367928058, 0.0008459942299586392395 ),
 .UNSPECIFIED. ) ;
#90107=PLANE ( 'NONE',  #61566 ) ;
#90110=CARTESIAN_POINT ( 'NONE',  ( -5.440088680355547268, -11.10298132251182146, 9.422509992056143702 ) ) ;
#90114=CARTESIAN_POINT ( 'NONE',  ( 13.14228782657339956, 0.5000000000000004441, -7.230509711182238064 ) ) ;
#90115=CARTESIAN_POINT ( 'NONE',  ( 13.82192141328812518, 15.00000000000000000, -4.382292601468683380 ) ) ;
#90119=DIRECTION ( 'NONE',  ( 0.000000000000000000, 1.000000000000000000, 0.000000000000000000 ) ) ;
#90124=ORIENTED_EDGE ( 'NONE', *, *, #16876, .F. ) ;
#90131=CARTESIAN_POINT ( 'NONE',  ( 8.839000071701287098, 14.95037109469702230, -11.81225584161899178 ) ) ;
#90132=TOROIDAL_SURFACE ( 'NONE', #47030, 14.49999999999999822, 0.5000000000000000000 ) ;
#90134=ORIENTED_EDGE ( 'NONE', *, *, #59954, .T. ) ;
#90135=CARTESIAN_POINT ( 'NONE',  ( -9.898881779040801021, -0.03417435944610275333, 10.25059215482569641 ) ) ;
#90137=ORIENTED_EDGE ( 'NONE', *, *, #3476, .T. ) ;
#90138=ORIENTED_EDGE ( 'NONE', *, *, #28800, .T. ) ;
#90139=DIRECTION ( 'NONE',  ( -0.7716245833877148907, 0.000000000000000000, -0.6360782202777701677 ) ) ;
#90154=CARTESIAN_POINT ( 'NONE',  ( -7.208316651077764980, -24.61606884899921255, -7.208316651077759651 ) ) ;
#90159=VERTEX_POINT ( 'NONE', #54931 ) ;
#90160=CARTESIAN_POINT ( 'NONE',  ( -0.9082943533638192513, 4.617951328659527895E-16, 14.47152380945584582 ) ) ;
#90168=CARTESIAN_POINT ( 'NONE',  ( 9.382169495545415572, 27.24863466993041428, -9.382169495545422677 ) ) ;
#90174=ORIENTED_EDGE ( 'NONE', *, *, #5571, .F. ) ;
#90185=DIRECTION ( 'NONE',  ( 0.9799247046208295897, 0.000000000000000000, -0.1993679344171971901 ) ) ;
#90188=CARTESIAN_POINT ( 'NONE',  ( -0.3093388210927633941, 0.5000000000000004441, -14.99680997725065978 ) ) ;
#90189=LINE ( 'NONE', #43706, #70640 ) ;
#90191=EDGE_CURVE ( 'NONE', #98827, #94698, #48913, .T. ) ;
#90193=EDGE_CURVE ( 'NONE', #41646, #22776, #90665, .T. ) ;
#90196=ORIENTED_EDGE ( 'NONE', *, *, #41225, .T. ) ;
#90205=CARTESIAN_POINT ( 'NONE',  ( 0.000000000000000000, 0.5000000000000004441, 0.000000000000000000 ) ) ;
#90213=CARTESIAN_POINT ( 'NONE',  ( -3.866399090317088838, 0.04922511925147263906, -14.23717170745777949 ) ) ;
#90218=ADVANCED_FACE ( 'NONE', ( #62934 ), #94415, .F. ) ;
#90220=CARTESIAN_POINT ( 'NONE',  ( -5.204170427930421283E-15, 6.412123368507812948, -11.92686044187656513 ) ) ;
#90226=CARTESIAN_POINT ( 'NONE',  ( 14.16423886937410437, 24.09541550158063572, 3.795296366450304770 ) ) ;
#90227=CONICAL_SURFACE ( 'NONE', #57058, 13.74999999999999467, 0.7853981633974458365 ) ;
#90230=LINE ( 'NONE', #84235, #38921 ) ;
#90238=PLANE ( 'NONE',  #53154 ) ;
#90240=DIRECTION ( 'NONE',  ( 0.000000000000000000, 0.000000000000000000, 1.000000000000000000 ) ) ;
#90241=AXIS2_PLACEMENT_3D ( 'NONE', #64730, #87741, #19253 ) ;
#90242=CARTESIAN_POINT ( 'NONE',  ( -0.9940297508538862292, -0.03417435944610275333, 14.21528771620248932 ) ) ;
#90254=CARTESIAN_POINT ( 'NONE',  ( 4.850097797904266983, 0.04962897333335813954, -13.93319274793802798 ) ) ;
#90272=ORIENTED_EDGE ( 'NONE', *, *, #93009, .T. ) ;
#90275=ORIENTED_EDGE ( 'NONE', *, *, #51717, .F. ) ;
#90280=LINE ( 'NONE', #65803, #71198 ) ;
#90283=EDGE_LOOP ( 'NONE', ( #95499, #16541, #47624, #53787, #10628, #88984 ) ) ;
#90286=VERTEX_POINT ( 'NONE', #56432 ) ;
#90292=PLANE ( 'NONE',  #6332 ) ;
#90296=EDGE_CURVE ( 'NONE', #3803, #34327, #24466, .T. ) ;
#90306=CARTESIAN_POINT ( 'NONE',  ( -14.02068044289382875, 0.5000000000000004441, 5.331089937175565119 ) ) ;
#90310=CARTESIAN_POINT ( 'NONE',  ( 0.000000000000000000, 14.49999999999999822, 0.000000000000000000 ) ) ;
#90320=CIRCLE ( 'NONE', #931, 15.00000000000000000 ) ;
#90327=CARTESIAN_POINT ( 'NONE',  ( -5.418184704451246780, 0.000000000000000000, 0.6173241701922714819 ) ) ;
#90328=EDGE_CURVE ( 'NONE', #70993, #72571, #37023, .T. ) ;
#90337=VECTOR ( 'NONE', #15238, 1000.000000000000000 ) ;
#90340=FACE_OUTER_BOUND ( 'NONE', #11285, .T. ) ;
#90342=CARTESIAN_POINT ( 'NONE',  ( 6.715867195167449566, 4.285122813354096929E-16, -12.85095824508326956 ) ) ;
#90348=CARTESIAN_POINT ( 'NONE',  ( -2.393480905992962704, 0.3639310596586416979, -14.80781041047758073 ) ) ;
#90361=CARTESIAN_POINT ( 'NONE',  ( 10.04796213703179220, 15.00000000000000888, -10.62905469192465091 ) ) ;
#90362=LINE ( 'NONE', #67887, #54359 ) ;
#90367=LINE ( 'NONE', #73896, #97029 ) ;
#90368=CARTESIAN_POINT ( 'NONE',  ( 3.469446951953614189E-15, 3.912123368507817833, 11.92686044187656513 ) ) ;
#90371=AXIS2_PLACEMENT_3D ( 'NONE', #27433, #56949, #87935 ) ;
#90377=CARTESIAN_POINT ( 'NONE',  ( -8.209432707285007069, 14.49999999999999112, 12.55409154915484393 ) ) ;
#90385=EDGE_CURVE ( 'NONE', #63123, #7097, #74173, .T. ) ;
#90392=CARTESIAN_POINT ( 'NONE',  ( -12.25993886608596029, 14.63606888159244690, -8.642563219313824874 ) ) ;
#90393=ORIENTED_EDGE ( 'NONE', *, *, #59994, .T. ) ;
#90401=DIRECTION ( 'NONE',  ( -0.000000000000000000, 1.000000000000000000, 0.000000000000000000 ) ) ;
#90406=CARTESIAN_POINT ( 'NONE',  ( 3.434112377981054287, -22.33469866340291077, -12.81628187352647608 ) ) ;
#90417=CARTESIAN_POINT ( 'NONE',  ( 0.000000000000000000, 14.49999999999999822, 0.000000000000000000 ) ) ;
#90418=ORIENTED_EDGE ( 'NONE', *, *, #83556, .F. ) ;
#90421=EDGE_CURVE ( 'NONE', #13765, #18862, #40563, .T. ) ;
#90424=ORIENTED_EDGE ( 'NONE', *, *, #56594, .T. ) ;
#90433=CARTESIAN_POINT ( 'NONE',  ( 0.000000000000000000, 15.00000000000000000, 0.000000000000000000 ) ) ;
#90438=FACE_OUTER_BOUND ( 'NONE', #62665, .T. ) ;
#90441=EDGE_CURVE ( 'NONE', #61835, #57201, #89434, .T. ) ;
#90443=VECTOR ( 'NONE', #81093, 1000.000000000000000 ) ;
#90448=EDGE_CURVE ( 'NONE', #19669, #62224, #42409, .T. ) ;
#90454=CARTESIAN_POINT ( 'NONE',  ( 0.000000000000000000, 14.49999999999999822, 0.000000000000000000 ) ) ;
#90464=VECTOR ( 'NONE', #90711, 1000.000000000000000 ) ;
#90466=CARTESIAN_POINT ( 'NONE',  ( -12.26659068614895354, -13.61291783175269643, -7.082119434687038861 ) ) ;
#90471=DIRECTION ( 'NONE',  ( 0.8433914458128921599, 0.000000000000000000, -0.5372996083468138950 ) ) ;
#90472=B_SPLINE_CURVE_WITH_KNOTS ( 'NONE', 3,
 ( #17883, #62880, #39894, #32869, #63369, #48856 ),
 .UNSPECIFIED., .F., .F.,
 ( 4, 2, 4 ),
 ( 3.409110551496086645E-05, 0.0004400426677367858127, 0.0008459942299586108334 ),
 .UNSPECIFIED. ) ;
#90474=CARTESIAN_POINT ( 'NONE',  ( 10.70613742633613796, 15.00000000000000000, 9.778988772292906972 ) ) ;
#90478=CARTESIAN_POINT ( 'NONE',  ( 1.114591949024916984, 15.00000000000000000, 14.45709807627962817 ) ) ;
#90479=B_SPLINE_CURVE_WITH_KNOTS ( 'NONE', 3,
 ( #73155, #96682, #97183, #50167, #88164, #88660 ),
 .UNSPECIFIED., .F., .F.,
 ( 4, 2, 4 ),
 ( 3.409110551496134756E-05, 0.0004400426677367868427, 0.0008459942299586123513 ),
 .UNSPECIFIED. ) ;
#90480=CARTESIAN_POINT ( 'NONE',  ( -5.204170427930421283E-15, 21.81368534415484106, -10.88017736071110342 ) ) ;
#90484=VECTOR ( 'NONE', #88403, 1000.000000000000114 ) ;
#90487=ORIENTED_EDGE ( 'NONE', *, *, #83129, .F. ) ;
#90490=FACE_OUTER_BOUND ( 'NONE', #40609, .T. ) ;
#90495=AXIS2_PLACEMENT_3D ( 'NONE', #69184, #69669, #46662 ) ;
#90501=EDGE_LOOP ( 'NONE', ( #37654, #39663, #71258, #90048 ) ) ;
#90502=PLANE ( 'NONE',  #71790 ) ;
#90507=DIRECTION ( 'NONE',  ( 0.000000000000000000, 0.000000000000000000, 1.000000000000000000 ) ) ;
#90511=CARTESIAN_POINT ( 'NONE',  ( 13.61464873478167981, 0.3640475087720990155, -6.296136897217838424 ) ) ;
#90514=EDGE_CURVE ( 'NONE', #74236, #78251, #64598, .T. ) ;
#90517=ORIENTED_EDGE ( 'NONE', *, *, #41583, .F. ) ;
#90532=DIRECTION ( 'NONE',  ( 0.000000000000000000, 0.000000000000000000, 1.000000000000000000 ) ) ;
#90533=CARTESIAN_POINT ( 'NONE',  ( 4.923371831947295441, 19.34226448433412671, -8.527530157486179263 ) ) ;
#90534=ORIENTED_EDGE ( 'NONE', *, *, #44400, .T. ) ;
#90536=LINE ( 'NONE', #83546, #95682 ) ;
#90538=TOROIDAL_SURFACE ( 'NONE', #33082, 14.49999999999999822, 0.5000000000000000000 ) ;
#90552=EDGE_CURVE ( 'NONE', #43285, #24087, #18225, .T. ) ;
#90560=TOROIDAL_SURFACE ( 'NONE', #61792, 14.49999999999999822, 0.5000000000000000000 ) ;
#90566=ORIENTED_EDGE ( 'NONE', *, *, #9899, .T. ) ;
#90567=CARTESIAN_POINT ( 'NONE',  ( 0.000000000000000000, 0.000000000000000000, 0.000000000000000000 ) ) ;
#90572=LINE ( 'NONE', #98617, #25105 ) ;
#90575=CARTESIAN_POINT ( 'NONE',  ( 13.21236992757670059, 0.000000000000000000, 5.338143956176803151 ) ) ;
#90576=ORIENTED_EDGE ( 'NONE', *, *, #2304, .T. ) ;
#90577=CARTESIAN_POINT ( 'NONE',  ( 11.59580422753459494, 0.2301505044262100452, -9.421229451859201021 ) ) ;
#90579=DIRECTION ( 'NONE',  ( -0.6626200482157305061, 0.000000000000000000, -0.7489557207890082946 ) ) ;
#90586=ORIENTED_EDGE ( 'NONE', *, *, #86995, .T. ) ;
#90587=ORIENTED_EDGE ( 'NONE', *, *, #42600, .F. ) ;
#90596=DIRECTION ( 'NONE',  ( -0.000000000000000000, -1.000000000000000000, -0.000000000000000000 ) ) ;
#90597=CIRCLE ( 'NONE', #88968, 15.00000000000000000 ) ;
#90600=CARTESIAN_POINT ( 'NONE',  ( -2.915334737309917656, -15.89464798917849109, 10.88017736071110164 ) ) ;
#90604=CARTESIAN_POINT ( 'NONE',  ( 11.35178980618967337, 14.49999999999999822, 9.804941009311999522 ) ) ;
#90605=CIRCLE ( 'NONE', #47505, 15.00000000000000000 ) ;
#90606=AXIS2_PLACEMENT_3D ( 'NONE', #76677, #78156, #93645 ) ;
#90617=ORIENTED_EDGE ( 'NONE', *, *, #94605, .T. ) ;
#90625=CARTESIAN_POINT ( 'NONE',  ( 8.721827932837868502, 14.99999999999802291, -11.74045266257544462 ) ) ;
#90631=VERTEX_POINT ( 'NONE', #63213 ) ;
#90632=VERTEX_POINT ( 'NONE', #24745 ) ;
#90649=CARTESIAN_POINT ( 'NONE',  ( -7.208316651077756099, -23.36606884899921255, 7.208316651077766757 ) ) ;
#90655=ORIENTED_EDGE ( 'NONE', *, *, #64354, .F. ) ;
#90656=CARTESIAN_POINT ( 'NONE',  ( 0.000000000000000000, 14.49999999999999822, 0.000000000000000000 ) ) ;
#90662=CIRCLE ( 'NONE', #69908, 14.49999999999999822 ) ;
#90665=B_SPLINE_CURVE_WITH_KNOTS ( 'NONE', 3,
 ( #9948, #78926, #69958, #40451, #39947, #16960 ),
 .UNSPECIFIED., .F., .F.,
 ( 4, 2, 4 ),
 ( 0.0002800591277523107204, 0.0006862649357714370240, 0.001092470743790563328 ),
 .UNSPECIFIED. ) ;
#90666=CARTESIAN_POINT ( 'NONE',  ( -3.434112377981067610, 23.08196800326375708, -12.81628187352647252 ) ) ;
#90667=ORIENTED_EDGE ( 'NONE', *, *, #28910, .T. ) ;
#90673=AXIS2_PLACEMENT_3D ( 'NONE', #29647, #28676, #83161 ) ;
#90678=DIRECTION ( 'NONE',  ( 0.6626200482157357241, 0.000000000000000000, 0.7489557207890036317 ) ) ;
#90683=CARTESIAN_POINT ( 'NONE',  ( 7.313705784284598721, 0.3640475087720987935, -13.09617149020744087 ) ) ;
#90685=CARTESIAN_POINT ( 'NONE',  ( -9.876730923139378504, 15.00000000000000000, 11.28938378619056415 ) ) ;
#90687=DIRECTION ( 'NONE',  ( -0.3665012267242880872, 0.000000000000000000, -0.9304175679820281264 ) ) ;
#90689=DIRECTION ( 'NONE',  ( -0.3173046564050965856, 0.000000000000000000, 0.9483236552061978797 ) ) ;
#90691=DIRECTION ( 'NONE',  ( 0.000000000000000000, 1.000000000000000000, 0.000000000000000000 ) ) ;
#90692=VERTEX_POINT ( 'NONE', #10234 ) ;
#90694=CARTESIAN_POINT ( 'NONE',  ( 0.000000000000000000, 0.5000000000000004441, 0.000000000000000000 ) ) ;
#90699=FACE_OUTER_BOUND ( 'NONE', #32611, .T. ) ;
#90705=ADVANCED_FACE ( 'NONE', ( #87196 ), #18719, .F. ) ;
#90708=ORIENTED_EDGE ( 'NONE', *, *, #44600, .T. ) ;
#90710=ORIENTED_EDGE ( 'NONE', *, *, #56567, .F. ) ;
#90711=DIRECTION ( 'NONE',  ( -0.000000000000000000, 1.000000000000000000, 0.000000000000000000 ) ) ;
#90716=CARTESIAN_POINT ( 'NONE',  ( 0.000000000000000000, 15.00000000000000000, 0.000000000000000000 ) ) ;
#90719=CARTESIAN_POINT ( 'NONE',  ( 5.419894505350628222, 14.49999999999999112, -13.98659156302463735 ) ) ;
#90722=( BOUNDED_CURVE ( )  B_SPLINE_CURVE ( 2, ( #79003, #94494, #62026, #85039, #16552, #58961, #57480, #4500, #11004, #3513, #50469, #65962, #20477 ),
 .UNSPECIFIED., .F., .T. ) 
 B_SPLINE_CURVE_WITH_KNOTS ( ( 3, 2, 2, 2, 2, 2, 3 ),
 ( 0.6333333333333334147, 0.6388888888888889506, 0.6444444444444445974, 0.6500000000000001332, 0.6555555555555556690, 0.6611111111111112049, 0.6666666666666667407 ),
 .UNSPECIFIED. ) 
 CURVE ( )  GEOMETRIC_REPRESENTATION_ITEM ( )  RATIONAL_B_SPLINE_CURVE ( ( 0.9999999999999993339, 0.9659258262890689783, 1.000000000000000000, 0.9659258262890683122, 1.000000000000000000, 0.9659258262890683122, 1.000000000000000000, 0.9659258262890683122, 1.000000000000000000, 0.9659258262890683122, 1.000000000000000000, 0.9659258262890676461, 1.000000000000000666 ) ) 
 REPRESENTATION_ITEM ( '' )  );
#90723=CARTESIAN_POINT ( 'NONE',  ( -12.26659068614895354, 21.38708216824730712, -7.082119434687038861 ) ) ;
#90737=CARTESIAN_POINT ( 'NONE',  ( -10.58981376305275468, 15.00000000000000000, -9.535111140613857117 ) ) ;
#90741=ORIENTED_EDGE ( 'NONE', *, *, #10215, .F. ) ;
#90744=CARTESIAN_POINT ( 'NONE',  ( -12.11331110855129367, 0.04922511925147014800, -8.421032842869621504 ) ) ;
#90748=DIRECTION ( 'NONE',  ( 0.000000000000000000, 0.000000000000000000, -1.000000000000000000 ) ) ;
#90749=CARTESIAN_POINT ( 'NONE',  ( -11.96291822454887033, 4.341775326899288507E-16, 8.193813980848993594 ) ) ;
#90753=CARTESIAN_POINT ( 'NONE',  ( 4.838527690343616960, 0.3639308167276188999, -14.19819177887730710 ) ) ;
#90755=B_SPLINE_CURVE_WITH_KNOTS ( 'NONE', 3,
 ( #45701, #98741, #30191, #38699, #38217, #60692 ),
 .UNSPECIFIED., .F., .F.,
 ( 4, 2, 4 ),
 ( 3.409110551494646689E-05, 0.0004400426677367933479, 0.0008459942299586402153 ),
 .UNSPECIFIED. ) ;
#90757=AXIS2_PLACEMENT_3D ( 'NONE', #79811, #72787, #4324 ) ;
#90760=B_SPLINE_CURVE_WITH_KNOTS ( 'NONE', 3,
 ( #28940, #49979, #13460, #80486, #45428, #38438 ),
 .UNSPECIFIED., .F., .F.,
 ( 4, 2, 4 ),
 ( 3.409110551496121881E-05, 0.0004400426677367874390, 0.0008459942299586136524 ),
 .UNSPECIFIED. ) ;
#90763=FACE_OUTER_BOUND ( 'NONE', #73051, .T. ) ;
#90769=EDGE_CURVE ( 'NONE', #85778, #85655, #52162, .T. ) ;
#90776=ORIENTED_EDGE ( 'NONE', *, *, #16528, .T. ) ;
#90778=VERTEX_POINT ( 'NONE', #34680 ) ;
#90785=CARTESIAN_POINT ( 'NONE',  ( 7.264509831664601514, 0.2301509507469222116, 13.05561747642794934 ) ) ;
#90788=ORIENTED_EDGE ( 'NONE', *, *, #52270, .T. ) ;
#90793=VERTEX_POINT ( 'NONE', #59655 ) ;
#90796=DIRECTION ( 'NONE',  ( 0.000000000000000000, 0.000000000000000000, 1.000000000000000000 ) ) ;
#90826=CARTESIAN_POINT ( 'NONE',  ( 14.71525861348293596, 14.49999999999999112, 2.908807992686717192 ) ) ;
#90829=ORIENTED_EDGE ( 'NONE', *, *, #70589, .F. ) ;
#90830=DIRECTION ( 'NONE',  ( 0.000000000000000000, 0.000000000000000000, 1.000000000000000000 ) ) ;
#90836=DIRECTION ( 'NONE',  ( 0.4461978131097943945, 0.000000000000000000, 0.8949343616020322134 ) ) ;
#90841=DIRECTION ( 'NONE',  ( 0.7253743710122775301, 0.000000000000000000, 0.6883545756937645699 ) ) ;
#90845=CARTESIAN_POINT ( 'NONE',  ( 1.377727649040772586E-15, 15.00000000000000000, 11.25000000000000178 ) ) ;
#90855=ORIENTED_EDGE ( 'NONE', *, *, #85476, .T. ) ;
#90862=CARTESIAN_POINT ( 'NONE',  ( -13.61464873478171533, 0.5000000000000004441, 6.296136897217742501 ) ) ;
#90868=CARTESIAN_POINT ( 'NONE',  ( -5.806616290881503772, -3.110304982317789662E-15, 13.42355087257358548 ) ) ;
#90883=LINE ( 'NONE', #43899, #31280 ) ;
#90903=B_SPLINE_CURVE_WITH_KNOTS ( 'NONE', 3,
 ( #38865, #76362, #84371, #53355, #15386, #60361 ),
 .UNSPECIFIED., .F., .F.,
 ( 4, 2, 4 ),
 ( 3.409110551494650755E-05, 0.0004400426677367948658, 0.0008459942299586432511 ),
 .UNSPECIFIED. ) ;
#90907=EDGE_LOOP ( 'NONE', ( #42706, #54372, #91654, #45135 ) ) ;
#90910=CARTESIAN_POINT ( 'NONE',  ( -5.204170427930421283E-15, -17.12636533006957862, -12.81628187352647608 ) ) ;
#90913=DIRECTION ( 'NONE',  ( -0.9588197348681908316, 0.000000000000000000, -0.2840153447039300283 ) ) ;
#90923=ORIENTED_EDGE ( 'NONE', *, *, #89075, .T. ) ;
#90924=CIRCLE ( 'NONE', #17444, 14.49999999999999822 ) ;
#90929=CARTESIAN_POINT ( 'NONE',  ( 12.98685442714197791, 15.00000000000000000, -6.449155920600934344 ) ) ;
#90947=DIRECTION ( 'NONE',  ( 0.000000000000000000, 1.000000000000000000, 0.000000000000000000 ) ) ;
#90949=CARTESIAN_POINT ( 'NONE',  ( -3.014428414850123250, 11.15970029564931565, 11.25000000000000178 ) ) ;
#90959=CARTESIAN_POINT ( 'NONE',  ( 10.36894250292379027, -16.32125116508603213, 10.36894250292378672 ) ) ;
#90972=VECTOR ( 'NONE', #14897, 1000.000000000000000 ) ;
#90975=CARTESIAN_POINT ( 'NONE',  ( -2.915334737309934532, 22.02201867748818742, -10.88017736071109987 ) ) ;
#90982=ORIENTED_EDGE ( 'NONE', *, *, #55391, .T. ) ;
#91002=DIRECTION ( 'NONE',  ( 0.000000000000000000, 0.000000000000000000, 1.000000000000000000 ) ) ;
#91006=CARTESIAN_POINT ( 'NONE',  ( 4.873787042390699931, -0.03417435944610275333, 13.39061984619922718 ) ) ;
#91008=CARTESIAN_POINT ( 'NONE',  ( 6.382347221874473675, 14.49999999999999112, -13.57444820018232079 ) ) ;
#91011=ORIENTED_EDGE ( 'NONE', *, *, #59162, .F. ) ;
#91022=EDGE_CURVE ( 'NONE', #39990, #92022, #26575, .T. ) ;
#91024=CARTESIAN_POINT ( 'NONE',  ( -14.37564666802077262, -2.717705211265421849E-15, 2.692451322017578530 ) ) ;
#91029=CARTESIAN_POINT ( 'NONE',  ( -7.208316651077764980, 15.38393115100078390, -7.208316651077759651 ) ) ;
#91030=VERTEX_POINT ( 'NONE', #64070 ) ;
#91031=ORIENTED_EDGE ( 'NONE', *, *, #1822, .T. ) ;
#91032=DIRECTION ( 'NONE',  ( 0.000000000000000000, 0.000000000000000000, 1.000000000000000000 ) ) ;
#91033=ORIENTED_EDGE ( 'NONE', *, *, #10726, .T. ) ;
#91048=ORIENTED_EDGE ( 'NONE', *, *, #49412, .F. ) ;
#91050=AXIS2_PLACEMENT_3D ( 'NONE', #38617, #649, #31098 ) ;
#91055=VECTOR ( 'NONE', #44321, 1000.000000000000000 ) ;
#91059=EDGE_LOOP ( 'NONE', ( #2275, #42359, #91774 ) ) ;
#91065=DIRECTION ( 'NONE',  ( -0.000000000000000000, -1.000000000000000000, -0.000000000000000000 ) ) ;
#91071=ORIENTED_EDGE ( 'NONE', *, *, #84820, .T. ) ;
#91072=CARTESIAN_POINT ( 'NONE',  ( 11.62719953690064933, 0.5000000000000004441, -9.476720473301794456 ) ) ;
#91081=B_SPLINE_CURVE_WITH_KNOTS ( 'NONE', 3,
 ( #3405, #17432, #40427, #56407, #47900, #33867 ),
 .UNSPECIFIED., .F., .F.,
 ( 4, 2, 4 ),
 ( 0.0002800075630785971810, 0.0006862128664729002202, 0.001092418169867203151 ),
 .UNSPECIFIED. ) ;
#91082=VECTOR ( 'NONE', #64610, 1000.000000000000000 ) ;
#91096=CARTESIAN_POINT ( 'NONE',  ( 5.440088680355549045, -13.60298132251182324, -9.422509992056141925 ) ) ;
#91098=CARTESIAN_POINT ( 'NONE',  ( 13.78891971893211021, 0.3639314269420867998, -5.904717858191556701 ) ) ;
#91100=CARTESIAN_POINT ( 'NONE',  ( 13.14228782657346528, 14.49999999999999112, -7.230509711182246058 ) ) ;
#91101=CARTESIAN_POINT ( 'NONE',  ( 14.16722289976685012, 0.5000000000000004441, -4.928467845925517565 ) ) ;
#91113=DIRECTION ( 'NONE',  ( -0.000000000000000000, -1.000000000000000000, -0.000000000000000000 ) ) ;
#91114=AXIS2_PLACEMENT_3D ( 'NONE', #62442, #8962, #39959 ) ;
#91116=VERTEX_POINT ( 'NONE', #78110 ) ;
#91126=PLANE ( 'NONE',  #53797 ) ;
#91128=CIRCLE ( 'NONE', #86358, 14.49999999999999822 ) ;
#91129=FACE_OUTER_BOUND ( 'NONE', #82300, .T. ) ;
#91146=CARTESIAN_POINT ( 'NONE',  ( 4.923371831947301658, -22.32440218233254470, 8.527530157486175710 ) ) ;
#91161=CARTESIAN_POINT ( 'NONE',  ( -12.81628187352647963, 18.91530133659709634, -3.434112377981046293 ) ) ;
#91162=ORIENTED_EDGE ( 'NONE', *, *, #77384, .T. ) ;
#91165=EDGE_LOOP ( 'NONE', ( #5698, #94141, #57368, #8096 ) ) ;
#91169=CARTESIAN_POINT ( 'NONE',  ( 13.16740645155967115, 0.04922511925147067535, 6.653232860246649061 ) ) ;
#91174=CARTESIAN_POINT ( 'NONE',  ( 7.003840667633727257, 6.657678965418798693E-16, -12.84073839985654608 ) ) ;
#91176=ORIENTED_EDGE ( 'NONE', *, *, #36022, .F. ) ;
#91177=DIRECTION ( 'NONE',  ( 0.000000000000000000, 0.000000000000000000, -1.000000000000000000 ) ) ;
#91183=CARTESIAN_POINT ( 'NONE',  ( 1.915564264621432589, 3.914659629196372862E-16, -14.37291249357990530 ) ) ;
#91186=FACE_OUTER_BOUND ( 'NONE', #25150, .T. ) ;
#91198=CARTESIAN_POINT ( 'NONE',  ( 11.61621867929611973, -0.03417435944610275333, -10.99731149103385874 ) ) ;
#91200=ORIENTED_EDGE ( 'NONE', *, *, #10994, .F. ) ;
#91201=CARTESIAN_POINT ( 'NONE',  ( 0.000000000000000000, 0.5000000000000004441, 0.000000000000000000 ) ) ;
#91213=CARTESIAN_POINT ( 'NONE',  ( 12.26659068614894466, 24.72041550158063217, -7.082119434687053960 ) ) ;
#91217=CIRCLE ( 'NONE', #260, 14.49999999999999822 ) ;
#91225=EDGE_CURVE ( 'NONE', #48243, #97330, #49562, .T. ) ;
#91230=DIRECTION ( 'NONE',  ( 0.8433914458128920488, 0.000000000000000000, -0.5372996083468137840 ) ) ;
#91235=ADVANCED_FACE ( 'NONE', ( #96078 ), #19574, .F. ) ;
#91236=ORIENTED_EDGE ( 'NONE', *, *, #59388, .F. ) ;
#91239=FACE_OUTER_BOUND ( 'NONE', #18744, .T. ) ;
#91249=AXIS2_PLACEMENT_3D ( 'NONE', #49055, #79558, #34031 ) ;
#91250=VERTEX_POINT ( 'NONE', #20568 ) ;
#91253=DIRECTION ( 'NONE',  ( 0.000000000000000000, 1.000000000000000000, 0.000000000000000000 ) ) ;
#91268=ADVANCED_FACE ( 'NONE', ( #80074 ), #35444, .T. ) ;
#91269=VERTEX_POINT ( 'NONE', #74539 ) ;
#91274=ORIENTED_EDGE ( 'NONE', *, *, #92796, .F. ) ;
#91279=CARTESIAN_POINT ( 'NONE',  ( 0.000000000000000000, 14.49999999999999822, 0.000000000000000000 ) ) ;
#91280=VERTEX_POINT ( 'NONE', #81060 ) ;
#91288=FACE_OUTER_BOUND ( 'NONE', #44779, .T. ) ;
#91293=ORIENTED_EDGE ( 'NONE', *, *, #54887, .F. ) ;
#91306=DIRECTION ( 'NONE',  ( 0.000000000000000000, 1.000000000000000000, 0.000000000000000000 ) ) ;
#91315=CIRCLE ( 'NONE', #48203, 15.00000000000000000 ) ;
#91317=PLANE ( 'NONE',  #3986 ) ;
#91322=VERTEX_POINT ( 'NONE', #95578 ) ;
#91323=DIRECTION ( 'NONE',  ( 0.000000000000000000, 0.000000000000000000, 1.000000000000000000 ) ) ;
#91325=CARTESIAN_POINT ( 'NONE',  ( -14.16722289976678617, 15.00000000000000000, -4.928467845925704083 ) ) ;
#91341=DIRECTION ( 'NONE',  ( 0.000000000000000000, 1.000000000000000000, 0.000000000000000000 ) ) ;
#91342=VERTEX_POINT ( 'NONE', #4590 ) ;
#91343=EDGE_CURVE ( 'NONE', #95512, #33681, #373, .T. ) ;
#91354=EDGE_CURVE ( 'NONE', #28441, #16892, #92974, .T. ) ;
#91355=ORIENTED_EDGE ( 'NONE', *, *, #16039, .F. ) ;
#91357=CARTESIAN_POINT ( 'NONE',  ( -11.35178980618966804, 14.49999999999999112, -9.804941009312102551 ) ) ;
#91368=LINE ( 'NONE', #22894, #13157 ) ;
#91370=AXIS2_PLACEMENT_3D ( 'NONE', #89559, #22066, #90532 ) ;
#91375=CARTESIAN_POINT ( 'NONE',  ( -7.771322705638593398, 15.00000000000000000, 12.24159072200411380 ) ) ;
#91384=ORIENTED_EDGE ( 'NONE', *, *, #88912, .T. ) ;
#91387=EDGE_CURVE ( 'NONE', #76539, #38225, #42851, .T. ) ;
#91391=VECTOR ( 'NONE', #28210, 1000.000000000000000 ) ;
#91395=CARTESIAN_POINT ( 'NONE',  ( -14.26328062697239751, 14.95037112300443383, -3.770429249334984245 ) ) ;
#91398=CARTESIAN_POINT ( 'NONE',  ( -5.795997163829992083, 0.000000000000000000, -13.01802277140713926 ) ) ;
#91399=AXIS2_PLACEMENT_3D ( 'NONE', #6827, #13839, #6325 ) ;
#91402=CIRCLE ( 'NONE', #51436, 14.49999999999999822 ) ;
#91405=VERTEX_POINT ( 'NONE', #68042 ) ;
#91408=CARTESIAN_POINT ( 'NONE',  ( 12.81628187352647252, -3.168031996736245137, -3.434112377981059172 ) ) ;
#91413=DIRECTION ( 'NONE',  ( 0.000000000000000000, 0.000000000000000000, 1.000000000000000000 ) ) ;
#91418=VECTOR ( 'NONE', #76943, 1000.000000000000000 ) ;
#91437=DIRECTION ( 'NONE',  ( 0.000000000000000000, 1.000000000000000000, 0.000000000000000000 ) ) ;
#91444=EDGE_CURVE ( 'NONE', #24643, #26555, #36832, .T. ) ;
#91459=LINE ( 'NONE', #45968, #91418 ) ;
#91464=CARTESIAN_POINT ( 'NONE',  ( -12.26659068614895354, -8.612917831752692877, -7.082119434687038861 ) ) ;
#91465=AXIS2_PLACEMENT_3D ( 'NONE', #59383, #28880, #81889 ) ;
#91469=VERTEX_POINT ( 'NONE', #69028 ) ;
#91472=LINE ( 'NONE', #39948, #17897 ) ;
#91476=AXIS2_PLACEMENT_3D ( 'NONE', #79411, #33878, #79889 ) ;
#91477=DIRECTION ( 'NONE',  ( 0.9890158633619187123, 0.000000000000000000, -0.1478094111295981949 ) ) ;
#91479=ADVANCED_FACE ( 'NONE', ( #68 ), #69013, .T. ) ;
#91484=CARTESIAN_POINT ( 'NONE',  ( -5.440088680355547268, 23.89701867748818387, 9.422509992056143702 ) ) ;
#91492=ORIENTED_EDGE ( 'NONE', *, *, #58102, .T. ) ;
#91495=CARTESIAN_POINT ( 'NONE',  ( -5.448048636097841957, 0.000000000000000000, -0.2378669404635215812 ) ) ;
#91501=DIRECTION ( 'NONE',  ( 0.000000000000000000, 1.000000000000000000, 0.000000000000000000 ) ) ;
#91505=DIRECTION ( 'NONE',  ( 0.000000000000000000, 0.000000000000000000, 1.000000000000000000 ) ) ;
#91511=VECTOR ( 'NONE', #10859, 1000.000000000000000 ) ;
#91521=ORIENTED_EDGE ( 'NONE', *, *, #16837, .F. ) ;
#91522=ORIENTED_EDGE ( 'NONE', *, *, #42417, .T. ) ;
#91523=AXIS2_PLACEMENT_3D ( 'NONE', #86267, #32757, #87237 ) ;
#91529=DIRECTION ( 'NONE',  ( 0.000000000000000000, 0.000000000000000000, 1.000000000000000000 ) ) ;
#91537=CARTESIAN_POINT ( 'NONE',  ( 3.469446951953614189E-15, 17.25893115100080166, 9.846743663894594434 ) ) ;
#91540=EDGE_LOOP ( 'NONE', ( #42586, #89184, #74165, #95328 ) ) ;
#91547=EDGE_CURVE ( 'NONE', #48799, #16296, #64197, .T. ) ;
#91550=TOROIDAL_SURFACE ( 'NONE', #3765, 14.49999999999999822, 0.5000000000000000000 ) ;
#91566=ORIENTED_EDGE ( 'NONE', *, *, #8526, .F. ) ;
#91570=CARTESIAN_POINT ( 'NONE',  ( 0.000000000000000000, 15.00000000000000000, 0.000000000000000000 ) ) ;
#91572=EDGE_CURVE ( 'NONE', #66663, #67824, #72580, .T. ) ;
#91579=ORIENTED_EDGE ( 'NONE', *, *, #91840, .T. ) ;
#91580=CARTESIAN_POINT ( 'NONE',  ( 0.000000000000000000, 0.000000000000000000, 0.000000000000000000 ) ) ;
#91585=CARTESIAN_POINT ( 'NONE',  ( -12.34086200392816757, 15.00000000000000000, -7.125000000000143885 ) ) ;
#91590=ORIENTED_EDGE ( 'NONE', *, *, #47982, .T. ) ;
#91591=ORIENTED_EDGE ( 'NONE', *, *, #61362, .F. ) ;
#91603=CARTESIAN_POINT ( 'NONE',  ( -9.422509992056136596, -6.519647989178492864, 5.440088680355559703 ) ) ;
#91608=CARTESIAN_POINT ( 'NONE',  ( -14.17193700899791153, -0.03417435944610275333, 1.489530601563921808 ) ) ;
#91614=AXIS2_PLACEMENT_3D ( 'NONE', #86715, #18219, #48699 ) ;
#91617=CARTESIAN_POINT ( 'NONE',  ( 13.82671409943293739, -0.03417435944610275333, 3.447387012295318076 ) ) ;
#91634=VERTEX_POINT ( 'NONE', #92497 ) ;
#91649=CARTESIAN_POINT ( 'NONE',  ( -4.923371831947302546, -24.82440218233254470, -8.527530157486173934 ) ) ;
#91650=VERTEX_POINT ( 'NONE', #71000 ) ;
#91654=ORIENTED_EDGE ( 'NONE', *, *, #95067, .F. ) ;
#91662=CARTESIAN_POINT ( 'NONE',  ( 0.000000000000000000, 0.000000000000000000, 0.000000000000000000 ) ) ;
#91665=CARTESIAN_POINT ( 'NONE',  ( 9.382169495545419124, 25.99863466993042849, 9.382169495545417348 ) ) ;
#91666=ORIENTED_EDGE ( 'NONE', *, *, #13689, .F. ) ;
#91678=CARTESIAN_POINT ( 'NONE',  ( -3.843478602184641435, 14.76930270348882068, 14.43834224996319904 ) ) ;
#91679=EDGE_CURVE ( 'NONE', #22307, #61223, #4833, .T. ) ;
#91681=VECTOR ( 'NONE', #1943, 1000.000000000000000 ) ;
#91682=CARTESIAN_POINT ( 'NONE',  ( -14.40939250470707478, 15.00000000000000000, -1.618458416369986219 ) ) ;
#91685=DIRECTION ( 'NONE',  ( -0.000000000000000000, -1.000000000000000000, -0.000000000000000000 ) ) ;
#91686=ADVANCED_FACE ( 'NONE', ( #25013 ), #46647, .T. ) ;
#91688=DIRECTION ( 'NONE',  ( 0.000000000000000000, 0.000000000000000000, -1.000000000000000000 ) ) ;
#91689=CARTESIAN_POINT ( 'NONE',  ( 11.35178980618970890, 0.3639309078821234555, 9.804941009312011957 ) ) ;
#91691=DIRECTION ( 'NONE',  ( 0.000000000000000000, 0.000000000000000000, -1.000000000000000000 ) ) ;
#91708=CARTESIAN_POINT ( 'NONE',  ( 0.000000000000000000, 14.49999999999999822, 0.000000000000000000 ) ) ;
#91712=LINE ( 'NONE', #23231, #18496 ) ;
#91713=DIRECTION ( 'NONE',  ( 0.5664062369248313855, 0.000000000000000000, -0.8241261886220166977 ) ) ;
#91719=CARTESIAN_POINT ( 'NONE',  ( 14.16423886937410259, 14.30374883491396965, -2.602085213965210642E-15 ) ) ;
#91728=ORIENTED_EDGE ( 'NONE', *, *, #6958, .T. ) ;
#91733=CARTESIAN_POINT ( 'NONE',  ( 0.000000000000000000, 0.000000000000000000, 0.000000000000000000 ) ) ;
#91735=DIRECTION ( 'NONE',  ( -0.000000000000000000, -1.000000000000000000, -0.000000000000000000 ) ) ;
#91739=EDGE_LOOP ( 'NONE', ( #45193, #24881, #8639, #91920, #79175, #55125 ) ) ;
#91749=CARTESIAN_POINT ( 'NONE',  ( 5.815502996284858561, 0.2306972965111901419, 13.76292046016126491 ) ) ;
#91754=CARTESIAN_POINT ( 'NONE',  ( -14.91886229468042835, 0.2301503527634116975, 0.8060919667643461350 ) ) ;
#91755=DIRECTION ( 'NONE',  ( 0.000000000000000000, 1.000000000000000000, 0.000000000000000000 ) ) ;
#91760=CARTESIAN_POINT ( 'NONE',  ( 0.000000000000000000, 0.5000000000000004441, 0.000000000000000000 ) ) ;
#91767=VECTOR ( 'NONE', #53587, 1000.000000000000000 ) ;
#91770=ORIENTED_EDGE ( 'NONE', *, *, #7727, .F. ) ;
#91774=ORIENTED_EDGE ( 'NONE', *, *, #24306, .F. ) ;
#91786=ORIENTED_EDGE ( 'NONE', *, *, #55130, .F. ) ;
#91791=CARTESIAN_POINT ( 'NONE',  ( 3.927832320392247389, -0.03417435944610275333, -13.69797916712104602 ) ) ;
#91797=EDGE_CURVE ( 'NONE', #15375, #3422, #45151, .T. ) ;
#91823=B_SPLINE_CURVE_WITH_KNOTS ( 'NONE', 3,
 ( #27547, #90511, #88549, #73536, #67037, #6049 ),
 .UNSPECIFIED., .F., .F.,
 ( 4, 2, 4 ),
 ( 3.409110551496111717E-05, 0.0004400426677367851622, 0.0008459942299586092071 ),
 .UNSPECIFIED. ) ;
#91835=EDGE_CURVE ( 'NONE', #30837, #67657, #41630, .T. ) ;
#91839=DIRECTION ( 'NONE',  ( -0.000000000000000000, 1.000000000000000000, -0.000000000000000000 ) ) ;
#91840=EDGE_CURVE ( 'NONE', #74794, #65046, #37186, .T. ) ;
#91851=DIRECTION ( 'NONE',  ( 0.000000000000000000, 0.000000000000000000, 1.000000000000000000 ) ) ;
#91858=CARTESIAN_POINT ( 'NONE',  ( -10.84451454130491399, 15.00000000000000000, -9.625305416630974165 ) ) ;
#91863=CARTESIAN_POINT ( 'NONE',  ( -14.93928340878672145, 14.76930270348881180, -0.2363597353051685723 ) ) ;
#91864=CARTESIAN_POINT ( 'NONE',  ( 8.209432707284861408, 0.5000000000000004441, -12.55409154915486170 ) ) ;
#91868=CARTESIAN_POINT ( 'NONE',  ( 5.376821459231094558, 14.76984886575368705, -13.93958558162744055 ) ) ;
#91869=CARTESIAN_POINT ( 'NONE',  ( -5.925933864965021947, 1.825967504928687424, -10.35061266127159563 ) ) ;
#91874=VECTOR ( 'NONE', #35141, 1000.000000000000000 ) ;
#91891=AXIS2_PLACEMENT_3D ( 'NONE', #25499, #61991, #2516 ) ;
#91898=CARTESIAN_POINT ( 'NONE',  ( -14.62617646268093807, 14.63606916781938594, 3.327906561566777999 ) ) ;
#91911=CIRCLE ( 'NONE', #68012, 14.49999999999999822 ) ;
#91912=EDGE_CURVE ( 'NONE', #12953, #54148, #76413, .T. ) ;
#91920=ORIENTED_EDGE ( 'NONE', *, *, #2392, .T. ) ;
#91924=PLANE ( 'NONE',  #71469 ) ;
#91931=DIRECTION ( 'NONE',  ( -0.9723699203976773342, 0.000000000000000000, 0.2334453638559024768 ) ) ;
#91933=ORIENTED_EDGE ( 'NONE', *, *, #10881, .F. ) ;
#91934=LINE ( 'NONE', #23462, #74098 ) ;
#91947=EDGE_LOOP ( 'NONE', ( #92276, #23579, #21823, #93371 ) ) ;
#91951=CARTESIAN_POINT ( 'NONE',  ( -9.641087339108761256, 14.95077488074853456, -11.16671550067062135 ) ) ;
#91955=CARTESIAN_POINT ( 'NONE',  ( 10.36894250292379027, -6.321251165086028578, 10.36894250292378672 ) ) ;
#91959=TOROIDAL_SURFACE ( 'NONE', #5746, 14.49999999999999822, 0.5000000000000000000 ) ;
#91972=CARTESIAN_POINT ( 'NONE',  ( -14.94699059465099822, 0.5000000000000004441, -1.259949270175015013 ) ) ;
#91978=DIRECTION ( 'NONE',  ( -0.000000000000000000, -1.000000000000000000, -0.000000000000000000 ) ) ;
#91998=CARTESIAN_POINT ( 'NONE',  ( 0.000000000000000000, 0.5000000000000004441, 0.000000000000000000 ) ) ;
#92001=AXIS2_PLACEMENT_3D ( 'NONE', #48156, #78669, #2697 ) ;
#92002=EDGE_CURVE ( 'NONE', #67942, #92547, #60418, .T. ) ;
#92004=CARTESIAN_POINT ( 'NONE',  ( 0.000000000000000000, 0.000000000000000000, 0.000000000000000000 ) ) ;
#92021=CARTESIAN_POINT ( 'NONE',  ( -7.208316651077764980, 25.38393115100079100, -7.208316651077759651 ) ) ;
#92022=VERTEX_POINT ( 'NONE', #15444 ) ;
#92024=B_SPLINE_CURVE_WITH_KNOTS ( 'NONE', 3,
 ( #78153, #47659, #33131, #94132, #18639, #9664 ),
 .UNSPECIFIED., .F., .F.,
 ( 4, 2, 4 ),
 ( 3.409110551494545045E-05, 0.0004400426677367704170, 0.0008459942299585954378 ),
 .UNSPECIFIED. ) ;
#92025=ORIENTED_EDGE ( 'NONE', *, *, #31633, .T. ) ;
#92040=ADVANCED_FACE ( 'NONE', ( #45414 ), #17977, .T. ) ;
#92048=CARTESIAN_POINT ( 'NONE',  ( -12.50534872682722565, 4.101355178835516792E-16, -7.339363270777700343 ) ) ;
#92049=TOROIDAL_SURFACE ( 'NONE', #72915, 14.49999999999999822, 0.5000000000000000000 ) ;
#92052=VERTEX_POINT ( 'NONE', #38917 ) ;
#92058=CARTESIAN_POINT ( 'NONE',  ( 3.469446951953614189E-15, 8.912123368507815613, 11.92686044187656513 ) ) ;
#92065=ORIENTED_EDGE ( 'NONE', *, *, #45429, .F. ) ;
#92072=EDGE_CURVE ( 'NONE', #81875, #54039, #72263, .T. ) ;
#92075=CARTESIAN_POINT ( 'NONE',  ( 0.000000000000000000, 0.5000000000000004441, 0.000000000000000000 ) ) ;
#92078=EDGE_LOOP ( 'NONE', ( #31538, #84846, #19015, #40878 ) ) ;
#92085=DIRECTION ( 'NONE',  ( 0.000000000000000000, 0.000000000000000000, 1.000000000000000000 ) ) ;
#92090=CARTESIAN_POINT ( 'NONE',  ( -7.964842623401172439, -1.311314655845159605, 7.964842623401183097 ) ) ;
#92102=VECTOR ( 'NONE', #68698, 1000.000000000000000 ) ;
#92107=ORIENTED_EDGE ( 'NONE', *, *, #41920, .T. ) ;
#92116=CARTESIAN_POINT ( 'NONE',  ( 0.7577696756375204012, 14.76984978199329568, 14.92139465029755385 ) ) ;
#92119=AXIS2_PLACEMENT_3D ( 'NONE', #94285, #79292, #87763 ) ;
#92121=CARTESIAN_POINT ( 'NONE',  ( 5.817157072110803462, 0.3639308157993877413, -13.82608706751090821 ) ) ;
#92124=EDGE_CURVE ( 'NONE', #65059, #49672, #29159, .T. ) ;
#92129=CIRCLE ( 'NONE', #63352, 14.49999999999999822 ) ;
#92141=CARTESIAN_POINT ( 'NONE',  ( 7.208316651077762316, -10.86606884899921610, -7.208316651077764980 ) ) ;
#92143=DIRECTION ( 'NONE',  ( -0.3987490689252593534, -0.000000000000000000, 0.9170600743851183845 ) ) ;
#92144=CARTESIAN_POINT ( 'NONE',  ( 4.873787042390699931, 15.00000000000000000, 13.39061984619922718 ) ) ;
#92152=DIRECTION ( 'NONE',  ( 0.000000000000000000, 0.000000000000000000, 1.000000000000000000 ) ) ;
#92155=CARTESIAN_POINT ( 'NONE',  ( 11.09922568453594671, 17.04030133659709279, -6.408140936763241591 ) ) ;
#92157=ORIENTED_EDGE ( 'NONE', *, *, #73815, .F. ) ;
#92168=ADVANCED_FACE ( 'NONE', ( #92880 ), #38745, .T. ) ;
#92169=CARTESIAN_POINT ( 'NONE',  ( 7.313705784284593392, 0.5000000000000004441, -13.09617149020743732 ) ) ;
#92170=VERTEX_POINT ( 'NONE', #18377 ) ;
#92171=CARTESIAN_POINT ( 'NONE',  ( -14.56372689393326780, 0.04962896412619356018, -2.356940382833208059 ) ) ;
#92173=CARTESIAN_POINT ( 'NONE',  ( -8.375939845167600595, 0.000000000000000000, -11.52849216984310310 ) ) ;
#92178=CARTESIAN_POINT ( 'NONE',  ( 6.728851239469011425, 15.00000000000000533, 12.98580270086205601 ) ) ;
#92180=CARTESIAN_POINT ( 'NONE',  ( -5.795997163829992083, 15.00000000000000000, -13.01802277140713926 ) ) ;
#92181=ORIENTED_EDGE ( 'NONE', *, *, #58344, .F. ) ;
#92183=CARTESIAN_POINT ( 'NONE',  ( -13.95806775979402303, 2.100641709190664841E-16, 4.371577651620636829 ) ) ;
#92199=LINE ( 'NONE', #14238, #44136 ) ;
#92208=CARTESIAN_POINT ( 'NONE',  ( 3.469446951953614189E-15, 23.05374883491398563, 14.16423886937410259 ) ) ;
#92211=CARTESIAN_POINT ( 'NONE',  ( 3.192513988408121950, 15.00000000000000000, -14.27292421863750604 ) ) ;
#92212=EDGE_CURVE ( 'NONE', #23913, #15375, #90472, .T. ) ;
#92217=ORIENTED_EDGE ( 'NONE', *, *, #88225, .T. ) ;
#92241=FACE_OUTER_BOUND ( 'NONE', #92278, .T. ) ;
#92243=AXIS2_PLACEMENT_3D ( 'NONE', #43065, #34064, #80073 ) ;
#92248=CARTESIAN_POINT ( 'NONE',  ( 11.25000000000000178, 5.213468844518207135, 3.014428414850127691 ) ) ;
#92253=DIRECTION ( 'NONE',  ( 0.6755902076156591329, 0.000000000000000000, -0.7372773368101250835 ) ) ;
#92258=CARTESIAN_POINT ( 'NONE',  ( 0.000000000000000000, 0.5000000000000004441, 0.000000000000000000 ) ) ;
#92267=ORIENTED_EDGE ( 'NONE', *, *, #40495, .T. ) ;
#92273=ORIENTED_EDGE ( 'NONE', *, *, #51299, .F. ) ;
#92276=ORIENTED_EDGE ( 'NONE', *, *, #9646, .F. ) ;
#92277=CARTESIAN_POINT ( 'NONE',  ( -2.393480905993250918, 15.00000000000000000, 14.80781041047749724 ) ) ;
#92278=EDGE_LOOP ( 'NONE', ( #8665, #4626, #54475, #91071, #71854, #60070, #77752, #35312, #46884, #42499, #60768, #67154, #23969, #40815, #76641, #13490, #79699, #89801, #47427, #48088, #48005, #3430, #85643, #60885, #89500, #3737, #77049, #98707, #98086, #94611, #37309, #88567, #77696, #17752, #79012, #32123, #62791, #66310, #91033, #13578, #28015, #56520, #36569, #52841, #95598, #85613, #98675, #98484, #42268, #94217, #21667, #17415, #68233, #80884, #71795, #87779, #43465, #97335, #27889, #74757, #16915, #47249, #24518, #73181, #53922, #34621, #29771, #2155, #46686, #34657, #93200, #7062, #34398, #98329, #45065, #21553, #49111, #20974, #6219, #9100, #95684, #44991, #96570, #86888, #69089, #35691, #52336, #43773, #48496, #78651, #85274, #60308, #52779, #22692, #95555, #61624, #86665, #74141, #54462, #68930, #24036, #50462, #9162, #34159, #19454, #62751, #11629, #24299, #1659, #20860, #73690, #42088, #66593, #7678, #20321, #34410, #2512, #60537, #25378, #97599, #22114, #61514, #75306, #81636, #63469, #22052, #34075, #28793, #78509, #94625, #2020, #69747, #2667, #21027, #78060, #5961, #18247, #12364, #4118, #55049, #12543, #15209, #56504, #39945, #17456, #72474, #85751, #92751, #98250, #89685, #81900, #47119, #90138, #11828, #28796, #51167, #64394, #14379, #57614, #57351, #79016, #5708, #83777, #13368, #21572, #1861, #29142, #86150, #8772, #55246, #65088, #17562, #5824, #80586, #65495, #77515, #60063, #72384, #1310, #34827, #36760, #7715, #17547, #46241, #79468, #31755, #73752, #47638, #52370, #94700, #10261, #7584, #8276, #30636, #33750, #29011, #77808, #9728, #91162, #80783, #35046, #72931, #9561, #97955, #55025, #33634, #11708, #53032, #93390, #29533, #54705, #64175, #22080, #3193, #13968, #47640, #85899, #6700, #27551, #23991, #51151, #56017, #93, #61869, #68036, #34858, #81118, #6147, #64200, #4343, #9757, #6593, #31561, #54648, #10168, #32147, #84907, #1802, #98711, #77365, #50840, #623, #6520, #76575, #5224, #63490, #67408, #66718, #82581, #36786, #59024, #63077, #48018, #85979, #34452, #10612, #98191, #95105, #33613, #38759, #60413, #75636, #37599, #31663, #47502, #56469, #44268, #9965, #62132, #57440 ) ) ;
#92294=CARTESIAN_POINT ( 'NONE',  ( 3.469446951953614189E-15, 11.36803362898265135, 11.25000000000000178 ) ) ;
#92323=DIRECTION ( 'NONE',  ( -0.06104853953484969814, 0.000000000000000000, -0.9981347984218674751 ) ) ;
#92327=CARTESIAN_POINT ( 'NONE',  ( -12.74305857943740428, -2.641472246012534819E-15, -7.177950183687037189 ) ) ;
#92335=CARTESIAN_POINT ( 'NONE',  ( 0.000000000000000000, 0.5000000000000004441, 0.000000000000000000 ) ) ;
#92342=ORIENTED_EDGE ( 'NONE', *, *, #79976, .T. ) ;
#92343=CARTESIAN_POINT ( 'NONE',  ( -2.913501739333859586, 15.00000000000000000, 14.20427779279530434 ) ) ;
#92349=DIRECTION ( 'NONE',  ( -0.000000000000000000, -1.000000000000000000, -0.000000000000000000 ) ) ;
#92375=CYLINDRICAL_SURFACE ( 'NONE', #53795, 11.25000000000000178 ) ;
#92380=CARTESIAN_POINT ( 'NONE',  ( -14.42525372082707236, 14.76984920709440452, -3.890283033989385242 ) ) ;
#92384=CARTESIAN_POINT ( 'NONE',  ( 9.997910040112534702, 4.470079180682592273E-16, 10.50199004140724490 ) ) ;
#92388=ORIENTED_EDGE ( 'NONE', *, *, #53885, .F. ) ;
#92393=CARTESIAN_POINT ( 'NONE',  ( -1.548803529118062405, 0.000000000000000000, 5.228673087012083442 ) ) ;
#92399=AXIS2_PLACEMENT_3D ( 'NONE', #41762, #73212, #12224 ) ;
#92402=VERTEX_POINT ( 'NONE', #90342 ) ;
#92406=EDGE_LOOP ( 'NONE', ( #45658, #92762, #51665, #35999 ) ) ;
#92412=CARTESIAN_POINT ( 'NONE',  ( -1.915564264621532287, 4.395349792408769378E-16, 14.37291249357989287 ) ) ;
#92425=CARTESIAN_POINT ( 'NONE',  ( -7.154372922009654800, 15.00000000000000000, 14.30707323420372035 ) ) ;
#92431=CARTESIAN_POINT ( 'NONE',  ( -3.866352809136022195, 14.95037102884348634, -14.23757791217075308 ) ) ;
#92435=CARTESIAN_POINT ( 'NONE',  ( 0.000000000000000000, 15.00000000000000000, 0.000000000000000000 ) ) ;
#92441=CARTESIAN_POINT ( 'NONE',  ( 7.082119434687047743, -4.862917831752689324, -12.26659068614894821 ) ) ;
#92447=DIRECTION ( 'NONE',  ( -0.000000000000000000, -1.000000000000000000, -0.000000000000000000 ) ) ;
#92449=DIRECTION ( 'NONE',  ( -0.6225146366376130835, 0.000000000000000000, -0.7826081568524191345 ) ) ;
#92454=CARTESIAN_POINT ( 'NONE',  ( 2.393480905993088381, 14.49999999999999112, 14.80781041047758784 ) ) ;
#92456=CARTESIAN_POINT ( 'NONE',  ( -12.83294900548068895, 15.00000000000000000, 7.766300266068274283 ) ) ;
#92475=CARTESIAN_POINT ( 'NONE',  ( 10.70613742633251420, 4.218616272510096815E-16, 9.778988772285311271 ) ) ;
#92477=DIRECTION ( 'NONE',  ( -0.000000000000000000, -1.000000000000000000, -0.000000000000000000 ) ) ;
#92490=CARTESIAN_POINT ( 'NONE',  ( 5.038135815954128738, 0.000000000000000000, 2.086864184045826853 ) ) ;
#92497=CARTESIAN_POINT ( 'NONE',  ( 0.9940297508537879745, 0.000000000000000000, -14.21528771620249820 ) ) ;
#92504=CARTESIAN_POINT ( 'NONE',  ( 8.606322355891263598, 15.00000000000000000, 11.66967075398811282 ) ) ;
#92505=CARTESIAN_POINT ( 'NONE',  ( 8.527530157486175710, 28.92559781766745886, -4.923371831947298993 ) ) ;
#92508=B_SPLINE_CURVE_WITH_KNOTS ( 'NONE', 3,
 ( #38013, #15518, #23512, #38502, #75006, #14026 ),
 .UNSPECIFIED., .F., .F.,
 ( 4, 2, 4 ),
 ( 3.409110551404661974E-05, 0.0004400426677358954116, 0.0008459942299577441222 ),
 .UNSPECIFIED. ) ;
#92529=CARTESIAN_POINT ( 'NONE',  ( 14.16722289976681814, 15.00000000000000000, 4.928467845925615265 ) ) ;
#92530=DIRECTION ( 'NONE',  ( -0.4305110968082986878, 0.000000000000000000, 0.9025852843498588518 ) ) ;
#92532=ORIENTED_EDGE ( 'NONE', *, *, #68311, .T. ) ;
#92540=VECTOR ( 'NONE', #6885, 1000.000000000000000 ) ;
#92547=VERTEX_POINT ( 'NONE', #11161 ) ;
#92553=VECTOR ( 'NONE', #78467, 1000.000000000000114 ) ;
#92554=FACE_OUTER_BOUND ( 'NONE', #69187, .T. ) ;
#92557=CARTESIAN_POINT ( 'NONE',  ( -6.091055032734486119, 3.184843881676169275E-16, 13.29802223412754003 ) ) ;
#92559=ORIENTED_EDGE ( 'NONE', *, *, #20324, .F. ) ;
#92561=VERTEX_POINT ( 'NONE', #95141 ) ;
#92567=CARTESIAN_POINT ( 'NONE',  ( 14.62617646268088478, 0.3640475087720987935, -3.327906561566882360 ) ) ;
#92569=B_SPLINE_CURVE_WITH_KNOTS ( 'NONE', 3,
 ( #25909, #87870, #19386, #81360, #63882, #42877 ),
 .UNSPECIFIED., .F., .F.,
 ( 4, 2, 4 ),
 ( 3.409110551496205229E-05, 0.0004400426677368001241, 0.0008459942299586382638 ),
 .UNSPECIFIED. ) ;
#92575=CARTESIAN_POINT ( 'NONE',  ( 10.88017736071110519, -4.436314655845152721, -2.602085213965210642E-15 ) ) ;
#92577=CARTESIAN_POINT ( 'NONE',  ( -1.780824192092276048, 14.49999999999999112, -14.89391369643522545 ) ) ;
#92578=EDGE_CURVE ( 'NONE', #26584, #60992, #89236, .T. ) ;
#92581=PLANE ( 'NONE',  #30507 ) ;
#92591=DIRECTION ( 'NONE',  ( 0.1822355254921578793, 0.000000000000000000, -0.9832549075639526182 ) ) ;
#92608=ORIENTED_EDGE ( 'NONE', *, *, #23736, .F. ) ;
#92623=CARTESIAN_POINT ( 'NONE',  ( -9.846743663894596210, -4.199402182332548250, -2.638427012816824124 ) ) ;
#92626=ORIENTED_EDGE ( 'NONE', *, *, #76791, .F. ) ;
#92632=PLANE ( 'NONE',  #24709 ) ;
#92640=ORIENTED_EDGE ( 'NONE', *, *, #79255, .T. ) ;
#92649=B_SPLINE_CURVE_WITH_KNOTS ( 'NONE', 3,
 ( #57117, #63146, #71158, #10162, #17670, #42139 ),
 .UNSPECIFIED., .F., .F.,
 ( 4, 2, 4 ),
 ( 3.409110551494519295E-05, 0.0004400426677367694954, 0.0008459942299585938115 ),
 .UNSPECIFIED. ) ;
#92653=VERTEX_POINT ( 'NONE', #29112 ) ;
#92665=B_SPLINE_CURVE_WITH_KNOTS ( 'NONE', 3,
 ( #31162, #15208, #67708, #219, #23200, #53675 ),
 .UNSPECIFIED., .F., .F.,
 ( 4, 2, 4 ),
 ( 0.0002800392683685244992, 0.0006862448819815560649, 0.001092450495594587739 ),
 .UNSPECIFIED. ) ;
#92676=EDGE_CURVE ( 'NONE', #77111, #42622, #75114, .T. ) ;
#92678=DIRECTION ( 'NONE',  ( 0.000000000000000000, 0.000000000000000000, 1.000000000000000000 ) ) ;
#92683=LINE ( 'NONE', #47174, #80723 ) ;
#92684=DIRECTION ( 'NONE',  ( -0.000000000000000000, -1.000000000000000000, -0.000000000000000000 ) ) ;
#92685=CARTESIAN_POINT ( 'NONE',  ( 13.21382278599133286, 15.00000000000000888, 6.271621331965612001 ) ) ;
#92686=AXIS2_PLACEMENT_3D ( 'NONE', #60988, #77468, #83510 ) ;
#92688=DIRECTION ( 'NONE',  ( 0.000000000000000000, 1.000000000000000000, 0.000000000000000000 ) ) ;
#92691=CARTESIAN_POINT ( 'NONE',  ( -10.88017736071110342, -36.93631465584515894, 3.903127820947815962E-15 ) ) ;
#92707=PLANE ( 'NONE',  #48727 ) ;
#92708=CARTESIAN_POINT ( 'NONE',  ( -13.50171220565604280, 14.99999999999793943, -5.622479820949179086 ) ) ;
#92712=ORIENTED_EDGE ( 'NONE', *, *, #56826, .F. ) ;
#92718=CYLINDRICAL_SURFACE ( 'NONE', #87328, 11.25000000000000178 ) ;
#92725=CIRCLE ( 'NONE', #64010, 15.00000000000000000 ) ;
#92729=ORIENTED_EDGE ( 'NONE', *, *, #32039, .T. ) ;
#92730=ORIENTED_EDGE ( 'NONE', *, *, #31800, .F. ) ;
#92739=CARTESIAN_POINT ( 'NONE',  ( 14.35840480524204210, 14.49999999999999112, 4.340070442838943165 ) ) ;
#92748=LINE ( 'NONE', #24272, #25121 ) ;
#92749=ORIENTED_EDGE ( 'NONE', *, *, #90441, .F. ) ;
#92751=ORIENTED_EDGE ( 'NONE', *, *, #67677, .T. ) ;
#92762=ORIENTED_EDGE ( 'NONE', *, *, #64993, .T. ) ;
#92765=DIRECTION ( 'NONE',  ( 0.000000000000000000, 1.000000000000000000, 0.000000000000000000 ) ) ;
#92771=ORIENTED_EDGE ( 'NONE', *, *, #17393, .F. ) ;
#92774=DIRECTION ( 'NONE',  ( 0.000000000000000000, 1.000000000000000000, 0.000000000000000000 ) ) ;
#92777=LINE ( 'NONE', #9783, #69069 ) ;
#92783=CARTESIAN_POINT ( 'NONE',  ( -9.402796353261225093, 14.49999999999999112, 11.68706210897757281 ) ) ;
#92796=EDGE_CURVE ( 'NONE', #68070, #18218, #65504, .T. ) ;
#92797=TOROIDAL_SURFACE ( 'NONE', #6581, 14.49999999999999822, 0.5000000000000000000 ) ;
#92812=CARTESIAN_POINT ( 'NONE',  ( 9.641450013144391207, 0.04962892333244047632, 11.16690429682355301 ) ) ;
#92818=EDGE_CURVE ( 'NONE', #68070, #43044, #69593, .T. ) ;
#92825=AXIS2_PLACEMENT_3D ( 'NONE', #72535, #42074, #34532 ) ;
#92832=CARTESIAN_POINT ( 'NONE',  ( 1.780824192092484326, 14.49999999999999112, -14.89391369643520058 ) ) ;
#92837=CARTESIAN_POINT ( 'NONE',  ( 14.09397099617988935, 0.04962897248923205107, 4.360881834954268399 ) ) ;
#92841=CARTESIAN_POINT ( 'NONE',  ( 14.52941021839283486, 15.00000000000000888, -1.683622718073039426 ) ) ;
#92849=CARTESIAN_POINT ( 'NONE',  ( 8.375939845167682307, 15.00000000000000000, 11.52849216984304448 ) ) ;
#92857=ORIENTED_EDGE ( 'NONE', *, *, #75291, .T. ) ;
#92871=DIRECTION ( 'NONE',  ( 0.000000000000000000, 0.000000000000000000, -1.000000000000000000 ) ) ;
#92880=FACE_OUTER_BOUND ( 'NONE', #5811, .T. ) ;
#92881=CARTESIAN_POINT ( 'NONE',  ( -14.16722289976683946, 14.49999999999999112, -4.928467845925748492 ) ) ;
#92884=EDGE_CURVE ( 'NONE', #93159, #73208, #11670, .T. ) ;
#92885=AXIS2_PLACEMENT_3D ( 'NONE', #29505, #84506, #15534 ) ;
#92891=VECTOR ( 'NONE', #45302, 1000.000000000000000 ) ;
#92892=VERTEX_POINT ( 'NONE', #46586 ) ;
#92893=FACE_OUTER_BOUND ( 'NONE', #92078, .T. ) ;
#92909=CARTESIAN_POINT ( 'NONE',  ( 2.888814634336794640, -2.736763452578643607E-15, -14.33747749179068620 ) ) ;
#92915=CARTESIAN_POINT ( 'NONE',  ( -14.16722289976691407, 0.3639312946971456353, 4.928467845925445623 ) ) ;
#92925=CARTESIAN_POINT ( 'NONE',  ( -12.60589901313210071, 0.5000000000000004441, -8.129656208642224158 ) ) ;
#92928=CARTESIAN_POINT ( 'NONE',  ( -3.795296366450322534, -9.237917831752689324, -14.16423886937409904 ) ) ;
#92936=DIRECTION ( 'NONE',  ( -3.907985046680550391E-14, 0.000000000000000000, 1.000000000000000000 ) ) ;
#92942=CARTESIAN_POINT ( 'NONE',  ( 0.000000000000000000, 0.5000000000000004441, 0.000000000000000000 ) ) ;
#92945=CARTESIAN_POINT ( 'NONE',  ( -14.94699059465103730, 0.3639308806416579611, -1.259949270175004132 ) ) ;
#92955=CARTESIAN_POINT ( 'NONE',  ( 0.000000000000000000, 14.49999999999999822, 0.000000000000000000 ) ) ;
#92956=VECTOR ( 'NONE', #31380, 1000.000000000000000 ) ;
#92964=DIRECTION ( 'NONE',  ( 0.000000000000000000, 0.000000000000000000, 1.000000000000000000 ) ) ;
#92967=ORIENTED_EDGE ( 'NONE', *, *, #81961, .F. ) ;
#92974=CIRCLE ( 'NONE', #13097, 14.49999999999999822 ) ;
#92979=VERTEX_POINT ( 'NONE', #93561 ) ;
#92985=ORIENTED_EDGE ( 'NONE', *, *, #73348, .T. ) ;
#92990=CARTESIAN_POINT ( 'NONE',  ( 4.880290883660371115, 0.000000000000000000, -2.433223276543791780 ) ) ;
#92998=VECTOR ( 'NONE', #91437, 1000.000000000000000 ) ;
#92999=CARTESIAN_POINT ( 'NONE',  ( 1.983216688680936812, -0.03417435944610275333, -14.11131997956737649 ) ) ;
#93000=CARTESIAN_POINT ( 'NONE',  ( -2.638427012816824124, 27.05059781766745886, 9.846743663894596210 ) ) ;
#93001=EDGE_LOOP ( 'NONE', ( #34579, #90741, #43795, #48362, #69417, #86748 ) ) ;
#93002=DIRECTION ( 'NONE',  ( 0.000000000000000000, 1.000000000000000000, 0.000000000000000000 ) ) ;
#93009=EDGE_CURVE ( 'NONE', #11604, #4363, #70128, .T. ) ;
#93010=TOROIDAL_SURFACE ( 'NONE', #40354, 14.49999999999999822, 0.5000000000000000000 ) ;
#93012=ORIENTED_EDGE ( 'NONE', *, *, #73699, .T. ) ;
#93015=ORIENTED_EDGE ( 'NONE', *, *, #51977, .T. ) ;
#93017=ORIENTED_EDGE ( 'NONE', *, *, #78846, .F. ) ;
#93023=CARTESIAN_POINT ( 'NONE',  ( -10.19513985507817821, 0.5000000000000004441, -11.00268709613231088 ) ) ;
#93024=SURFACE_SIDE_STYLE ('',( #86031 ) ) ;
#93026=EDGE_LOOP ( 'NONE', ( #58543, #63514, #61528, #11526 ) ) ;
#93039=FACE_OUTER_BOUND ( 'NONE', #76486, .T. ) ;
#93040=CARTESIAN_POINT ( 'NONE',  ( -12.34086200392816757, -0.03417435944610275333, -7.125000000000143885 ) ) ;
#93043=ORIENTED_EDGE ( 'NONE', *, *, #95980, .T. ) ;
#93052=VERTEX_POINT ( 'NONE', #92577 ) ;
#93061=CARTESIAN_POINT ( 'NONE',  ( 0.000000000000000000, 0.5000000000000004441, 0.000000000000000000 ) ) ;
#93065=CARTESIAN_POINT ( 'NONE',  ( 10.88017736071110164, 5.355352010821507136, 2.915334737309921209 ) ) ;
#93069=CARTESIAN_POINT ( 'NONE',  ( 0.000000000000000000, 14.49999999999999822, 0.000000000000000000 ) ) ;
#93076=CARTESIAN_POINT ( 'NONE',  ( 12.80781515976310203, 0.000000000000000000, 6.246788841744411513 ) ) ;
#93097=ORIENTED_EDGE ( 'NONE', *, *, #94597, .F. ) ;
#93107=AXIS2_PLACEMENT_3D ( 'NONE', #96617, #59582, #4136 ) ;
#93109=CYLINDRICAL_SURFACE ( 'NONE', #44358, 15.00000000000000000 ) ;
#93112=CARTESIAN_POINT ( 'NONE',  ( 7.208316651077764980, -12.11606884899921255, 7.208316651077762316 ) ) ;
#93113=EDGE_LOOP ( 'NONE', ( #17755, #32876, #33359, #29401 ) ) ;
#93114=CARTESIAN_POINT ( 'NONE',  ( 10.82078848414219330, 15.00000000000000000, -11.78082904627298433 ) ) ;
#93115=AXIS2_PLACEMENT_3D ( 'NONE', #66833, #58330, #51341 ) ;
#93122=CARTESIAN_POINT ( 'NONE',  ( 0.000000000000000000, 15.00000000000000000, 0.000000000000000000 ) ) ;
#93124=EDGE_CURVE ( 'NONE', #3849, #79719, #10562, .T. ) ;
#93127=VERTEX_POINT ( 'NONE', #51659 ) ;
#93129=VERTEX_POINT ( 'NONE', #43650 ) ;
#93131=ORIENTED_EDGE ( 'NONE', *, *, #48685, .T. ) ;
#93133=DIRECTION ( 'NONE',  ( 0.1650476058606878405, 0.000000000000000000, -0.9862856015372296614 ) ) ;
#93140=PLANE ( 'NONE',  #58472 ) ;
#93141=ORIENTED_EDGE ( 'NONE', *, *, #47309, .F. ) ;
#93143=ADVANCED_FACE ( 'NONE', ( #50164 ), #66656, .F. ) ;
#93152=CARTESIAN_POINT ( 'NONE',  ( 5.171435456984235124, 0.000000000000000000, -1.730338099013976727 ) ) ;
#93159=VERTEX_POINT ( 'NONE', #38511 ) ;
#93168=DIRECTION ( 'NONE',  ( 0.000000000000000000, 0.000000000000000000, 1.000000000000000000 ) ) ;
#93174=DIRECTION ( 'NONE',  ( -0.9366721892483947931, 0.000000000000000000, -0.3502073812594747593 ) ) ;
#93176=CARTESIAN_POINT ( 'NONE',  ( -14.11917416961171945, 14.76930270348881002, 4.887430353538848138 ) ) ;
#93179=CARTESIAN_POINT ( 'NONE',  ( -14.16423886937410437, 31.59541550158062861, -3.795296366450299885 ) ) ;
#93195=CARTESIAN_POINT ( 'NONE',  ( -13.78891971893204804, 14.49999999999999112, -5.904717858191772528 ) ) ;
#93200=ORIENTED_EDGE ( 'NONE', *, *, #9817, .T. ) ;
#93201=LINE ( 'NONE', #48686, #58893 ) ;
#93209=CARTESIAN_POINT ( 'NONE',  ( 0.000000000000000000, 15.00000000000000000, 0.000000000000000000 ) ) ;
#93213=ORIENTED_EDGE ( 'NONE', *, *, #36345, .F. ) ;
#93214=VERTEX_POINT ( 'NONE', #31961 ) ;
#93216=CARTESIAN_POINT ( 'NONE',  ( 12.60874940350940321, 15.00000000000000000, 7.160268045227115685 ) ) ;
#93224=DIRECTION ( 'NONE',  ( 0.02617694830786938473, 0.000000000000000000, 0.9996573249755573709 ) ) ;
#93228=EDGE_CURVE ( 'NONE', #52174, #89575, #60550, .T. ) ;
#93229=CARTESIAN_POINT ( 'NONE',  ( -10.84451454131299997, 15.00000000000000000, 9.625305416633544553 ) ) ;
#93237=EDGE_LOOP ( 'NONE', ( #56351, #88866, #92967, #31134 ) ) ;
#93241=CARTESIAN_POINT ( 'NONE',  ( 0.000000000000000000, 14.49999999999999822, 0.000000000000000000 ) ) ;
#93242=EDGE_CURVE ( 'NONE', #28267, #94977, #37322, .T. ) ;
#93246=CIRCLE ( 'NONE', #91614, 15.00000000000000000 ) ;
#93249=CARTESIAN_POINT ( 'NONE',  ( 6.408140936763243367, 0.7903013365970906756, 11.09922568453594494 ) ) ;
#93250=ORIENTED_EDGE ( 'NONE', *, *, #58058, .T. ) ;
#93265=ADVANCED_FACE ( 'NONE', ( #85980 ), #73975, .T. ) ;
#93268=CARTESIAN_POINT ( 'NONE',  ( 9.322910753577883014, 0.04922511925147178558, 11.43369735623883621 ) ) ;
#93272=EDGE_CURVE ( 'NONE', #79142, #49345, #77189, .T. ) ;
#93273=LINE ( 'NONE', #47771, #59492 ) ;
#93291=ORIENTED_EDGE ( 'NONE', *, *, #90193, .T. ) ;
#93303=CARTESIAN_POINT ( 'NONE',  ( 0.000000000000000000, 0.5000000000000004441, 0.000000000000000000 ) ) ;
#93312=DIRECTION ( 'NONE',  ( -0.000000000000000000, -1.000000000000000000, -0.000000000000000000 ) ) ;
#93315=DIRECTION ( 'NONE',  ( -0.8788171126619616080, 0.000000000000000000, -0.4771587602596153999 ) ) ;
#93322=AXIS2_PLACEMENT_3D ( 'NONE', #23116, #29592, #135 ) ;
#93323=DIRECTION ( 'NONE',  ( -0.1132032137679106348, 0.000000000000000000, 0.9935718556765870124 ) ) ;
#93335=FACE_OUTER_BOUND ( 'NONE', #63107, .T. ) ;
#93353=ORIENTED_EDGE ( 'NONE', *, *, #40495, .F. ) ;
#93354=EDGE_CURVE ( 'NONE', #39731, #47627, #11741, .T. ) ;
#93359=ORIENTED_EDGE ( 'NONE', *, *, #28024, .T. ) ;
#93363=CARTESIAN_POINT ( 'NONE',  ( 0.000000000000000000, 0.5000000000000004441, 0.000000000000000000 ) ) ;
#93371=ORIENTED_EDGE ( 'NONE', *, *, #31638, .F. ) ;
#93383=DIRECTION ( 'NONE',  ( -0.000000000000000000, -1.000000000000000000, -0.000000000000000000 ) ) ;
#93385=ORIENTED_EDGE ( 'NONE', *, *, #81489, .F. ) ;
#93389=EDGE_CURVE ( 'NONE', #48771, #94701, #96440, .T. ) ;
#93390=ORIENTED_EDGE ( 'NONE', *, *, #51139, .T. ) ;
#93395=CARTESIAN_POINT ( 'NONE',  ( 10.27090289957535596, 15.00000000000000711, -10.41235154178105127 ) ) ;
#93398=DIRECTION ( 'NONE',  ( 0.6087614290087297597, 0.000000000000000000, -0.7933533402912281707 ) ) ;
#93404=ORIENTED_EDGE ( 'NONE', *, *, #18708, .T. ) ;
#93409=CIRCLE ( 'NONE', #8771, 15.00000000000000000 ) ;
#93421=CARTESIAN_POINT ( 'NONE',  ( 12.07856007377828078, 15.00000000000000000, -8.022367888854837759 ) ) ;
#93426=CARTESIAN_POINT ( 'NONE',  ( 10.93781366033347346, 14.63595249122789177, -10.26470809774066417 ) ) ;
#93430=CARTESIAN_POINT ( 'NONE',  ( -7.313705784284680433, 0.5000000000000004441, 13.09617149020738935 ) ) ;
#93431=CARTESIAN_POINT ( 'NONE',  ( 3.795296366450314540, -1.737917831752697317, 14.16423886937410082 ) ) ;
#93433=DIRECTION ( 'NONE',  ( -0.3502073812594687086, 0.000000000000000000, 0.9366721892483971246 ) ) ;
#93434=ORIENTED_EDGE ( 'NONE', *, *, #37851, .T. ) ;
#93437=CARTESIAN_POINT ( 'NONE',  ( 1.780824192092492986, 0.3639308653491441503, -14.89391369643516860 ) ) ;
#93445=DIRECTION ( 'NONE',  ( -0.000000000000000000, -1.000000000000000000, -0.000000000000000000 ) ) ;
#93455=EDGE_CURVE ( 'NONE', #17335, #83513, #80438, .T. ) ;
#93466=CARTESIAN_POINT ( 'NONE',  ( 0.000000000000000000, 15.00000000000000000, 0.000000000000000000 ) ) ;
#93478=ORIENTED_EDGE ( 'NONE', *, *, #67747, .T. ) ;
#93479=DIRECTION ( 'NONE',  ( 0.000000000000000000, 0.000000000000000000, 1.000000000000000000 ) ) ;
#93487=VECTOR ( 'NONE', #18511, 1000.000000000000114 ) ;
#93489=CARTESIAN_POINT ( 'NONE',  ( -5.204170427930421283E-15, 11.67180217785154817, -11.25000000000000178 ) ) ;
#93495=ADVANCED_FACE ( 'NONE', ( #35416 ), #2209, .T. ) ;
#93496=CARTESIAN_POINT ( 'NONE',  ( -9.065164099344370285, 15.00000000000000000, -11.95084933600779564 ) ) ;
#93499=CARTESIAN_POINT ( 'NONE',  ( -9.382169495545422677, -41.50136533006958217, -9.382169495545417348 ) ) ;
#93509=EDGE_CURVE ( 'NONE', #4363, #73542, #4453, .T. ) ;
#93511=EDGE_LOOP ( 'NONE', ( #2138, #38311, #68975, #96590 ) ) ;
#93519=DIRECTION ( 'NONE',  ( 0.7253743710122775301, 0.000000000000000000, 0.6883545756937645699 ) ) ;
#93524=CARTESIAN_POINT ( 'NONE',  ( 14.09394518620610270, 4.258544466044566969E-16, 3.407449058785454898 ) ) ;
#93533=CARTESIAN_POINT ( 'NONE',  ( 13.61464873478166737, 0.5000000000000004441, -6.296136897217838424 ) ) ;
#93543=CARTESIAN_POINT ( 'NONE',  ( 0.2851577207221809851, 14.76930270348882068, 14.93843163678289443 ) ) ;
#93547=ORIENTED_EDGE ( 'NONE', *, *, #39686, .T. ) ;
#93556=CARTESIAN_POINT ( 'NONE',  ( 14.24131928502211686, 0.000000000000000000, -0.4973178280105898241 ) ) ;
#93559=CARTESIAN_POINT ( 'NONE',  ( 9.422509992056141925, 5.980352010821511577, -5.440088680355554374 ) ) ;
#93561=CARTESIAN_POINT ( 'NONE',  ( 4.431036607602602651, 14.49999999999999112, -14.33059365769916305 ) ) ;
#93571=B_SPLINE_CURVE_WITH_KNOTS ( 'NONE', 3,
 ( #45345, #30831, #92812, #67864, #54804, #76340 ),
 .UNSPECIFIED., .F., .F.,
 ( 4, 2, 4 ),
 ( 0.0002800289709865101998, 0.0006862344838253363246, 0.001092439996664162612 ),
 .UNSPECIFIED. ) ;
#93575=CARTESIAN_POINT ( 'NONE',  ( -2.621477372531479055, -0.03417435944610275333, -15.77990027919564575 ) ) ;
#93588=AXIS2_PLACEMENT_3D ( 'NONE', #11144, #72131, #77297 ) ;
#93592=TOROIDAL_SURFACE ( 'NONE', #24957, 14.49999999999999822, 0.5000000000000000000 ) ;
#93594=ORIENTED_EDGE ( 'NONE', *, *, #59478, .T. ) ;
#93609=CARTESIAN_POINT ( 'NONE',  ( -8.527530157486173934, -8.574402182332546474, 4.923371831947302546 ) ) ;
#93613=CARTESIAN_POINT ( 'NONE',  ( 0.000000000000000000, 0.000000000000000000, -13.74999999999999467 ) ) ;
#93620=CARTESIAN_POINT ( 'NONE',  ( -13.34948392230367453, 14.95077488074854166, -6.279918722515163587 ) ) ;
#93621=CARTESIAN_POINT ( 'NONE',  ( -9.641450013144547526, 14.95037107666755816, 11.16690429682342511 ) ) ;
#93622=VECTOR ( 'NONE', #54186, 1000.000000000000000 ) ;
#93623=VECTOR ( 'NONE', #66840, 1000.000000000000000 ) ;
#93624=CIRCLE ( 'NONE', #84069, 15.00000000000000000 ) ;
#93626=VERTEX_POINT ( 'NONE', #86947 ) ;
#93633=CARTESIAN_POINT ( 'NONE',  ( -0.3093388210927896509, 14.49999999999999112, 14.99680997725072373 ) ) ;
#93638=CARTESIAN_POINT ( 'NONE',  ( -1.983216688680738082, -0.03417435944610275333, -14.11131997956740491 ) ) ;
#93642=DIRECTION ( 'NONE',  ( 0.5075383629607025382, 0.000000000000000000, -0.8616291604415267091 ) ) ;
#93644=FACE_OUTER_BOUND ( 'NONE', #21809, .T. ) ;
#93645=DIRECTION ( 'NONE',  ( 0.000000000000000000, 0.000000000000000000, -1.000000000000000000 ) ) ;
#93648=DIRECTION ( 'NONE',  ( -0.000000000000000000, -1.000000000000000000, -0.000000000000000000 ) ) ;
#93653=LINE ( 'NONE', #70675, #49597 ) ;
#93664=ORIENTED_EDGE ( 'NONE', *, *, #73087, .F. ) ;
#93670=CARTESIAN_POINT ( 'NONE',  ( 13.96521320569125102, 14.95077488074853456, -4.755935267939162436 ) ) ;
#93671=CARTESIAN_POINT ( 'NONE',  ( 0.000000000000000000, 15.00000000000000000, 0.000000000000000000 ) ) ;
#93672=CARTESIAN_POINT ( 'NONE',  ( -3.243710765982268818, 0.000000000000000000, -4.383623511354931779 ) ) ;
#93675=CARTESIAN_POINT ( 'NONE',  ( 10.88017736071110164, -34.64464798917848753, 2.915334737309921209 ) ) ;
#93678=LINE ( 'NONE', #10195, #17031 ) ;
#93684=TOROIDAL_SURFACE ( 'NONE', #85701, 14.49999999999999822, 0.5000000000000000000 ) ;
#93698=CARTESIAN_POINT ( 'NONE',  ( 8.375939845167682307, -0.03417435944610275333, 11.52849216984304448 ) ) ;
#93710=EDGE_LOOP ( 'NONE', ( #25376, #40865, #436, #64690, #16285, #81573 ) ) ;
#93712=PLANE ( 'NONE',  #73421 ) ;
#93720=CARTESIAN_POINT ( 'NONE',  ( 13.95806775979394487, 15.00000000000000888, 4.371577651620829563 ) ) ;
#93731=CARTESIAN_POINT ( 'NONE',  ( -14.04391541078765826, 15.00000000000000000, 3.608107528142729503 ) ) ;
#93732=ORIENTED_EDGE ( 'NONE', *, *, #26045, .T. ) ;
#93734=VERTEX_POINT ( 'NONE', #67481 ) ;
#93741=CARTESIAN_POINT ( 'NONE',  ( 0.000000000000000000, 15.00000000000000000, 0.000000000000000000 ) ) ;
#93742=VECTOR ( 'NONE', #50611, 1000.000000000000227 ) ;
#93743=CARTESIAN_POINT ( 'NONE',  ( -11.09922568453594316, -5.459698663402908103, 6.408140936763246920 ) ) ;
#93748=AXIS2_PLACEMENT_3D ( 'NONE', #86735, #8277, #38775 ) ;
#93759=CARTESIAN_POINT ( 'NONE',  ( 1.326261724322855828, 0.2301504087165518186, 14.88164196614421186 ) ) ;
#93761=CARTESIAN_POINT ( 'NONE',  ( 9.240973841163532043, 4.236086333263440692E-16, 11.17382667070378943 ) ) ;
#93765=DIRECTION ( 'NONE',  ( -0.7372773368101205316, 0.000000000000000000, -0.6755902076156641289 ) ) ;
#93768=DIRECTION ( 'NONE',  ( -0.000000000000000000, -1.000000000000000000, -0.000000000000000000 ) ) ;
#93772=CARTESIAN_POINT ( 'NONE',  ( 14.42956166533735640, -2.687212025164267037E-15, 2.386684097925098502 ) ) ;
#93773=DIRECTION ( 'NONE',  ( -0.000000000000000000, -1.000000000000000000, -0.000000000000000000 ) ) ;
#93784=ADVANCED_FACE ( 'NONE', ( #8810 ), #40527, .T. ) ;
#93802=ORIENTED_EDGE ( 'NONE', *, *, #9899, .F. ) ;
#93804=EDGE_CURVE ( 'NONE', #37334, #56877, #61781, .T. ) ;
#93809=CARTESIAN_POINT ( 'NONE',  ( 3.420591144908454950, 14.63595249122788999, 14.60477854057959490 ) ) ;
#93814=ORIENTED_EDGE ( 'NONE', *, *, #63242, .T. ) ;
#93816=CARTESIAN_POINT ( 'NONE',  ( 2.815433093577111467, 14.49999999999999112, -14.73340885523756683 ) ) ;
#93831=VECTOR ( 'NONE', #2188, 1000.000000000000114 ) ;
#93832=AXIS2_PLACEMENT_3D ( 'NONE', #24012, #98557, #84509 ) ;
#93846=EDGE_CURVE ( 'NONE', #67150, #41155, #9854, .T. ) ;
#93858=DIRECTION ( 'NONE',  ( 0.000000000000000000, 0.000000000000000000, 1.000000000000000000 ) ) ;
#93879=ORIENTED_EDGE ( 'NONE', *, *, #88542, .T. ) ;
#93882=ORIENTED_EDGE ( 'NONE', *, *, #71711, .T. ) ;
#93883=DIRECTION ( 'NONE',  ( -0.8616291604415338146, -0.000000000000000000, 0.5075383629606904368 ) ) ;
#93890=CARTESIAN_POINT ( 'NONE',  ( -1.881645754503963541, -3.304699043712651590E-15, 14.50406564081095162 ) ) ;
#93893=LINE ( 'NONE', #25420, #32484 ) ;
#93899=ORIENTED_EDGE ( 'NONE', *, *, #4880, .T. ) ;
#93900=CIRCLE ( 'NONE', #55584, 15.00000000000000000 ) ;
#93914=CARTESIAN_POINT ( 'NONE',  ( -9.898881779040587858, -0.03417435944610275333, -10.25059215482589714 ) ) ;
#93918=B_SPLINE_CURVE_WITH_KNOTS ( 'NONE', 3,
 ( #88598, #20109, #50612, #94138, #4141, #11135 ),
 .UNSPECIFIED., .F., .F.,
 ( 4, 2, 4 ),
 ( 0.0002800484630363999933, 0.0006862541666483234701, 0.001092459870260246947 ),
 .UNSPECIFIED. ) ;
#93921=DIRECTION ( 'NONE',  ( -0.000000000000000000, -1.000000000000000000, -0.000000000000000000 ) ) ;
#93922=CYLINDRICAL_SURFACE ( 'NONE', #44893, 15.00000000000000000 ) ;
#93924=LINE ( 'NONE', #25450, #52217 ) ;
#93925=CARTESIAN_POINT ( 'NONE',  ( 12.26659068614894821, 8.887082168247301794, 7.082119434687044190 ) ) ;
#93931=EDGE_CURVE ( 'NONE', #12953, #48484, #38552, .T. ) ;
#93932=EDGE_CURVE ( 'NONE', #97330, #9538, #30877, .T. ) ;
#93933=CARTESIAN_POINT ( 'NONE',  ( -6.382347221874242749, 0.5000000000000004441, -13.57444820018235987 ) ) ;
#93961=DIRECTION ( 'NONE',  ( -0.000000000000000000, -1.000000000000000000, -0.000000000000000000 ) ) ;
#93962=ORIENTED_EDGE ( 'NONE', *, *, #75438, .F. ) ;
#93976=CARTESIAN_POINT ( 'NONE',  ( 0.000000000000000000, 0.000000000000000000, 0.000000000000000000 ) ) ;
#93977=AXIS2_PLACEMENT_3D ( 'NONE', #37059, #90042, #51057 ) ;
#93983=CARTESIAN_POINT ( 'NONE',  ( 13.78891971893204804, 0.3640475087720924097, 5.904717858191625979 ) ) ;
#93992=CARTESIAN_POINT ( 'NONE',  ( 8.527530157486175710, 23.92559781766745530, -4.923371831947298993 ) ) ;
#93994=CARTESIAN_POINT ( 'NONE',  ( -8.564643372776448160, 15.00000000000000000, -12.31449893000752205 ) ) ;
#94001=CARTESIAN_POINT ( 'NONE',  ( -14.73513795193453824, 0.04922511925147073086, -0.7223639599948814549 ) ) ;
#94009=CIRCLE ( 'NONE', #22148, 15.00000000000000000 ) ;
#94013=EDGE_CURVE ( 'NONE', #97221, #77130, #38893, .T. ) ;
#94015=( LENGTH_UNIT ( ) NAMED_UNIT ( * ) SI_UNIT ( .MILLI., .METRE. ) );
#94018=ORIENTED_EDGE ( 'NONE', *, *, #37137, .F. ) ;
#94019=DIRECTION ( 'NONE',  ( 0.9832549075639562819, 0.000000000000000000, -0.1822355254921381451 ) ) ;
#94022=CARTESIAN_POINT ( 'NONE',  ( 11.35178980618980304, 14.49999999999999112, -9.804941009311946232 ) ) ;
#94027=B_SPLINE_CURVE_WITH_KNOTS ( 'NONE', 3,
 ( #97282, #49776, #19775, #58758 ),
 .UNSPECIFIED., .F., .F.,
 ( 4, 4 ),
 ( 2.070562745361082850E-16, 0.003685997162761518991 ),
 .UNSPECIFIED. ) ;
#94043=EDGE_CURVE ( 'NONE', #9024, #60175, #3843, .T. ) ;
#94046=EDGE_CURVE ( 'NONE', #39776, #31701, #64384, .T. ) ;
#94057=CARTESIAN_POINT ( 'NONE',  ( -5.440088680355558814, 7.230352010821512465, -9.422509992056136596 ) ) ;
#94063=CARTESIAN_POINT ( 'NONE',  ( 11.22915323889580463, -0.03417435944610275333, -8.773176023390609757 ) ) ;
#94066=CARTESIAN_POINT ( 'NONE',  ( 8.157527544166590872, 14.76984925469195886, -12.51706795611453593 ) ) ;
#94067=CARTESIAN_POINT ( 'NONE',  ( 11.92686044187656336, 11.97997603579417891, 3.195792623639526653 ) ) ;
#94080=EDGE_CURVE ( 'NONE', #58432, #54272, #73048, .T. ) ;
#94087=LINE ( 'NONE', #49078, #96931 ) ;
#94089=DIRECTION ( 'NONE',  ( 0.000000000000000000, 0.000000000000000000, 1.000000000000000000 ) ) ;
#94101=CARTESIAN_POINT ( 'NONE',  ( -4.923371831947302546, -9.824402182332548250, -8.527530157486173934 ) ) ;
#94104=ORIENTED_EDGE ( 'NONE', *, *, #40008, .F. ) ;
#94116=ORIENTED_EDGE ( 'NONE', *, *, #79248, .T. ) ;
#94120=VECTOR ( 'NONE', #20702, 1000.000000000000000 ) ;
#94125=EDGE_CURVE ( 'NONE', #70377, #58998, #14756, .T. ) ;
#94128=DIRECTION ( 'NONE',  ( 0.000000000000000000, 1.000000000000000000, 0.000000000000000000 ) ) ;
#94129=VERTEX_POINT ( 'NONE', #68720 ) ;
#94132=CARTESIAN_POINT ( 'NONE',  ( -14.49120296996854940, 0.04922511925147123046, -2.766068805437723377 ) ) ;
#94134=LINE ( 'NONE', #55147, #93831 ) ;
#94138=CARTESIAN_POINT ( 'NONE',  ( -3.384479038598111167, 0.2301507000107681222, -14.55223509985382435 ) ) ;
#94140=DIRECTION ( 'NONE',  ( 0.000000000000000000, 1.000000000000000000, 0.000000000000000000 ) ) ;
#94141=ORIENTED_EDGE ( 'NONE', *, *, #85796, .F. ) ;
#94142=CARTESIAN_POINT ( 'NONE',  ( 5.817157072110804350, 14.49999999999999112, -13.82608706751093663 ) ) ;
#94150=CARTESIAN_POINT ( 'NONE',  ( 12.67147417979171031, 14.95037112956503655, 7.555862176155596188 ) ) ;
#94151=EDGE_CURVE ( 'NONE', #27398, #87174, #60710, .T. ) ;
#94152=ORIENTED_EDGE ( 'NONE', *, *, #80380, .T. ) ;
#94155=DIRECTION ( 'NONE',  ( 0.000000000000000000, 0.000000000000000000, 1.000000000000000000 ) ) ;
#94158=CARTESIAN_POINT ( 'NONE',  ( 10.00676502675680446, 12.82908929790087527, -5.835523404638878198 ) ) ;
#94159=CARTESIAN_POINT ( 'NONE',  ( 10.93781366033348768, 0.3639309795253655722, -10.26470809774068371 ) ) ;
#94160=DIRECTION ( 'NONE',  ( -0.000000000000000000, -1.000000000000000000, -0.000000000000000000 ) ) ;
#94161=CARTESIAN_POINT ( 'NONE',  ( -12.80781515976305762, -0.03417435944610275333, -6.246788841744501219 ) ) ;
#94163=CARTESIAN_POINT ( 'NONE',  ( 9.422509992056141925, -34.85298132251183034, 5.440088680355547268 ) ) ;
#94166=CARTESIAN_POINT ( 'NONE',  ( -11.22915323889568562, -0.03417435944610275333, -8.773176023390764300 ) ) ;
#94178=CARTESIAN_POINT ( 'NONE',  ( -14.04867373755345561, 15.00000000000000000, -7.649324326489842285 ) ) ;
#94184=ORIENTED_EDGE ( 'NONE', *, *, #76649, .F. ) ;
#94193=AXIS2_PLACEMENT_3D ( 'NONE', #73817, #11354, #57342 ) ;
#94198=ORIENTED_EDGE ( 'NONE', *, *, #46213, .T. ) ;
#94217=ORIENTED_EDGE ( 'NONE', *, *, #60315, .T. ) ;
#94219=EDGE_LOOP ( 'NONE', ( #26225, #19079, #31748, #84164 ) ) ;
#94227=CARTESIAN_POINT ( 'NONE',  ( -12.81628187352647252, -0.6680319967362452482, 3.434112377981066722 ) ) ;
#94236=CARTESIAN_POINT ( 'NONE',  ( 14.40939250469966026, 4.578996266948430760E-16, -1.618458416365756714 ) ) ;
#94241=CIRCLE ( 'NONE', #6460, 14.49999999999999822 ) ;
#94248=TOROIDAL_SURFACE ( 'NONE', #68714, 14.49999999999999822, 0.5000000000000000000 ) ;
#94249=CARTESIAN_POINT ( 'NONE',  ( 11.62006642627357778, -3.022637072276969577E-15, 8.881585844847220912 ) ) ;
#94261=CARTESIAN_POINT ( 'NONE',  ( 4.850097797904172836, 14.95037102666663920, 13.93319274793806173 ) ) ;
#94266=( NAMED_UNIT ( * ) PLANE_ANGLE_UNIT ( ) SI_UNIT ( $, .RADIAN. ) );
#94267=CARTESIAN_POINT ( 'NONE',  ( -14.04391541078765826, 15.00000000000000000, 3.608107528142729503 ) ) ;
#94274=DIRECTION ( 'NONE',  ( 0.000000000000000000, 0.000000000000000000, 1.000000000000000000 ) ) ;
#94278=CIRCLE ( 'NONE', #38421, 11.92686044187656513 ) ;
#94285=CARTESIAN_POINT ( 'NONE',  ( 0.000000000000000000, 0.5000000000000004441, 0.000000000000000000 ) ) ;
#94288=DIRECTION ( 'NONE',  ( 0.9426414910921783186, 0.000000000000000000, -0.3338068592337714025 ) ) ;
#94292=CARTESIAN_POINT ( 'NONE',  ( 2.393480905993150998, 0.5000000000000004441, -14.80781041047751323 ) ) ;
#94296=DIRECTION ( 'NONE',  ( 0.000000000000000000, 0.000000000000000000, 1.000000000000000000 ) ) ;
#94306=EDGE_CURVE ( 'NONE', #87326, #42998, #57223, .T. ) ;
#94311=CARTESIAN_POINT ( 'NONE',  ( -12.00809552683971759, 14.49999999999999112, 8.989195838243478676 ) ) ;
#94337=ORIENTED_EDGE ( 'NONE', *, *, #77886, .T. ) ;
#94343=EDGE_LOOP ( 'NONE', ( #45052, #10710, #24389, #91591 ) ) ;
#94354=ORIENTED_EDGE ( 'NONE', *, *, #39176, .F. ) ;
#94356=EDGE_LOOP ( 'NONE', ( #89196, #22036 ) ) ;
#94360=CARTESIAN_POINT ( 'NONE',  ( 5.991992585808519678, 15.00000000000000000, 13.20401548210297271 ) ) ;
#94363=EDGE_CURVE ( 'NONE', #54280, #83059, #74107, .T. ) ;
#94364=VECTOR ( 'NONE', #41453, 1000.000000000000000 ) ;
#94368=ORIENTED_EDGE ( 'NONE', *, *, #61317, .T. ) ;
#94371=ORIENTED_EDGE ( 'NONE', *, *, #47675, .F. ) ;
#94372=CARTESIAN_POINT ( 'NONE',  ( -1.983216688680738082, -0.03417435944610275333, -14.11131997956740491 ) ) ;
#94382=CARTESIAN_POINT ( 'NONE',  ( 0.000000000000000000, 14.49999999999999822, 0.000000000000000000 ) ) ;
#94385=AXIS2_PLACEMENT_3D ( 'NONE', #36, #30978, #30482 ) ;
#94392=CIRCLE ( 'NONE', #86502, 14.49999999999999822 ) ;
#94393=CARTESIAN_POINT ( 'NONE',  ( -13.07751017358212131, 15.00000000000000000, 6.263284095430918796 ) ) ;
#94394=EDGE_CURVE ( 'NONE', #48509, #27622, #78906, .T. ) ;
#94401=B_SPLINE_CURVE_WITH_KNOTS ( 'NONE', 3,
 ( #28658, #5679, #66665, #36667, #97190, #6653 ),
 .UNSPECIFIED., .F., .F.,
 ( 4, 2, 4 ),
 ( 3.409110551495797298E-05, 0.0004400426677367831022, 0.0008459942299586082314 ),
 .UNSPECIFIED. ) ;
#94403=CARTESIAN_POINT ( 'NONE',  ( -13.59972906620404487, 0.04962881387626322943, 5.718800721548481292 ) ) ;
#94405=ORIENTED_EDGE ( 'NONE', *, *, #54300, .T. ) ;
#94407=CARTESIAN_POINT ( 'NONE',  ( -12.21130863673195499, -2.649095542537823522E-15, -8.049375889233145287 ) ) ;
#94410=CARTESIAN_POINT ( 'NONE',  ( -7.082119434687058401, 5.970415501580637496, -12.26659068614894110 ) ) ;
#94415=PLANE ( 'NONE',  #19870 ) ;
#94419=CARTESIAN_POINT ( 'NONE',  ( 11.10175276307597336, 14.95037105032437807, -9.716398248524681591 ) ) ;
#94421=CARTESIAN_POINT ( 'NONE',  ( 10.27191093752563411, 9.181837148236613703E-16, -10.41278984915626360 ) ) ;
#94426=CARTESIAN_POINT ( 'NONE',  ( 3.420591144908446957, 0.5000000000000004441, 14.60477854057958425 ) ) ;
#94433=VERTEX_POINT ( 'NONE', #1714 ) ;
#94436=ADVANCED_FACE ( 'NONE', ( #62674 ), #72473, .T. ) ;
#94453=VERTEX_POINT ( 'NONE', #25687 ) ;
#94457=AXIS2_PLACEMENT_3D ( 'NONE', #32568, #95033, #70091 ) ;
#94458=VERTEX_POINT ( 'NONE', #39708 ) ;
#94459=CARTESIAN_POINT ( 'NONE',  ( 6.898461952320324109, 15.00000000000000000, 12.75387089053312373 ) ) ;
#94472=EDGE_CURVE ( 'NONE', #33681, #87486, #49156, .T. ) ;
#94473=DIRECTION ( 'NONE',  ( -0.000000000000000000, -1.000000000000000000, -0.000000000000000000 ) ) ;
#94475=CARTESIAN_POINT ( 'NONE',  ( 12.81628187352647608, -38.37636533006957507, -2.602085213965210642E-15 ) ) ;
#94476=ORIENTED_EDGE ( 'NONE', *, *, #75080, .T. ) ;
#94477=VECTOR ( 'NONE', #46557, 1000.000000000000000 ) ;
#94485=EDGE_CURVE ( 'NONE', #25245, #38271, #32171, .T. ) ;
#94488=VERTEX_POINT ( 'NONE', #79659 ) ;
#94491=ORIENTED_EDGE ( 'NONE', *, *, #58344, .T. ) ;
#94494=CARTESIAN_POINT ( 'NONE',  ( 3.195792623639591490, 6.146642702460846763, 11.92686044187652961 ) ) ;
#94499=CARTESIAN_POINT ( 'NONE',  ( 5.302565485995492267, 0.000000000000000000, -1.273033341818833541 ) ) ;
#94503=AXIS2_PLACEMENT_3D ( 'NONE', #2760, #33213, #74158 ) ;
#94504=CARTESIAN_POINT ( 'NONE',  ( 14.62617646268085281, 0.5000000000000004441, 3.327906561566980503 ) ) ;
#94512=ADVANCED_FACE ( 'NONE', ( #11155 ), #86672, .F. ) ;
#94515=DIRECTION ( 'NONE',  ( 0.000000000000000000, 0.000000000000000000, -1.000000000000000000 ) ) ;
#94525=CARTESIAN_POINT ( 'NONE',  ( 8.439016546559892973, 15.00000000000000000, -11.79122553964970876 ) ) ;
#94528=CARTESIAN_POINT ( 'NONE',  ( -7.082119434687044190, -37.36291783175269643, 12.26659068614894998 ) ) ;
#94532=ORIENTED_EDGE ( 'NONE', *, *, #85438, .T. ) ;
#94539=PLANE ( 'NONE',  #12922 ) ;
#94544=CARTESIAN_POINT ( 'NONE',  ( 9.422509992056141925, 10.98035201082150891, -5.440088680355554374 ) ) ;
#94549=CYLINDRICAL_SURFACE ( 'NONE', #91249, 15.00000000000000000 ) ;
#94550=EDGE_CURVE ( 'NONE', #8774, #95706, #60059, .T. ) ;
#94551=FACE_OUTER_BOUND ( 'NONE', #92406, .T. ) ;
#94554=CARTESIAN_POINT ( 'NONE',  ( 15.61289147378509057, 15.00000000000000000, 3.480663193108788800 ) ) ;
#94563=VERTEX_POINT ( 'NONE', #10672 ) ;
#94572=DIRECTION ( 'NONE',  ( 0.2334453638559156052, 0.000000000000000000, -0.9723699203976741146 ) ) ;
#94577=ORIENTED_EDGE ( 'NONE', *, *, #88643, .F. ) ;
#94579=AXIS2_PLACEMENT_3D ( 'NONE', #2907, #48373, #26853 ) ;
#94592=CARTESIAN_POINT ( 'NONE',  ( -8.527530157486182816, 5.592264484334121377, -4.923371831947288335 ) ) ;
#94597=EDGE_CURVE ( 'NONE', #58863, #1208, #27713, .T. ) ;
#94598=ORIENTED_EDGE ( 'NONE', *, *, #18765, .T. ) ;
#94603=CARTESIAN_POINT ( 'NONE',  ( -9.876730923139412255, 14.63606899087332636, 11.28938378619058547 ) ) ;
#94604=AXIS2_PLACEMENT_3D ( 'NONE', #81596, #74596, #90579 ) ;
#94605=EDGE_CURVE ( 'NONE', #27759, #56243, #85198, .T. ) ;
#94611=ORIENTED_EDGE ( 'NONE', *, *, #38673, .T. ) ;
#94612=AXIS2_PLACEMENT_3D ( 'NONE', #16904, #54387, #84899 ) ;
#94622=DIRECTION ( 'NONE',  ( 0.000000000000000000, 0.000000000000000000, 1.000000000000000000 ) ) ;
#94625=ORIENTED_EDGE ( 'NONE', *, *, #37970, .T. ) ;
#94631=CARTESIAN_POINT ( 'NONE',  ( 10.14667048435145169, 15.00000000000000000, -10.35833375027041292 ) ) ;
#94634=CARTESIAN_POINT ( 'NONE',  ( 8.157527544166429223, 0.2301507453079258969, 12.51706795611453593 ) ) ;
#94638=ORIENTED_EDGE ( 'NONE', *, *, #59300, .F. ) ;
#94639=LINE ( 'NONE', #19135, #19281 ) ;
#94651=FACE_OUTER_BOUND ( 'NONE', #68191, .T. ) ;
#94656=CARTESIAN_POINT ( 'NONE',  ( 13.61464873478162829, 14.49999999999999822, 6.296136897217933459 ) ) ;
#94660=CARTESIAN_POINT ( 'NONE',  ( -2.915334737309934532, -37.97798132251182324, -10.88017736071109987 ) ) ;
#94664=CARTESIAN_POINT ( 'NONE',  ( 8.564643372776536978, 0.5000000000000004441, 12.31449893000746343 ) ) ;
#94665=DIRECTION ( 'NONE',  ( 0.3173046564051031360, 0.000000000000000000, -0.9483236552061955482 ) ) ;
#94677=DIRECTION ( 'NONE',  ( -0.1822355254921381451, 0.000000000000000000, -0.9832549075639562819 ) ) ;
#94685=CARTESIAN_POINT ( 'NONE',  ( -14.71525861348285957, 15.00000000000000000, -2.908807992686776700 ) ) ;
#94694=AXIS2_PLACEMENT_3D ( 'NONE', #81041, #29016, #59526 ) ;
#94695=FACE_OUTER_BOUND ( 'NONE', #9219, .T. ) ;
#94697=EDGE_CURVE ( 'NONE', #89452, #46043, #37391, .T. ) ;
#94698=VERTEX_POINT ( 'NONE', #35632 ) ;
#94700=ORIENTED_EDGE ( 'NONE', *, *, #94485, .T. ) ;
#94701=VERTEX_POINT ( 'NONE', #57143 ) ;
#94702=CARTESIAN_POINT ( 'NONE',  ( -5.204170427930421283E-15, 11.67180217785154817, -11.25000000000000178 ) ) ;
#94716=ORIENTED_EDGE ( 'NONE', *, *, #56594, .F. ) ;
#94720=ORIENTED_EDGE ( 'NONE', *, *, #54069, .F. ) ;
#94728=CARTESIAN_POINT ( 'NONE',  ( -12.81628187352647963, -11.08469866340290899, -3.434112377981046293 ) ) ;
#94729=ADVANCED_FACE ( 'NONE', ( #66117 ), #64626, .F. ) ;
#94741=DIRECTION ( 'NONE',  ( -0.9588197348681908316, 0.000000000000000000, -0.2840153447039300283 ) ) ;
#94742=CARTESIAN_POINT ( 'NONE',  ( -14.94699059465106572, 14.63606911935818289, 1.259949270174702818 ) ) ;
#94746=AXIS2_PLACEMENT_3D ( 'NONE', #77651, #24183, #90689 ) ;
#94748=AXIS2_PLACEMENT_3D ( 'NONE', #44132, #42673, #46010 ) ;
#94754=VECTOR ( 'NONE', #73224, 1000.000000000000000 ) ;
#94756=CARTESIAN_POINT ( 'NONE',  ( 14.56372689393328734, 0.04962896412619403896, 2.356940382833113024 ) ) ;
#94760=CARTESIAN_POINT ( 'NONE',  ( 9.520529577030492518, 2.507217523872729004E-16, -11.10395710204420716 ) ) ;
#94767=ORIENTED_EDGE ( 'NONE', *, *, #389, .F. ) ;
#94786=CARTESIAN_POINT ( 'NONE',  ( -6.741983435833607707, 14.95077488074853456, 13.12218577464082614 ) ) ;
#94794=ORIENTED_EDGE ( 'NONE', *, *, #78519, .F. ) ;
#94802=CARTESIAN_POINT ( 'NONE',  ( -13.07751017357375112, 4.831904710033835254E-16, -6.263284095430687870 ) ) ;
#94831=CARTESIAN_POINT ( 'NONE',  ( 3.243710765982298128, 0.000000000000000000, 4.383623511354910463 ) ) ;
#94833=ORIENTED_EDGE ( 'NONE', *, *, #934, .T. ) ;
#94836=EDGE_CURVE ( 'NONE', #52439, #65339, #86897, .T. ) ;
#94849=CARTESIAN_POINT ( 'NONE',  ( 0.000000000000000000, 15.00000000000000000, 0.000000000000000000 ) ) ;
#94863=CARTESIAN_POINT ( 'NONE',  ( 1.983216688680843109, -0.03417435944610275333, 14.11131997956739070 ) ) ;
#94869=LINE ( 'NONE', #71875, #40905 ) ;
#94871=CARTESIAN_POINT ( 'NONE',  ( 14.29541133317244217, 0.2306972965111902807, -4.345028136609535352 ) ) ;
#94883=CARTESIAN_POINT ( 'NONE',  ( 3.469446951953614189E-15, 6.368033628982654903, 11.25000000000000178 ) ) ;
#94901=CARTESIAN_POINT ( 'NONE',  ( -10.36894250292379205, 1.178748834913966315, -10.36894250292378672 ) ) ;
#94906=CARTESIAN_POINT ( 'NONE',  ( -14.91937968691865990, 14.76930270348881535, 0.8063277559917156889 ) ) ;
#94911=CARTESIAN_POINT ( 'NONE',  ( -7.313705784284425526, 14.63595249122788999, -13.09617149020754034 ) ) ;
#94918=DIRECTION ( 'NONE',  ( -0.000000000000000000, -1.000000000000000000, -0.000000000000000000 ) ) ;
#94925=EDGE_LOOP ( 'NONE', ( #62591, #95710, #86427, #92065 ) ) ;
#94926=AXIS2_PLACEMENT_3D ( 'NONE', #91760, #51292, #81777 ) ;
#94928=EDGE_CURVE ( 'NONE', #36109, #88333, #66624, .T. ) ;
#94935=VERTEX_POINT ( 'NONE', #51631 ) ;
#94937=CARTESIAN_POINT ( 'NONE',  ( 0.000000000000000000, 0.5000000000000004441, 0.000000000000000000 ) ) ;
#94944=ORIENTED_EDGE ( 'NONE', *, *, #63163, .F. ) ;
#94947=CARTESIAN_POINT ( 'NONE',  ( -5.419894505350392855, 14.49999999999999822, -13.98659156302466045 ) ) ;
#94948=ORIENTED_EDGE ( 'NONE', *, *, #65210, .F. ) ;
#94954=DIRECTION ( 'NONE',  ( -0.000000000000000000, -1.000000000000000000, -0.000000000000000000 ) ) ;
#94964=CARTESIAN_POINT ( 'NONE',  ( 11.09922568453594671, -37.95969866340291077, -6.408140936763241591 ) ) ;
#94975=VECTOR ( 'NONE', #392, 1000.000000000000114 ) ;
#94977=VERTEX_POINT ( 'NONE', #83608 ) ;
#94982=CARTESIAN_POINT ( 'NONE',  ( 10.14667048435135577, 15.00000000000000000, 10.35833375027046976 ) ) ;
#94988=EDGE_CURVE ( 'NONE', #70649, #33114, #75604, .T. ) ;
#94999=CARTESIAN_POINT ( 'NONE',  ( 0.000000000000000000, 0.5000000000000004441, 0.000000000000000000 ) ) ;
#95013=CARTESIAN_POINT ( 'NONE',  ( 3.795296366450314540, -36.73791783175269643, 14.16423886937410082 ) ) ;
#95024=CARTESIAN_POINT ( 'NONE',  ( -14.52844422123737012, 14.99999999999803713, -1.683098224411851307 ) ) ;
#95030=CARTESIAN_POINT ( 'NONE',  ( 9.422509992056141925, 10.14701867748817676, 5.440088680355547268 ) ) ;
#95033=DIRECTION ( 'NONE',  ( 0.000000000000000000, 1.000000000000000000, 0.000000000000000000 ) ) ;
#95034=ADVANCED_FACE ( 'NONE', ( #67116 ), #75107, .T. ) ;
#95039=CIRCLE ( 'NONE', #29580, 15.00000000000000000 ) ;
#95048=ORIENTED_EDGE ( 'NONE', *, *, #85248, .T. ) ;
#95056=CARTESIAN_POINT ( 'NONE',  ( -8.502721643905040594, 14.95037103750416563, -12.05657636697581658 ) ) ;
#95058=EDGE_CURVE ( 'NONE', #37334, #5292, #6613, .T. ) ;
#95059=AXIS2_PLACEMENT_3D ( 'NONE', #7356, #46810, #60338 ) ;
#95062=ORIENTED_EDGE ( 'NONE', *, *, #43644, .F. ) ;
#95067=EDGE_CURVE ( 'NONE', #12737, #325, #95847, .T. ) ;
#95070=CARTESIAN_POINT ( 'NONE',  ( 10.58521204051726627, -0.03417435944610275333, 11.99294302885416563 ) ) ;
#95074=DIRECTION ( 'NONE',  ( 0.000000000000000000, 1.000000000000000000, -0.000000000000000000 ) ) ;
#95077=CARTESIAN_POINT ( 'NONE',  ( 4.923371831947301658, 2.675597817667456191, 8.527530157486175710 ) ) ;
#95082=ORIENTED_EDGE ( 'NONE', *, *, #69435, .F. ) ;
#95087=CIRCLE ( 'NONE', #40864, 15.00000000000000000 ) ;
#95091=EDGE_LOOP ( 'NONE', ( #35475, #32236, #83559, #21084, #93012, #29098 ) ) ;
#95093=ORIENTED_EDGE ( 'NONE', *, *, #7658, .F. ) ;
#95102=CARTESIAN_POINT ( 'NONE',  ( -5.991992585808714189, 4.061121054423934144E-16, 13.20401548210291054 ) ) ;
#95103=VECTOR ( 'NONE', #83106, 1000.000000000000000 ) ;
#95105=ORIENTED_EDGE ( 'NONE', *, *, #18604, .T. ) ;
#95110=CARTESIAN_POINT ( 'NONE',  ( -5.204170427930421283E-15, 11.41212336850781739, -11.92686044187656513 ) ) ;
#95111=ORIENTED_EDGE ( 'NONE', *, *, #57106, .T. ) ;
#95112=DIRECTION ( 'NONE',  ( 0.000000000000000000, -1.000000000000000000, 0.000000000000000000 ) ) ;
#95117=ORIENTED_EDGE ( 'NONE', *, *, #65020, .F. ) ;
#95121=CIRCLE ( 'NONE', #32823, 14.49999999999999822 ) ;
#95127=CARTESIAN_POINT ( 'NONE',  ( 0.7166339456633684657, 0.000000000000000000, -15.98010739087745868 ) ) ;
#95128=ORIENTED_EDGE ( 'NONE', *, *, #54940, .F. ) ;
#95136=CARTESIAN_POINT ( 'NONE',  ( 9.011287250621787592, 0.2306972965111906138, -11.91783356064788535 ) ) ;
#95139=CARTESIAN_POINT ( 'NONE',  ( -2.915334737309934532, -22.97798132251182324, -10.88017736071109987 ) ) ;
#95141=CARTESIAN_POINT ( 'NONE',  ( -14.16722289976693894, 14.49999999999999112, 4.928467845925465163 ) ) ;
#95142=EDGE_CURVE ( 'NONE', #54039, #4498, #88637, .T. ) ;
#95144=CARTESIAN_POINT ( 'NONE',  ( 8.549892366338765370, 0.2306972965111890594, 12.25305656628361106 ) ) ;
#95145=CARTESIAN_POINT ( 'NONE',  ( -10.17177286909455525, 14.76984972048479783, -10.94336654633696604 ) ) ;
#95153=ADVANCED_FACE ( 'NONE', ( #68607 ), #84594, .F. ) ;
#95158=PLANE ( 'NONE',  #82292 ) ;
#95159=TOROIDAL_SURFACE ( 'NONE', #74389, 14.49999999999999822, 0.5000000000000000000 ) ;
#95164=VERTEX_POINT ( 'NONE', #36632 ) ;
#95175=ORIENTED_EDGE ( 'NONE', *, *, #63531, .F. ) ;
#95176=CARTESIAN_POINT ( 'NONE',  ( 12.34086200392826882, 15.00000000000000000, -7.124999999999971578 ) ) ;
#95178=ORIENTED_EDGE ( 'NONE', *, *, #13361, .T. ) ;
#95191=DIRECTION ( 'NONE',  ( 0.1305261922200583458, 0.000000000000000000, -0.9914448613738096050 ) ) ;
#95195=CARTESIAN_POINT ( 'NONE',  ( 14.03351048042397231, -0.03417435944610275333, -2.474486531753715024 ) ) ;
#95197=DIRECTION ( 'NONE',  ( 0.000000000000000000, 0.000000000000000000, 1.000000000000000000 ) ) ;
#95198=ORIENTED_EDGE ( 'NONE', *, *, #89735, .T. ) ;
#95200=EDGE_LOOP ( 'NONE', ( #48958, #49670, #39048, #50340 ) ) ;
#95205=EDGE_CURVE ( 'NONE', #53280, #73183, #72539, .T. ) ;
#95209=CARTESIAN_POINT ( 'NONE',  ( 11.09922568453594671, 7.040301336597089232, -6.408140936763241591 ) ) ;
#95213=VERTEX_POINT ( 'NONE', #17582 ) ;
#95214=EDGE_LOOP ( 'NONE', ( #63946, #3160, #58716, #10580 ) ) ;
#95219=CARTESIAN_POINT ( 'NONE',  ( 12.83294900548062678, 14.49999999999999112, 7.766300266068507874 ) ) ;
#95226=CARTESIAN_POINT ( 'NONE',  ( 13.48255862861923937, 4.031870098369226268E-16, 5.335786055104250636 ) ) ;
#95232=DIRECTION ( 'NONE',  ( -0.000000000000000000, -1.000000000000000000, -0.000000000000000000 ) ) ;
#95236=DIRECTION ( 'NONE',  ( -0.5664062369248369366, 0.000000000000000000, 0.8241261886220128119 ) ) ;
#95246=VECTOR ( 'NONE', #64960, 1000.000000000000227 ) ;
#95251=AXIS2_PLACEMENT_3D ( 'NONE', #50622, #81113, #66610 ) ;
#95253=ORIENTED_EDGE ( 'NONE', *, *, #81629, .F. ) ;
#95267=CARTESIAN_POINT ( 'NONE',  ( 12.50534872682727539, 3.894361491432412218E-16, 7.339363270777609749 ) ) ;
#95268=CARTESIAN_POINT ( 'NONE',  ( -12.21238578215998771, 15.00000000000000888, -8.049595036947295057 ) ) ;
#95279=FACE_OUTER_BOUND ( 'NONE', #39721, .T. ) ;
#95293=CARTESIAN_POINT ( 'NONE',  ( -1.983216688681034068, -0.03417435944610275333, 14.11131997956736406 ) ) ;
#95298=CARTESIAN_POINT ( 'NONE',  ( -4.547378612396732578, 0.000000000000000000, -3.009844244835570670 ) ) ;
#95304=DIRECTION ( 'NONE',  ( 0.000000000000000000, 0.000000000000000000, 1.000000000000000000 ) ) ;
#95310=DIRECTION ( 'NONE',  ( 0.000000000000000000, 1.000000000000000000, 0.000000000000000000 ) ) ;
#95316=CARTESIAN_POINT ( 'NONE',  ( 1.457314710996481688, 0.000000000000000000, 5.254907083456974881 ) ) ;
#95321=VERTEX_POINT ( 'NONE', #93556 ) ;
#95328=ORIENTED_EDGE ( 'NONE', *, *, #78614, .T. ) ;
#95333=DIRECTION ( 'NONE',  ( 0.000000000000000000, 0.000000000000000000, 1.000000000000000000 ) ) ;
#95341=EDGE_LOOP ( 'NONE', ( #57671, #56767, #65545, #66060 ) ) ;
#95342=FACE_OUTER_BOUND ( 'NONE', #41142, .T. ) ;
#95348=CARTESIAN_POINT ( 'NONE',  ( -14.02068044289372395, 14.63595249122790598, -5.331089937175856441 ) ) ;
#95351=ORIENTED_EDGE ( 'NONE', *, *, #37719, .T. ) ;
#95354=CARTESIAN_POINT ( 'NONE',  ( 0.000000000000000000, 0.5000000000000004441, 0.000000000000000000 ) ) ;
#95359=ORIENTED_EDGE ( 'NONE', *, *, #97466, .F. ) ;
#95366=DIRECTION ( 'NONE',  ( 0.000000000000000000, 1.000000000000000000, 0.000000000000000000 ) ) ;
#95367=CARTESIAN_POINT ( 'NONE',  ( 0.9082943533637201083, 4.650128654361622927E-16, -14.47152380945585115 ) ) ;
#95373=ORIENTED_EDGE ( 'NONE', *, *, #22531, .F. ) ;
#95375=CARTESIAN_POINT ( 'NONE',  ( -0.3093388210927633941, 14.49999999999999822, -14.99680997725065978 ) ) ;
#95383=CARTESIAN_POINT ( 'NONE',  ( -6.689969769699040114, 0.000000000000000000, 12.58200319823965785 ) ) ;
#95388=CARTESIAN_POINT ( 'NONE',  ( 12.21130863673206157, 15.00000000000000533, -8.049375889232978309 ) ) ;
#95390=CARTESIAN_POINT ( 'NONE',  ( -13.40508947812170781, 4.272460637706398645E-16, 5.527528931046010285 ) ) ;
#95392=VECTOR ( 'NONE', #89857, 1000.000000000000000 ) ;
#95393=ORIENTED_EDGE ( 'NONE', *, *, #39772, .F. ) ;
#95397=AXIS2_PLACEMENT_3D ( 'NONE', #39457, #10427, #63893 ) ;
#95399=AXIS2_PLACEMENT_3D ( 'NONE', #12796, #43297, #56823 ) ;
#95403=ORIENTED_EDGE ( 'NONE', *, *, #11493, .F. ) ;
#95405=CARTESIAN_POINT ( 'NONE',  ( -14.97687855664609913, 14.63595249122789177, 0.8325315005899581733 ) ) ;
#95407=DIRECTION ( 'NONE',  ( -0.000000000000000000, -1.000000000000000000, -0.000000000000000000 ) ) ;
#95410=EDGE_CURVE ( 'NONE', #23460, #81310, #39592, .T. ) ;
#95411=CARTESIAN_POINT ( 'NONE',  ( -14.35840480524195861, 14.63595249122789177, -4.340070442839036424 ) ) ;
#95419=CARTESIAN_POINT ( 'NONE',  ( 0.000000000000000000, 15.00000000000000000, 0.000000000000000000 ) ) ;
#95424=PLANE ( 'NONE',  #53762 ) ;
#95425=CARTESIAN_POINT ( 'NONE',  ( -12.80781515976318907, -0.03417435944610275333, 6.246788841744232990 ) ) ;
#95429=B_SPLINE_CURVE_WITH_KNOTS ( 'NONE', 3,
 ( #17793, #10288, #2810, #40787, #41776, #57244 ),
 .UNSPECIFIED., .F., .F.,
 ( 4, 2, 4 ),
 ( 0.0002800001171771102754, 0.0006862053477396429148, 0.001092410578302175500 ),
 .UNSPECIFIED. ) ;
#95451=ADVANCED_FACE ( 'NONE', ( #85080 ), #69588, .F. ) ;
#95453=CARTESIAN_POINT ( 'NONE',  ( 6.091055032734395525, 3.591419696358233438E-16, -13.29802223412757911 ) ) ;
#95455=VERTEX_POINT ( 'NONE', #62558 ) ;
#95459=CARTESIAN_POINT ( 'NONE',  ( -8.564643372776718167, 14.49999999999999112, 12.31449893000741369 ) ) ;
#95470=CARTESIAN_POINT ( 'NONE',  ( 3.469446951953614189E-15, -34.62636533006957507, 12.81628187352647608 ) ) ;
#95474=AXIS2_PLACEMENT_3D ( 'NONE', #31808, #29841, #37374 ) ;
#95480=CARTESIAN_POINT ( 'NONE',  ( 0.000000000000000000, 14.49999999999999822, 0.000000000000000000 ) ) ;
#95485=LINE ( 'NONE', #95984, #50528 ) ;
#95494=EDGE_CURVE ( 'NONE', #20560, #91650, #47006, .T. ) ;
#95499=ORIENTED_EDGE ( 'NONE', *, *, #54687, .T. ) ;
#95500=CARTESIAN_POINT ( 'NONE',  ( -8.722765153436430552, 1.609362599783170644E-16, 11.74102699209679912 ) ) ;
#95502=VERTEX_POINT ( 'NONE', #10557 ) ;
#95506=FACE_OUTER_BOUND ( 'NONE', #49343, .T. ) ;
#95511=CARTESIAN_POINT ( 'NONE',  ( 14.71525861348287734, 15.00000000000000000, 2.908807992686682109 ) ) ;
#95512=VERTEX_POINT ( 'NONE', #41068 ) ;
#95519=CARTESIAN_POINT ( 'NONE',  ( 12.00809552683959502, 0.3640475087720981828, -8.989195838243551506 ) ) ;
#95521=CARTESIAN_POINT ( 'NONE',  ( 7.082119434687047743, -29.86291783175269643, -12.26659068614894821 ) ) ;
#95522=AXIS2_PLACEMENT_3D ( 'NONE', #72942, #94954, #49451 ) ;
#95525=EDGE_CURVE ( 'NONE', #97969, #51220, #62992, .T. ) ;
#95536=EDGE_CURVE ( 'NONE', #14505, #28596, #21826, .T. ) ;
#95539=CARTESIAN_POINT ( 'NONE',  ( 2.915334737309928315, 9.522018677488167882, 10.88017736071109987 ) ) ;
#95541=CARTESIAN_POINT ( 'NONE',  ( -11.75249112336545387, 0.04962895880866165232, -8.918310463590589876 ) ) ;
#95545=AXIS2_PLACEMENT_3D ( 'NONE', #88066, #34561, #86610 ) ;
#95555=ORIENTED_EDGE ( 'NONE', *, *, #18082, .T. ) ;
#95565=CARTESIAN_POINT ( 'NONE',  ( -3.927832320392339316, 15.00000000000000000, 13.69797916712101404 ) ) ;
#95567=B_SPLINE_CURVE_WITH_KNOTS ( 'NONE', 3,
 ( #74079, #13095, #51097, #59083, #80617, #44076 ),
 .UNSPECIFIED., .F., .F.,
 ( 4, 2, 4 ),
 ( 3.409110551377157120E-05, 0.0004400426677356206748, 0.0008459942299574697106 ),
 .UNSPECIFIED. ) ;
#95571=ORIENTED_EDGE ( 'NONE', *, *, #47534, .T. ) ;
#95578=CARTESIAN_POINT ( 'NONE',  ( -3.897244926436313150, 4.087811286569849197E-16, 13.96644127841328142 ) ) ;
#95582=B_SPLINE_CURVE_WITH_KNOTS ( 'NONE', 3,
 ( #3800, #18301, #9819, #33283, #95268, #9317 ),
 .UNSPECIFIED., .F., .F.,
 ( 4, 2, 4 ),
 ( 3.409110551494648044E-05, 0.0004400426677367923179, 0.0008459942299586381553 ),
 .UNSPECIFIED. ) ;
#95583=CARTESIAN_POINT ( 'NONE',  ( -4.862001128006231632, 15.00000000000000000, -13.66056166603291189 ) ) ;
#95585=CARTESIAN_POINT ( 'NONE',  ( -2.638427012816824124, 2.050597817667449974, 9.846743663894596210 ) ) ;
#95586=ORIENTED_EDGE ( 'NONE', *, *, #34725, .F. ) ;
#95589=ORIENTED_EDGE ( 'NONE', *, *, #47875, .F. ) ;
#95598=ORIENTED_EDGE ( 'NONE', *, *, #71722, .T. ) ;
#95608=CIRCLE ( 'NONE', #98855, 14.49999999999999822 ) ;
#95611=CARTESIAN_POINT ( 'NONE',  ( -9.722841580490317881, 15.00000000000000000, -12.70211588817950066 ) ) ;
#95614=VERTEX_POINT ( 'NONE', #41570 ) ;
#95617=EDGE_CURVE ( 'NONE', #52000, #87579, #43844, .T. ) ;
#95618=CARTESIAN_POINT ( 'NONE',  ( 4.838527690343521925, 0.5000000000000004441, 14.19819177887730177 ) ) ;
#95621=CARTESIAN_POINT ( 'NONE',  ( -1.354709868695416208, 14.63595249122790598, -14.93870011653153895 ) ) ;
#95622=CARTESIAN_POINT ( 'NONE',  ( 1.354709868695618935, 0.5000000000000004441, -14.93870011653151586 ) ) ;
#95625=CARTESIAN_POINT ( 'NONE',  ( 0.000000000000000000, 15.00000000000000000, 0.000000000000000000 ) ) ;
#95636=CYLINDRICAL_SURFACE ( 'NONE', #36101, 11.92686044187656513 ) ;
#95652=CARTESIAN_POINT ( 'NONE',  ( -5.440088680355558814, -22.76964798917849109, -9.422509992056136596 ) ) ;
#95657=DIRECTION ( 'NONE',  ( -0.000000000000000000, -1.000000000000000000, -0.000000000000000000 ) ) ;
#95659=CARTESIAN_POINT ( 'NONE',  ( 1.780824192092386404, 14.49999999999999112, 14.89391369643520946 ) ) ;
#95667=CARTESIAN_POINT ( 'NONE',  ( -14.88640444357865711, 14.76930270348885088, -1.277895705730453413 ) ) ;
#95676=CARTESIAN_POINT ( 'NONE',  ( 12.25993886608599581, 15.00000000000000000, 8.642563219313704082 ) ) ;
#95682=VECTOR ( 'NONE', #7061, 1000.000000000000114 ) ;
#95684=ORIENTED_EDGE ( 'NONE', *, *, #75311, .T. ) ;
#95685=B_SPLINE_CURVE_WITH_KNOTS ( 'NONE', 3,
 ( #45464, #61446, #54923, #67981, #16946, #7975 ),
 .UNSPECIFIED., .F., .F.,
 ( 4, 2, 4 ),
 ( 0.0002800086601672329388, 0.0006862139742886589440, 0.001092419288410084949 ),
 .UNSPECIFIED. ) ;
#95686=CARTESIAN_POINT ( 'NONE',  ( 8.209432707284774366, 14.49999999999999822, 12.55409154915492032 ) ) ;
#95696=CARTESIAN_POINT ( 'NONE',  ( -14.54804176595373555, 15.00000000000000000, -6.650705016170777917 ) ) ;
#95705=CARTESIAN_POINT ( 'NONE',  ( 8.527530157486179263, -36.90773551566588395, 4.923371831947292776 ) ) ;
#95706=VERTEX_POINT ( 'NONE', #50030 ) ;
#95708=ORIENTED_EDGE ( 'NONE', *, *, #68527, .F. ) ;
#95710=ORIENTED_EDGE ( 'NONE', *, *, #64564, .F. ) ;
#95718=CARTESIAN_POINT ( 'NONE',  ( -6.408140936763246032, 13.29030133659709456, -11.09922568453594316 ) ) ;
#95719=ORIENTED_EDGE ( 'NONE', *, *, #31633, .F. ) ;
#95721=ORIENTED_EDGE ( 'NONE', *, *, #33098, .F. ) ;
#95723=AXIS2_PLACEMENT_3D ( 'NONE', #73036, #88044, #88541 ) ;
#95730=TOROIDAL_SURFACE ( 'NONE', #22311, 14.49999999999999822, 0.5000000000000000000 ) ;
#95733=ORIENTED_EDGE ( 'NONE', *, *, #25776, .F. ) ;
#95735=CARTESIAN_POINT ( 'NONE',  ( 14.71525861348295727, 14.49999999999999112, -2.908807992686619048 ) ) ;
#95739=DIRECTION ( 'NONE',  ( 3.375077994860475883E-14, 0.000000000000000000, 1.000000000000000000 ) ) ;
#95753=DIRECTION ( 'NONE',  ( 0.000000000000000000, 0.000000000000000000, 1.000000000000000000 ) ) ;
#95758=CARTESIAN_POINT ( 'NONE',  ( 14.99847009497945649, 14.63595249122788999, 0.2142307401081327833 ) ) ;
#95760=ORIENTED_EDGE ( 'NONE', *, *, #69832, .F. ) ;
#95761=CARTESIAN_POINT ( 'NONE',  ( -8.235571585149864760, 3.546802177851540172, 8.235571585149875418 ) ) ;
#95765=DIRECTION ( 'NONE',  ( 0.000000000000000000, 0.000000000000000000, 1.000000000000000000 ) ) ;
#95768=CIRCLE ( 'NONE', #9544, 15.00000000000000000 ) ;
#95777=CARTESIAN_POINT ( 'NONE',  ( -13.78891971893212443, 15.00000000000000000, 5.904717858191433244 ) ) ;
#95787=CARTESIAN_POINT ( 'NONE',  ( -4.431036607602373500, 15.00000000000000000, -14.33059365769916838 ) ) ;
#95801=FACE_OUTER_BOUND ( 'NONE', #67204, .T. ) ;
#95803=CARTESIAN_POINT ( 'NONE',  ( 5.803070148808231465, 15.00000000000000000, 13.28812917035392260 ) ) ;
#95806=CARTESIAN_POINT ( 'NONE',  ( -14.40939250469964783, 15.00000000000000000, 1.618458416365647023 ) ) ;
#95811=EDGE_LOOP ( 'NONE', ( #80022, #73196, #69623, #1274, #40052, #46353 ) ) ;
#95822=CARTESIAN_POINT ( 'NONE',  ( 14.47650479471822216, 15.00000000000000000, -3.928206833722012625 ) ) ;
#95830=EDGE_CURVE ( 'NONE', #94433, #46057, #52487, .T. ) ;
#95832=CARTESIAN_POINT ( 'NONE',  ( 0.000000000000000000, 14.49999999999999822, 0.000000000000000000 ) ) ;
#95833=ORIENTED_EDGE ( 'NONE', *, *, #65959, .F. ) ;
#95837=LINE ( 'NONE', #82670, #98418 ) ;
#95847=B_SPLINE_CURVE_WITH_KNOTS ( 'NONE', 3,
 ( #61089, #68115, #7627, #84101, #46101, #98131 ),
 .UNSPECIFIED., .F., .F.,
 ( 4, 2, 4 ),
 ( 0.0002800008091676943586, 0.0006862060465022846306, 0.001092411283836874957 ),
 .UNSPECIFIED. ) ;
#95849=EDGE_CURVE ( 'NONE', #40524, #24045, #36156, .T. ) ;
#95854=AXIS2_PLACEMENT_3D ( 'NONE', #84307, #46292, #8296 ) ;
#95856=EDGE_CURVE ( 'NONE', #70759, #66028, #13457, .T. ) ;
#95867=CARTESIAN_POINT ( 'NONE',  ( -7.618485323809357723, 15.00000000000000711, 12.48587314215754773 ) ) ;
#95868=B_SPLINE_CURVE_WITH_KNOTS ( 'NONE', 3,
 ( #12357, #227, #65843, #43344, #42864, #12844 ),
 .UNSPECIFIED., .F., .F.,
 ( 4, 2, 4 ),
 ( 0.0002800553958269955037, 0.0006862611673083459643, 0.001092466938789696425 ),
 .UNSPECIFIED. ) ;
#95887=CARTESIAN_POINT ( 'NONE',  ( 15.86177583122252344, 15.00000000000000000, -2.069169861586653170 ) ) ;
#95891=DIRECTION ( 'NONE',  ( 0.9681476403781049678, 0.000000000000000000, 0.2503800040544527095 ) ) ;
#95894=EDGE_CURVE ( 'NONE', #87579, #79151, #15805, .T. ) ;
#95899=DIRECTION ( 'NONE',  ( 0.000000000000000000, 1.000000000000000000, 0.000000000000000000 ) ) ;
#95908=CIRCLE ( 'NONE', #24042, 15.00000000000000000 ) ;
#95911=DIRECTION ( 'NONE',  ( 0.000000000000000000, 1.000000000000000000, 0.000000000000000000 ) ) ;
#95915=CARTESIAN_POINT ( 'NONE',  ( -13.55255535720589322, 15.00000000000000000, -4.403492169843143067 ) ) ;
#95918=ORIENTED_EDGE ( 'NONE', *, *, #35562, .T. ) ;
#95919=DIRECTION ( 'NONE',  ( 0.000000000000000000, 0.000000000000000000, 1.000000000000000000 ) ) ;
#95925=CARTESIAN_POINT ( 'NONE',  ( 4.265659168453312944, 0.04922511925147125822, -14.12268572233451991 ) ) ;
#95939=ORIENTED_EDGE ( 'NONE', *, *, #73384, .F. ) ;
#95950=EDGE_CURVE ( 'NONE', #76280, #18387, #22505, .T. ) ;
#95964=DIRECTION ( 'NONE',  ( -0.1132032137679106348, 0.000000000000000000, 0.9935718556765871234 ) ) ;
#95969=CARTESIAN_POINT ( 'NONE',  ( 6.408140936763243367, -29.20969866340290721, 11.09922568453594494 ) ) ;
#95978=CARTESIAN_POINT ( 'NONE',  ( -14.61146088927472064, 2.507217523872729004E-16, -0.6660010753336522704 ) ) ;
#95979=AXIS2_PLACEMENT_3D ( 'NONE', #72139, #33153, #24693 ) ;
#95980=EDGE_CURVE ( 'NONE', #49746, #30157, #15009, .T. ) ;
#95981=CARTESIAN_POINT ( 'NONE',  ( 8.375939845167682307, -0.03417435944610275333, 11.52849216984304448 ) ) ;
#95982=ORIENTED_EDGE ( 'NONE', *, *, #46564, .F. ) ;
#95984=CARTESIAN_POINT ( 'NONE',  ( 0.9940297508537879745, 15.00000000000000000, -14.21528771620249820 ) ) ;
#95985=EDGE_CURVE ( 'NONE', #90632, #6306, #9961, .T. ) ;
#95987=CIRCLE ( 'NONE', #89556, 15.00000000000000000 ) ;
#95989=ORIENTED_EDGE ( 'NONE', *, *, #50459, .T. ) ;
#95998=ORIENTED_EDGE ( 'NONE', *, *, #71933, .F. ) ;
#95999=DIRECTION ( 'NONE',  ( 0.000000000000000000, 1.000000000000000000, -0.000000000000000000 ) ) ;
#96001=ORIENTED_EDGE ( 'NONE', *, *, #13059, .T. ) ;
#96003=EDGE_CURVE ( 'NONE', #77971, #56319, #82001, .T. ) ;
#96015=VECTOR ( 'NONE', #69334, 1000.000000000000000 ) ;
#96022=CARTESIAN_POINT ( 'NONE',  ( -3.795296366450300773, -37.15458449841936783, 14.16423886937410437 ) ) ;
#96024=AXIS2_PLACEMENT_3D ( 'NONE', #91580, #76074, #7604 ) ;
#96031=CARTESIAN_POINT ( 'NONE',  ( 14.62617646268086524, 14.63595249122788999, 3.327906561566979615 ) ) ;
#96036=CARTESIAN_POINT ( 'NONE',  ( -9.422509992056136596, 13.48035201082151069, 5.440088680355559703 ) ) ;
#96042=DIRECTION ( 'NONE',  ( -0.000000000000000000, -1.000000000000000000, -0.000000000000000000 ) ) ;
#96052=DIRECTION ( 'NONE',  ( -0.000000000000000000, -1.000000000000000000, -0.000000000000000000 ) ) ;
#96054=ORIENTED_EDGE ( 'NONE', *, *, #16788, .F. ) ;
#96069=DIRECTION ( 'NONE',  ( -0.9999619230641711987, 0.000000000000000000, -0.008726535498381204903 ) ) ;
#96072=ORIENTED_EDGE ( 'NONE', *, *, #9639, .T. ) ;
#96077=DIRECTION ( 'NONE',  ( 0.000000000000000000, 0.000000000000000000, 1.000000000000000000 ) ) ;
#96078=FACE_OUTER_BOUND ( 'NONE', #7531, .T. ) ;
#96079=LINE ( 'NONE', #11581, #61144 ) ;
#96081=LINE ( 'NONE', #81065, #22111 ) ;
#96084=CARTESIAN_POINT ( 'NONE',  ( 4.923371831947295441, 4.342264484334126706, -8.527530157486179263 ) ) ;
#96086=CARTESIAN_POINT ( 'NONE',  ( 14.17193700899790265, -0.03417435944610275333, -1.489530601564018175 ) ) ;
#96110=DIRECTION ( 'NONE',  ( 0.000000000000000000, 1.000000000000000000, 0.000000000000000000 ) ) ;
#96120=B_SPLINE_CURVE_WITH_KNOTS ( 'NONE', 3,
 ( #49265, #51234, #26755, #58219, #11757, #57250 ),
 .UNSPECIFIED., .F., .F.,
 ( 4, 2, 4 ),
 ( 0.0002800020636817301435, 0.0006862073132860486719, 0.001092412562890367200 ),
 .UNSPECIFIED. ) ;
#96129=EDGE_LOOP ( 'NONE', ( #84285, #84657, #28801, #50201 ) ) ;
#96130=LINE ( 'NONE', #26149, #91082 ) ;
#96145=CARTESIAN_POINT ( 'NONE',  ( 11.33568117652998986, 12.60026003655735849, -0.6654292126732216373 ) ) ;
#96152=CARTESIAN_POINT ( 'NONE',  ( 9.422509992056141925, -29.85298132251182324, 5.440088680355547268 ) ) ;
#96161=CIRCLE ( 'NONE', #70612, 15.00000000000000000 ) ;
#96165=DIRECTION ( 'NONE',  ( -0.5807029557109515405, -0.000000000000000000, 0.8141155183563107967 ) ) ;
#96178=DIRECTION ( 'NONE',  ( 0.000000000000000000, 0.000000000000000000, -1.000000000000000000 ) ) ;
#96179=CARTESIAN_POINT ( 'NONE',  ( -3.468686501387143295, 0.000000000000000000, -4.207853202970329498 ) ) ;
#96180=ADVANCED_FACE ( 'NONE', ( #31451 ), #89960, .T. ) ;
#96182=CIRCLE ( 'NONE', #53057, 14.49999999999999822 ) ;
#96183=LINE ( 'NONE', #27666, #65851 ) ;
#96186=ORIENTED_EDGE ( 'NONE', *, *, #97896, .T. ) ;
#96197=EDGE_CURVE ( 'NONE', #79151, #47550, #77445, .T. ) ;
#96201=DIRECTION ( 'NONE',  ( 0.000000000000000000, 0.000000000000000000, -1.000000000000000000 ) ) ;
#96204=CARTESIAN_POINT ( 'NONE',  ( 2.638427012816835227, -32.53273551566588395, 9.846743663894590881 ) ) ;
#96208=ORIENTED_EDGE ( 'NONE', *, *, #53411, .F. ) ;
#96213=CARTESIAN_POINT ( 'NONE',  ( 14.71525861348295727, 14.49999999999999112, -2.908807992686619048 ) ) ;
#96218=CARTESIAN_POINT ( 'NONE',  ( -11.09922568453595382, 3.706968003263755307, -6.408140936763226492 ) ) ;
#96235=AXIS2_PLACEMENT_3D ( 'NONE', #32381, #93383, #17410 ) ;
#96236=LINE ( 'NONE', #71751, #19522 ) ;
#96238=CARTESIAN_POINT ( 'NONE',  ( 0.000000000000000000, 14.49999999999999822, 0.000000000000000000 ) ) ;
#96242=ORIENTED_EDGE ( 'NONE', *, *, #49412, .T. ) ;
#96244=CARTESIAN_POINT ( 'NONE',  ( -13.16740645155962852, 0.04922511925147048800, -6.653232860246741431 ) ) ;
#96249=CARTESIAN_POINT ( 'NONE',  ( 8.839000071697000749, 0.04962890530003118833, 11.81225584161647113 ) ) ;
#96261=AXIS2_PLACEMENT_3D ( 'NONE', #5630, #59596, #98629 ) ;
#96269=CARTESIAN_POINT ( 'NONE',  ( 5.795997163830165277, 15.00000000000000000, -13.01802277140705932 ) ) ;
#96274=CARTESIAN_POINT ( 'NONE',  ( 2.962741594153077251, -0.03417435944610275333, -13.93860331045673107 ) ) ;
#96281=CARTESIAN_POINT ( 'NONE',  ( 11.59580422753452922, 14.76984949557379245, 9.421229451859275628 ) ) ;
#96287=FACE_OUTER_BOUND ( 'NONE', #63718, .T. ) ;
#96289=ADVANCED_FACE ( 'NONE', ( #50395 ), #3760, .T. ) ;
#96293=ORIENTED_EDGE ( 'NONE', *, *, #31738, .F. ) ;
#96298=VECTOR ( 'NONE', #71846, 1000.000000000000000 ) ;
#96302=CARTESIAN_POINT ( 'NONE',  ( -13.55101055326594839, 14.76984994142488361, 6.292244619294627306 ) ) ;
#96306=DIRECTION ( 'NONE',  ( 0.000000000000000000, 1.000000000000000000, 0.000000000000000000 ) ) ;
#96311=EDGE_CURVE ( 'NONE', #83450, #53280, #89805, .T. ) ;
#96313=ORIENTED_EDGE ( 'NONE', *, *, #42600, .T. ) ;
#96315=CARTESIAN_POINT ( 'NONE',  ( 1.983216688680843109, -0.03417435944610275333, 14.11131997956739070 ) ) ;
#96320=CARTESIAN_POINT ( 'NONE',  ( 0.000000000000000000, 14.49999999999999822, 0.000000000000000000 ) ) ;
#96326=DIRECTION ( 'NONE',  ( -0.000000000000000000, -1.000000000000000000, -0.000000000000000000 ) ) ;
#96332=ORIENTED_EDGE ( 'NONE', *, *, #97672, .T. ) ;
#96334=ORIENTED_EDGE ( 'NONE', *, *, #66898, .T. ) ;
#96336=DIRECTION ( 'NONE',  ( -0.8038568606172203923, 0.000000000000000000, 0.5948227867513371514 ) ) ;
#96337=DIRECTION ( 'NONE',  ( 0.3826834323650877834, -0.000000000000000000, 0.9238795325112876267 ) ) ;
#96347=ORIENTED_EDGE ( 'NONE', *, *, #10295, .T. ) ;
#96351=ORIENTED_EDGE ( 'NONE', *, *, #50335, .F. ) ;
#96356=CARTESIAN_POINT ( 'NONE',  ( -7.443082168244859353, 2.043284506775928211, -9.050130897022322429 ) ) ;
#96367=DIRECTION ( 'NONE',  ( -0.1650476058606676344, 0.000000000000000000, -0.9862856015372331031 ) ) ;
#96373=LINE ( 'NONE', #75698, #77840 ) ;
#96379=VERTEX_POINT ( 'NONE', #13892 ) ;
#96393=CARTESIAN_POINT ( 'NONE',  ( -4.873787042390612001, -0.03417435944610275333, -13.39061984619925916 ) ) ;
#96399=DIRECTION ( 'NONE',  ( -0.000000000000000000, -1.000000000000000000, -0.000000000000000000 ) ) ;
#96407=DIRECTION ( 'NONE',  ( 0.000000000000000000, 0.000000000000000000, 1.000000000000000000 ) ) ;
#96410=CARTESIAN_POINT ( 'NONE',  ( -10.32896413005679648, 10.10497603579418247, 5.963430220938290560 ) ) ;
#96413=ORIENTED_EDGE ( 'NONE', *, *, #71490, .F. ) ;
#96416=DIRECTION ( 'NONE',  ( 0.000000000000000000, 0.000000000000000000, 1.000000000000000000 ) ) ;
#96419=LINE ( 'NONE', #58382, #40715 ) ;
#96421=CARTESIAN_POINT ( 'NONE',  ( 8.375939845167756914, 0.000000000000000000, -11.52849216984298941 ) ) ;
#96429=EDGE_CURVE ( 'NONE', #46057, #78138, #36390, .T. ) ;
#96432=EDGE_CURVE ( 'NONE', #4350, #30913, #66884, .T. ) ;
#96439=ORIENTED_EDGE ( 'NONE', *, *, #26204, .F. ) ;
#96440=LINE ( 'NONE', #88426, #34073 ) ;
#96441=CARTESIAN_POINT ( 'NONE',  ( 0.000000000000000000, 14.49999999999999822, 0.000000000000000000 ) ) ;
#96443=DIRECTION ( 'NONE',  ( 0.000000000000000000, 1.000000000000000000, 0.000000000000000000 ) ) ;
#96451=CARTESIAN_POINT ( 'NONE',  ( -12.03768810259473732, 15.00000000000000533, -8.306778944023500699 ) ) ;
#96459=CARTESIAN_POINT ( 'NONE',  ( 0.000000000000000000, 14.49999999999999822, 0.000000000000000000 ) ) ;
#96462=B_SPLINE_CURVE_WITH_KNOTS ( 'NONE', 3,
 ( #87922, #2985, #18952, #49927, #11440, #2499 ),
 .UNSPECIFIED., .F., .F.,
 ( 4, 2, 4 ),
 ( 3.409110551494641945E-05, 0.0004400426677367920468, 0.0008459942299586376132 ),
 .UNSPECIFIED. ) ;
#96465=CARTESIAN_POINT ( 'NONE',  ( -10.19513985507840736, 0.5000000000000004441, 11.00268709613209950 ) ) ;
#96470=CARTESIAN_POINT ( 'NONE',  ( 11.09922568453595026, -18.79303199673624292, 6.408140936763232709 ) ) ;
#96478=EDGE_CURVE ( 'NONE', #1436, #73387, #83369, .T. ) ;
#96486=VECTOR ( 'NONE', #10189, 1000.000000000000000 ) ;
#96495=DIRECTION ( 'NONE',  ( 0.9588197348681964938, 0.000000000000000000, -0.2840153447039108214 ) ) ;
#96501=ORIENTED_EDGE ( 'NONE', *, *, #2089, .T. ) ;
#96505=DIRECTION ( 'NONE',  ( 0.1822355254921448342, 0.000000000000000000, 0.9832549075639550606 ) ) ;
#96508=ADVANCED_FACE ( 'NONE', ( #45362 ), #45292, .T. ) ;
#96524=CARTESIAN_POINT ( 'NONE',  ( 10.36894250292379027, -31.32125116508602858, 10.36894250292378672 ) ) ;
#96527=ORIENTED_EDGE ( 'NONE', *, *, #67082, .F. ) ;
#96528=CARTESIAN_POINT ( 'NONE',  ( -11.48952521350030587, 15.00000000000000000, 8.845383562533664090 ) ) ;
#96538=CARTESIAN_POINT ( 'NONE',  ( -5.440088680355547268, 13.89701867748818032, 9.422509992056143702 ) ) ;
#96545=CARTESIAN_POINT ( 'NONE',  ( -13.61464873478165138, 14.49999999999999112, -6.296136897218031159 ) ) ;
#96553=CARTESIAN_POINT ( 'NONE',  ( 3.195792623639593266, 9.120456701841145986, 11.92686044187653494 ) ) ;
#96556=VERTEX_POINT ( 'NONE', #84370 ) ;
#96558=AXIS2_PLACEMENT_3D ( 'NONE', #33049, #1605, #32054 ) ;
#96560=CARTESIAN_POINT ( 'NONE',  ( 6.689969769698956625, 15.00000000000000000, -12.58200319823970226 ) ) ;
#96567=CARTESIAN_POINT ( 'NONE',  ( 13.40508947812166873, 4.119406375368599477E-16, -5.527528931046103544 ) ) ;
#96570=ORIENTED_EDGE ( 'NONE', *, *, #91225, .T. ) ;
#96581=CARTESIAN_POINT ( 'NONE',  ( 12.25993886608605976, 14.63595249122790953, -8.642563219313631251 ) ) ;
#96585=CARTESIAN_POINT ( 'NONE',  ( -3.469446951953614189E-15, -0.2410688489992082739, -9.846743663894594434 ) ) ;
#96588=VERTEX_POINT ( 'NONE', #55829 ) ;
#96590=ORIENTED_EDGE ( 'NONE', *, *, #54183, .T. ) ;
#96596=AXIS2_PLACEMENT_3D ( 'NONE', #17645, #46638, #47633 ) ;
#96599=ORIENTED_EDGE ( 'NONE', *, *, #33254, .F. ) ;
#96604=ORIENTED_EDGE ( 'NONE', *, *, #88957, .F. ) ;
#96608=LINE ( 'NONE', #74072, #4290 ) ;
#96615=ORIENTED_EDGE ( 'NONE', *, *, #49353, .T. ) ;
#96617=CARTESIAN_POINT ( 'NONE',  ( 0.000000000000000000, 15.00000000000000000, 0.000000000000000000 ) ) ;
#96619=EDGE_LOOP ( 'NONE', ( #93962, #76941, #78037, #96439 ) ) ;
#96621=DIRECTION ( 'NONE',  ( -0.5519369853120501546, 0.000000000000000000, -0.8338858220671735433 ) ) ;
#96622=DIRECTION ( 'NONE',  ( 0.7604059656000297096, 0.000000000000000000, 0.6494480483301851015 ) ) ;
#96627=DIRECTION ( 'NONE',  ( 0.000000000000000000, 0.000000000000000000, -1.000000000000000000 ) ) ;
#96632=EDGE_CURVE ( 'NONE', #27349, #24643, #47322, .T. ) ;
#96637=CIRCLE ( 'NONE', #88614, 14.49999999999999822 ) ;
#96638=ORIENTED_EDGE ( 'NONE', *, *, #94043, .T. ) ;
#96646=CARTESIAN_POINT ( 'NONE',  ( -9.972640495195461696, -0.03417435944610275333, 12.50695158660338890 ) ) ;
#96651=CARTESIAN_POINT ( 'NONE',  ( -9.422509992056136596, -31.51964798917848753, 5.440088680355559703 ) ) ;
#96656=CIRCLE ( 'NONE', #63089, 15.00000000000000000 ) ;
#96658=DIRECTION ( 'NONE',  ( 0.9914448613738104932, 0.000000000000000000, -0.1305261922200514901 ) ) ;
#96665=CARTESIAN_POINT ( 'NONE',  ( 4.838527690343618737, 15.00000000000000000, -14.19819177887726624 ) ) ;
#96666=ADVANCED_FACE ( 'NONE', ( #85833 ), #77330, .F. ) ;
#96680=TOROIDAL_SURFACE ( 'NONE', #23237, 14.49999999999999822, 0.5000000000000000000 ) ;
#96681=CARTESIAN_POINT ( 'NONE',  ( -2.962741594152892510, -0.03417435944610275333, -13.93860331045676837 ) ) ;
#96682=CARTESIAN_POINT ( 'NONE',  ( 8.209432707284868513, 0.3640475087720981828, -12.55409154915486525 ) ) ;
#96684=VECTOR ( 'NONE', #59533, 1000.000000000000000 ) ;
#96703=CARTESIAN_POINT ( 'NONE',  ( 14.48718990079890112, 15.00000000000000000, -0.6093675230840328583 ) ) ;
#96706=CARTESIAN_POINT ( 'NONE',  ( -9.846743663894590881, -38.78273551566588395, 2.638427012816840111 ) ) ;
#96707=ORIENTED_EDGE ( 'NONE', *, *, #94046, .F. ) ;
#96708=DIRECTION ( 'NONE',  ( 0.000000000000000000, 1.000000000000000000, 0.000000000000000000 ) ) ;
#96714=EDGE_CURVE ( 'NONE', #60892, #27552, #74204, .T. ) ;
#96715=PLANE ( 'NONE',  #86142 ) ;
#96718=B_SPLINE_CURVE_WITH_KNOTS ( 'NONE', 3,
 ( #31173, #38213, #52699, #719, #16191, #98229 ),
 .UNSPECIFIED., .F., .F.,
 ( 4, 2, 4 ),
 ( 0.0002800338592613166202, 0.0006862394199319977583, 0.001092444980602678842 ),
 .UNSPECIFIED. ) ;
#96719=CARTESIAN_POINT ( 'NONE',  ( -3.434112377981067610, 8.081968003263751754, -12.81628187352647252 ) ) ;
#96720=ORIENTED_EDGE ( 'NONE', *, *, #1810, .F. ) ;
#96732=DIRECTION ( 'NONE',  ( -3.730349362740526607E-14, 0.000000000000000000, 1.000000000000000000 ) ) ;
#96738=CARTESIAN_POINT ( 'NONE',  ( 2.849309504156536832, 0.000000000000000000, -4.649650521509789414 ) ) ;
#96742=VERTEX_POINT ( 'NONE', #78317 ) ;
#96743=CARTESIAN_POINT ( 'NONE',  ( -9.520529577030568902, 4.404571325722360777E-16, 11.10395710204414499 ) ) ;
#96753=EDGE_CURVE ( 'NONE', #21313, #58402, #23869, .T. ) ;
#96759=VECTOR ( 'NONE', #14862, 1000.000000000000114 ) ;
#96767=CARTESIAN_POINT ( 'NONE',  ( 0.000000000000000000, 0.5000000000000004441, 0.000000000000000000 ) ) ;
#96773=CARTESIAN_POINT ( 'NONE',  ( 14.16423886937410082, 9.512082168247301794, -3.795296366450314096 ) ) ;
#96781=ORIENTED_EDGE ( 'NONE', *, *, #88065, .T. ) ;
#96785=CARTESIAN_POINT ( 'NONE',  ( 0.000000000000000000, 14.49999999999999822, 0.000000000000000000 ) ) ;
#96791=EDGE_CURVE ( 'NONE', #2489, #71703, #86323, .T. ) ;
#96794=CARTESIAN_POINT ( 'NONE',  ( -12.84737282370062061, -0.03417435944610275333, -9.530079116402557560 ) ) ;
#96800=CARTESIAN_POINT ( 'NONE',  ( 8.564643372776615138, 0.5000000000000004441, -12.31449893000740836 ) ) ;
#96801=DIRECTION ( 'NONE',  ( 0.9914448613738104932, 0.000000000000000000, -0.1305261922200514901 ) ) ;
#96834=DIRECTION ( 'NONE',  ( -0.6755902076156540259, 0.000000000000000000, -0.7372773368101297464 ) ) ;
#96835=VECTOR ( 'NONE', #10660, 999.9999999999998863 ) ;
#96847=ORIENTED_EDGE ( 'NONE', *, *, #63090, .T. ) ;
#96851=CARTESIAN_POINT ( 'NONE',  ( 0.000000000000000000, 15.00000000000000000, 0.000000000000000000 ) ) ;
#96854=TOROIDAL_SURFACE ( 'NONE', #5835, 14.49999999999999822, 0.5000000000000000000 ) ;
#96856=ORIENTED_EDGE ( 'NONE', *, *, #37300, .T. ) ;
#96857=AXIS2_PLACEMENT_3D ( 'NONE', #22108, #14620, #43115 ) ;
#96863=ORIENTED_EDGE ( 'NONE', *, *, #28457, .T. ) ;
#96868=CARTESIAN_POINT ( 'NONE',  ( -7.313705784284733724, 14.49999999999999112, 13.09617149020743199 ) ) ;
#96871=CARTESIAN_POINT ( 'NONE',  ( 0.000000000000000000, 15.00000000000000000, 0.000000000000000000 ) ) ;
#96875=EDGE_CURVE ( 'NONE', #86520, #23897, #64601, .T. ) ;
#96877=ORIENTED_EDGE ( 'NONE', *, *, #56988, .F. ) ;
#96878=CARTESIAN_POINT ( 'NONE',  ( -10.91061041304835300, 14.76930270348882068, 10.20767530377041332 ) ) ;
#96879=DIRECTION ( 'NONE',  ( -0.000000000000000000, -1.000000000000000000, -0.000000000000000000 ) ) ;
#96882=CARTESIAN_POINT ( 'NONE',  ( 3.014428414850129911, 8.659700295649312096, -11.25000000000000000 ) ) ;
#96899=CARTESIAN_POINT ( 'NONE',  ( 0.000000000000000000, 0.5000000000000004441, 0.000000000000000000 ) ) ;
#96906=AXIS2_PLACEMENT_3D ( 'NONE', #73097, #11624, #35606 ) ;
#96908=DIRECTION ( 'NONE',  ( 0.9914448613738084948, 0.000000000000000000, 0.1305261922200653124 ) ) ;
#96909=CARTESIAN_POINT ( 'NONE',  ( -9.742785792574940373, 7.505135511184873209, -5.624999999999991118 ) ) ;
#96914=EDGE_LOOP ( 'NONE', ( #5123, #19038, #74081, #30985, #1318, #11502 ) ) ;
#96919=CARTESIAN_POINT ( 'NONE',  ( 1.354709868695515684, 15.00000000000000000, 14.93870011653152652 ) ) ;
#96928=VECTOR ( 'NONE', #21409, 1000.000000000000227 ) ;
#96931=VECTOR ( 'NONE', #10106, 1000.000000000000114 ) ;
#96943=DIRECTION ( 'NONE',  ( 0.9483236552062023206, 0.000000000000000000, -0.3173046564050834295 ) ) ;
#96948=ORIENTED_EDGE ( 'NONE', *, *, #6450, .T. ) ;
#96953=CARTESIAN_POINT ( 'NONE',  ( -2.962741594153171842, -0.03417435944610275333, 13.93860331045670975 ) ) ;
#96954=ORIENTED_EDGE ( 'NONE', *, *, #37571, .F. ) ;
#96965=CIRCLE ( 'NONE', #82514, 11.92686044187656513 ) ;
#96966=DIRECTION ( 'NONE',  ( 0.7716245833877193316, 0.000000000000000000, -0.6360782202777648386 ) ) ;
#96971=CARTESIAN_POINT ( 'NONE',  ( 3.434112377981060948, -14.41803199673624469, 12.81628187352647430 ) ) ;
#96978=AXIS2_PLACEMENT_3D ( 'NONE', #66766, #22763, #13769 ) ;
#96980=DIRECTION ( 'NONE',  ( -0.000000000000000000, -1.000000000000000000, -0.000000000000000000 ) ) ;
#97004=EDGE_CURVE ( 'NONE', #54629, #5586, #47220, .T. ) ;
#97014=CARTESIAN_POINT ( 'NONE',  ( 5.419894505350588254, 0.3640475087720895231, -13.98659156302459472 ) ) ;
#97023=CARTESIAN_POINT ( 'NONE',  ( -10.36894250292378317, -22.57125116508603213, 10.36894250292379560 ) ) ;
#97027=EDGE_LOOP ( 'NONE', ( #35535, #43641, #16544, #33478, #93015, #69052 ) ) ;
#97029=VECTOR ( 'NONE', #81888, 1000.000000000000000 ) ;
#97034=CARTESIAN_POINT ( 'NONE',  ( 2.827051895225687783, 14.76984989550149407, 14.67071941139715108 ) ) ;
#97037=DIRECTION ( 'NONE',  ( 0.000000000000000000, 0.000000000000000000, 1.000000000000000000 ) ) ;
#97040=CARTESIAN_POINT ( 'NONE',  ( -9.422509992056136596, 33.48035201082149825, 5.440088680355559703 ) ) ;
#97043=CARTESIAN_POINT ( 'NONE',  ( 0.000000000000000000, 14.49999999999999822, 0.000000000000000000 ) ) ;
#97054=CARTESIAN_POINT ( 'NONE',  ( 10.32896413005680181, 9.745456701841140656, 5.963430220938278126 ) ) ;
#97055=DIRECTION ( 'NONE',  ( -6.217248937900876626E-14, 0.000000000000000000, 1.000000000000000000 ) ) ;
#97065=VECTOR ( 'NONE', #78120, 1000.000000000000114 ) ;
#97069=CARTESIAN_POINT ( 'NONE',  ( -4.326345305608673364, 0.000000000000000000, 3.319721512309553368 ) ) ;
#97071=DIRECTION ( 'NONE',  ( 0.000000000000000000, -1.000000000000000000, 0.000000000000000000 ) ) ;
#97072=AXIS2_PLACEMENT_3D ( 'NONE', #46215, #92684, #60222 ) ;
#97075=AXIS2_PLACEMENT_3D ( 'NONE', #85746, #31741, #40734 ) ;
#97076=VERTEX_POINT ( 'NONE', #8261 ) ;
#97090=CARTESIAN_POINT ( 'NONE',  ( 3.469446951953614189E-15, 22.25893115100079100, 9.846743663894594434 ) ) ;
#97101=EDGE_CURVE ( 'NONE', #98966, #39344, #62225, .T. ) ;
#97109=VERTEX_POINT ( 'NONE', #78219 ) ;
#97115=CARTESIAN_POINT ( 'NONE',  ( 0.000000000000000000, 15.00000000000000000, 0.000000000000000000 ) ) ;
#97116=VECTOR ( 'NONE', #85502, 1000.000000000000114 ) ;
#97117=VERTEX_POINT ( 'NONE', #16745 ) ;
#97120=ORIENTED_EDGE ( 'NONE', *, *, #40419, .T. ) ;
#97122=CARTESIAN_POINT ( 'NONE',  ( 4.862001128006681938, 4.613545383394330660E-16, 13.66056166602463229 ) ) ;
#97125=TOROIDAL_SURFACE ( 'NONE', #17321, 14.49999999999999822, 0.5000000000000000000 ) ;
#97126=ORIENTED_EDGE ( 'NONE', *, *, #85946, .F. ) ;
#97132=VERTEX_POINT ( 'NONE', #32214 ) ;
#97133=DIRECTION ( 'NONE',  ( -0.008726535498367549160, 0.000000000000000000, -0.9999619230641714207 ) ) ;
#97135=FACE_OUTER_BOUND ( 'NONE', #42855, .T. ) ;
#97141=VECTOR ( 'NONE', #47004, 1000.000000000000000 ) ;
#97142=CARTESIAN_POINT ( 'NONE',  ( -6.382347221874512755, 0.5000000000000004441, 13.57444820018223375 ) ) ;
#97149=CARTESIAN_POINT ( 'NONE',  ( 9.159723438033203990, 0.000000000000000000, -10.91613331444542645 ) ) ;
#97152=CARTESIAN_POINT ( 'NONE',  ( -4.873787042390612001, 15.00000000000000000, -13.39061984619925916 ) ) ;
#97153=DIRECTION ( 'NONE',  ( 0.000000000000000000, 0.000000000000000000, 1.000000000000000000 ) ) ;
#97158=CARTESIAN_POINT ( 'NONE',  ( 10.88017736071110519, -29.43631465584515894, -2.602085213965210642E-15 ) ) ;
#97162=DIRECTION ( 'NONE',  ( -0.6360782202777597316, 0.000000000000000000, -0.7716245833877234395 ) ) ;
#97163=CARTESIAN_POINT ( 'NONE',  ( 13.95697193428312310, 15.00000000000000711, -4.371663894958823349 ) ) ;
#97173=VERTEX_POINT ( 'NONE', #62715 ) ;
#97183=CARTESIAN_POINT ( 'NONE',  ( 8.157990163924791815, 0.2306972965111897811, -12.51739793958113722 ) ) ;
#97184=EDGE_LOOP ( 'NONE', ( #78023, #44566, #35304, #4913, #85258, #40249 ) ) ;
#97185=CIRCLE ( 'NONE', #13733, 15.00000000000000000 ) ;
#97189=ORIENTED_EDGE ( 'NONE', *, *, #53885, .T. ) ;
#97190=CARTESIAN_POINT ( 'NONE',  ( -14.52941021839283131, -2.744386749103930633E-16, -1.683622718073243263 ) ) ;
#97206=CARTESIAN_POINT ( 'NONE',  ( 9.846743663894590881, -21.69940218233254470, 2.638427012816828565 ) ) ;
#97207=ORIENTED_EDGE ( 'NONE', *, *, #54333, .F. ) ;
#97210=ORIENTED_EDGE ( 'NONE', *, *, #96311, .T. ) ;
#97215=AXIS2_PLACEMENT_3D ( 'NONE', #40129, #85137, #40627 ) ;
#97220=CARTESIAN_POINT ( 'NONE',  ( 12.81628187352647608, 6.415301336597086568, 3.434112377981052511 ) ) ;
#97221=VERTEX_POINT ( 'NONE', #85241 ) ;
#97227=AXIS2_PLACEMENT_3D ( 'NONE', #60188, #37221, #59692 ) ;
#97231=CARTESIAN_POINT ( 'NONE',  ( 5.991992585808628036, 4.207234274712436881E-16, -13.20401548210295140 ) ) ;
#97234=EDGE_CURVE ( 'NONE', #98695, #35712, #9731, .T. ) ;
#97236=FACE_OUTER_BOUND ( 'NONE', #98120, .T. ) ;
#97237=CARTESIAN_POINT ( 'NONE',  ( -10.19513985507817821, 0.5000000000000004441, -11.00268709613231088 ) ) ;
#97245=CARTESIAN_POINT ( 'NONE',  ( -13.07734668325334759, 2.727446090158847092E-16, -6.551438809693111764 ) ) ;
#97249=CARTESIAN_POINT ( 'NONE',  ( -14.26295192185806293, 0.04922511925147220885, -3.770186020345214661 ) ) ;
#97251=CARTESIAN_POINT ( 'NONE',  ( -10.82344394350217875, 0.04922511925147111944, -10.02492699998892967 ) ) ;
#97256=CARTESIAN_POINT ( 'NONE',  ( -8.731067818237040257, 7.037123368507812060, -8.731067818237033151 ) ) ;
#97260=CARTESIAN_POINT ( 'NONE',  ( -3.836325488035988496, 0.3640475087720956293, -14.50112432709428667 ) ) ;
#97270=CARTESIAN_POINT ( 'NONE',  ( -14.16423886937409726, 7.012082168247292913, 3.795296366450320757 ) ) ;
#97273=CARTESIAN_POINT ( 'NONE',  ( 12.67122524790586269, 0.04922511925147014800, 7.555537761805852348 ) ) ;
#97282=CARTESIAN_POINT ( 'NONE',  ( 10.69820648722788015, 1.823139558123380688, 5.272416709312279792 ) ) ;
#97283=CARTESIAN_POINT ( 'NONE',  ( 2.826948239413825892, 0.2306972965111907248, 14.67127868811027724 ) ) ;
#97288=CARTESIAN_POINT ( 'NONE',  ( -12.83294900548053086, 0.3640475087720986824, -7.766300266068548730 ) ) ;
#97313=DIRECTION ( 'NONE',  ( 0.000000000000000000, 0.000000000000000000, -1.000000000000000000 ) ) ;
#97319=VERTEX_POINT ( 'NONE', #781 ) ;
#97321=EDGE_CURVE ( 'NONE', #14921, #75327, #86103, .T. ) ;
#97326=CARTESIAN_POINT ( 'NONE',  ( -1.780824192092292924, 0.5000000000000004441, -14.89391369643515795 ) ) ;
#97327=ORIENTED_EDGE ( 'NONE', *, *, #53839, .T. ) ;
#97330=VERTEX_POINT ( 'NONE', #79203 ) ;
#97335=ORIENTED_EDGE ( 'NONE', *, *, #77853, .T. ) ;
#97344=ADVANCED_FACE ( 'NONE', ( #87190 ), #21379, .T. ) ;
#97361=CARTESIAN_POINT ( 'NONE',  ( -3.753761956877471384, 0.000000000000000000, -3.955639745193241019 ) ) ;
#97377=LINE ( 'NONE', #59348, #4803 ) ;
#97384=CARTESIAN_POINT ( 'NONE',  ( -12.83294900548073336, 14.49999999999999112, 7.766300266068329350 ) ) ;
#97385=ADVANCED_FACE ( 'NONE', ( #63696 ), #69286, .T. ) ;
#97402=EDGE_CURVE ( 'NONE', #63527, #46976, #65665, .T. ) ;
#97409=DIRECTION ( 'NONE',  ( 0.000000000000000000, 0.000000000000000000, 1.000000000000000000 ) ) ;
#97414=DIRECTION ( 'NONE',  ( -0.000000000000000000, 1.000000000000000000, -0.000000000000000000 ) ) ;
#97433=ORIENTED_EDGE ( 'NONE', *, *, #35938, .T. ) ;
#97436=AXIS2_PLACEMENT_3D ( 'NONE', #4740, #57716, #41759 ) ;
#97438=EDGE_CURVE ( 'NONE', #68868, #8246, #55493, .T. ) ;
#97441=ORIENTED_EDGE ( 'NONE', *, *, #31434, .F. ) ;
#97451=CARTESIAN_POINT ( 'NONE',  ( 8.439016546559823695, 15.00000000000000000, 11.79122553964979048 ) ) ;
#97457=CARTESIAN_POINT ( 'NONE',  ( 9.382169495545419124, -14.00136533006957329, 9.382169495545417348 ) ) ;
#97465=B_SPLINE_CURVE_WITH_KNOTS ( 'NONE', 3,
 ( #45439, #68454, #60931, #15938, #15465, #22461 ),
 .UNSPECIFIED., .F., .F.,
 ( 4, 2, 4 ),
 ( 3.409110551494480670E-05, 0.0004400426677367911253, 0.0008459942299586375048 ),
 .UNSPECIFIED. ) ;
#97466=EDGE_CURVE ( 'NONE', #21190, #47609, #80065, .T. ) ;
#97487=VECTOR ( 'NONE', #19184, 1000.000000000000000 ) ;
#97512=EDGE_CURVE ( 'NONE', #15924, #84126, #19685, .T. ) ;
#97515=CARTESIAN_POINT ( 'NONE',  ( -3.795296366450322534, -24.23791783175269643, -14.16423886937409904 ) ) ;
#97519=ORIENTED_EDGE ( 'NONE', *, *, #38608, .T. ) ;
#97527=TOROIDAL_SURFACE ( 'NONE', #33603, 14.49999999999999822, 0.5000000000000000000 ) ;
#97530=CARTESIAN_POINT ( 'NONE',  ( -9.422509992056145478, 27.64701867748817321, -5.440088680355541939 ) ) ;
#97535=ORIENTED_EDGE ( 'NONE', *, *, #2514, .T. ) ;
#97561=CARTESIAN_POINT ( 'NONE',  ( 0.000000000000000000, 15.00000000000000000, 0.000000000000000000 ) ) ;
#97562=DIRECTION ( 'NONE',  ( -0.3173046564050965856, 0.000000000000000000, 0.9483236552061978797 ) ) ;
#97569=DIRECTION ( 'NONE',  ( -0.000000000000000000, -1.000000000000000000, -0.000000000000000000 ) ) ;
#97575=EDGE_CURVE ( 'NONE', #76622, #2401, #33201, .T. ) ;
#97580=CARTESIAN_POINT ( 'NONE',  ( 0.000000000000000000, 15.00000000000000000, 0.000000000000000000 ) ) ;
#97581=CARTESIAN_POINT ( 'NONE',  ( -4.923371831947302546, 20.17559781766745175, -8.527530157486173934 ) ) ;
#97582=ORIENTED_EDGE ( 'NONE', *, *, #97402, .F. ) ;
#97583=EDGE_LOOP ( 'NONE', ( #24407, #56035, #93250, #90137 ) ) ;
#97584=DIRECTION ( 'NONE',  ( 0.000000000000000000, 0.000000000000000000, 1.000000000000000000 ) ) ;
#97596=VERTEX_POINT ( 'NONE', #27670 ) ;
#97599=ORIENTED_EDGE ( 'NONE', *, *, #68918, .T. ) ;
#97600=EDGE_CURVE ( 'NONE', #60663, #90632, #93246, .T. ) ;
#97606=CARTESIAN_POINT ( 'NONE',  ( -13.55255535720598026, -0.03417435944610275333, 4.403492169842870396 ) ) ;
#97611=EDGE_CURVE ( 'NONE', #13980, #47708, #89164, .T. ) ;
#97621=CARTESIAN_POINT ( 'NONE',  ( 14.97653319723437626, 15.00000000000000000, 5.619684139539351975 ) ) ;
#97625=CARTESIAN_POINT ( 'NONE',  ( 9.282040431732685448, 15.00000000000000711, -11.30407325590339696 ) ) ;
#97629=DIRECTION ( 'NONE',  ( -0.000000000000000000, -1.000000000000000000, -0.000000000000000000 ) ) ;
#97639=CARTESIAN_POINT ( 'NONE',  ( -10.14667048435130781, 4.359436697371537845E-16, -10.35833375027055148 ) ) ;
#97642=CARTESIAN_POINT ( 'NONE',  ( 0.000000000000000000, 14.49999999999999822, 0.000000000000000000 ) ) ;
#97646=CARTESIAN_POINT ( 'NONE',  ( -7.964842623401179544, -7.561314655845157162, -7.964842623401174215 ) ) ;
#97651=CARTESIAN_POINT ( 'NONE',  ( -15.61289147378506748, 15.00000000000000000, -3.480663193108890496 ) ) ;
#97652=EDGE_CURVE ( 'NONE', #33114, #98886, #5403, .T. ) ;
#97663=LINE ( 'NONE', #89641, #76528 ) ;
#97670=FACE_OUTER_BOUND ( 'NONE', #12382, .T. ) ;
#97672=EDGE_CURVE ( 'NONE', #47550, #66028, #74146, .T. ) ;
#97677=EDGE_CURVE ( 'NONE', #39990, #16062, #94401, .T. ) ;
#97691=EDGE_CURVE ( 'NONE', #14505, #52889, #5185, .T. ) ;
#97696=CARTESIAN_POINT ( 'NONE',  ( -2.638427012816824124, -27.94940218233254470, 9.846743663894596210 ) ) ;
#97699=VERTEX_POINT ( 'NONE', #52154 ) ;
#97707=DIRECTION ( 'NONE',  ( -0.000000000000000000, -1.000000000000000000, -0.000000000000000000 ) ) ;
#97712=CARTESIAN_POINT ( 'NONE',  ( 3.434112377981054287, 22.66530133659709634, -12.81628187352647608 ) ) ;
#97713=VERTEX_POINT ( 'NONE', #51670 ) ;
#97714=AXIS2_PLACEMENT_3D ( 'NONE', #23806, #92765, #61768 ) ;
#97723=CIRCLE ( 'NONE', #37040, 15.00000000000000000 ) ;
#97725=CARTESIAN_POINT ( 'NONE',  ( -5.038135815954129626, 0.000000000000000000, 2.086864184045826853 ) ) ;
#97728=EDGE_CURVE ( 'NONE', #15789, #92979, #74652, .T. ) ;
#97729=DIRECTION ( 'NONE',  ( 0.9762960071199331402, -0.000000000000000000, 0.2164396139381037087 ) ) ;
#97732=LINE ( 'NONE', #29193, #10985 ) ;
#97733=DIRECTION ( 'NONE',  ( -0.000000000000000000, -1.000000000000000000, -0.000000000000000000 ) ) ;
#97740=CARTESIAN_POINT ( 'NONE',  ( -14.35840480524203855, 0.3640475087720986824, 4.340070442838750431 ) ) ;
#97744=CARTESIAN_POINT ( 'NONE',  ( -4.431036607602702126, 14.49999999999999112, 14.33059365769913462 ) ) ;
#97750=DIRECTION ( 'NONE',  ( -0.8616291604415232674, 0.000000000000000000, -0.5075383629607084224 ) ) ;
#97760=CARTESIAN_POINT ( 'NONE',  ( 13.40508947812163143, 15.00000000000000000, 5.527528931046191474 ) ) ;
#97768=CARTESIAN_POINT ( 'NONE',  ( 7.082119434687054849, 13.47041550158064460, 12.26659068614894288 ) ) ;
#97771=DIRECTION ( 'NONE',  ( 0.000000000000000000, 0.000000000000000000, 1.000000000000000000 ) ) ;
#97776=CARTESIAN_POINT ( 'NONE',  ( 0.000000000000000000, 15.00000000000000000, 0.000000000000000000 ) ) ;
#97789=ORIENTED_EDGE ( 'NONE', *, *, #38762, .T. ) ;
#97798=CARTESIAN_POINT ( 'NONE',  ( -12.25993886608613792, 0.3639311184075819106, 8.642563219313560197 ) ) ;
#97806=VECTOR ( 'NONE', #84460, 1000.000000000000114 ) ;
#97807=EDGE_CURVE ( 'NONE', #1901, #35164, #42010, .T. ) ;
#97810=CARTESIAN_POINT ( 'NONE',  ( -5.204170427930421283E-15, 6.671802177851543725, -11.25000000000000178 ) ) ;
#97815=LINE ( 'NONE', #60270, #43904 ) ;
#97816=EDGE_CURVE ( 'NONE', #42622, #48181, #11014, .T. ) ;
#97825=ORIENTED_EDGE ( 'NONE', *, *, #21255, .F. ) ;
#97832=VERTEX_POINT ( 'NONE', #33983 ) ;
#97834=ORIENTED_EDGE ( 'NONE', *, *, #70485, .F. ) ;
#97855=CARTESIAN_POINT ( 'NONE',  ( -8.375939845167836850, -0.03417435944610275333, 11.52849216984293257 ) ) ;
#97859=DIRECTION ( 'NONE',  ( 0.000000000000000000, 0.000000000000000000, -1.000000000000000000 ) ) ;
#97864=CIRCLE ( 'NONE', #54717, 15.00000000000000000 ) ;
#97867=DIRECTION ( 'NONE',  ( -0.000000000000000000, -1.000000000000000000, -0.000000000000000000 ) ) ;
#97868=CARTESIAN_POINT ( 'NONE',  ( -1.915564264621532287, 4.395349792408769378E-16, 14.37291249357989287 ) ) ;
#97874=ORIENTED_EDGE ( 'NONE', *, *, #7044, .F. ) ;
#97885=ORIENTED_EDGE ( 'NONE', *, *, #66413, .F. ) ;
#97886=CARTESIAN_POINT ( 'NONE',  ( -14.35840480524194440, 0.5000000000000004441, -4.340070442839038201 ) ) ;
#97888=EDGE_CURVE ( 'NONE', #97596, #26759, #41033, .T. ) ;
#97892=VECTOR ( 'NONE', #47767, 1000.000000000000000 ) ;
#97894=CARTESIAN_POINT ( 'NONE',  ( 0.000000000000000000, 14.49999999999999822, 0.000000000000000000 ) ) ;
#97896=EDGE_CURVE ( 'NONE', #46043, #57430, #68220, .T. ) ;
#97912=CARTESIAN_POINT ( 'NONE',  ( 0.000000000000000000, 15.00000000000000000, 0.000000000000000000 ) ) ;
#97913=CARTESIAN_POINT ( 'NONE',  ( 10.58981376305282041, -0.03417435944610275333, 9.535111140613782510 ) ) ;
#97926=TOROIDAL_SURFACE ( 'NONE', #72396, 14.49999999999999822, 0.5000000000000000000 ) ;
#97935=VECTOR ( 'NONE', #30590, 1000.000000000000000 ) ;
#97946=CARTESIAN_POINT ( 'NONE',  ( 10.58981376305288613, -0.03417435944610275333, -9.535111140613709679 ) ) ;
#97950=CARTESIAN_POINT ( 'NONE',  ( 0.000000000000000000, 15.00000000000000000, 0.000000000000000000 ) ) ;
#97955=ORIENTED_EDGE ( 'NONE', *, *, #70277, .T. ) ;
#97957=CARTESIAN_POINT ( 'NONE',  ( 6.408140936763236262, -22.54303199673624292, -11.09922568453595026 ) ) ;
#97958=ADVANCED_FACE ( 'NONE', ( #71534 ), #77315, .T. ) ;
#97961=CARTESIAN_POINT ( 'NONE',  ( 0.000000000000000000, 15.00000000000000000, 0.000000000000000000 ) ) ;
#97968=DIRECTION ( 'NONE',  ( 0.000000000000000000, 0.000000000000000000, 1.000000000000000000 ) ) ;
#97969=VERTEX_POINT ( 'NONE', #63515 ) ;
#97982=PLANE ( 'NONE',  #19560 ) ;
#97983=LINE ( 'NONE', #67959, #72916 ) ;
#97985=ORIENTED_EDGE ( 'NONE', *, *, #43014, .F. ) ;
#97987=CARTESIAN_POINT ( 'NONE',  ( 0.3093388210927780491, 0.3639309406664013036, 14.99680997725069531 ) ) ;
#98000=DIRECTION ( 'NONE',  ( -0.000000000000000000, -1.000000000000000000, -0.000000000000000000 ) ) ;
#98008=ADVANCED_FACE ( 'NONE', ( #18517 ), #11500, .F. ) ;
#98011=CARTESIAN_POINT ( 'NONE',  ( -7.082119434687044190, -22.36291783175269288, 12.26659068614894998 ) ) ;
#98015=ORIENTED_EDGE ( 'NONE', *, *, #76326, .F. ) ;
#98024=CARTESIAN_POINT ( 'NONE',  ( -10.88017736071110164, 22.85535201082150891, -2.915334737309917212 ) ) ;
#98029=CARTESIAN_POINT ( 'NONE',  ( -15.33206046421386759, -0.03417435944610275333, -4.561284726668966449 ) ) ;
#98030=ORIENTED_EDGE ( 'NONE', *, *, #22055, .T. ) ;
#98035=EDGE_CURVE ( 'NONE', #59012, #47538, #35958, .T. ) ;
#98054=LINE ( 'NONE', #14046, #36196 ) ;
#98057=EDGE_LOOP ( 'NONE', ( #86038, #51608, #86357, #28790, #30740, #41036 ) ) ;
#98071=CARTESIAN_POINT ( 'NONE',  ( 9.846743663894590881, 18.71726448433412315, -2.638427012816833894 ) ) ;
#98073=VERTEX_POINT ( 'NONE', #42497 ) ;
#98076=ORIENTED_EDGE ( 'NONE', *, *, #17240, .T. ) ;
#98083=EDGE_CURVE ( 'NONE', #48512, #67942, #2065, .T. ) ;
#98086=ORIENTED_EDGE ( 'NONE', *, *, #65153, .T. ) ;
#98095=CARTESIAN_POINT ( 'NONE',  ( 0.000000000000000000, 0.5000000000000004441, 0.000000000000000000 ) ) ;
#98104=DIRECTION ( 'NONE',  ( -0.000000000000000000, -1.000000000000000000, -0.000000000000000000 ) ) ;
#98108=CARTESIAN_POINT ( 'NONE',  ( 9.159723438033129383, 15.00000000000000000, 10.91613331444548507 ) ) ;
#98110=CARTESIAN_POINT ( 'NONE',  ( -3.195792623639464924, 5.729976035794186018, 11.92686044187660421 ) ) ;
#98112=DIRECTION ( 'NONE',  ( -4.707345624410664362E-14, 0.000000000000000000, 1.000000000000000000 ) ) ;
#98116=EDGE_CURVE ( 'NONE', #90692, #73812, #13475, .T. ) ;
#98118=CARTESIAN_POINT ( 'NONE',  ( 0.000000000000000000, 35.00000000000000000, 0.000000000000000000 ) ) ;
#98119=VECTOR ( 'NONE', #49991, 1000.000000000000114 ) ;
#98120=EDGE_LOOP ( 'NONE', ( #45173, #83286, #89562, #85226, #47101, #93213 ) ) ;
#98131=CARTESIAN_POINT ( 'NONE',  ( -14.35840480524194440, 0.5000000000000004441, -4.340070442839038201 ) ) ;
#98132=FACE_OUTER_BOUND ( 'NONE', #4198, .T. ) ;
#98136=CARTESIAN_POINT ( 'NONE',  ( -5.204170427930421283E-15, -18.18631465584515894, -10.88017736071110342 ) ) ;
#98139=EDGE_CURVE ( 'NONE', #74236, #11914, #58972, .T. ) ;
#98147=B_SPLINE_CURVE_WITH_KNOTS ( 'NONE', 3,
 ( #10673, #86185, #93176, #10190, #11651, #89125 ),
 .UNSPECIFIED., .F., .F.,
 ( 4, 2, 4 ),
 ( 3.409110551478550352E-05, 0.0004400426677366311512, 0.0008459942299584768260 ),
 .UNSPECIFIED. ) ;
#98148=EDGE_CURVE ( 'NONE', #41784, #62860, #69341, .T. ) ;
#98149=CARTESIAN_POINT ( 'NONE',  ( -12.35505582470280572, 15.00000000000000000, 10.16021613965622095 ) ) ;
#98155=ORIENTED_EDGE ( 'NONE', *, *, #76214, .F. ) ;
#98157=EDGE_CURVE ( 'NONE', #52889, #93734, #6462, .T. ) ;
#98158=FACE_OUTER_BOUND ( 'NONE', #62386, .T. ) ;
#98170=ORIENTED_EDGE ( 'NONE', *, *, #87102, .F. ) ;
#98172=CARTESIAN_POINT ( 'NONE',  ( 4.431036607602561794, 15.00000000000000000, -14.33059365769911153 ) ) ;
#98187=CARTESIAN_POINT ( 'NONE',  ( -9.846743663894590881, -28.78273551566588040, 2.638427012816840111 ) ) ;
#98188=ORIENTED_EDGE ( 'NONE', *, *, #28594, .F. ) ;
#98191=ORIENTED_EDGE ( 'NONE', *, *, #27880, .T. ) ;
#98200=DIRECTION ( 'NONE',  ( 0.000000000000000000, 0.000000000000000000, 1.000000000000000000 ) ) ;
#98204=CARTESIAN_POINT ( 'NONE',  ( -9.382169495545413795, 19.74863466993042138, 9.382169495545428006 ) ) ;
#98208=ORIENTED_EDGE ( 'NONE', *, *, #67989, .T. ) ;
#98217=ORIENTED_EDGE ( 'NONE', *, *, #3195, .T. ) ;
#98218=TOROIDAL_SURFACE ( 'NONE', #56651, 14.49999999999999822, 0.5000000000000000000 ) ;
#98222=DIRECTION ( 'NONE',  ( 0.000000000000000000, 0.000000000000000000, 1.000000000000000000 ) ) ;
#98224=FACE_OUTER_BOUND ( 'NONE', #53074, .T. ) ;
#98229=CARTESIAN_POINT ( 'NONE',  ( -11.62719953690055164, 14.49999999999999112, -9.476720473302012948 ) ) ;
#98244=DIRECTION ( 'NONE',  ( 0.000000000000000000, 1.000000000000000000, 0.000000000000000000 ) ) ;
#98246=EDGE_LOOP ( 'NONE', ( #18169, #63024, #93732, #74671 ) ) ;
#98249=EDGE_CURVE ( 'NONE', #51046, #40424, #4995, .T. ) ;
#98250=ORIENTED_EDGE ( 'NONE', *, *, #36018, .T. ) ;
#98258=CARTESIAN_POINT ( 'NONE',  ( 13.59972906620397026, 14.95037118612373384, 5.718800721548674915 ) ) ;
#98262=AXIS2_PLACEMENT_3D ( 'NONE', #94999, #35484, #64981 ) ;
#98265=CARTESIAN_POINT ( 'NONE',  ( 3.795296366450306547, 25.34541550158063927, -14.16423886937410259 ) ) ;
#98268=EDGE_CURVE ( 'NONE', #62480, #51116, #57385, .T. ) ;
#98269=CARTESIAN_POINT ( 'NONE',  ( -9.997910040112678587, 4.195612547371048347E-16, 10.50199004140710812 ) ) ;
#98272=ORIENTED_EDGE ( 'NONE', *, *, #15084, .T. ) ;
#98279=AXIS2_PLACEMENT_3D ( 'NONE', #83821, #75821, #31786 ) ;
#98283=ORIENTED_EDGE ( 'NONE', *, *, #41805, .T. ) ;
#98285=ADVANCED_FACE ( 'NONE', ( #90438 ), #21981, .T. ) ;
#98291=CARTESIAN_POINT ( 'NONE',  ( 0.000000000000000000, 0.5000000000000004441, 0.000000000000000000 ) ) ;
#98297=EDGE_CURVE ( 'NONE', #49746, #28421, #50482, .T. ) ;
#98302=CARTESIAN_POINT ( 'NONE',  ( 0.000000000000000000, 0.000000000000000000, -14.25000000000000000 ) ) ;
#98312=CARTESIAN_POINT ( 'NONE',  ( 3.469446951953614189E-15, 9.171802177851546389, 11.25000000000000355 ) ) ;
#98315=ORIENTED_EDGE ( 'NONE', *, *, #98297, .F. ) ;
#98320=AXIS2_PLACEMENT_3D ( 'NONE', #81727, #34751, #42760 ) ;
#98329=ORIENTED_EDGE ( 'NONE', *, *, #1387, .T. ) ;
#98339=EDGE_CURVE ( 'NONE', #60281, #13116, #6226, .T. ) ;
#98340=AXIS2_PLACEMENT_3D ( 'NONE', #85927, #70431, #9424 ) ;
#98344=CARTESIAN_POINT ( 'NONE',  ( -1.175527996597229841, 6.200281173901476510E-16, 14.57931687975697876 ) ) ;
#98352=FACE_OUTER_BOUND ( 'NONE', #77098, .T. ) ;
#98363=EDGE_LOOP ( 'NONE', ( #45294, #17733, #68201, #16549 ) ) ;
#98372=DIRECTION ( 'NONE',  ( 0.000000000000000000, 1.000000000000000000, 0.000000000000000000 ) ) ;
#98383=AXIS2_PLACEMENT_3D ( 'NONE', #12534, #42540, #73024 ) ;
#98384=FACE_OUTER_BOUND ( 'NONE', #71480, .T. ) ;
#98386=CARTESIAN_POINT ( 'NONE',  ( 0.000000000000000000, 14.49999999999999822, 0.000000000000000000 ) ) ;
#98395=CARTESIAN_POINT ( 'NONE',  ( 4.391700990647064984, 14.76930270348882956, 14.28114200970192016 ) ) ;
#98401=ORIENTED_EDGE ( 'NONE', *, *, #51744, .F. ) ;
#98402=EDGE_CURVE ( 'NONE', #86489, #52526, #91934, .T. ) ;
#98408=DIRECTION ( 'NONE',  ( 1.545430450278217904E-13, 0.000000000000000000, 1.000000000000000000 ) ) ;
#98409=LINE ( 'NONE', #58894, #6466 ) ;
#98413=CARTESIAN_POINT ( 'NONE',  ( 4.880290883660320489, 0.000000000000000000, 2.433223276543894364 ) ) ;
#98414=CARTESIAN_POINT ( 'NONE',  ( 14.97687855664607781, 0.5000000000000004441, 0.8325315005901553489 ) ) ;
#98418=VECTOR ( 'NONE', #7680, 1000.000000000000114 ) ;
#98433=VERTEX_POINT ( 'NONE', #60446 ) ;
#98439=EDGE_LOOP ( 'NONE', ( #34695, #19016, #72204, #66863 ) ) ;
#98441=PLANE ( 'NONE',  #48221 ) ;
#98446=CARTESIAN_POINT ( 'NONE',  ( -15.41943733314634635, 15.00000000000000000, 4.256565371896233962 ) ) ;
#98451=ORIENTED_EDGE ( 'NONE', *, *, #98463, .F. ) ;
#98453=CARTESIAN_POINT ( 'NONE',  ( 12.81628187352647608, -23.37636533006957507, -2.602085213965210642E-15 ) ) ;
#98463=EDGE_CURVE ( 'NONE', #48799, #24087, #17812, .T. ) ;
#98465=FACE_OUTER_BOUND ( 'NONE', #7086, .T. ) ;
#98476=CARTESIAN_POINT ( 'NONE',  ( 14.88585913060025945, 14.76984981697140142, -1.278057234793439800 ) ) ;
#98484=ORIENTED_EDGE ( 'NONE', *, *, #18200, .T. ) ;
#98486=EDGE_CURVE ( 'NONE', #55365, #22543, #77569, .T. ) ;
#98499=CARTESIAN_POINT ( 'NONE',  ( -9.742785792574940373, 9.701366962315987053, -5.624999999999991118 ) ) ;
#98503=VECTOR ( 'NONE', #285, 999.9999999999998863 ) ;
#98507=CARTESIAN_POINT ( 'NONE',  ( 14.26139399674457309, 4.693468746458063789E-16, -2.619664342929806988 ) ) ;
#98510=CARTESIAN_POINT ( 'NONE',  ( 14.16423886937410259, -25.69625116508602858, -2.602085213965210642E-15 ) ) ;
#98516=ORIENTED_EDGE ( 'NONE', *, *, #15946, .F. ) ;
#98522=FACE_OUTER_BOUND ( 'NONE', #47458, .T. ) ;
#98528=CARTESIAN_POINT ( 'NONE',  ( 7.964842623401177768, 31.18868534415484461, -7.964842623401181321 ) ) ;
#98534=ORIENTED_EDGE ( 'NONE', *, *, #95617, .T. ) ;
#98535=EDGE_CURVE ( 'NONE', #70022, #1146, #70999, .T. ) ;
#98538=LINE ( 'NONE', #91495, #59270 ) ;
#98557=DIRECTION ( 'NONE',  ( 0.000000000000000000, 1.000000000000000000, 0.000000000000000000 ) ) ;
#98559=CARTESIAN_POINT ( 'NONE',  ( 6.336100170400922771, 14.76984879808201434, -13.53056138701887967 ) ) ;
#98562=ORIENTED_EDGE ( 'NONE', *, *, #88208, .T. ) ;
#98567=CARTESIAN_POINT ( 'NONE',  ( 4.096035146093531587, 15.00000000000000000, -13.90943910019259278 ) ) ;
#98578=CARTESIAN_POINT ( 'NONE',  ( -8.527530157486173934, 16.42559781766746241, 4.923371831947302546 ) ) ;
#98579=AXIS2_PLACEMENT_3D ( 'NONE', #47765, #96110, #40766 ) ;
#98580=ORIENTED_EDGE ( 'NONE', *, *, #68707, .F. ) ;
#98583=EDGE_LOOP ( 'NONE', ( #77627, #87983, #96351, #84697 ) ) ;
#98591=EDGE_CURVE ( 'NONE', #48625, #24045, #37473, .T. ) ;
#98592=VECTOR ( 'NONE', #46552, 999.9999999999998863 ) ;
#98594=EDGE_LOOP ( 'NONE', ( #94833, #8643, #81671, #84067, #82794, #76561 ) ) ;
#98599=ORIENTED_EDGE ( 'NONE', *, *, #74975, .T. ) ;
#98610=ORIENTED_EDGE ( 'NONE', *, *, #39906, .F. ) ;
#98611=CARTESIAN_POINT ( 'NONE',  ( 1.983216688680936812, 15.00000000000000000, -14.11131997956737649 ) ) ;
#98617=CARTESIAN_POINT ( 'NONE',  ( 4.431036607602466759, 15.00000000000000000, 14.33059365769913818 ) ) ;
#98618=DIRECTION ( 'NONE',  ( -0.000000000000000000, -1.000000000000000000, -0.000000000000000000 ) ) ;
#98622=CARTESIAN_POINT ( 'NONE',  ( 11.62719953690066355, 0.3639310419529870333, -9.476720473301831760 ) ) ;
#98624=CARTESIAN_POINT ( 'NONE',  ( 6.761389522993885848, 14.76930270348881002, -13.32372569557300146 ) ) ;
#98629=DIRECTION ( 'NONE',  ( 0.000000000000000000, 0.000000000000000000, 1.000000000000000000 ) ) ;
#98639=B_SPLINE_CURVE_WITH_KNOTS ( 'NONE', 3,
 ( #23223, #76211, #68709, #30688, #76690, #59216 ),
 .UNSPECIFIED., .F., .F.,
 ( 4, 2, 4 ),
 ( 0.0002800124554063431175, 0.0006862178066574521314, 0.001092423157908561145 ),
 .UNSPECIFIED. ) ;
#98640=CARTESIAN_POINT ( 'NONE',  ( 7.109031286574862385, 14.95037114371795894, -12.92745085449638509 ) ) ;
#98641=EDGE_CURVE ( 'NONE', #93159, #57516, #14973, .T. ) ;
#98645=CARTESIAN_POINT ( 'NONE',  ( 9.422509992056141925, -9.019647989178487535, -5.440088680355554374 ) ) ;
#98649=CARTESIAN_POINT ( 'NONE',  ( 14.97687855664608314, 0.3640475087720990155, 0.8325315005901587906 ) ) ;
#98650=AXIS2_PLACEMENT_3D ( 'NONE', #46337, #76823, #69834 ) ;
#98651=EDGE_CURVE ( 'NONE', #46867, #48771, #64458, .T. ) ;
#98653=DIRECTION ( 'NONE',  ( -0.000000000000000000, -1.000000000000000000, -0.000000000000000000 ) ) ;
#98666=DIRECTION ( 'NONE',  ( 0.000000000000000000, 0.000000000000000000, 1.000000000000000000 ) ) ;
#98675=ORIENTED_EDGE ( 'NONE', *, *, #68407, .T. ) ;
#98676=VERTEX_POINT ( 'NONE', #39922 ) ;
#98690=CARTESIAN_POINT ( 'NONE',  ( 2.638427012816829897, -30.44940218233254825, -9.846743663894592657 ) ) ;
#98691=ORIENTED_EDGE ( 'NONE', *, *, #67760, .F. ) ;
#98693=VERTEX_POINT ( 'NONE', #95375 ) ;
#98695=VERTEX_POINT ( 'NONE', #2439 ) ;
#98696=CARTESIAN_POINT ( 'NONE',  ( -0.7577696756377649834, 0.2301502180065688186, 14.92139465029743839 ) ) ;
#98702=EDGE_CURVE ( 'NONE', #19349, #91342, #64371, .T. ) ;
#98703=CONICAL_SURFACE ( 'NONE', #22028, 11.25000000000000178, 0.7853981633974497223 ) ;
#98706=CARTESIAN_POINT ( 'NONE',  ( -11.09922568453595382, 23.70696800326376064, -6.408140936763226492 ) ) ;
#98707=ORIENTED_EDGE ( 'NONE', *, *, #17287, .T. ) ;
#98709=ORIENTED_EDGE ( 'NONE', *, *, #3851, .T. ) ;
#98711=ORIENTED_EDGE ( 'NONE', *, *, #57984, .T. ) ;
#98721=TOROIDAL_SURFACE ( 'NONE', #12464, 14.49999999999999822, 0.5000000000000000000 ) ;
#98722=CARTESIAN_POINT ( 'NONE',  ( 7.108715748589172101, 0.04922511925147215334, -12.92719074505367161 ) ) ;
#98733=CARTESIAN_POINT ( 'NONE',  ( 5.803070148808231465, 3.918713670743053586E-16, 13.28812917035392260 ) ) ;
#98736=CARTESIAN_POINT ( 'NONE',  ( -14.09356342482601043, 0.04922511925147129291, 4.360913911515280184 ) ) ;
#98740=B_SPLINE_CURVE_WITH_KNOTS ( 'NONE', 3,
 ( #63252, #70290, #25773, #56267, #32262, #25290 ),
 .UNSPECIFIED., .F., .F.,
 ( 4, 2, 4 ),
 ( 3.409110551493946023E-05, 0.0004400426677367865174, 0.0008459942299586336017 ),
 .UNSPECIFIED. ) ;
#98741=CARTESIAN_POINT ( 'NONE',  ( -9.402796353261210882, 14.63595249122789177, 11.68706210897751951 ) ) ;
#98750=ORIENTED_EDGE ( 'NONE', *, *, #80288, .T. ) ;
#98763=CARTESIAN_POINT ( 'NONE',  ( -7.082119434687058401, 25.97041550158063572, -12.26659068614894110 ) ) ;
#98766=CARTESIAN_POINT ( 'NONE',  ( -10.09792486685197943, 0.04962894416274191839, 10.75589247084405109 ) ) ;
#98771=DIRECTION ( 'NONE',  ( 0.000000000000000000, 0.000000000000000000, -1.000000000000000000 ) ) ;
#98778=CARTESIAN_POINT ( 'NONE',  ( -14.03351048042399007, -0.03417435944610275333, 2.474486531753619989 ) ) ;
#98798=ORIENTED_EDGE ( 'NONE', *, *, #89195, .F. ) ;
#98801=CARTESIAN_POINT ( 'NONE',  ( 8.564643372776615138, 0.5000000000000004441, -12.31449893000740836 ) ) ;
#98826=ORIENTED_EDGE ( 'NONE', *, *, #9396, .F. ) ;
#98827=VERTEX_POINT ( 'NONE', #20368 ) ;
#98830=AXIS2_PLACEMENT_3D ( 'NONE', #46721, #9715, #85228 ) ;
#98836=CARTESIAN_POINT ( 'NONE',  ( 11.96291822454881348, 3.986488846351010315E-16, -8.193813980849080636 ) ) ;
#98850=LINE ( 'NONE', #69310, #6913 ) ;
#98855=AXIS2_PLACEMENT_3D ( 'NONE', #70630, #86125, #2159 ) ;
#98859=ORIENTED_EDGE ( 'NONE', *, *, #60675, .T. ) ;
#98860=AXIS2_PLACEMENT_3D ( 'NONE', #89923, #43921, #27937 ) ;
#98862=FACE_OUTER_BOUND ( 'NONE', #66822, .T. ) ;
#98872=LINE ( 'NONE', #76817, #84595 ) ;
#98876=CARTESIAN_POINT ( 'NONE',  ( -2.518025504887116739, 0.000000000000000000, 4.837081990145610355 ) ) ;
#98886=VERTEX_POINT ( 'NONE', #36350 ) ;
#98890=CARTESIAN_POINT ( 'NONE',  ( 4.431036607602467647, 14.49999999999999822, 14.33059365769914351 ) ) ;
#98896=VERTEX_POINT ( 'NONE', #80867 ) ;
#98897=DIRECTION ( 'NONE',  ( 0.000000000000000000, 0.000000000000000000, 1.000000000000000000 ) ) ;
#98898=CARTESIAN_POINT ( 'NONE',  ( -11.35178980618961830, 14.63595249122790065, -9.804941009312081235 ) ) ;
#98903=CARTESIAN_POINT ( 'NONE',  ( 9.876730923139335871, 14.63606899087332991, -11.28938378619065297 ) ) ;
#98909=CARTESIAN_POINT ( 'NONE',  ( -3.270119481323481736, 14.95077488074853456, -14.38584091150425337 ) ) ;
#98911=ADVANCED_FACE ( 'NONE', ( #51845 ), #4879, .T. ) ;
#98919=CARTESIAN_POINT ( 'NONE',  ( 13.61464873478162652, 0.5000000000000004441, 6.296136897217931683 ) ) ;
#98925=ORIENTED_EDGE ( 'NONE', *, *, #38845, .F. ) ;
#98926=ADVANCED_FACE ( 'NONE', ( #74331 ), #88858, .T. ) ;
#98929=VECTOR ( 'NONE', #23554, 1000.000000000000000 ) ;
#98938=DIRECTION ( 'NONE',  ( 0.6626200482157357241, 0.000000000000000000, 0.7489557207890036317 ) ) ;
#98942=DIRECTION ( 'NONE',  ( -0.000000000000000000, -1.000000000000000000, -0.000000000000000000 ) ) ;
#98944=CARTESIAN_POINT ( 'NONE',  ( 4.873787042390789637, 0.000000000000000000, -13.39061984619918988 ) ) ;
#98948=CARTESIAN_POINT ( 'NONE',  ( 6.408140936763236262, -7.543031996736241140, -11.09922568453595026 ) ) ;
#98952=CARTESIAN_POINT ( 'NONE',  ( 0.000000000000000000, 14.49999999999999822, 0.000000000000000000 ) ) ;
#98960=ORIENTED_EDGE ( 'NONE', *, *, #55564, .T. ) ;
#98965=EDGE_CURVE ( 'NONE', #88314, #13980, #19134, .T. ) ;
#98966=VERTEX_POINT ( 'NONE', #21353 ) ;
#98973=DIRECTION ( 'NONE',  ( 0.000000000000000000, 1.000000000000000000, 0.000000000000000000 ) ) ;
#98976=DIRECTION ( 'NONE',  ( 0.000000000000000000, 1.000000000000000000, -0.000000000000000000 ) ) ;
#98985=CARTESIAN_POINT ( 'NONE',  ( -14.40939250469967448, 4.171366831970869137E-16, 1.618458416365661012 ) ) ;
ENDSEC;
END-ISO-10303-21;
